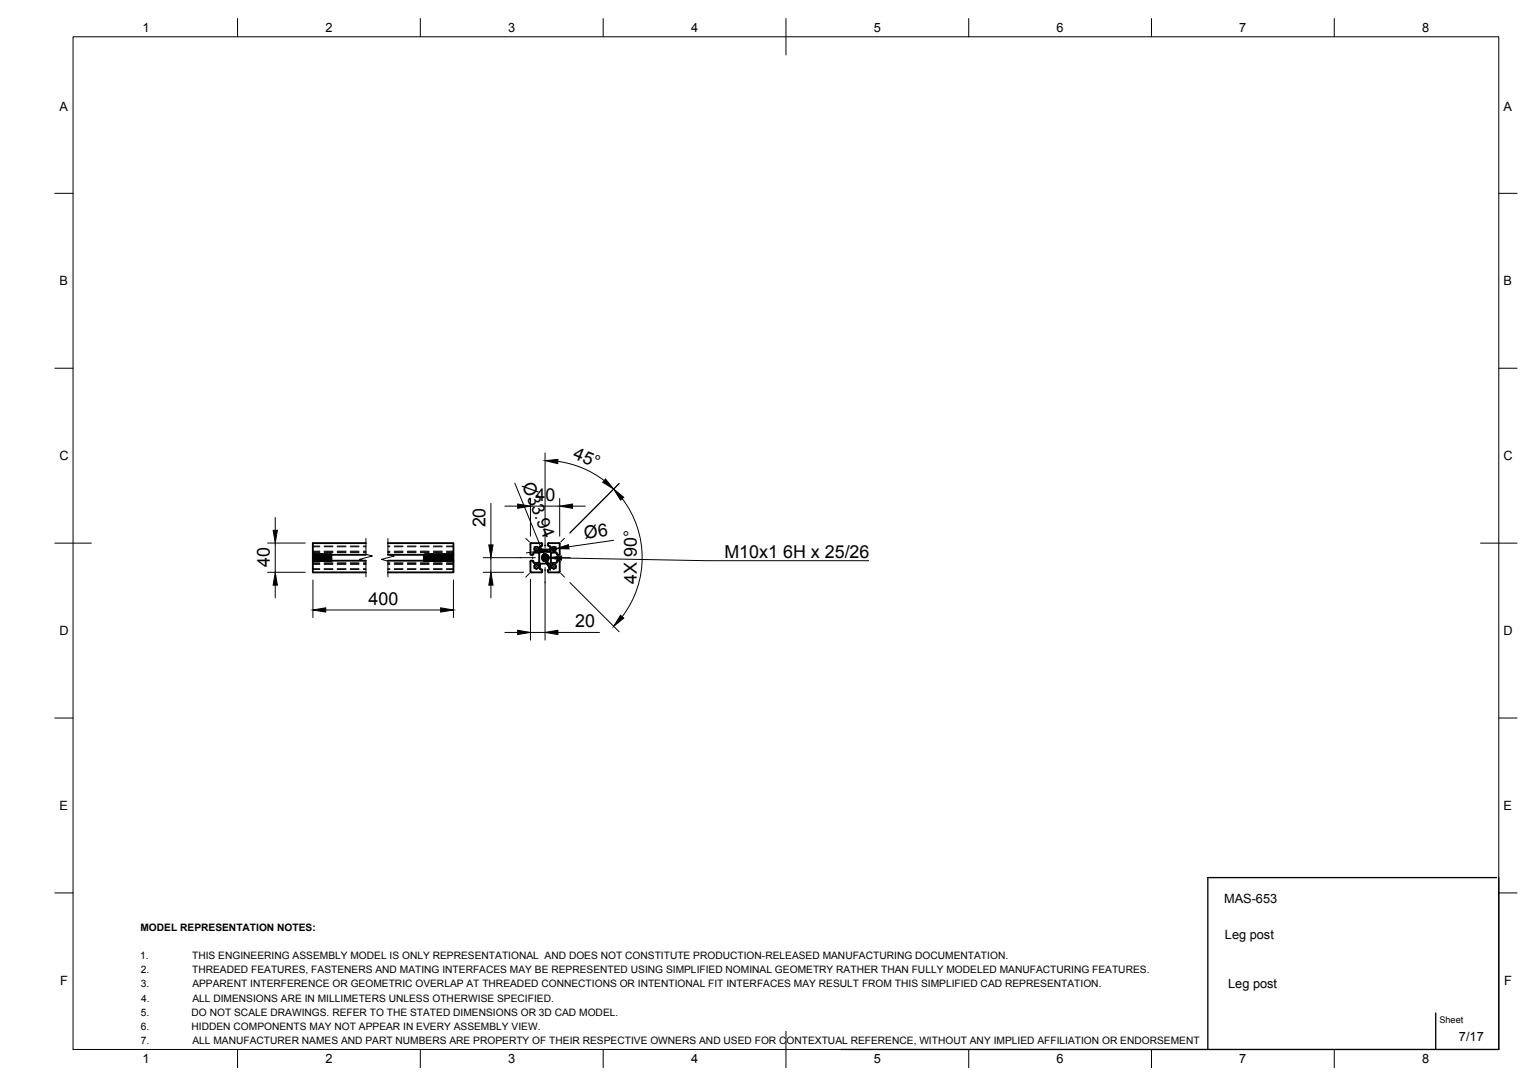
ISO-10303-21;
HEADER;
/* Generated by software containing ST-Developer
 * from STEP Tools, Inc. (www.steptools.com) 
 */

FILE_DESCRIPTION(
/* description */ ('Independent compact industrial fixture table, bolted aluminum worktop
 on connected adjustable support base. Whole-mm nominal dimensions. No
 load rating assigned.'),
/* implementation_level */ '2;1');

FILE_NAME(
/* name */ 'Leg post.step',
/* time_stamp */ '2026-11-07T17:47:58-08:00',
/* author */ (''),
/* organization */ (''),
/* preprocessor_version */ 'ST-DEVELOPER v20.2',
/* originating_system */ 'Autodesk Translation Framework v15.17.0.0',
/* authorisation */ '');

FILE_SCHEMA (('AUTOMOTIVE_DESIGN { 1 0 10303 214 3 1 1 }'));
ENDSEC;

DATA;
#10=MECHANICAL_DESIGN_GEOMETRIC_PRESENTATION_REPRESENTATION('',(#2255),#97475);
#344=B_SPLINE_SURFACE_WITH_KNOTS('',3,3,((#45406,#45407,#45408,#45409,#45410,
#45411,#45412,#45413,#45414,#45415,#45416,#45417,#45418,#45419,#45420,#45421,
#45422,#45423,#45424,#45425,#45426,#45427,#45428,#45429,#45430,#45431,#45432,
#45433,#45434,#45435,#45436,#45437,#45438,#45439,#45440,#45441,#45442,#45443,
#45444,#45445,#45446,#45447,#45448,#45449,#45450,#45451,#45452,#45453,#45454,
#45455,#45456,#45457,#45458,#45459,#45460,#45461,#45462,#45463,#45464,#45465,
#45466,#45467,#45468,#45469,#45470,#45471,#45472,#45473,#45474,#45475,#45476,
#45477,#45478,#45479,#45480,#45481,#45482,#45483,#45484,#45485,#45486,#45487,
#45488,#45489,#45490,#45491,#45492,#45493,#45494,#45495,#45496,#45497,#45498,
#45499,#45500,#45501,#45502,#45503,#45504,#45505,#45506,#45507,#45508,#45509,
#45510,#45511,#45512,#45513,#45514,#45515,#45516,#45517,#45518,#45519,#45520,
#45521,#45522,#45523,#45524,#45525,#45526,#45527,#45528,#45529,#45530,#45531,
#45532,#45533,#45534,#45535,#45536,#45537,#45538,#45539,#45540,#45541,#45542,
#45543,#45544,#45545,#45546,#45547,#45548,#45549,#45550,#45551,#45552,#45553,
#45554,#45555,#45556,#45557,#45558,#45559,#45560,#45561,#45562,#45563,#45564,
#45565,#45566,#45567,#45568,#45569,#45570,#45571,#45572,#45573,#45574,#45575,
#45576,#45577,#45578,#45579,#45580,#45581,#45582,#45583,#45584,#45585,#45586,
#45587,#45588,#45589,#45590,#45591,#45592,#45593,#45594,#45595,#45596,#45597,
#45598,#45599,#45600,#45601,#45602,#45603,#45604,#45605,#45606,#45607,#45608,
#45609,#45610,#45611,#45612,#45613,#45614,#45615,#45616,#45617,#45618,#45619,
#45620,#45621,#45622,#45623,#45624,#45625,#45626,#45627,#45628,#45629,#45630,
#45631,#45632,#45633,#45634,#45635,#45636,#45637,#45638,#45639,#45640,#45641,
#45642,#45643,#45644,#45645,#45646,#45647,#45648,#45649,#45650,#45651,#45652,
#45653,#45654,#45655,#45656,#45657,#45658,#45659,#45660,#45661,#45662,#45663,
#45664,#45665,#45666,#45667,#45668,#45669,#45670,#45671,#45672,#45673,#45674,
#45675,#45676,#45677,#45678,#45679,#45680,#45681,#45682,#45683,#45684,#45685,
#45686,#45687,#45688,#45689,#45690,#45691,#45692,#45693,#45694,#45695,#45696,
#45697,#45698,#45699,#45700,#45701,#45702,#45703,#45704,#45705,#45706,#45707,
#45708,#45709,#45710,#45711,#45712,#45713,#45714,#45715,#45716,#45717,#45718,
#45719,#45720,#45721,#45722,#45723,#45724,#45725,#45726,#45727,#45728,#45729,
#45730,#45731,#45732,#45733,#45734,#45735,#45736,#45737,#45738,#45739,#45740,
#45741,#45742,#45743,#45744,#45745,#45746,#45747,#45748,#45749,#45750,#45751,
#45752,#45753,#45754,#45755,#45756,#45757,#45758,#45759,#45760,#45761,#45762,
#45763,#45764,#45765,#45766,#45767,#45768,#45769,#45770,#45771,#45772,#45773,
#45774,#45775,#45776,#45777,#45778,#45779,#45780,#45781,#45782,#45783,#45784,
#45785,#45786,#45787,#45788,#45789,#45790,#45791,#45792,#45793,#45794,#45795,
#45796,#45797,#45798,#45799,#45800,#45801,#45802,#45803,#45804,#45805,#45806,
#45807,#45808,#45809,#45810,#45811,#45812,#45813,#45814,#45815,#45816,#45817,
#45818,#45819,#45820,#45821,#45822,#45823,#45824,#45825,#45826,#45827,#45828,
#45829,#45830,#45831,#45832,#45833,#45834,#45835,#45836,#45837,#45838,#45839,
#45840,#45841,#45842,#45843,#45844,#45845,#45846,#45847,#45848,#45849,#45850,
#45851,#45852,#45853,#45854,#45855,#45856,#45857,#45858,#45859,#45860,#45861,
#45862,#45863,#45864,#45865,#45866,#45867,#45868,#45869,#45870,#45871,#45872,
#45873,#45874,#45875,#45876,#45877,#45878,#45879,#45880,#45881,#45882,#45883,
#45884,#45885,#45886,#45887,#45888,#45889,#45890,#45891,#45892,#45893,#45894,
#45895,#45896,#45897,#45898,#45899,#45900,#45901,#45902),(#45903,#45904,
#45905,#45906,#45907,#45908,#45909,#45910,#45911,#45912,#45913,#45914,#45915,
#45916,#45917,#45918,#45919,#45920,#45921,#45922,#45923,#45924,#45925,#45926,
#45927,#45928,#45929,#45930,#45931,#45932,#45933,#45934,#45935,#45936,#45937,
#45938,#45939,#45940,#45941,#45942,#45943,#45944,#45945,#45946,#45947,#45948,
#45949,#45950,#45951,#45952,#45953,#45954,#45955,#45956,#45957,#45958,#45959,
#45960,#45961,#45962,#45963,#45964,#45965,#45966,#45967,#45968,#45969,#45970,
#45971,#45972,#45973,#45974,#45975,#45976,#45977,#45978,#45979,#45980,#45981,
#45982,#45983,#45984,#45985,#45986,#45987,#45988,#45989,#45990,#45991,#45992,
#45993,#45994,#45995,#45996,#45997,#45998,#45999,#46000,#46001,#46002,#46003,
#46004,#46005,#46006,#46007,#46008,#46009,#46010,#46011,#46012,#46013,#46014,
#46015,#46016,#46017,#46018,#46019,#46020,#46021,#46022,#46023,#46024,#46025,
#46026,#46027,#46028,#46029,#46030,#46031,#46032,#46033,#46034,#46035,#46036,
#46037,#46038,#46039,#46040,#46041,#46042,#46043,#46044,#46045,#46046,#46047,
#46048,#46049,#46050,#46051,#46052,#46053,#46054,#46055,#46056,#46057,#46058,
#46059,#46060,#46061,#46062,#46063,#46064,#46065,#46066,#46067,#46068,#46069,
#46070,#46071,#46072,#46073,#46074,#46075,#46076,#46077,#46078,#46079,#46080,
#46081,#46082,#46083,#46084,#46085,#46086,#46087,#46088,#46089,#46090,#46091,
#46092,#46093,#46094,#46095,#46096,#46097,#46098,#46099,#46100,#46101,#46102,
#46103,#46104,#46105,#46106,#46107,#46108,#46109,#46110,#46111,#46112,#46113,
#46114,#46115,#46116,#46117,#46118,#46119,#46120,#46121,#46122,#46123,#46124,
#46125,#46126,#46127,#46128,#46129,#46130,#46131,#46132,#46133,#46134,#46135,
#46136,#46137,#46138,#46139,#46140,#46141,#46142,#46143,#46144,#46145,#46146,
#46147,#46148,#46149,#46150,#46151,#46152,#46153,#46154,#46155,#46156,#46157,
#46158,#46159,#46160,#46161,#46162,#46163,#46164,#46165,#46166,#46167,#46168,
#46169,#46170,#46171,#46172,#46173,#46174,#46175,#46176,#46177,#46178,#46179,
#46180,#46181,#46182,#46183,#46184,#46185,#46186,#46187,#46188,#46189,#46190,
#46191,#46192,#46193,#46194,#46195,#46196,#46197,#46198,#46199,#46200,#46201,
#46202,#46203,#46204,#46205,#46206,#46207,#46208,#46209,#46210,#46211,#46212,
#46213,#46214,#46215,#46216,#46217,#46218,#46219,#46220,#46221,#46222,#46223,
#46224,#46225,#46226,#46227,#46228,#46229,#46230,#46231,#46232,#46233,#46234,
#46235,#46236,#46237,#46238,#46239,#46240,#46241,#46242,#46243,#46244,#46245,
#46246,#46247,#46248,#46249,#46250,#46251,#46252,#46253,#46254,#46255,#46256,
#46257,#46258,#46259,#46260,#46261,#46262,#46263,#46264,#46265,#46266,#46267,
#46268,#46269,#46270,#46271,#46272,#46273,#46274,#46275,#46276,#46277,#46278,
#46279,#46280,#46281,#46282,#46283,#46284,#46285,#46286,#46287,#46288,#46289,
#46290,#46291,#46292,#46293,#46294,#46295,#46296,#46297,#46298,#46299,#46300,
#46301,#46302,#46303,#46304,#46305,#46306,#46307,#46308,#46309,#46310,#46311,
#46312,#46313,#46314,#46315,#46316,#46317,#46318,#46319,#46320,#46321,#46322,
#46323,#46324,#46325,#46326,#46327,#46328,#46329,#46330,#46331,#46332,#46333,
#46334,#46335,#46336,#46337,#46338,#46339,#46340,#46341,#46342,#46343,#46344,
#46345,#46346,#46347,#46348,#46349,#46350,#46351,#46352,#46353,#46354,#46355,
#46356,#46357,#46358,#46359,#46360,#46361,#46362,#46363,#46364,#46365,#46366,
#46367,#46368,#46369,#46370,#46371,#46372,#46373,#46374,#46375,#46376,#46377,
#46378,#46379,#46380,#46381,#46382,#46383,#46384,#46385,#46386,#46387,#46388,
#46389,#46390,#46391,#46392,#46393,#46394,#46395,#46396,#46397,#46398,#46399),
(#46400,#46401,#46402,#46403,#46404,#46405,#46406,#46407,#46408,#46409,
#46410,#46411,#46412,#46413,#46414,#46415,#46416,#46417,#46418,#46419,#46420,
#46421,#46422,#46423,#46424,#46425,#46426,#46427,#46428,#46429,#46430,#46431,
#46432,#46433,#46434,#46435,#46436,#46437,#46438,#46439,#46440,#46441,#46442,
#46443,#46444,#46445,#46446,#46447,#46448,#46449,#46450,#46451,#46452,#46453,
#46454,#46455,#46456,#46457,#46458,#46459,#46460,#46461,#46462,#46463,#46464,
#46465,#46466,#46467,#46468,#46469,#46470,#46471,#46472,#46473,#46474,#46475,
#46476,#46477,#46478,#46479,#46480,#46481,#46482,#46483,#46484,#46485,#46486,
#46487,#46488,#46489,#46490,#46491,#46492,#46493,#46494,#46495,#46496,#46497,
#46498,#46499,#46500,#46501,#46502,#46503,#46504,#46505,#46506,#46507,#46508,
#46509,#46510,#46511,#46512,#46513,#46514,#46515,#46516,#46517,#46518,#46519,
#46520,#46521,#46522,#46523,#46524,#46525,#46526,#46527,#46528,#46529,#46530,
#46531,#46532,#46533,#46534,#46535,#46536,#46537,#46538,#46539,#46540,#46541,
#46542,#46543,#46544,#46545,#46546,#46547,#46548,#46549,#46550,#46551,#46552,
#46553,#46554,#46555,#46556,#46557,#46558,#46559,#46560,#46561,#46562,#46563,
#46564,#46565,#46566,#46567,#46568,#46569,#46570,#46571,#46572,#46573,#46574,
#46575,#46576,#46577,#46578,#46579,#46580,#46581,#46582,#46583,#46584,#46585,
#46586,#46587,#46588,#46589,#46590,#46591,#46592,#46593,#46594,#46595,#46596,
#46597,#46598,#46599,#46600,#46601,#46602,#46603,#46604,#46605,#46606,#46607,
#46608,#46609,#46610,#46611,#46612,#46613,#46614,#46615,#46616,#46617,#46618,
#46619,#46620,#46621,#46622,#46623,#46624,#46625,#46626,#46627,#46628,#46629,
#46630,#46631,#46632,#46633,#46634,#46635,#46636,#46637,#46638,#46639,#46640,
#46641,#46642,#46643,#46644,#46645,#46646,#46647,#46648,#46649,#46650,#46651,
#46652,#46653,#46654,#46655,#46656,#46657,#46658,#46659,#46660,#46661,#46662,
#46663,#46664,#46665,#46666,#46667,#46668,#46669,#46670,#46671,#46672,#46673,
#46674,#46675,#46676,#46677,#46678,#46679,#46680,#46681,#46682,#46683,#46684,
#46685,#46686,#46687,#46688,#46689,#46690,#46691,#46692,#46693,#46694,#46695,
#46696,#46697,#46698,#46699,#46700,#46701,#46702,#46703,#46704,#46705,#46706,
#46707,#46708,#46709,#46710,#46711,#46712,#46713,#46714,#46715,#46716,#46717,
#46718,#46719,#46720,#46721,#46722,#46723,#46724,#46725,#46726,#46727,#46728,
#46729,#46730,#46731,#46732,#46733,#46734,#46735,#46736,#46737,#46738,#46739,
#46740,#46741,#46742,#46743,#46744,#46745,#46746,#46747,#46748,#46749,#46750,
#46751,#46752,#46753,#46754,#46755,#46756,#46757,#46758,#46759,#46760,#46761,
#46762,#46763,#46764,#46765,#46766,#46767,#46768,#46769,#46770,#46771,#46772,
#46773,#46774,#46775,#46776,#46777,#46778,#46779,#46780,#46781,#46782,#46783,
#46784,#46785,#46786,#46787,#46788,#46789,#46790,#46791,#46792,#46793,#46794,
#46795,#46796,#46797,#46798,#46799,#46800,#46801,#46802,#46803,#46804,#46805,
#46806,#46807,#46808,#46809,#46810,#46811,#46812,#46813,#46814,#46815,#46816,
#46817,#46818,#46819,#46820,#46821,#46822,#46823,#46824,#46825,#46826,#46827,
#46828,#46829,#46830,#46831,#46832,#46833,#46834,#46835,#46836,#46837,#46838,
#46839,#46840,#46841,#46842,#46843,#46844,#46845,#46846,#46847,#46848,#46849,
#46850,#46851,#46852,#46853,#46854,#46855,#46856,#46857,#46858,#46859,#46860,
#46861,#46862,#46863,#46864,#46865,#46866,#46867,#46868,#46869,#46870,#46871,
#46872,#46873,#46874,#46875,#46876,#46877,#46878,#46879,#46880,#46881,#46882,
#46883,#46884,#46885,#46886,#46887,#46888,#46889,#46890,#46891,#46892,#46893,
#46894,#46895,#46896),(#46897,#46898,#46899,#46900,#46901,#46902,#46903,
#46904,#46905,#46906,#46907,#46908,#46909,#46910,#46911,#46912,#46913,#46914,
#46915,#46916,#46917,#46918,#46919,#46920,#46921,#46922,#46923,#46924,#46925,
#46926,#46927,#46928,#46929,#46930,#46931,#46932,#46933,#46934,#46935,#46936,
#46937,#46938,#46939,#46940,#46941,#46942,#46943,#46944,#46945,#46946,#46947,
#46948,#46949,#46950,#46951,#46952,#46953,#46954,#46955,#46956,#46957,#46958,
#46959,#46960,#46961,#46962,#46963,#46964,#46965,#46966,#46967,#46968,#46969,
#46970,#46971,#46972,#46973,#46974,#46975,#46976,#46977,#46978,#46979,#46980,
#46981,#46982,#46983,#46984,#46985,#46986,#46987,#46988,#46989,#46990,#46991,
#46992,#46993,#46994,#46995,#46996,#46997,#46998,#46999,#47000,#47001,#47002,
#47003,#47004,#47005,#47006,#47007,#47008,#47009,#47010,#47011,#47012,#47013,
#47014,#47015,#47016,#47017,#47018,#47019,#47020,#47021,#47022,#47023,#47024,
#47025,#47026,#47027,#47028,#47029,#47030,#47031,#47032,#47033,#47034,#47035,
#47036,#47037,#47038,#47039,#47040,#47041,#47042,#47043,#47044,#47045,#47046,
#47047,#47048,#47049,#47050,#47051,#47052,#47053,#47054,#47055,#47056,#47057,
#47058,#47059,#47060,#47061,#47062,#47063,#47064,#47065,#47066,#47067,#47068,
#47069,#47070,#47071,#47072,#47073,#47074,#47075,#47076,#47077,#47078,#47079,
#47080,#47081,#47082,#47083,#47084,#47085,#47086,#47087,#47088,#47089,#47090,
#47091,#47092,#47093,#47094,#47095,#47096,#47097,#47098,#47099,#47100,#47101,
#47102,#47103,#47104,#47105,#47106,#47107,#47108,#47109,#47110,#47111,#47112,
#47113,#47114,#47115,#47116,#47117,#47118,#47119,#47120,#47121,#47122,#47123,
#47124,#47125,#47126,#47127,#47128,#47129,#47130,#47131,#47132,#47133,#47134,
#47135,#47136,#47137,#47138,#47139,#47140,#47141,#47142,#47143,#47144,#47145,
#47146,#47147,#47148,#47149,#47150,#47151,#47152,#47153,#47154,#47155,#47156,
#47157,#47158,#47159,#47160,#47161,#47162,#47163,#47164,#47165,#47166,#47167,
#47168,#47169,#47170,#47171,#47172,#47173,#47174,#47175,#47176,#47177,#47178,
#47179,#47180,#47181,#47182,#47183,#47184,#47185,#47186,#47187,#47188,#47189,
#47190,#47191,#47192,#47193,#47194,#47195,#47196,#47197,#47198,#47199,#47200,
#47201,#47202,#47203,#47204,#47205,#47206,#47207,#47208,#47209,#47210,#47211,
#47212,#47213,#47214,#47215,#47216,#47217,#47218,#47219,#47220,#47221,#47222,
#47223,#47224,#47225,#47226,#47227,#47228,#47229,#47230,#47231,#47232,#47233,
#47234,#47235,#47236,#47237,#47238,#47239,#47240,#47241,#47242,#47243,#47244,
#47245,#47246,#47247,#47248,#47249,#47250,#47251,#47252,#47253,#47254,#47255,
#47256,#47257,#47258,#47259,#47260,#47261,#47262,#47263,#47264,#47265,#47266,
#47267,#47268,#47269,#47270,#47271,#47272,#47273,#47274,#47275,#47276,#47277,
#47278,#47279,#47280,#47281,#47282,#47283,#47284,#47285,#47286,#47287,#47288,
#47289,#47290,#47291,#47292,#47293,#47294,#47295,#47296,#47297,#47298,#47299,
#47300,#47301,#47302,#47303,#47304,#47305,#47306,#47307,#47308,#47309,#47310,
#47311,#47312,#47313,#47314,#47315,#47316,#47317,#47318,#47319,#47320,#47321,
#47322,#47323,#47324,#47325,#47326,#47327,#47328,#47329,#47330,#47331,#47332,
#47333,#47334,#47335,#47336,#47337,#47338,#47339,#47340,#47341,#47342,#47343,
#47344,#47345,#47346,#47347,#47348,#47349,#47350,#47351,#47352,#47353,#47354,
#47355,#47356,#47357,#47358,#47359,#47360,#47361,#47362,#47363,#47364,#47365,
#47366,#47367,#47368,#47369,#47370,#47371,#47372,#47373,#47374,#47375,#47376,
#47377,#47378,#47379,#47380,#47381,#47382,#47383,#47384,#47385,#47386,#47387,
#47388,#47389,#47390,#47391,#47392,#47393)),.UNSPECIFIED.,.F.,.F.,.F.,(4,
4),(4,1,1,1,1,1,1,1,1,1,1,1,1,1,1,1,1,1,1,1,1,1,1,1,1,1,1,1,1,1,1,1,1,1,
1,1,1,1,1,1,1,1,1,1,1,1,1,1,1,1,1,1,1,1,1,1,1,1,1,1,1,1,1,1,1,1,1,1,1,1,
1,1,1,1,1,1,1,1,1,1,1,1,1,1,1,1,1,1,1,1,1,1,1,1,1,1,1,1,1,1,1,1,1,1,1,1,
1,1,1,1,1,1,1,1,1,1,1,1,1,1,1,1,1,1,1,1,1,1,1,1,1,1,1,1,1,1,1,1,1,1,1,1,
1,1,1,1,1,1,1,1,1,1,1,1,1,1,1,1,1,1,1,1,1,1,1,1,1,1,1,1,1,1,1,1,1,1,1,1,
1,1,1,1,1,1,1,1,1,1,1,1,1,1,1,1,1,1,1,1,1,1,1,1,1,1,1,1,1,1,1,1,1,1,1,1,
1,1,1,1,1,1,1,1,1,1,1,1,1,1,1,1,1,1,1,1,1,1,1,1,1,1,1,1,1,1,1,1,1,1,1,1,
1,1,1,1,1,1,1,1,1,1,1,1,1,1,1,1,1,1,1,1,1,1,1,1,1,1,1,1,1,1,1,1,1,1,1,1,
1,1,1,1,1,1,1,1,1,1,1,1,1,1,1,1,1,1,1,1,1,1,1,1,1,1,1,1,1,1,1,1,1,1,1,1,
1,1,1,1,1,1,1,1,1,1,1,1,1,1,1,1,1,1,1,1,1,1,1,1,1,1,1,1,1,1,1,1,1,1,1,1,
1,1,1,1,1,1,1,1,1,1,1,1,1,1,1,1,1,1,1,1,1,1,1,1,1,1,1,1,1,1,1,1,1,1,1,1,
1,1,1,1,1,1,1,1,1,1,1,1,1,1,1,1,1,1,1,1,1,1,1,1,1,1,1,1,1,1,1,1,1,1,1,1,
1,1,1,1,1,1,1,1,1,1,1,1,1,1,1,1,1,1,1,1,1,1,1,1,1,1,1,1,1,1,1,1,1,1,1,1,
1,1,1,1,1,1,1,1,1,1,1,1,1,1,1,1,1,1,1,1,1,1,1,1,1,1,1,1,4),(0.,0.0641840294258107),
(11.8589888623082,12.3576971556948,12.8564054490814,13.355113742468,13.8538220358547,
14.3525303292413,14.8512386226279,15.3499469160145,15.8486552094011,16.3473635027878,
16.8460717961744,17.344780089561,17.8434883829476,18.3421966763342,18.8409049697209,
19.3396132631075,19.8383215564941,20.3370298498807,20.8357381432673,21.334446436654,
21.8331547300406,22.3318630234272,22.8305713168138,23.3292796102004,23.8279879035871,
24.3266961969737,24.8254044903603,25.3241127837469,25.8228210771335,26.3215293705201,
26.8202376639068,27.3189459572934,27.81765425068,28.3163625440666,28.8150708374532,
29.3137791308399,29.8124874242265,30.3111957176131,30.8099040109997,31.3086123043863,
31.807320597773,32.3060288911596,32.8047371845462,33.3034454779328,33.8021537713194,
34.3008620647061,34.7995703580927,35.2982786514793,35.7969869448659,36.2956952382525,
36.7944035316392,37.2931118250258,37.7918201184124,38.290528411799,38.7892367051856,
39.2879449985723,39.7866532919589,40.2853615853455,40.7840698787321,41.2827781721187,
41.7814864655054,42.280194758892,42.7789030522786,43.2776113456652,43.7763196390518,
44.2750279324384,44.7737362258251,45.2724445192117,45.7711528125983,46.2698611059849,
46.7685693993716,47.2672776927582,47.7659859861448,48.2646942795314,48.763402572918,
49.2621108663046,49.7608191596913,50.2595274530779,50.7582357464645,51.2569440398511,
51.7556523332377,52.2543606266244,52.753068920011,53.2517772133976,53.7504855067842,
54.2491938001708,54.7479020935575,55.2466103869441,55.7453186803307,56.2440269737173,
56.7427352671039,57.2414435604906,57.7401518538772,58.2388601472638,58.7375684406504,
59.236276734037,59.7349850274237,60.2336933208103,60.7324016141969,61.2311099075835,
61.7298182009701,62.2285264943567,62.7272347877434,63.22594308113,63.7246513745166,
64.2233596679032,64.7220679612898,65.2207762546765,65.7194845480631,66.2181928414497,
66.7169011348363,67.2156094282229,67.7143177216096,68.2130260149962,68.7117343083828,
69.2104426017694,69.709150895156,70.2078591885427,70.7065674819293,71.2052757753159,
71.7039840687025,72.2026923620891,72.7014006554758,73.2001089488624,73.698817242249,
74.1975255356356,74.6962338290222,75.1949421224089,75.6936504157955,76.1923587091821,
76.6910670025687,77.1897752959553,77.6884835893419,78.1871918827286,78.6859001761152,
79.1846084695018,79.6833167628884,80.1820250562751,80.6807333496617,81.1794416430483,
81.6781499364349,82.1768582298215,82.6755665232081,83.1742748165948,83.6729831099814,
84.171691403368,84.6703996967546,85.1691079901412,85.6678162835279,86.1665245769145,
86.6652328703011,87.1639411636877,87.6626494570743,88.161357750461,88.6600660438476,
89.1587743372342,89.6574826306208,90.1561909240074,90.654899217394,91.1536075107807,
91.6523158041673,92.1510240975539,92.6497323909405,93.1484406843271,93.6471489777138,
94.1458572711004,94.644565564487,95.1432738578736,95.6419821512603,96.1406904446469,
96.6393987380335,97.1381070314201,97.6368153248067,98.1355236181933,98.63423191158,
99.1329402049666,99.6316484983532,100.13035679174,100.629065085126,101.127773378513,
101.6264816719,102.125189965286,102.623898258673,103.12260655206,103.621314845446,
104.120023138833,104.618731432219,105.117439725606,105.616148018993,106.114856312379,
106.613564605766,107.112272899152,107.610981192539,108.109689485926,108.608397779312,
109.107106072699,109.605814366086,110.104522659472,110.603230952859,111.101939246245,
111.600647539632,112.099355833019,112.598064126405,113.096772419792,113.595480713179,
114.094189006565,114.592897299952,115.091605593338,115.590313886725,116.089022180112,
116.587730473498,117.086438766885,117.585147060271,118.083855353658,118.582563647045,
119.081271940431,119.579980233818,120.078688527205,120.577396820591,121.076105113978,
121.574813407364,122.073521700751,122.572229994138,123.070938287524,123.569646580911,
124.068354874298,124.567063167684,125.065771461071,125.564479754457,126.063188047844,
126.561896341231,127.060604634617,127.559312928004,128.058021221391,128.556729514777,
129.055437808164,129.55414610155,130.052854394937,130.551562688324,131.05027098171,
131.548979275097,132.54639586187,133.543812448643,134.541229035417,135.53864562219,
136.536062208963,137.533478795736,138.53089538251,139.528311969283,140.525728556056,
141.523145142829,142.520561729602,143.517978316376,144.515394903149,145.512811489922,
146.011519783309,146.510228076695,147.008936370082,147.507644663469,148.006352956855,
148.505061250242,149.003769543629,149.502477837015,150.001186130402,150.499894423788,
150.998602717175,151.497311010562,151.996019303948,152.494727597335,152.993435890721,
153.492144184108,153.990852477495,154.489560770881,154.988269064268,155.486977357655,
155.985685651041,156.484393944428,156.983102237814,157.481810531201,157.980518824588,
158.479227117974,158.977935411361,159.476643704748,159.975351998134,160.474060291521,
160.972768584907,161.471476878294,161.970185171681,162.468893465067,162.967601758454,
163.466310051841,163.965018345227,164.463726638614,164.962434932,165.461143225387,
165.959851518774,166.45855981216,166.957268105547,167.455976398933,167.95468469232,
168.453392985707,168.952101279093,169.45080957248,169.949517865867,170.448226159253,
170.94693445264,171.445642746026,171.944351039413,172.4430593328,172.941767626186,
173.440475919573,173.93918421296,174.437892506346,174.936600799733,175.435309093119,
175.934017386506,176.432725679893,176.931433973279,177.430142266666,177.928850560052,
178.427558853439,178.926267146826,179.424975440212,179.923683733599,180.422392026986,
180.921100320372,181.419808613759,181.918516907145,182.417225200532,182.915933493919,
183.414641787305,183.913350080692,184.412058374079,184.910766667465,185.409474960852,
185.908183254238,186.406891547625,186.905599841012,187.404308134398,187.903016427785,
188.401724721171,188.900433014558,189.399141307945,189.897849601331,190.396557894718,
190.895266188105,191.393974481491,191.892682774878,192.391391068264,192.890099361651,
193.388807655038,193.887515948424,194.386224241811,194.884932535198,195.383640828584,
195.882349121971,196.381057415357,196.879765708744,197.378474002131,197.877182295517,
198.375890588904,198.87459888229,199.373307175677,199.872015469064,200.37072376245,
200.869432055837,201.368140349224,201.86684864261,202.365556935997,202.864265229383,
203.36297352277,203.861681816157,204.360390109543,204.85909840293,205.357806696317,
205.856514989703,206.35522328309,206.853931576476,207.352639869863,207.85134816325,
208.350056456636,208.848764750023,209.347473043409,209.846181336796,210.344889630183,
210.843597923569,211.342306216956,211.841014510343,212.339722803729,212.838431097116,
213.337139390502,213.835847683889,214.334555977276,214.833264270662,215.331972564049,
215.830680857436,216.329389150822,216.828097444209,217.326805737595,217.825514030982,
218.324222324369,218.822930617755,219.321638911142,219.820347204529,220.319055497915,
220.817763791302,221.316472084688,221.815180378075,222.313888671462,222.812596964848,
223.311305258235,223.810013551621,224.308721845008,224.807430138395,225.306138431781,
225.804846725168,226.303555018555,226.802263311941,227.300971605328,227.799679898714,
228.298388192101,228.797096485488,229.295804778874,229.794513072261,230.293221365647,
230.791929659034,231.290637952421,231.789346245807,232.288054539194,232.786762832581,
233.285471125967,233.784179419354,234.28288771274,234.781596006127,235.280304299514,
235.7790125929,236.277720886287,236.776429179674,237.27513747306,237.773845766447,
238.272554059833,238.77126235322,239.269970646607,239.768678939993,240.26738723338,
240.766095526767,241.264803820153,241.76351211354,242.262220406926,242.760928700313,
243.2596369937,243.758345287086,244.257053580473,244.755761873859,245.254470167246,
245.753178460633,246.251886754019,246.750595047406,247.249303340793,247.748011634179,
248.246719927566,248.745428220952,249.244136514339,249.742844807726,250.241553101112,
250.740261394499,251.238969687886,251.737677981272,252.236386274659,252.735094568045,
253.233802861432,253.732511154819,254.231219448205,254.729927741592,255.228636034978,
255.727344328365,256.226052621752,256.724760915138,257.223469208525,257.722177501912,
258.220885795298,258.719594088685,259.218302382071,259.717010675458,260.215718968845,
260.714427262231,261.213135555618,261.711843849004,262.210552142391,262.709260435778,
263.207968729164,263.706677022551,264.205385315938,264.704093609324,265.202801902711),
 .UNSPECIFIED.);
#345=B_SPLINE_SURFACE_WITH_KNOTS('',3,3,((#47543,#47544,#47545,#47546,#47547,
#47548,#47549,#47550,#47551,#47552,#47553,#47554,#47555,#47556,#47557,#47558,
#47559,#47560,#47561,#47562,#47563,#47564,#47565,#47566,#47567,#47568,#47569,
#47570,#47571,#47572,#47573,#47574,#47575,#47576,#47577,#47578,#47579,#47580,
#47581,#47582,#47583,#47584,#47585,#47586,#47587,#47588,#47589,#47590,#47591,
#47592,#47593,#47594,#47595,#47596,#47597,#47598,#47599,#47600,#47601,#47602,
#47603,#47604,#47605,#47606,#47607,#47608,#47609,#47610,#47611,#47612,#47613,
#47614,#47615,#47616,#47617,#47618,#47619,#47620,#47621,#47622,#47623,#47624,
#47625,#47626,#47627,#47628,#47629,#47630,#47631,#47632,#47633,#47634,#47635,
#47636,#47637,#47638,#47639,#47640,#47641,#47642,#47643,#47644,#47645,#47646,
#47647,#47648,#47649,#47650,#47651,#47652,#47653,#47654,#47655,#47656,#47657,
#47658,#47659,#47660,#47661,#47662,#47663,#47664,#47665,#47666,#47667,#47668,
#47669,#47670,#47671,#47672,#47673,#47674,#47675,#47676,#47677,#47678,#47679,
#47680,#47681,#47682,#47683,#47684,#47685,#47686,#47687,#47688,#47689,#47690,
#47691,#47692,#47693,#47694,#47695,#47696,#47697,#47698,#47699,#47700,#47701,
#47702,#47703,#47704,#47705,#47706,#47707,#47708,#47709,#47710,#47711,#47712,
#47713,#47714,#47715,#47716,#47717,#47718,#47719,#47720,#47721,#47722,#47723,
#47724,#47725,#47726,#47727,#47728,#47729,#47730,#47731,#47732,#47733,#47734,
#47735,#47736,#47737,#47738,#47739,#47740,#47741,#47742,#47743,#47744,#47745,
#47746,#47747,#47748,#47749,#47750,#47751,#47752,#47753,#47754,#47755,#47756,
#47757,#47758,#47759,#47760,#47761,#47762,#47763,#47764,#47765,#47766,#47767,
#47768,#47769,#47770,#47771,#47772,#47773,#47774,#47775,#47776,#47777,#47778,
#47779,#47780,#47781,#47782,#47783,#47784,#47785,#47786,#47787,#47788,#47789,
#47790,#47791,#47792,#47793,#47794,#47795,#47796,#47797,#47798,#47799,#47800,
#47801,#47802,#47803,#47804,#47805,#47806,#47807,#47808,#47809,#47810,#47811,
#47812,#47813,#47814,#47815,#47816,#47817,#47818,#47819,#47820,#47821,#47822,
#47823,#47824,#47825,#47826,#47827,#47828,#47829,#47830,#47831,#47832,#47833,
#47834,#47835,#47836,#47837,#47838,#47839,#47840,#47841,#47842,#47843,#47844,
#47845,#47846,#47847,#47848,#47849,#47850,#47851,#47852,#47853,#47854,#47855,
#47856,#47857,#47858,#47859,#47860,#47861,#47862,#47863,#47864,#47865,#47866,
#47867,#47868,#47869,#47870,#47871,#47872,#47873,#47874,#47875,#47876,#47877,
#47878,#47879,#47880,#47881,#47882,#47883,#47884,#47885,#47886,#47887,#47888,
#47889,#47890,#47891,#47892,#47893,#47894,#47895,#47896,#47897,#47898,#47899,
#47900,#47901,#47902,#47903,#47904,#47905,#47906,#47907,#47908,#47909,#47910,
#47911,#47912,#47913,#47914,#47915,#47916,#47917,#47918,#47919,#47920,#47921,
#47922,#47923,#47924,#47925,#47926,#47927,#47928,#47929,#47930,#47931,#47932,
#47933,#47934,#47935,#47936,#47937,#47938,#47939,#47940,#47941,#47942,#47943,
#47944,#47945,#47946,#47947,#47948,#47949,#47950,#47951,#47952,#47953,#47954,
#47955,#47956,#47957,#47958,#47959,#47960,#47961,#47962,#47963,#47964,#47965,
#47966,#47967,#47968,#47969,#47970,#47971,#47972,#47973,#47974,#47975,#47976,
#47977,#47978,#47979,#47980,#47981,#47982,#47983,#47984,#47985,#47986,#47987,
#47988,#47989,#47990,#47991,#47992,#47993,#47994,#47995,#47996,#47997,#47998,
#47999,#48000,#48001,#48002,#48003,#48004,#48005,#48006,#48007,#48008,#48009,
#48010,#48011,#48012,#48013,#48014,#48015,#48016,#48017,#48018,#48019,#48020,
#48021,#48022,#48023,#48024,#48025,#48026,#48027,#48028,#48029,#48030,#48031,
#48032,#48033,#48034,#48035,#48036,#48037,#48038,#48039),(#48040,#48041,
#48042,#48043,#48044,#48045,#48046,#48047,#48048,#48049,#48050,#48051,#48052,
#48053,#48054,#48055,#48056,#48057,#48058,#48059,#48060,#48061,#48062,#48063,
#48064,#48065,#48066,#48067,#48068,#48069,#48070,#48071,#48072,#48073,#48074,
#48075,#48076,#48077,#48078,#48079,#48080,#48081,#48082,#48083,#48084,#48085,
#48086,#48087,#48088,#48089,#48090,#48091,#48092,#48093,#48094,#48095,#48096,
#48097,#48098,#48099,#48100,#48101,#48102,#48103,#48104,#48105,#48106,#48107,
#48108,#48109,#48110,#48111,#48112,#48113,#48114,#48115,#48116,#48117,#48118,
#48119,#48120,#48121,#48122,#48123,#48124,#48125,#48126,#48127,#48128,#48129,
#48130,#48131,#48132,#48133,#48134,#48135,#48136,#48137,#48138,#48139,#48140,
#48141,#48142,#48143,#48144,#48145,#48146,#48147,#48148,#48149,#48150,#48151,
#48152,#48153,#48154,#48155,#48156,#48157,#48158,#48159,#48160,#48161,#48162,
#48163,#48164,#48165,#48166,#48167,#48168,#48169,#48170,#48171,#48172,#48173,
#48174,#48175,#48176,#48177,#48178,#48179,#48180,#48181,#48182,#48183,#48184,
#48185,#48186,#48187,#48188,#48189,#48190,#48191,#48192,#48193,#48194,#48195,
#48196,#48197,#48198,#48199,#48200,#48201,#48202,#48203,#48204,#48205,#48206,
#48207,#48208,#48209,#48210,#48211,#48212,#48213,#48214,#48215,#48216,#48217,
#48218,#48219,#48220,#48221,#48222,#48223,#48224,#48225,#48226,#48227,#48228,
#48229,#48230,#48231,#48232,#48233,#48234,#48235,#48236,#48237,#48238,#48239,
#48240,#48241,#48242,#48243,#48244,#48245,#48246,#48247,#48248,#48249,#48250,
#48251,#48252,#48253,#48254,#48255,#48256,#48257,#48258,#48259,#48260,#48261,
#48262,#48263,#48264,#48265,#48266,#48267,#48268,#48269,#48270,#48271,#48272,
#48273,#48274,#48275,#48276,#48277,#48278,#48279,#48280,#48281,#48282,#48283,
#48284,#48285,#48286,#48287,#48288,#48289,#48290,#48291,#48292,#48293,#48294,
#48295,#48296,#48297,#48298,#48299,#48300,#48301,#48302,#48303,#48304,#48305,
#48306,#48307,#48308,#48309,#48310,#48311,#48312,#48313,#48314,#48315,#48316,
#48317,#48318,#48319,#48320,#48321,#48322,#48323,#48324,#48325,#48326,#48327,
#48328,#48329,#48330,#48331,#48332,#48333,#48334,#48335,#48336,#48337,#48338,
#48339,#48340,#48341,#48342,#48343,#48344,#48345,#48346,#48347,#48348,#48349,
#48350,#48351,#48352,#48353,#48354,#48355,#48356,#48357,#48358,#48359,#48360,
#48361,#48362,#48363,#48364,#48365,#48366,#48367,#48368,#48369,#48370,#48371,
#48372,#48373,#48374,#48375,#48376,#48377,#48378,#48379,#48380,#48381,#48382,
#48383,#48384,#48385,#48386,#48387,#48388,#48389,#48390,#48391,#48392,#48393,
#48394,#48395,#48396,#48397,#48398,#48399,#48400,#48401,#48402,#48403,#48404,
#48405,#48406,#48407,#48408,#48409,#48410,#48411,#48412,#48413,#48414,#48415,
#48416,#48417,#48418,#48419,#48420,#48421,#48422,#48423,#48424,#48425,#48426,
#48427,#48428,#48429,#48430,#48431,#48432,#48433,#48434,#48435,#48436,#48437,
#48438,#48439,#48440,#48441,#48442,#48443,#48444,#48445,#48446,#48447,#48448,
#48449,#48450,#48451,#48452,#48453,#48454,#48455,#48456,#48457,#48458,#48459,
#48460,#48461,#48462,#48463,#48464,#48465,#48466,#48467,#48468,#48469,#48470,
#48471,#48472,#48473,#48474,#48475,#48476,#48477,#48478,#48479,#48480,#48481,
#48482,#48483,#48484,#48485,#48486,#48487,#48488,#48489,#48490,#48491,#48492,
#48493,#48494,#48495,#48496,#48497,#48498,#48499,#48500,#48501,#48502,#48503,
#48504,#48505,#48506,#48507,#48508,#48509,#48510,#48511,#48512,#48513,#48514,
#48515,#48516,#48517,#48518,#48519,#48520,#48521,#48522,#48523,#48524,#48525,
#48526,#48527,#48528,#48529,#48530,#48531,#48532,#48533,#48534,#48535,#48536),
(#48537,#48538,#48539,#48540,#48541,#48542,#48543,#48544,#48545,#48546,
#48547,#48548,#48549,#48550,#48551,#48552,#48553,#48554,#48555,#48556,#48557,
#48558,#48559,#48560,#48561,#48562,#48563,#48564,#48565,#48566,#48567,#48568,
#48569,#48570,#48571,#48572,#48573,#48574,#48575,#48576,#48577,#48578,#48579,
#48580,#48581,#48582,#48583,#48584,#48585,#48586,#48587,#48588,#48589,#48590,
#48591,#48592,#48593,#48594,#48595,#48596,#48597,#48598,#48599,#48600,#48601,
#48602,#48603,#48604,#48605,#48606,#48607,#48608,#48609,#48610,#48611,#48612,
#48613,#48614,#48615,#48616,#48617,#48618,#48619,#48620,#48621,#48622,#48623,
#48624,#48625,#48626,#48627,#48628,#48629,#48630,#48631,#48632,#48633,#48634,
#48635,#48636,#48637,#48638,#48639,#48640,#48641,#48642,#48643,#48644,#48645,
#48646,#48647,#48648,#48649,#48650,#48651,#48652,#48653,#48654,#48655,#48656,
#48657,#48658,#48659,#48660,#48661,#48662,#48663,#48664,#48665,#48666,#48667,
#48668,#48669,#48670,#48671,#48672,#48673,#48674,#48675,#48676,#48677,#48678,
#48679,#48680,#48681,#48682,#48683,#48684,#48685,#48686,#48687,#48688,#48689,
#48690,#48691,#48692,#48693,#48694,#48695,#48696,#48697,#48698,#48699,#48700,
#48701,#48702,#48703,#48704,#48705,#48706,#48707,#48708,#48709,#48710,#48711,
#48712,#48713,#48714,#48715,#48716,#48717,#48718,#48719,#48720,#48721,#48722,
#48723,#48724,#48725,#48726,#48727,#48728,#48729,#48730,#48731,#48732,#48733,
#48734,#48735,#48736,#48737,#48738,#48739,#48740,#48741,#48742,#48743,#48744,
#48745,#48746,#48747,#48748,#48749,#48750,#48751,#48752,#48753,#48754,#48755,
#48756,#48757,#48758,#48759,#48760,#48761,#48762,#48763,#48764,#48765,#48766,
#48767,#48768,#48769,#48770,#48771,#48772,#48773,#48774,#48775,#48776,#48777,
#48778,#48779,#48780,#48781,#48782,#48783,#48784,#48785,#48786,#48787,#48788,
#48789,#48790,#48791,#48792,#48793,#48794,#48795,#48796,#48797,#48798,#48799,
#48800,#48801,#48802,#48803,#48804,#48805,#48806,#48807,#48808,#48809,#48810,
#48811,#48812,#48813,#48814,#48815,#48816,#48817,#48818,#48819,#48820,#48821,
#48822,#48823,#48824,#48825,#48826,#48827,#48828,#48829,#48830,#48831,#48832,
#48833,#48834,#48835,#48836,#48837,#48838,#48839,#48840,#48841,#48842,#48843,
#48844,#48845,#48846,#48847,#48848,#48849,#48850,#48851,#48852,#48853,#48854,
#48855,#48856,#48857,#48858,#48859,#48860,#48861,#48862,#48863,#48864,#48865,
#48866,#48867,#48868,#48869,#48870,#48871,#48872,#48873,#48874,#48875,#48876,
#48877,#48878,#48879,#48880,#48881,#48882,#48883,#48884,#48885,#48886,#48887,
#48888,#48889,#48890,#48891,#48892,#48893,#48894,#48895,#48896,#48897,#48898,
#48899,#48900,#48901,#48902,#48903,#48904,#48905,#48906,#48907,#48908,#48909,
#48910,#48911,#48912,#48913,#48914,#48915,#48916,#48917,#48918,#48919,#48920,
#48921,#48922,#48923,#48924,#48925,#48926,#48927,#48928,#48929,#48930,#48931,
#48932,#48933,#48934,#48935,#48936,#48937,#48938,#48939,#48940,#48941,#48942,
#48943,#48944,#48945,#48946,#48947,#48948,#48949,#48950,#48951,#48952,#48953,
#48954,#48955,#48956,#48957,#48958,#48959,#48960,#48961,#48962,#48963,#48964,
#48965,#48966,#48967,#48968,#48969,#48970,#48971,#48972,#48973,#48974,#48975,
#48976,#48977,#48978,#48979,#48980,#48981,#48982,#48983,#48984,#48985,#48986,
#48987,#48988,#48989,#48990,#48991,#48992,#48993,#48994,#48995,#48996,#48997,
#48998,#48999,#49000,#49001,#49002,#49003,#49004,#49005,#49006,#49007,#49008,
#49009,#49010,#49011,#49012,#49013,#49014,#49015,#49016,#49017,#49018,#49019,
#49020,#49021,#49022,#49023,#49024,#49025,#49026,#49027,#49028,#49029,#49030,
#49031,#49032,#49033),(#49034,#49035,#49036,#49037,#49038,#49039,#49040,
#49041,#49042,#49043,#49044,#49045,#49046,#49047,#49048,#49049,#49050,#49051,
#49052,#49053,#49054,#49055,#49056,#49057,#49058,#49059,#49060,#49061,#49062,
#49063,#49064,#49065,#49066,#49067,#49068,#49069,#49070,#49071,#49072,#49073,
#49074,#49075,#49076,#49077,#49078,#49079,#49080,#49081,#49082,#49083,#49084,
#49085,#49086,#49087,#49088,#49089,#49090,#49091,#49092,#49093,#49094,#49095,
#49096,#49097,#49098,#49099,#49100,#49101,#49102,#49103,#49104,#49105,#49106,
#49107,#49108,#49109,#49110,#49111,#49112,#49113,#49114,#49115,#49116,#49117,
#49118,#49119,#49120,#49121,#49122,#49123,#49124,#49125,#49126,#49127,#49128,
#49129,#49130,#49131,#49132,#49133,#49134,#49135,#49136,#49137,#49138,#49139,
#49140,#49141,#49142,#49143,#49144,#49145,#49146,#49147,#49148,#49149,#49150,
#49151,#49152,#49153,#49154,#49155,#49156,#49157,#49158,#49159,#49160,#49161,
#49162,#49163,#49164,#49165,#49166,#49167,#49168,#49169,#49170,#49171,#49172,
#49173,#49174,#49175,#49176,#49177,#49178,#49179,#49180,#49181,#49182,#49183,
#49184,#49185,#49186,#49187,#49188,#49189,#49190,#49191,#49192,#49193,#49194,
#49195,#49196,#49197,#49198,#49199,#49200,#49201,#49202,#49203,#49204,#49205,
#49206,#49207,#49208,#49209,#49210,#49211,#49212,#49213,#49214,#49215,#49216,
#49217,#49218,#49219,#49220,#49221,#49222,#49223,#49224,#49225,#49226,#49227,
#49228,#49229,#49230,#49231,#49232,#49233,#49234,#49235,#49236,#49237,#49238,
#49239,#49240,#49241,#49242,#49243,#49244,#49245,#49246,#49247,#49248,#49249,
#49250,#49251,#49252,#49253,#49254,#49255,#49256,#49257,#49258,#49259,#49260,
#49261,#49262,#49263,#49264,#49265,#49266,#49267,#49268,#49269,#49270,#49271,
#49272,#49273,#49274,#49275,#49276,#49277,#49278,#49279,#49280,#49281,#49282,
#49283,#49284,#49285,#49286,#49287,#49288,#49289,#49290,#49291,#49292,#49293,
#49294,#49295,#49296,#49297,#49298,#49299,#49300,#49301,#49302,#49303,#49304,
#49305,#49306,#49307,#49308,#49309,#49310,#49311,#49312,#49313,#49314,#49315,
#49316,#49317,#49318,#49319,#49320,#49321,#49322,#49323,#49324,#49325,#49326,
#49327,#49328,#49329,#49330,#49331,#49332,#49333,#49334,#49335,#49336,#49337,
#49338,#49339,#49340,#49341,#49342,#49343,#49344,#49345,#49346,#49347,#49348,
#49349,#49350,#49351,#49352,#49353,#49354,#49355,#49356,#49357,#49358,#49359,
#49360,#49361,#49362,#49363,#49364,#49365,#49366,#49367,#49368,#49369,#49370,
#49371,#49372,#49373,#49374,#49375,#49376,#49377,#49378,#49379,#49380,#49381,
#49382,#49383,#49384,#49385,#49386,#49387,#49388,#49389,#49390,#49391,#49392,
#49393,#49394,#49395,#49396,#49397,#49398,#49399,#49400,#49401,#49402,#49403,
#49404,#49405,#49406,#49407,#49408,#49409,#49410,#49411,#49412,#49413,#49414,
#49415,#49416,#49417,#49418,#49419,#49420,#49421,#49422,#49423,#49424,#49425,
#49426,#49427,#49428,#49429,#49430,#49431,#49432,#49433,#49434,#49435,#49436,
#49437,#49438,#49439,#49440,#49441,#49442,#49443,#49444,#49445,#49446,#49447,
#49448,#49449,#49450,#49451,#49452,#49453,#49454,#49455,#49456,#49457,#49458,
#49459,#49460,#49461,#49462,#49463,#49464,#49465,#49466,#49467,#49468,#49469,
#49470,#49471,#49472,#49473,#49474,#49475,#49476,#49477,#49478,#49479,#49480,
#49481,#49482,#49483,#49484,#49485,#49486,#49487,#49488,#49489,#49490,#49491,
#49492,#49493,#49494,#49495,#49496,#49497,#49498,#49499,#49500,#49501,#49502,
#49503,#49504,#49505,#49506,#49507,#49508,#49509,#49510,#49511,#49512,#49513,
#49514,#49515,#49516,#49517,#49518,#49519,#49520,#49521,#49522,#49523,#49524,
#49525,#49526,#49527,#49528,#49529,#49530)),.UNSPECIFIED.,.F.,.F.,.F.,(4,
4),(4,1,1,1,1,1,1,1,1,1,1,1,1,1,1,1,1,1,1,1,1,1,1,1,1,1,1,1,1,1,1,1,1,1,
1,1,1,1,1,1,1,1,1,1,1,1,1,1,1,1,1,1,1,1,1,1,1,1,1,1,1,1,1,1,1,1,1,1,1,1,
1,1,1,1,1,1,1,1,1,1,1,1,1,1,1,1,1,1,1,1,1,1,1,1,1,1,1,1,1,1,1,1,1,1,1,1,
1,1,1,1,1,1,1,1,1,1,1,1,1,1,1,1,1,1,1,1,1,1,1,1,1,1,1,1,1,1,1,1,1,1,1,1,
1,1,1,1,1,1,1,1,1,1,1,1,1,1,1,1,1,1,1,1,1,1,1,1,1,1,1,1,1,1,1,1,1,1,1,1,
1,1,1,1,1,1,1,1,1,1,1,1,1,1,1,1,1,1,1,1,1,1,1,1,1,1,1,1,1,1,1,1,1,1,1,1,
1,1,1,1,1,1,1,1,1,1,1,1,1,1,1,1,1,1,1,1,1,1,1,1,1,1,1,1,1,1,1,1,1,1,1,1,
1,1,1,1,1,1,1,1,1,1,1,1,1,1,1,1,1,1,1,1,1,1,1,1,1,1,1,1,1,1,1,1,1,1,1,1,
1,1,1,1,1,1,1,1,1,1,1,1,1,1,1,1,1,1,1,1,1,1,1,1,1,1,1,1,1,1,1,1,1,1,1,1,
1,1,1,1,1,1,1,1,1,1,1,1,1,1,1,1,1,1,1,1,1,1,1,1,1,1,1,1,1,1,1,1,1,1,1,1,
1,1,1,1,1,1,1,1,1,1,1,1,1,1,1,1,1,1,1,1,1,1,1,1,1,1,1,1,1,1,1,1,1,1,1,1,
1,1,1,1,1,1,1,1,1,1,1,1,1,1,1,1,1,1,1,1,1,1,1,1,1,1,1,1,1,1,1,1,1,1,1,1,
1,1,1,1,1,1,1,1,1,1,1,1,1,1,1,1,1,1,1,1,1,1,1,1,1,1,1,1,1,1,1,1,1,1,1,1,
1,1,1,1,1,1,1,1,1,1,1,1,1,1,1,1,1,1,1,1,1,1,1,1,1,1,1,1,4),(0.,0.0641840294258107),
(14.3989442667815,14.8976525601681,15.3963608535547,15.8950691469414,16.393777440328,
16.8924857337146,17.3911940271012,17.8899023204878,18.3886106138744,18.8873189072611,
19.3860272006477,19.8847354940343,20.3834437874209,20.8821520808075,21.3808603741942,
21.8795686675808,22.3782769609674,22.876985254354,23.3756935477406,23.8744018411273,
24.3731101345139,24.8718184279005,25.3705267212871,25.8692350146737,26.3679433080604,
26.866651601447,27.3653598948336,27.8640681882202,28.3627764816068,28.8614847749935,
29.3601930683801,29.8589013617667,30.3576096551533,30.8563179485399,31.3550262419266,
31.8537345353132,32.3524428286998,32.8511511220864,33.349859415473,33.8485677088597,
34.3472760022463,34.8459842956329,35.3446925890195,35.8434008824061,36.3421091757927,
36.8408174691794,37.339525762566,37.8382340559526,38.3369423493392,38.8356506427259,
39.3343589361125,39.8330672294991,40.3317755228857,40.8304838162723,41.3291921096589,
41.8279004030456,42.3266086964322,42.8253169898188,43.3240252832054,43.822733576592,
44.3214418699787,44.8201501633653,45.3188584567519,45.8175667501385,46.3162750435251,
46.8149833369118,47.3136916302984,47.812399923685,48.3111082170716,48.8098165104582,
49.3085248038449,49.8072330972315,50.3059413906181,50.8046496840047,51.3033579773913,
51.802066270778,52.3007745641646,52.7994828575512,53.2981911509378,53.7968994443244,
54.2956077377111,54.7943160310977,55.2930243244843,55.7917326178709,56.2904409112575,
56.7891492046442,57.2878574980308,57.7865657914174,58.285274084804,58.7839823781906,
59.2826906715772,59.7813989649639,60.2801072583505,60.7788155517371,61.2775238451237,
61.7762321385104,62.274940431897,62.7736487252836,63.2723570186702,63.7710653120568,
64.2697736054434,64.7684818988301,65.2671901922167,65.7658984856033,66.2646067789899,
66.7633150723765,67.2620233657632,67.7607316591498,68.2594399525364,68.758148245923,
69.2568565393096,69.7555648326963,70.2542731260829,70.7529814194695,71.2516897128561,
71.7503980062427,72.2491062996294,72.747814593016,73.2465228864026,73.7452311797892,
74.2439394731758,74.7426477665625,75.2413560599491,75.7400643533357,76.2387726467223,
76.7374809401089,77.2361892334956,77.7348975268822,78.2336058202688,78.7323141136554,
79.231022407042,79.7297307004287,80.2284389938153,80.7271472872019,81.2258555805885,
81.7245638739751,82.2232721673618,82.7219804607484,83.220688754135,83.7193970475216,
84.2181053409082,84.7168136342949,85.2155219276815,85.7142302210681,86.2129385144547,
86.7116468078413,87.2103551012279,87.7090633946146,88.2077716880012,88.7064799813878,
89.2051882747744,89.703896568161,90.2026048615477,90.7013131549343,91.2000214483209,
91.6987297417075,92.1974380350942,92.6961463284808,93.1948546218674,93.693562915254,
94.1922712086406,94.6909795020272,95.1896877954139,95.6883960888005,96.1871043821871,
96.6858126755737,97.1845209689603,97.683229262347,98.1819375557336,98.6806458491202,
99.1793541425068,99.6780624358935,100.17677072928,100.675479022667,101.174187316053,
101.67289560944,102.171603902827,102.670312196213,103.1690204896,103.667728782986,
104.166437076373,104.66514536976,105.163853663146,105.662561956533,106.161270249919,
106.659978543306,107.158686836693,107.657395130079,108.156103423466,108.654811716853,
109.153520010239,109.652228303626,110.150936597012,110.649644890399,111.148353183786,
111.647061477172,112.145769770559,112.644478063946,113.143186357332,113.641894650719,
114.140602944105,114.639311237492,115.138019530879,115.636727824265,116.135436117652,
116.634144411039,117.132852704425,117.631560997812,118.130269291198,118.628977584585,
119.127685877972,119.626394171358,120.125102464745,120.623810758131,121.122519051518,
121.621227344905,122.119935638291,122.618643931678,123.117352225065,123.616060518451,
124.114768811838,124.613477105224,125.112185398611,125.610893691998,126.109601985384,
126.608310278771,127.107018572158,127.605726865544,128.104435158931,128.603143452317,
129.101851745704,129.600560039091,130.099268332477,130.597976625864,131.09668491925,
131.595393212637,132.094101506024,132.59280979941,133.091518092797,133.590226386184,
134.08893467957,135.086351266343,136.083767853117,137.08118443989,138.078601026663,
139.076017613436,140.07343420021,141.070850786983,142.068267373756,143.065683960529,
144.063100547303,145.060517134076,146.057933720849,147.055350307622,148.052766894396,
148.551475187782,149.050183481169,149.548891774555,150.047600067942,150.546308361329,
151.045016654715,151.543724948102,152.042433241488,152.541141534875,153.039849828262,
153.538558121648,154.037266415035,154.535974708422,155.034683001808,155.533391295195,
156.032099588581,156.530807881968,157.029516175355,157.528224468741,158.026932762128,
158.525641055515,159.024349348901,159.523057642288,160.021765935674,160.520474229061,
161.019182522448,161.517890815834,162.016599109221,162.515307402608,163.014015695994,
163.512723989381,164.011432282767,164.510140576154,165.008848869541,165.507557162927,
166.006265456314,166.5049737497,167.003682043087,167.502390336474,168.00109862986,
168.499806923247,168.998515216634,169.49722351002,169.995931803407,170.494640096793,
170.99334839018,171.492056683567,171.990764976953,172.48947327034,172.988181563726,
173.486889857113,173.9855981505,174.484306443886,174.983014737273,175.48172303066,
175.980431324046,176.479139617433,176.977847910819,177.476556204206,177.975264497593,
178.473972790979,178.972681084366,179.471389377753,179.970097671139,180.468805964526,
180.967514257912,181.466222551299,181.964930844686,182.463639138072,182.962347431459,
183.461055724845,183.959764018232,184.458472311619,184.957180605005,185.455888898392,
185.954597191779,186.453305485165,186.952013778552,187.450722071938,187.949430365325,
188.448138658712,188.946846952098,189.445555245485,189.944263538872,190.442971832258,
190.941680125645,191.440388419031,191.939096712418,192.437805005805,192.936513299191,
193.435221592578,193.933929885965,194.432638179351,194.931346472738,195.430054766124,
195.928763059511,196.427471352898,196.926179646284,197.424887939671,197.923596233057,
198.422304526444,198.921012819831,199.419721113217,199.918429406604,200.417137699991,
200.915845993377,201.414554286764,201.91326258015,202.411970873537,202.910679166924,
203.40938746031,203.908095753697,204.406804047084,204.90551234047,205.404220633857,
205.902928927243,206.40163722063,206.900345514017,207.399053807403,207.89776210079,
208.396470394177,208.895178687563,209.39388698095,209.892595274336,210.391303567723,
210.89001186111,211.388720154496,211.887428447883,212.386136741269,212.884845034656,
213.383553328043,213.882261621429,214.380969914816,214.879678208203,215.378386501589,
215.877094794976,216.375803088362,216.874511381749,217.373219675136,217.871927968522,
218.370636261909,218.869344555295,219.368052848682,219.866761142069,220.365469435455,
220.864177728842,221.362886022229,221.861594315615,222.360302609002,222.859010902388,
223.357719195775,223.856427489162,224.355135782548,224.853844075935,225.352552369322,
225.851260662708,226.349968956095,226.848677249481,227.347385542868,227.846093836255,
228.344802129641,228.843510423028,229.342218716414,229.840927009801,230.339635303188,
230.838343596574,231.337051889961,231.835760183348,232.334468476734,232.833176770121,
233.331885063507,233.830593356894,234.329301650281,234.828009943667,235.326718237054,
235.825426530441,236.324134823827,236.822843117214,237.3215514106,237.820259703987,
238.318967997374,238.81767629076,239.316384584147,239.815092877534,240.31380117092,
240.812509464307,241.311217757693,241.80992605108,242.308634344467,242.807342637853,
243.30605093124,243.804759224626,244.303467518013,244.8021758114,245.300884104786,
245.799592398173,246.29830069156,246.797008984946,247.295717278333,247.794425571719,
248.293133865106,248.791842158493,249.290550451879,249.789258745266,250.287967038653,
250.786675332039,251.285383625426,251.784091918812,252.282800212199,252.781508505586,
253.280216798972,253.778925092359,254.277633385745,254.776341679132,255.275049972519,
255.773758265905,256.272466559292,256.771174852679,257.269883146065,257.768591439452,
258.267299732838,258.766008026225,259.264716319612,259.763424612998,260.262132906385,
260.760841199772,261.259549493158,261.758257786545,262.256966079931,262.755674373318,
263.254382666705,263.753090960091,264.251799253478,264.750507546865,265.249215840251,
265.747924133638,266.246632427024,266.745340720411,267.244049013798,267.742757307184),
 .UNSPECIFIED.);
#346=B_SPLINE_SURFACE_WITH_KNOTS('',3,3,((#49923,#49924,#49925,#49926,#49927,
#49928,#49929,#49930,#49931,#49932,#49933,#49934,#49935,#49936,#49937,#49938,
#49939,#49940,#49941,#49942,#49943,#49944,#49945,#49946,#49947,#49948,#49949,
#49950,#49951,#49952,#49953,#49954,#49955,#49956,#49957,#49958,#49959,#49960,
#49961,#49962,#49963,#49964,#49965,#49966,#49967,#49968,#49969,#49970,#49971,
#49972,#49973,#49974,#49975,#49976,#49977,#49978,#49979,#49980,#49981,#49982,
#49983,#49984,#49985,#49986,#49987,#49988,#49989,#49990,#49991,#49992,#49993,
#49994,#49995,#49996,#49997,#49998,#49999,#50000,#50001,#50002,#50003,#50004,
#50005,#50006,#50007,#50008,#50009,#50010,#50011,#50012,#50013,#50014,#50015,
#50016,#50017,#50018,#50019,#50020,#50021,#50022,#50023,#50024,#50025,#50026,
#50027,#50028,#50029,#50030,#50031,#50032,#50033,#50034,#50035,#50036,#50037,
#50038,#50039,#50040,#50041,#50042,#50043,#50044,#50045,#50046,#50047,#50048,
#50049,#50050,#50051,#50052,#50053,#50054,#50055,#50056,#50057,#50058,#50059,
#50060,#50061,#50062,#50063,#50064,#50065,#50066,#50067,#50068,#50069,#50070,
#50071,#50072,#50073,#50074,#50075,#50076,#50077,#50078,#50079,#50080,#50081,
#50082,#50083,#50084,#50085,#50086,#50087,#50088,#50089,#50090,#50091,#50092,
#50093,#50094,#50095,#50096,#50097,#50098,#50099,#50100,#50101,#50102,#50103,
#50104,#50105,#50106,#50107,#50108,#50109,#50110,#50111,#50112,#50113,#50114,
#50115,#50116,#50117,#50118,#50119,#50120,#50121,#50122,#50123,#50124,#50125,
#50126,#50127,#50128,#50129,#50130,#50131,#50132,#50133,#50134,#50135,#50136,
#50137,#50138,#50139,#50140,#50141,#50142,#50143,#50144,#50145,#50146,#50147,
#50148,#50149,#50150,#50151,#50152,#50153,#50154,#50155,#50156,#50157,#50158,
#50159,#50160,#50161,#50162,#50163,#50164,#50165,#50166,#50167,#50168,#50169,
#50170,#50171,#50172,#50173,#50174,#50175,#50176,#50177,#50178,#50179,#50180,
#50181,#50182,#50183,#50184,#50185,#50186,#50187,#50188,#50189,#50190,#50191,
#50192,#50193,#50194,#50195,#50196,#50197,#50198,#50199,#50200,#50201,#50202,
#50203,#50204,#50205,#50206,#50207,#50208,#50209,#50210,#50211,#50212,#50213,
#50214,#50215,#50216,#50217,#50218,#50219,#50220,#50221,#50222,#50223,#50224,
#50225,#50226,#50227,#50228,#50229,#50230,#50231,#50232,#50233,#50234,#50235,
#50236,#50237,#50238,#50239,#50240,#50241,#50242,#50243,#50244,#50245),
(#50246,#50247,#50248,#50249,#50250,#50251,#50252,#50253,#50254,#50255,
#50256,#50257,#50258,#50259,#50260,#50261,#50262,#50263,#50264,#50265,#50266,
#50267,#50268,#50269,#50270,#50271,#50272,#50273,#50274,#50275,#50276,#50277,
#50278,#50279,#50280,#50281,#50282,#50283,#50284,#50285,#50286,#50287,#50288,
#50289,#50290,#50291,#50292,#50293,#50294,#50295,#50296,#50297,#50298,#50299,
#50300,#50301,#50302,#50303,#50304,#50305,#50306,#50307,#50308,#50309,#50310,
#50311,#50312,#50313,#50314,#50315,#50316,#50317,#50318,#50319,#50320,#50321,
#50322,#50323,#50324,#50325,#50326,#50327,#50328,#50329,#50330,#50331,#50332,
#50333,#50334,#50335,#50336,#50337,#50338,#50339,#50340,#50341,#50342,#50343,
#50344,#50345,#50346,#50347,#50348,#50349,#50350,#50351,#50352,#50353,#50354,
#50355,#50356,#50357,#50358,#50359,#50360,#50361,#50362,#50363,#50364,#50365,
#50366,#50367,#50368,#50369,#50370,#50371,#50372,#50373,#50374,#50375,#50376,
#50377,#50378,#50379,#50380,#50381,#50382,#50383,#50384,#50385,#50386,#50387,
#50388,#50389,#50390,#50391,#50392,#50393,#50394,#50395,#50396,#50397,#50398,
#50399,#50400,#50401,#50402,#50403,#50404,#50405,#50406,#50407,#50408,#50409,
#50410,#50411,#50412,#50413,#50414,#50415,#50416,#50417,#50418,#50419,#50420,
#50421,#50422,#50423,#50424,#50425,#50426,#50427,#50428,#50429,#50430,#50431,
#50432,#50433,#50434,#50435,#50436,#50437,#50438,#50439,#50440,#50441,#50442,
#50443,#50444,#50445,#50446,#50447,#50448,#50449,#50450,#50451,#50452,#50453,
#50454,#50455,#50456,#50457,#50458,#50459,#50460,#50461,#50462,#50463,#50464,
#50465,#50466,#50467,#50468,#50469,#50470,#50471,#50472,#50473,#50474,#50475,
#50476,#50477,#50478,#50479,#50480,#50481,#50482,#50483,#50484,#50485,#50486,
#50487,#50488,#50489,#50490,#50491,#50492,#50493,#50494,#50495,#50496,#50497,
#50498,#50499,#50500,#50501,#50502,#50503,#50504,#50505,#50506,#50507,#50508,
#50509,#50510,#50511,#50512,#50513,#50514,#50515,#50516,#50517,#50518,#50519,
#50520,#50521,#50522,#50523,#50524,#50525,#50526,#50527,#50528,#50529,#50530,
#50531,#50532,#50533,#50534,#50535,#50536,#50537,#50538,#50539,#50540,#50541,
#50542,#50543,#50544,#50545,#50546,#50547,#50548,#50549,#50550,#50551,#50552,
#50553,#50554,#50555,#50556,#50557,#50558,#50559,#50560,#50561,#50562,#50563,
#50564,#50565,#50566,#50567,#50568),(#50569,#50570,#50571,#50572,#50573,
#50574,#50575,#50576,#50577,#50578,#50579,#50580,#50581,#50582,#50583,#50584,
#50585,#50586,#50587,#50588,#50589,#50590,#50591,#50592,#50593,#50594,#50595,
#50596,#50597,#50598,#50599,#50600,#50601,#50602,#50603,#50604,#50605,#50606,
#50607,#50608,#50609,#50610,#50611,#50612,#50613,#50614,#50615,#50616,#50617,
#50618,#50619,#50620,#50621,#50622,#50623,#50624,#50625,#50626,#50627,#50628,
#50629,#50630,#50631,#50632,#50633,#50634,#50635,#50636,#50637,#50638,#50639,
#50640,#50641,#50642,#50643,#50644,#50645,#50646,#50647,#50648,#50649,#50650,
#50651,#50652,#50653,#50654,#50655,#50656,#50657,#50658,#50659,#50660,#50661,
#50662,#50663,#50664,#50665,#50666,#50667,#50668,#50669,#50670,#50671,#50672,
#50673,#50674,#50675,#50676,#50677,#50678,#50679,#50680,#50681,#50682,#50683,
#50684,#50685,#50686,#50687,#50688,#50689,#50690,#50691,#50692,#50693,#50694,
#50695,#50696,#50697,#50698,#50699,#50700,#50701,#50702,#50703,#50704,#50705,
#50706,#50707,#50708,#50709,#50710,#50711,#50712,#50713,#50714,#50715,#50716,
#50717,#50718,#50719,#50720,#50721,#50722,#50723,#50724,#50725,#50726,#50727,
#50728,#50729,#50730,#50731,#50732,#50733,#50734,#50735,#50736,#50737,#50738,
#50739,#50740,#50741,#50742,#50743,#50744,#50745,#50746,#50747,#50748,#50749,
#50750,#50751,#50752,#50753,#50754,#50755,#50756,#50757,#50758,#50759,#50760,
#50761,#50762,#50763,#50764,#50765,#50766,#50767,#50768,#50769,#50770,#50771,
#50772,#50773,#50774,#50775,#50776,#50777,#50778,#50779,#50780,#50781,#50782,
#50783,#50784,#50785,#50786,#50787,#50788,#50789,#50790,#50791,#50792,#50793,
#50794,#50795,#50796,#50797,#50798,#50799,#50800,#50801,#50802,#50803,#50804,
#50805,#50806,#50807,#50808,#50809,#50810,#50811,#50812,#50813,#50814,#50815,
#50816,#50817,#50818,#50819,#50820,#50821,#50822,#50823,#50824,#50825,#50826,
#50827,#50828,#50829,#50830,#50831,#50832,#50833,#50834,#50835,#50836,#50837,
#50838,#50839,#50840,#50841,#50842,#50843,#50844,#50845,#50846,#50847,#50848,
#50849,#50850,#50851,#50852,#50853,#50854,#50855,#50856,#50857,#50858,#50859,
#50860,#50861,#50862,#50863,#50864,#50865,#50866,#50867,#50868,#50869,#50870,
#50871,#50872,#50873,#50874,#50875,#50876,#50877,#50878,#50879,#50880,#50881,
#50882,#50883,#50884,#50885,#50886,#50887,#50888,#50889,#50890,#50891),
(#50892,#50893,#50894,#50895,#50896,#50897,#50898,#50899,#50900,#50901,
#50902,#50903,#50904,#50905,#50906,#50907,#50908,#50909,#50910,#50911,#50912,
#50913,#50914,#50915,#50916,#50917,#50918,#50919,#50920,#50921,#50922,#50923,
#50924,#50925,#50926,#50927,#50928,#50929,#50930,#50931,#50932,#50933,#50934,
#50935,#50936,#50937,#50938,#50939,#50940,#50941,#50942,#50943,#50944,#50945,
#50946,#50947,#50948,#50949,#50950,#50951,#50952,#50953,#50954,#50955,#50956,
#50957,#50958,#50959,#50960,#50961,#50962,#50963,#50964,#50965,#50966,#50967,
#50968,#50969,#50970,#50971,#50972,#50973,#50974,#50975,#50976,#50977,#50978,
#50979,#50980,#50981,#50982,#50983,#50984,#50985,#50986,#50987,#50988,#50989,
#50990,#50991,#50992,#50993,#50994,#50995,#50996,#50997,#50998,#50999,#51000,
#51001,#51002,#51003,#51004,#51005,#51006,#51007,#51008,#51009,#51010,#51011,
#51012,#51013,#51014,#51015,#51016,#51017,#51018,#51019,#51020,#51021,#51022,
#51023,#51024,#51025,#51026,#51027,#51028,#51029,#51030,#51031,#51032,#51033,
#51034,#51035,#51036,#51037,#51038,#51039,#51040,#51041,#51042,#51043,#51044,
#51045,#51046,#51047,#51048,#51049,#51050,#51051,#51052,#51053,#51054,#51055,
#51056,#51057,#51058,#51059,#51060,#51061,#51062,#51063,#51064,#51065,#51066,
#51067,#51068,#51069,#51070,#51071,#51072,#51073,#51074,#51075,#51076,#51077,
#51078,#51079,#51080,#51081,#51082,#51083,#51084,#51085,#51086,#51087,#51088,
#51089,#51090,#51091,#51092,#51093,#51094,#51095,#51096,#51097,#51098,#51099,
#51100,#51101,#51102,#51103,#51104,#51105,#51106,#51107,#51108,#51109,#51110,
#51111,#51112,#51113,#51114,#51115,#51116,#51117,#51118,#51119,#51120,#51121,
#51122,#51123,#51124,#51125,#51126,#51127,#51128,#51129,#51130,#51131,#51132,
#51133,#51134,#51135,#51136,#51137,#51138,#51139,#51140,#51141,#51142,#51143,
#51144,#51145,#51146,#51147,#51148,#51149,#51150,#51151,#51152,#51153,#51154,
#51155,#51156,#51157,#51158,#51159,#51160,#51161,#51162,#51163,#51164,#51165,
#51166,#51167,#51168,#51169,#51170,#51171,#51172,#51173,#51174,#51175,#51176,
#51177,#51178,#51179,#51180,#51181,#51182,#51183,#51184,#51185,#51186,#51187,
#51188,#51189,#51190,#51191,#51192,#51193,#51194,#51195,#51196,#51197,#51198,
#51199,#51200,#51201,#51202,#51203,#51204,#51205,#51206,#51207,#51208,#51209,
#51210,#51211,#51212,#51213,#51214)),.UNSPECIFIED.,.F.,.F.,.F.,(4,4),(4,
1,1,1,1,1,1,1,1,1,1,1,1,1,1,1,1,1,1,1,1,1,1,1,1,1,1,1,1,1,1,1,1,1,1,1,1,
1,1,1,1,1,1,1,1,1,1,1,1,1,1,1,1,1,1,1,1,1,1,1,1,1,1,1,1,1,1,1,1,1,1,1,1,
1,1,1,1,1,1,1,1,1,1,1,1,1,1,1,1,1,1,1,1,1,1,1,1,1,1,1,1,1,1,1,1,1,1,1,1,
1,1,1,1,1,1,1,1,1,1,1,1,1,1,1,1,1,1,1,1,1,1,1,1,1,1,1,1,1,1,1,1,1,1,1,1,
1,1,1,1,1,1,1,1,1,1,1,1,1,1,1,1,1,1,1,1,1,1,1,1,1,1,1,1,1,1,1,1,1,1,1,1,
1,1,1,1,1,1,1,1,1,1,1,1,1,1,1,1,1,1,1,1,1,1,1,1,1,1,1,1,1,1,1,1,1,1,1,1,
1,1,1,1,1,1,1,1,1,1,1,1,1,1,1,1,1,1,1,1,1,1,1,1,1,1,1,1,1,1,1,1,1,1,1,1,
1,1,1,1,1,1,1,1,1,1,1,1,1,1,1,1,1,1,1,1,1,1,1,1,1,1,1,1,1,1,1,1,1,1,1,1,
1,1,1,1,1,1,1,1,1,1,1,1,1,1,1,1,1,1,1,1,1,1,1,1,1,1,1,1,1,1,1,4),(0.,0.0641840294258124),
(11.8589888623079,12.3561639667852,12.8533390712624,13.3505141757396,13.8476892802168,
14.344864384694,14.8420394891712,15.3392145936484,15.8363896981257,16.3335648026029,
16.8307399070801,17.3279150115573,17.8250901160345,18.3222652205117,18.8194403249889,
19.3166154294662,19.8137905339434,20.3109656384206,20.8081407428978,21.305315847375,
21.8024909518522,22.2996660563294,22.7968411608067,23.2940162652839,23.7911913697611,
24.2883664742383,24.7855415787155,25.2827166831927,25.7798917876699,26.2770668921472,
26.7742419966244,27.2714171011016,27.7685922055788,28.265767310056,28.7629424145332,
29.2601175190104,29.7572926234877,30.2544677279649,30.7516428324421,31.2488179369193,
31.7459930413965,32.2431681458737,32.7403432503509,33.2375183548282,33.7346934593054,
34.2318685637826,34.7290436682598,35.226218772737,35.7233938772142,36.2205689816915,
36.7177440861687,37.2149191906459,37.7120942951231,38.2092693996003,38.7064445040775,
39.2036196085547,39.700794713032,40.1979698175092,40.6951449219864,41.1923200264636,
41.6894951309408,42.186670235418,42.6838453398952,43.1810204443725,43.6781955488497,
44.1753706533269,44.6725457578041,45.1697208622813,45.6668959667585,46.1640710712357,
46.661246175713,47.1584212801902,47.6555963846674,48.1527714891446,48.6499465936218,
49.147121698099,49.6442968025762,50.1414719070535,50.6386470115307,51.1358221160079,
51.6329972204851,52.1301723249623,52.6273474294395,53.1245225339167,53.621697638394,
54.1188727428712,54.6160478473484,55.1132229518256,55.6103980563028,56.10757316078,
56.6047482652572,57.1019233697345,57.5990984742117,58.0962735786889,58.5934486831661,
59.0906237876433,59.5877988921205,60.0849739965977,60.582149101075,61.0793242055522,
61.5764993100294,62.0736744145066,62.5708495189838,63.068024623461,63.5651997279382,
64.0623748324155,64.5595499368927,65.0567250413699,65.5539001458471,66.0510752503243,
66.5482503548015,67.0454254592788,67.542600563756,68.0397756682332,68.5369507727104,
69.0341258771876,69.5313009816648,70.028476086142,70.5256511906192,71.0228262950965,
71.5200013995737,72.0171765040509,72.5143516085281,73.0115267130053,73.5087018174825,
74.0058769219598,74.503052026437,75.0002271309142,75.4974022353914,75.9945773398686,
76.4917524443458,76.988927548823,77.4861026533003,77.9832777577775,78.4804528622547,
78.9776279667319,79.4748030712091,79.9719781756863,80.4691532801635,80.9663283846407,
81.463503489118,81.9606785935952,82.4578536980724,82.9550288025496,83.4522039070268,
83.949379011504,84.4465541159813,84.9437292204585,85.4409043249357,85.9380794294129,
86.4352545338901,86.9324296383673,87.4296047428445,87.9267798473217,88.423954951799,
88.9211300562762,89.4183051607534,89.9154802652306,90.4126553697078,90.909830474185,
91.4070055786623,91.9041806831395,92.4013557876167,92.8985308920939,93.3957059965711,
93.8928811010483,94.3900562055255,94.8872313100028,95.38440641448,95.8815815189572,
96.3787566234344,96.8759317279116,97.3731068323888,97.870281936866,98.3674570413433,
98.8646321458205,99.3618072502977,99.8589823547749,100.356157459252,100.853332563729,
101.350507668207,101.847682772684,102.344857877161,102.842032981638,103.339208086115,
103.836383190593,104.33355829507,104.830733399547,105.327908504024,105.825083608501,
106.322258712979,106.819433817456,107.316608921933,107.81378402641,108.310959130888,
108.808134235365,109.305309339842,109.802484444319,110.299659548796,110.796834653274,
111.294009757751,111.791184862228,112.288359966705,112.785535071182,113.28271017566,
113.779885280137,114.277060384614,114.774235489091,115.271410593569,115.768585698046,
116.265760802523,116.762935907,117.260111011477,117.757286115955,118.254461220432,
118.751636324909,119.248811429386,119.745986533863,120.243161638341,120.740336742818,
121.237511847295,121.734686951772,122.23186205625,122.729037160727,123.226212265204,
123.723387369681,124.220562474158,124.717737578636,125.214912683113,125.71208778759,
126.209262892067,126.706437996544,127.203613101022,127.700788205499,128.197963309976,
128.695138414453,129.192313518931,129.689488623408,130.186663727885,130.683838832362,
131.181013936839,131.678189041317,132.175364145794,132.672539250271,133.169714354748,
133.666889459226,134.164064563703,134.66123966818,135.158414772657,135.655589877134,
136.152764981612,136.649940086089,137.147115190566,137.644290295043,138.14146539952,
138.638640503998,139.135815608475,139.632990712952,140.130165817429,140.627340921906,
141.124516026384,141.621691130861,142.118866235338,142.616041339815,143.113216444293,
143.61039154877,144.107566653247,144.604741757724,145.101916862201,145.599091966679,
146.096267071156,146.593442175633,147.09061728011,147.587792384587,148.084967489065,
148.582142593542,149.079317698019,149.576492802496,150.073667906974,150.570843011451,
151.068018115928,151.565193220405,152.062368324882,152.55954342936,153.056718533837,
153.553893638314,154.051068742791,154.548243847269,155.045418951746,155.542594056223,
156.0397691607,156.536944265177,157.034119369655,157.531294474132,158.028469578609,
158.525644683086,159.022819787563,159.519994892041,160.017169996518,160.514345100995,
161.011520205472,161.508695309949,162.005870414427,162.503045518904,163.000220623381,
163.497395727858,163.994570832336,164.491745936813,164.98892104129,165.486096145767,
165.983271250244,166.480446354722,166.977621459199,167.474796563676,167.971971668153,
168.46914677263,168.966321877108,169.463496981585,169.960672086062,170.457847190539,
170.955022295017),.UNSPECIFIED.);
#347=B_SPLINE_SURFACE_WITH_KNOTS('',3,3,((#51364,#51365,#51366,#51367,#51368,
#51369,#51370,#51371,#51372,#51373,#51374,#51375,#51376,#51377,#51378,#51379,
#51380,#51381,#51382,#51383,#51384,#51385,#51386,#51387,#51388,#51389,#51390,
#51391,#51392,#51393,#51394,#51395,#51396,#51397,#51398,#51399,#51400,#51401,
#51402,#51403,#51404,#51405,#51406,#51407,#51408,#51409,#51410,#51411,#51412,
#51413,#51414,#51415,#51416,#51417,#51418,#51419,#51420,#51421,#51422,#51423,
#51424,#51425,#51426,#51427,#51428,#51429,#51430,#51431,#51432,#51433,#51434,
#51435,#51436,#51437,#51438,#51439,#51440,#51441,#51442,#51443,#51444,#51445,
#51446,#51447,#51448,#51449,#51450,#51451,#51452,#51453,#51454,#51455,#51456,
#51457,#51458,#51459,#51460,#51461,#51462,#51463,#51464,#51465,#51466,#51467,
#51468,#51469,#51470,#51471,#51472,#51473,#51474,#51475,#51476,#51477,#51478,
#51479,#51480,#51481,#51482,#51483,#51484,#51485,#51486,#51487,#51488,#51489,
#51490,#51491,#51492,#51493,#51494,#51495,#51496,#51497,#51498,#51499,#51500,
#51501,#51502,#51503,#51504,#51505,#51506,#51507,#51508,#51509,#51510,#51511,
#51512,#51513,#51514,#51515,#51516,#51517,#51518,#51519,#51520,#51521,#51522,
#51523,#51524,#51525,#51526,#51527,#51528,#51529,#51530,#51531,#51532,#51533,
#51534,#51535,#51536,#51537,#51538,#51539,#51540,#51541,#51542,#51543,#51544,
#51545,#51546,#51547,#51548,#51549,#51550,#51551,#51552,#51553,#51554,#51555,
#51556,#51557,#51558,#51559,#51560,#51561,#51562,#51563,#51564,#51565,#51566,
#51567,#51568,#51569,#51570,#51571,#51572,#51573,#51574,#51575,#51576,#51577,
#51578,#51579,#51580,#51581,#51582,#51583,#51584,#51585,#51586,#51587,#51588,
#51589,#51590,#51591,#51592,#51593,#51594,#51595,#51596,#51597,#51598,#51599,
#51600,#51601,#51602,#51603,#51604,#51605,#51606,#51607,#51608,#51609,#51610,
#51611,#51612,#51613,#51614,#51615,#51616,#51617,#51618,#51619,#51620,#51621,
#51622,#51623,#51624,#51625,#51626,#51627,#51628,#51629,#51630,#51631,#51632,
#51633,#51634,#51635,#51636,#51637,#51638,#51639,#51640,#51641,#51642,#51643,
#51644,#51645,#51646,#51647,#51648,#51649,#51650,#51651,#51652,#51653,#51654,
#51655,#51656,#51657,#51658,#51659,#51660,#51661,#51662,#51663,#51664,#51665,
#51666,#51667,#51668,#51669,#51670,#51671,#51672,#51673,#51674,#51675,#51676,
#51677,#51678,#51679,#51680,#51681,#51682,#51683,#51684,#51685,#51686),
(#51687,#51688,#51689,#51690,#51691,#51692,#51693,#51694,#51695,#51696,
#51697,#51698,#51699,#51700,#51701,#51702,#51703,#51704,#51705,#51706,#51707,
#51708,#51709,#51710,#51711,#51712,#51713,#51714,#51715,#51716,#51717,#51718,
#51719,#51720,#51721,#51722,#51723,#51724,#51725,#51726,#51727,#51728,#51729,
#51730,#51731,#51732,#51733,#51734,#51735,#51736,#51737,#51738,#51739,#51740,
#51741,#51742,#51743,#51744,#51745,#51746,#51747,#51748,#51749,#51750,#51751,
#51752,#51753,#51754,#51755,#51756,#51757,#51758,#51759,#51760,#51761,#51762,
#51763,#51764,#51765,#51766,#51767,#51768,#51769,#51770,#51771,#51772,#51773,
#51774,#51775,#51776,#51777,#51778,#51779,#51780,#51781,#51782,#51783,#51784,
#51785,#51786,#51787,#51788,#51789,#51790,#51791,#51792,#51793,#51794,#51795,
#51796,#51797,#51798,#51799,#51800,#51801,#51802,#51803,#51804,#51805,#51806,
#51807,#51808,#51809,#51810,#51811,#51812,#51813,#51814,#51815,#51816,#51817,
#51818,#51819,#51820,#51821,#51822,#51823,#51824,#51825,#51826,#51827,#51828,
#51829,#51830,#51831,#51832,#51833,#51834,#51835,#51836,#51837,#51838,#51839,
#51840,#51841,#51842,#51843,#51844,#51845,#51846,#51847,#51848,#51849,#51850,
#51851,#51852,#51853,#51854,#51855,#51856,#51857,#51858,#51859,#51860,#51861,
#51862,#51863,#51864,#51865,#51866,#51867,#51868,#51869,#51870,#51871,#51872,
#51873,#51874,#51875,#51876,#51877,#51878,#51879,#51880,#51881,#51882,#51883,
#51884,#51885,#51886,#51887,#51888,#51889,#51890,#51891,#51892,#51893,#51894,
#51895,#51896,#51897,#51898,#51899,#51900,#51901,#51902,#51903,#51904,#51905,
#51906,#51907,#51908,#51909,#51910,#51911,#51912,#51913,#51914,#51915,#51916,
#51917,#51918,#51919,#51920,#51921,#51922,#51923,#51924,#51925,#51926,#51927,
#51928,#51929,#51930,#51931,#51932,#51933,#51934,#51935,#51936,#51937,#51938,
#51939,#51940,#51941,#51942,#51943,#51944,#51945,#51946,#51947,#51948,#51949,
#51950,#51951,#51952,#51953,#51954,#51955,#51956,#51957,#51958,#51959,#51960,
#51961,#51962,#51963,#51964,#51965,#51966,#51967,#51968,#51969,#51970,#51971,
#51972,#51973,#51974,#51975,#51976,#51977,#51978,#51979,#51980,#51981,#51982,
#51983,#51984,#51985,#51986,#51987,#51988,#51989,#51990,#51991,#51992,#51993,
#51994,#51995,#51996,#51997,#51998,#51999,#52000,#52001,#52002,#52003,#52004,
#52005,#52006,#52007,#52008,#52009),(#52010,#52011,#52012,#52013,#52014,
#52015,#52016,#52017,#52018,#52019,#52020,#52021,#52022,#52023,#52024,#52025,
#52026,#52027,#52028,#52029,#52030,#52031,#52032,#52033,#52034,#52035,#52036,
#52037,#52038,#52039,#52040,#52041,#52042,#52043,#52044,#52045,#52046,#52047,
#52048,#52049,#52050,#52051,#52052,#52053,#52054,#52055,#52056,#52057,#52058,
#52059,#52060,#52061,#52062,#52063,#52064,#52065,#52066,#52067,#52068,#52069,
#52070,#52071,#52072,#52073,#52074,#52075,#52076,#52077,#52078,#52079,#52080,
#52081,#52082,#52083,#52084,#52085,#52086,#52087,#52088,#52089,#52090,#52091,
#52092,#52093,#52094,#52095,#52096,#52097,#52098,#52099,#52100,#52101,#52102,
#52103,#52104,#52105,#52106,#52107,#52108,#52109,#52110,#52111,#52112,#52113,
#52114,#52115,#52116,#52117,#52118,#52119,#52120,#52121,#52122,#52123,#52124,
#52125,#52126,#52127,#52128,#52129,#52130,#52131,#52132,#52133,#52134,#52135,
#52136,#52137,#52138,#52139,#52140,#52141,#52142,#52143,#52144,#52145,#52146,
#52147,#52148,#52149,#52150,#52151,#52152,#52153,#52154,#52155,#52156,#52157,
#52158,#52159,#52160,#52161,#52162,#52163,#52164,#52165,#52166,#52167,#52168,
#52169,#52170,#52171,#52172,#52173,#52174,#52175,#52176,#52177,#52178,#52179,
#52180,#52181,#52182,#52183,#52184,#52185,#52186,#52187,#52188,#52189,#52190,
#52191,#52192,#52193,#52194,#52195,#52196,#52197,#52198,#52199,#52200,#52201,
#52202,#52203,#52204,#52205,#52206,#52207,#52208,#52209,#52210,#52211,#52212,
#52213,#52214,#52215,#52216,#52217,#52218,#52219,#52220,#52221,#52222,#52223,
#52224,#52225,#52226,#52227,#52228,#52229,#52230,#52231,#52232,#52233,#52234,
#52235,#52236,#52237,#52238,#52239,#52240,#52241,#52242,#52243,#52244,#52245,
#52246,#52247,#52248,#52249,#52250,#52251,#52252,#52253,#52254,#52255,#52256,
#52257,#52258,#52259,#52260,#52261,#52262,#52263,#52264,#52265,#52266,#52267,
#52268,#52269,#52270,#52271,#52272,#52273,#52274,#52275,#52276,#52277,#52278,
#52279,#52280,#52281,#52282,#52283,#52284,#52285,#52286,#52287,#52288,#52289,
#52290,#52291,#52292,#52293,#52294,#52295,#52296,#52297,#52298,#52299,#52300,
#52301,#52302,#52303,#52304,#52305,#52306,#52307,#52308,#52309,#52310,#52311,
#52312,#52313,#52314,#52315,#52316,#52317,#52318,#52319,#52320,#52321,#52322,
#52323,#52324,#52325,#52326,#52327,#52328,#52329,#52330,#52331,#52332),
(#52333,#52334,#52335,#52336,#52337,#52338,#52339,#52340,#52341,#52342,
#52343,#52344,#52345,#52346,#52347,#52348,#52349,#52350,#52351,#52352,#52353,
#52354,#52355,#52356,#52357,#52358,#52359,#52360,#52361,#52362,#52363,#52364,
#52365,#52366,#52367,#52368,#52369,#52370,#52371,#52372,#52373,#52374,#52375,
#52376,#52377,#52378,#52379,#52380,#52381,#52382,#52383,#52384,#52385,#52386,
#52387,#52388,#52389,#52390,#52391,#52392,#52393,#52394,#52395,#52396,#52397,
#52398,#52399,#52400,#52401,#52402,#52403,#52404,#52405,#52406,#52407,#52408,
#52409,#52410,#52411,#52412,#52413,#52414,#52415,#52416,#52417,#52418,#52419,
#52420,#52421,#52422,#52423,#52424,#52425,#52426,#52427,#52428,#52429,#52430,
#52431,#52432,#52433,#52434,#52435,#52436,#52437,#52438,#52439,#52440,#52441,
#52442,#52443,#52444,#52445,#52446,#52447,#52448,#52449,#52450,#52451,#52452,
#52453,#52454,#52455,#52456,#52457,#52458,#52459,#52460,#52461,#52462,#52463,
#52464,#52465,#52466,#52467,#52468,#52469,#52470,#52471,#52472,#52473,#52474,
#52475,#52476,#52477,#52478,#52479,#52480,#52481,#52482,#52483,#52484,#52485,
#52486,#52487,#52488,#52489,#52490,#52491,#52492,#52493,#52494,#52495,#52496,
#52497,#52498,#52499,#52500,#52501,#52502,#52503,#52504,#52505,#52506,#52507,
#52508,#52509,#52510,#52511,#52512,#52513,#52514,#52515,#52516,#52517,#52518,
#52519,#52520,#52521,#52522,#52523,#52524,#52525,#52526,#52527,#52528,#52529,
#52530,#52531,#52532,#52533,#52534,#52535,#52536,#52537,#52538,#52539,#52540,
#52541,#52542,#52543,#52544,#52545,#52546,#52547,#52548,#52549,#52550,#52551,
#52552,#52553,#52554,#52555,#52556,#52557,#52558,#52559,#52560,#52561,#52562,
#52563,#52564,#52565,#52566,#52567,#52568,#52569,#52570,#52571,#52572,#52573,
#52574,#52575,#52576,#52577,#52578,#52579,#52580,#52581,#52582,#52583,#52584,
#52585,#52586,#52587,#52588,#52589,#52590,#52591,#52592,#52593,#52594,#52595,
#52596,#52597,#52598,#52599,#52600,#52601,#52602,#52603,#52604,#52605,#52606,
#52607,#52608,#52609,#52610,#52611,#52612,#52613,#52614,#52615,#52616,#52617,
#52618,#52619,#52620,#52621,#52622,#52623,#52624,#52625,#52626,#52627,#52628,
#52629,#52630,#52631,#52632,#52633,#52634,#52635,#52636,#52637,#52638,#52639,
#52640,#52641,#52642,#52643,#52644,#52645,#52646,#52647,#52648,#52649,#52650,
#52651,#52652,#52653,#52654,#52655)),.UNSPECIFIED.,.F.,.F.,.F.,(4,4),(4,
1,1,1,1,1,1,1,1,1,1,1,1,1,1,1,1,1,1,1,1,1,1,1,1,1,1,1,1,1,1,1,1,1,1,1,1,
1,1,1,1,1,1,1,1,1,1,1,1,1,1,1,1,1,1,1,1,1,1,1,1,1,1,1,1,1,1,1,1,1,1,1,1,
1,1,1,1,1,1,1,1,1,1,1,1,1,1,1,1,1,1,1,1,1,1,1,1,1,1,1,1,1,1,1,1,1,1,1,1,
1,1,1,1,1,1,1,1,1,1,1,1,1,1,1,1,1,1,1,1,1,1,1,1,1,1,1,1,1,1,1,1,1,1,1,1,
1,1,1,1,1,1,1,1,1,1,1,1,1,1,1,1,1,1,1,1,1,1,1,1,1,1,1,1,1,1,1,1,1,1,1,1,
1,1,1,1,1,1,1,1,1,1,1,1,1,1,1,1,1,1,1,1,1,1,1,1,1,1,1,1,1,1,1,1,1,1,1,1,
1,1,1,1,1,1,1,1,1,1,1,1,1,1,1,1,1,1,1,1,1,1,1,1,1,1,1,1,1,1,1,1,1,1,1,1,
1,1,1,1,1,1,1,1,1,1,1,1,1,1,1,1,1,1,1,1,1,1,1,1,1,1,1,1,1,1,1,1,1,1,1,1,
1,1,1,1,1,1,1,1,1,1,1,1,1,1,1,1,1,1,1,1,1,1,1,1,1,1,1,1,1,1,1,4),(0.,0.0641840294258124),
(14.398944266781,14.8961193712582,15.3932944757354,15.8904695802126,16.3876446846898,
16.884819789167,17.3819948936443,17.8791699981215,18.3763451025987,18.8735202070759,
19.3706953115531,19.8678704160303,20.3650455205075,20.8622206249848,21.359395729462,
21.8565708339392,22.3537459384164,22.8509210428936,23.3480961473708,23.845271251848,
24.3424463563253,24.8396214608025,25.3367965652797,25.8339716697569,26.3311467742341,
26.8283218787113,27.3254969831885,27.8226720876658,28.319847192143,28.8170222966202,
29.3141974010974,29.8113725055746,30.3085476100518,30.805722714529,31.3028978190063,
31.8000729234835,32.2972480279607,32.7944231324379,33.2915982369151,33.7887733413923,
34.2859484458695,34.7831235503468,35.280298654824,35.7774737593012,36.2746488637784,
36.7718239682556,37.2689990727328,37.76617417721,38.2633492816873,38.7605243861645,
39.2576994906417,39.7548745951189,40.2520496995961,40.7492248040733,41.2463999085505,
41.7435750130278,42.240750117505,42.7379252219822,43.2351003264594,43.7322754309366,
44.2294505354138,44.726625639891,45.2238007443683,45.7209758488455,46.2181509533227,
46.7153260577999,47.2125011622771,47.7096762667543,48.2068513712315,48.7040264757088,
49.201201580186,49.6983766846632,50.1955517891404,50.6927268936176,51.1899019980948,
51.687077102572,52.1842522070493,52.6814273115265,53.1786024160037,53.6757775204809,
54.1729526249581,54.6701277294353,55.1673028339125,55.6644779383898,56.161653042867,
56.6588281473442,57.1560032518214,57.6531783562986,58.1503534607758,58.647528565253,
59.1447036697303,59.6418787742075,60.1390538786847,60.6362289831619,61.1334040876391,
61.6305791921163,62.1277542965935,62.6249294010708,63.122104505548,63.6192796100252,
64.1164547145024,64.6136298189796,65.1108049234568,65.607980027934,66.1051551324113,
66.6023302368885,67.0995053413657,67.5966804458429,68.0938555503201,68.5910306547973,
69.0882057592745,69.5853808637518,70.082555968229,70.5797310727062,71.0769061771834,
71.5740812816606,72.0712563861378,72.568431490615,73.0656065950923,73.5627816995695,
74.0599568040467,74.5571319085239,75.0543070130011,75.5514821174783,76.0486572219556,
76.5458323264328,77.04300743091,77.5401825353872,78.0373576398644,78.5345327443416,
79.0317078488188,79.528882953296,80.0260580577733,80.5232331622505,81.0204082667277,
81.5175833712049,82.0147584756821,82.5119335801593,83.0091086846365,83.5062837891138,
84.003458893591,84.5006339980682,84.9978091025454,85.4949842070226,85.9921593114998,
86.4893344159771,86.9865095204543,87.4836846249315,87.9808597294087,88.4780348338859,
88.9752099383631,89.4723850428403,89.9695601473175,90.4667352517948,90.963910356272,
91.4610854607492,91.9582605652264,92.4554356697036,92.9526107741808,93.449785878658,
93.9469609831353,94.4441360876125,94.9413111920897,95.4384862965669,95.9356614010441,
96.4328365055213,96.9300116099986,97.4271867144758,97.924361818953,98.4215369234302,
98.9187120279074,99.4158871323846,99.9130622368618,100.410237341339,100.907412445816,
101.404587550293,101.901762654771,102.398937759248,102.896112863725,103.393287968202,
103.89046307268,104.387638177157,104.884813281634,105.381988386111,105.879163490588,
106.376338595066,106.873513699543,107.37068880402,107.867863908497,108.365039012974,
108.862214117452,109.359389221929,109.856564326406,110.353739430883,110.850914535361,
111.348089639838,111.845264744315,112.342439848792,112.839614953269,113.336790057747,
113.833965162224,114.331140266701,114.828315371178,115.325490475655,115.822665580133,
116.31984068461,116.817015789087,117.314190893564,117.811365998042,118.308541102519,
118.805716206996,119.302891311473,119.80006641595,120.297241520428,120.794416624905,
121.291591729382,121.788766833859,122.285941938336,122.783117042814,123.280292147291,
123.777467251768,124.274642356245,124.771817460723,125.2689925652,125.766167669677,
126.263342774154,126.760517878631,127.257692983109,127.754868087586,128.252043192063,
128.74921829654,129.246393401017,129.743568505495,130.240743609972,130.737918714449,
131.235093818926,131.732268923404,132.229444027881,132.726619132358,133.223794236835,
133.720969341312,134.21814444579,134.715319550267,135.212494654744,135.709669759221,
136.206844863698,136.704019968176,137.201195072653,137.69837017713,138.195545281607,
138.692720386085,139.189895490562,139.687070595039,140.184245699516,140.681420803993,
141.178595908471,141.675771012948,142.172946117425,142.670121221902,143.167296326379,
143.664471430857,144.161646535334,144.658821639811,145.155996744288,145.653171848766,
146.150346953243,146.64752205772,147.144697162197,147.641872266674,148.139047371152,
148.636222475629,149.133397580106,149.630572684583,150.12774778906,150.624922893538,
151.122097998015,151.619273102492,152.116448206969,152.613623311447,153.110798415924,
153.607973520401,154.105148624878,154.602323729355,155.099498833833,155.59667393831,
156.093849042787,156.591024147264,157.088199251742,157.585374356219,158.082549460696,
158.579724565173,159.07689966965,159.574074774128,160.071249878605,160.568424983082,
161.065600087559,161.562775192036,162.059950296514,162.557125400991,163.054300505468,
163.551475609945,164.048650714422,164.5458258189,165.043000923377,165.540176027854,
166.037351132331,166.534526236809,167.031701341286,167.528876445763,168.02605155024,
168.523226654717,169.020401759195,169.517576863672,170.014751968149,170.511927072626,
171.009102177104,171.506277281581,172.003452386058,172.500627490535,172.997802595012,
173.49497769949),.UNSPECIFIED.);
#641=B_SPLINE_CURVE_WITH_KNOTS('',3,(#37345,#37346,#37347,#37348,#37349,
#37350,#37351),.UNSPECIFIED.,.F.,.F.,(4,3,4),(158.388651680658,158.598858328231,
159.096033432709),.UNSPECIFIED.);
#642=B_SPLINE_CURVE_WITH_KNOTS('',3,(#37359,#37360,#37361,#37362,#37363,
#37364,#37365,#37366,#37367,#37368,#37369,#37370,#37371,#37372,#37373,#37374),
 .UNSPECIFIED.,.F.,.F.,(4,3,3,3,3,4),(-157.079632679489,-156.610157910323,
-156.112982805845,-155.615807701368,-155.118632596891,-154.645421777951),
 .UNSPECIFIED.);
#643=B_SPLINE_CURVE_WITH_KNOTS('',3,(#37379,#37380,#37381,#37382,#37383,
#37384,#37385,#37386,#37387,#37388,#37389,#37390,#37391,#37392,#37393,#37394,
#37395,#37396,#37397,#37398,#37399,#37400,#37401,#37402,#37403,#37404,#37405,
#37406,#37407,#37408,#37409,#37410,#37411,#37412,#37413,#37414,#37415,#37416,
#37417,#37418,#37419,#37420,#37421),.UNSPECIFIED.,.F.,.F.,(4,3,3,3,3,3,
3,3,3,3,3,3,3,3,4),(152.105466373478,152.135581970028,152.632757074505,
153.129932178982,153.627107283459,154.124282387936,154.621457492414,155.118632596891,
155.615807701368,156.112982805845,156.610157910323,157.1073330148,157.604508119277,
158.101683223754,158.388651680658),.UNSPECIFIED.);
#644=B_SPLINE_CURVE_WITH_KNOTS('',3,(#37422,#37423,#37424,#37425,#37426,
#37427,#37428,#37429,#37430,#37431,#37432,#37433,#37434,#37435,#37436,#37437,
#37438,#37439,#37440,#37441,#37442,#37443,#37444,#37445,#37446,#37447,#37448,
#37449,#37450,#37451,#37452,#37453,#37454,#37455,#37456,#37457,#37458,#37459,
#37460,#37461,#37462,#37463,#37464),.UNSPECIFIED.,.F.,.F.,(4,3,3,3,3,3,
3,3,3,3,3,3,3,3,4),(-154.645421777951,-154.621457492414,-154.124282387936,
-153.627107283459,-153.129932178982,-152.632757074505,-152.135581970028,
-151.63840686555,-151.141231761073,-150.644056656596,-150.146881552119,
-149.649706447642,-149.152531343164,-148.655356238687,-148.362236470772),
 .UNSPECIFIED.);
#645=B_SPLINE_CURVE_WITH_KNOTS('',3,(#37469,#37470,#37471,#37472,#37473,
#37474,#37475,#37476,#37477,#37478,#37479,#37480,#37481,#37482,#37483,#37484,
#37485,#37486,#37487,#37488,#37489,#37490,#37491,#37492,#37493,#37494,#37495,
#37496,#37497,#37498,#37499,#37500,#37501,#37502,#37503,#37504,#37505,#37506,
#37507,#37508),.UNSPECIFIED.,.F.,.F.,(4,3,3,3,3,3,3,3,3,3,3,3,3,4),(145.822281066299,
146.169480716301,146.666655820778,147.163830925255,147.661006029733,148.15818113421,
148.655356238687,149.152531343164,149.649706447642,150.146881552119,150.644056656596,
151.141231761073,151.63840686555,152.105466373478),.UNSPECIFIED.);
#646=B_SPLINE_CURVE_WITH_KNOTS('',3,(#37509,#37510,#37511,#37512,#37513,
#37514,#37515,#37516,#37517,#37518,#37519,#37520,#37521,#37522,#37523,#37524,
#37525,#37526,#37527,#37528,#37529,#37530,#37531,#37532,#37533,#37534,#37535,
#37536,#37537,#37538,#37539,#37540,#37541,#37542,#37543,#37544,#37545,#37546,
#37547,#37548,#37549,#37550,#37551),.UNSPECIFIED.,.F.,.F.,(4,3,3,3,3,3,
3,3,3,3,3,3,3,3,4),(-148.362236470772,-148.15818113421,-147.661006029733,
-147.163830925255,-146.666655820778,-146.169480716301,-145.672305611824,
-145.175130507347,-144.677955402869,-144.180780298392,-143.683605193915,
-143.186430089438,-142.689254984961,-142.192079880483,-142.079051163592),
 .UNSPECIFIED.);
#647=B_SPLINE_CURVE_WITH_KNOTS('',3,(#37556,#37557,#37558,#37559,#37560,
#37561,#37562,#37563,#37564,#37565,#37566,#37567,#37568,#37569,#37570,#37571,
#37572,#37573,#37574,#37575,#37576,#37577,#37578,#37579,#37580,#37581,#37582,
#37583,#37584,#37585,#37586,#37587,#37588,#37589,#37590,#37591,#37592,#37593,
#37594,#37595,#37596,#37597,#37598),.UNSPECIFIED.,.F.,.F.,(4,3,3,3,3,3,
3,3,3,3,3,3,3,3,4),(139.539095759119,139.706204358097,140.203379462574,
140.700554567052,141.197729671529,141.694904776006,142.192079880483,142.689254984961,
143.186430089438,143.683605193915,144.180780298392,144.677955402869,145.175130507347,
145.672305611824,145.822281066299),.UNSPECIFIED.);
#648=B_SPLINE_CURVE_WITH_KNOTS('',3,(#37599,#37600,#37601,#37602,#37603,
#37604,#37605,#37606,#37607,#37608,#37609,#37610,#37611,#37612,#37613,#37614,
#37615,#37616,#37617,#37618,#37619,#37620,#37621,#37622,#37623,#37624,#37625,
#37626,#37627,#37628,#37629,#37630,#37631,#37632,#37633,#37634,#37635,#37636,
#37637,#37638),.UNSPECIFIED.,.F.,.F.,(4,3,3,3,3,3,3,3,3,3,3,3,3,4),(-142.079051163592,
-141.694904776006,-141.197729671529,-140.700554567052,-140.203379462574,
-139.706204358097,-139.20902925362,-138.711854149143,-138.214679044666,
-137.717503940188,-137.220328835711,-136.723153731234,-136.225978626757,
-135.795865856412),.UNSPECIFIED.);
#649=B_SPLINE_CURVE_WITH_KNOTS('',3,(#37643,#37644,#37645,#37646,#37647,
#37648,#37649,#37650,#37651,#37652,#37653,#37654,#37655,#37656,#37657,#37658,
#37659,#37660,#37661,#37662,#37663,#37664,#37665,#37666,#37667,#37668,#37669,
#37670,#37671,#37672,#37673,#37674,#37675,#37676,#37677,#37678,#37679,#37680,
#37681,#37682),.UNSPECIFIED.,.F.,.F.,(4,3,3,3,3,3,3,3,3,3,3,3,3,4),(133.255910451939,
133.740103104371,134.237278208848,134.734453313325,135.231628417802,135.72880352228,
136.225978626757,136.723153731234,137.220328835711,137.717503940188,138.214679044666,
138.711854149143,139.20902925362,139.539095759119),.UNSPECIFIED.);
#650=B_SPLINE_CURVE_WITH_KNOTS('',3,(#37683,#37684,#37685,#37686,#37687,
#37688,#37689,#37690,#37691,#37692,#37693,#37694,#37695,#37696,#37697,#37698,
#37699,#37700,#37701,#37702,#37703,#37704,#37705,#37706,#37707,#37708,#37709,
#37710,#37711,#37712,#37713,#37714,#37715,#37716,#37717,#37718,#37719,#37720,
#37721,#37722,#37723,#37724,#37725),.UNSPECIFIED.,.F.,.F.,(4,3,3,3,3,3,
3,3,3,3,3,3,3,3,4),(-135.795865856412,-135.72880352228,-135.231628417802,
-134.734453313325,-134.237278208848,-133.740103104371,-133.242927999893,
-132.745752895416,-132.248577790939,-131.751402686462,-131.254227581985,
-130.757052477507,-130.25987737303,-129.762702268553,-129.512680549233),
 .UNSPECIFIED.);
#651=B_SPLINE_CURVE_WITH_KNOTS('',3,(#37730,#37731,#37732,#37733,#37734,
#37735,#37736,#37737,#37738,#37739,#37740,#37741,#37742,#37743,#37744,#37745,
#37746,#37747,#37748,#37749,#37750,#37751,#37752,#37753,#37754,#37755,#37756,
#37757,#37758,#37759,#37760,#37761,#37762,#37763,#37764,#37765,#37766,#37767,
#37768,#37769,#37770,#37771,#37772),.UNSPECIFIED.,.F.,.F.,(4,3,3,3,3,3,
3,3,3,3,3,3,3,3,4),(126.97272514476,127.276826746167,127.774001850644,128.271176955121,
128.768352059598,129.265527164076,129.762702268553,130.25987737303,130.757052477507,
131.254227581985,131.751402686462,132.248577790939,132.745752895416,133.242927999893,
133.255910451939),.UNSPECIFIED.);
#652=B_SPLINE_CURVE_WITH_KNOTS('',3,(#37773,#37774,#37775,#37776,#37777,
#37778,#37779,#37780,#37781,#37782,#37783,#37784,#37785,#37786,#37787,#37788,
#37789,#37790,#37791,#37792,#37793,#37794,#37795,#37796,#37797,#37798,#37799,
#37800,#37801,#37802,#37803,#37804,#37805,#37806,#37807,#37808,#37809,#37810,
#37811,#37812,#37813,#37814,#37815),.UNSPECIFIED.,.F.,.F.,(4,3,3,3,3,3,
3,3,3,3,3,3,3,3,4),(-129.512680549233,-129.265527164076,-128.768352059599,
-128.271176955121,-127.774001850644,-127.276826746167,-126.77965164169,
-126.282476537213,-125.785301432735,-125.288126328258,-124.790951223781,
-124.293776119304,-123.796601014826,-123.299425910349,-123.229495242054),
 .UNSPECIFIED.);
#653=B_SPLINE_CURVE_WITH_KNOTS('',3,(#37820,#37821,#37822,#37823,#37824,
#37825,#37826,#37827,#37828,#37829,#37830,#37831,#37832,#37833,#37834,#37835,
#37836,#37837,#37838,#37839,#37840,#37841,#37842,#37843,#37844,#37845,#37846,
#37847,#37848,#37849,#37850,#37851,#37852,#37853,#37854,#37855,#37856,#37857,
#37858,#37859,#37860,#37861,#37862),.UNSPECIFIED.,.F.,.F.,(4,3,3,3,3,3,
3,3,3,3,3,3,3,3,4),(120.68953983758,120.813550387963,121.31072549244,121.807900596918,
122.305075701395,122.802250805872,123.299425910349,123.796601014826,124.293776119304,
124.790951223781,125.288126328258,125.785301432735,126.282476537212,126.77965164169,
126.97272514476),.UNSPECIFIED.);
#654=B_SPLINE_CURVE_WITH_KNOTS('',3,(#37863,#37864,#37865,#37866,#37867,
#37868,#37869,#37870,#37871,#37872,#37873,#37874,#37875,#37876,#37877,#37878,
#37879,#37880,#37881,#37882,#37883,#37884,#37885,#37886,#37887,#37888,#37889,
#37890,#37891,#37892,#37893,#37894,#37895,#37896,#37897,#37898,#37899,#37900,
#37901,#37902),.UNSPECIFIED.,.F.,.F.,(4,3,3,3,3,3,3,3,3,3,3,3,3,4),(-123.229495242054,
-122.802250805872,-122.305075701395,-121.807900596918,-121.31072549244,
-120.813550387963,-120.316375283486,-119.819200179009,-119.322025074531,
-118.824849970054,-118.327674865577,-117.8304997611,-117.333324656623,-116.946309934874),
 .UNSPECIFIED.);
#655=B_SPLINE_CURVE_WITH_KNOTS('',3,(#37907,#37908,#37909,#37910,#37911,
#37912,#37913,#37914,#37915,#37916,#37917,#37918,#37919,#37920,#37921,#37922,
#37923,#37924,#37925,#37926,#37927,#37928,#37929,#37930,#37931,#37932,#37933,
#37934,#37935,#37936,#37937,#37938,#37939,#37940,#37941,#37942,#37943,#37944,
#37945,#37946),.UNSPECIFIED.,.F.,.F.,(4,3,3,3,3,3,3,3,3,3,3,3,3,4),(114.406354530401,
114.847449134237,115.344624238714,115.841799343191,116.338974447668,116.836149552145,
117.333324656623,117.8304997611,118.327674865577,118.824849970054,119.322025074531,
119.819200179009,120.316375283486,120.68953983758),.UNSPECIFIED.);
#656=B_SPLINE_CURVE_WITH_KNOTS('',3,(#37947,#37948,#37949,#37950,#37951,
#37952,#37953,#37954,#37955,#37956,#37957,#37958,#37959,#37960,#37961,#37962,
#37963,#37964,#37965,#37966,#37967,#37968,#37969,#37970,#37971,#37972,#37973,
#37974,#37975,#37976,#37977,#37978,#37979,#37980,#37981,#37982,#37983,#37984,
#37985,#37986,#37987,#37988,#37989),.UNSPECIFIED.,.F.,.F.,(4,3,3,3,3,3,
3,3,3,3,3,3,3,3,4),(-116.946309934874,-116.836149552145,-116.338974447668,
-115.841799343191,-115.344624238714,-114.847449134237,-114.350274029759,
-113.853098925282,-113.355923820805,-112.858748716328,-112.36157361185,
-111.864398507373,-111.367223402896,-110.870048298419,-110.663124627694),
 .UNSPECIFIED.);
#657=B_SPLINE_CURVE_WITH_KNOTS('',3,(#37994,#37995,#37996,#37997,#37998,
#37999,#38000,#38001,#38002,#38003,#38004,#38005,#38006,#38007,#38008,#38009,
#38010,#38011,#38012,#38013,#38014,#38015,#38016,#38017,#38018,#38019,#38020,
#38021,#38022,#38023,#38024,#38025,#38026,#38027,#38028,#38029,#38030,#38031,
#38032,#38033,#38034,#38035,#38036),.UNSPECIFIED.,.F.,.F.,(4,3,3,3,3,3,
3,3,3,3,3,3,3,3,4),(108.123169223221,108.384172776033,108.88134788051,109.378522984987,
109.875698089464,110.372873193942,110.870048298419,111.367223402896,111.864398507373,
112.36157361185,112.858748716328,113.355923820805,113.853098925282,114.350274029759,
114.406354530401),.UNSPECIFIED.);
#658=B_SPLINE_CURVE_WITH_KNOTS('',3,(#38037,#38038,#38039,#38040,#38041,
#38042,#38043,#38044,#38045,#38046,#38047,#38048,#38049,#38050,#38051,#38052,
#38053,#38054,#38055,#38056,#38057,#38058,#38059,#38060,#38061,#38062,#38063,
#38064,#38065,#38066,#38067,#38068,#38069,#38070,#38071,#38072,#38073,#38074,
#38075,#38076,#38077,#38078,#38079),.UNSPECIFIED.,.F.,.F.,(4,3,3,3,3,3,
3,3,3,3,3,3,3,3,4),(-110.663124627694,-110.372873193942,-109.875698089464,
-109.378522984987,-108.88134788051,-108.384172776033,-107.886997671556,
-107.389822567078,-106.892647462601,-106.395472358124,-105.898297253647,
-105.401122149169,-104.903947044692,-104.406771940215,-104.379939320514),
 .UNSPECIFIED.);
#659=B_SPLINE_CURVE_WITH_KNOTS('',3,(#38084,#38085,#38086,#38087,#38088,
#38089,#38090,#38091,#38092,#38093,#38094,#38095,#38096,#38097,#38098,#38099,
#38100,#38101,#38102,#38103,#38104,#38105,#38106,#38107,#38108,#38109,#38110,
#38111,#38112,#38113,#38114,#38115,#38116,#38117,#38118,#38119,#38120,#38121,
#38122,#38123,#38124,#38125,#38126),.UNSPECIFIED.,.F.,.F.,(4,3,3,3,3,3,
3,3,3,3,3,3,3,3,4),(101.839983916041,101.920896417829,102.418071522306,
102.915246626783,103.412421731261,103.909596835738,104.406771940215,104.903947044692,
105.401122149169,105.898297253647,106.395472358124,106.892647462601,107.389822567078,
107.886997671556,108.123169223221),.UNSPECIFIED.);
#660=B_SPLINE_CURVE_WITH_KNOTS('',3,(#38127,#38128,#38129,#38130,#38131,
#38132,#38133,#38134,#38135,#38136,#38137,#38138,#38139,#38140,#38141,#38142,
#38143,#38144,#38145,#38146,#38147,#38148,#38149,#38150,#38151,#38152,#38153,
#38154,#38155,#38156,#38157,#38158,#38159,#38160,#38161,#38162,#38163,#38164,
#38165,#38166),.UNSPECIFIED.,.F.,.F.,(4,3,3,3,3,3,3,3,3,3,3,3,3,4),(-104.379939320514,
-103.909596835738,-103.412421731261,-102.915246626783,-102.418071522306,
-101.920896417829,-101.423721313352,-100.926546208875,-100.429371104397,
-99.9321959999201,-99.4350208954429,-98.9378457909657,-98.4406706864885,
-98.0967540133348),.UNSPECIFIED.);
#661=B_SPLINE_CURVE_WITH_KNOTS('',3,(#38171,#38172,#38173,#38174,#38175,
#38176,#38177,#38178,#38179,#38180,#38181,#38182,#38183,#38184,#38185,#38186,
#38187,#38188,#38189,#38190,#38191,#38192,#38193,#38194,#38195,#38196,#38197,
#38198,#38199,#38200,#38201,#38202,#38203,#38204,#38205,#38206,#38207,#38208,
#38209,#38210),.UNSPECIFIED.,.F.,.F.,(4,3,3,3,3,3,3,3,3,3,3,3,3,4),(95.5567986088618,
95.9547951641024,96.4519702685796,96.9491453730568,97.446320477534,97.9434955820112,
98.4406706864884,98.9378457909657,99.4350208954429,99.9321959999201,100.429371104397,
100.926546208875,101.423721313352,101.839983916041),.UNSPECIFIED.);
#662=B_SPLINE_CURVE_WITH_KNOTS('',3,(#38211,#38212,#38213,#38214,#38215,
#38216,#38217,#38218,#38219,#38220,#38221,#38222,#38223,#38224,#38225,#38226,
#38227,#38228,#38229,#38230,#38231,#38232,#38233,#38234,#38235,#38236,#38237,
#38238,#38239,#38240,#38241,#38242,#38243,#38244,#38245,#38246,#38247,#38248,
#38249,#38250,#38251,#38252,#38253),.UNSPECIFIED.,.F.,.F.,(4,3,3,3,3,3,
3,3,3,3,3,3,3,3,4),(-98.0967540133348,-97.9434955820113,-97.446320477534,
-96.9491453730568,-96.4519702685796,-95.9547951641024,-95.4576200596252,
-94.960444955148,-94.4632698506707,-93.9660947461935,-93.4689196417163,
-92.9717445372391,-92.4745694327619,-91.9773943282847,-91.8135687061551),
 .UNSPECIFIED.);
#663=B_SPLINE_CURVE_WITH_KNOTS('',3,(#38258,#38259,#38260,#38261,#38262,
#38263,#38264,#38265,#38266,#38267,#38268,#38269,#38270,#38271,#38272,#38273,
#38274,#38275,#38276,#38277,#38278,#38279,#38280,#38281,#38282,#38283,#38284,
#38285,#38286,#38287,#38288,#38289,#38290,#38291,#38292,#38293,#38294,#38295,
#38296,#38297,#38298,#38299,#38300),.UNSPECIFIED.,.F.,.F.,(4,3,3,3,3,3,
3,3,3,3,3,3,3,3,4),(89.2736133016821,89.4915188058986,89.9886939103758,
90.485869014853,90.9830441193302,91.4802192238075,91.9773943282847,92.4745694327619,
92.9717445372391,93.4689196417163,93.9660947461935,94.4632698506707,94.9604449551479,
95.4576200596252,95.5567986088618),.UNSPECIFIED.);
#664=B_SPLINE_CURVE_WITH_KNOTS('',3,(#38301,#38302,#38303,#38304,#38305,
#38306,#38307,#38308,#38309,#38310,#38311,#38312,#38313,#38314,#38315,#38316,
#38317,#38318,#38319,#38320,#38321,#38322,#38323,#38324,#38325,#38326,#38327,
#38328,#38329,#38330,#38331,#38332,#38333,#38334,#38335,#38336,#38337,#38338,
#38339,#38340),.UNSPECIFIED.,.F.,.F.,(4,3,3,3,3,3,3,3,3,3,3,3,3,4),(-91.8135687061551,
-91.4802192238075,-90.9830441193302,-90.485869014853,-89.9886939103758,
-89.4915188058986,-88.9943437014214,-88.4971685969442,-87.9999934924669,
-87.5028183879897,-87.0056432835125,-86.5084681790353,-86.0112930745581,
-85.5303833989759),.UNSPECIFIED.);
#665=B_SPLINE_CURVE_WITH_KNOTS('',3,(#38345,#38346,#38347,#38348,#38349,
#38350,#38351,#38352,#38353,#38354,#38355,#38356,#38357,#38358,#38359,#38360,
#38361,#38362,#38363,#38364,#38365,#38366,#38367,#38368,#38369,#38370,#38371,
#38372,#38373,#38374,#38375,#38376,#38377,#38378,#38379,#38380,#38381,#38382,
#38383,#38384,#38385,#38386,#38387),.UNSPECIFIED.,.F.,.F.,(4,3,3,3,3,3,
3,3,3,3,3,3,3,3,4),(82.9904279945029,83.0282424476948,83.525417552172,84.0225926566493,
84.5197677611265,85.0169428656037,85.5141179700809,86.0112930745581,86.5084681790353,
87.0056432835125,87.5028183879897,87.9999934924669,88.4971685969441,88.9943437014214,
89.2736133016821),.UNSPECIFIED.);
#666=B_SPLINE_CURVE_WITH_KNOTS('',3,(#38388,#38389,#38390,#38391,#38392,
#38393,#38394,#38395,#38396,#38397,#38398,#38399,#38400,#38401,#38402,#38403,
#38404,#38405,#38406,#38407,#38408,#38409,#38410,#38411,#38412,#38413,#38414,
#38415,#38416,#38417,#38418,#38419,#38420,#38421,#38422,#38423,#38424,#38425,
#38426,#38427,#38428,#38429,#38430),.UNSPECIFIED.,.F.,.F.,(4,3,3,3,3,3,
3,3,3,3,3,3,3,3,4),(-85.5303833989759,-85.5141179700809,-85.0169428656037,
-84.5197677611264,-84.0225926566492,-83.525417552172,-83.0282424476948,
-82.5310673432176,-82.0338922387404,-81.5367171342632,-81.039542029786,
-80.5423669253087,-80.0451918208315,-79.5480167163543,-79.2471980917962),
 .UNSPECIFIED.);
#667=B_SPLINE_CURVE_WITH_KNOTS('',3,(#38435,#38436,#38437,#38438,#38439,
#38440,#38441,#38442,#38443,#38444,#38445,#38446,#38447,#38448,#38449,#38450,
#38451,#38452,#38453,#38454,#38455,#38456,#38457,#38458,#38459,#38460,#38461,
#38462,#38463,#38464,#38465,#38466,#38467,#38468,#38469,#38470,#38471,#38472,
#38473,#38474),.UNSPECIFIED.,.F.,.F.,(4,3,3,3,3,3,3,3,3,3,3,3,3,4),(76.7072426873232,
77.0621411939682,77.5593162984454,78.0564914029227,78.5536665073999,79.0508416118771,
79.5480167163543,80.0451918208315,80.5423669253087,81.0395420297859,81.5367171342632,
82.0338922387404,82.5310673432176,82.9904279945029),.UNSPECIFIED.);
#668=B_SPLINE_CURVE_WITH_KNOTS('',3,(#38475,#38476,#38477,#38478,#38479,
#38480,#38481,#38482,#38483,#38484,#38485,#38486,#38487,#38488,#38489,#38490,
#38491,#38492,#38493,#38494,#38495,#38496,#38497,#38498,#38499,#38500,#38501,
#38502,#38503,#38504,#38505,#38506,#38507,#38508,#38509,#38510,#38511,#38512,
#38513,#38514,#38515,#38516,#38517),.UNSPECIFIED.,.F.,.F.,(4,3,3,3,3,3,
3,3,3,3,3,3,3,3,4),(-79.2471980917962,-79.0508416118771,-78.5536665073999,
-78.0564914029227,-77.5593162984455,-77.0621411939683,-76.564966089491,
-76.0677909850138,-75.5706158805366,-75.0734407760594,-74.5762656715822,
-74.079090567105,-73.5819154626277,-73.0847403581505,-72.9640127846165),
 .UNSPECIFIED.);
#669=B_SPLINE_CURVE_WITH_KNOTS('',3,(#38522,#38523,#38524,#38525,#38526,
#38527,#38528,#38529,#38530,#38531,#38532,#38533,#38534,#38535,#38536,#38537,
#38538,#38539,#38540,#38541,#38542,#38543,#38544,#38545,#38546,#38547,#38548,
#38549,#38550,#38551,#38552,#38553,#38554,#38555,#38556,#38557,#38558,#38559,
#38560,#38561,#38562,#38563,#38564),.UNSPECIFIED.,.F.,.F.,(4,3,3,3,3,3,
3,3,3,3,3,3,3,3,4),(70.4240573801435,70.5988648357644,71.0960399402417,
71.5932150447189,72.0903901491961,72.5875652536733,73.0847403581505,73.5819154626277,
74.0790905671049,74.5762656715822,75.0734407760594,75.5706158805366,76.0677909850138,
76.564966089491,76.7072426873232),.UNSPECIFIED.);
#670=B_SPLINE_CURVE_WITH_KNOTS('',3,(#38565,#38566,#38567,#38568,#38569,
#38570,#38571,#38572,#38573,#38574,#38575,#38576,#38577,#38578,#38579,#38580,
#38581,#38582,#38583,#38584,#38585,#38586,#38587,#38588,#38589,#38590,#38591,
#38592,#38593,#38594,#38595,#38596,#38597,#38598,#38599,#38600,#38601,#38602,
#38603,#38604),.UNSPECIFIED.,.F.,.F.,(4,3,3,3,3,3,3,3,3,3,3,3,3,4),(-72.9640127846165,
-72.5875652536733,-72.0903901491961,-71.5932150447189,-71.0960399402417,
-70.5988648357645,-70.1016897312873,-69.60451462681,-69.1073395223328,-68.6101644178556,
-68.1129893133784,-67.6158142089012,-67.1186391044239,-66.6808274774369),
 .UNSPECIFIED.);
#671=B_SPLINE_CURVE_WITH_KNOTS('',3,(#38609,#38610,#38611,#38612,#38613,
#38614,#38615,#38616,#38617,#38618,#38619,#38620,#38621,#38622,#38623,#38624,
#38625,#38626,#38627,#38628,#38629,#38630,#38631,#38632,#38633,#38634,#38635,
#38636,#38637,#38638,#38639,#38640,#38641,#38642,#38643,#38644,#38645,#38646,
#38647,#38648),.UNSPECIFIED.,.F.,.F.,(4,3,3,3,3,3,3,3,3,3,3,3,3,4),(64.1408720729639,
64.6327635820379,65.1299386865151,65.6271137909923,66.1242888954695,66.6214639999467,
67.1186391044239,67.6158142089012,68.1129893133784,68.6101644178556,69.1073395223328,
69.60451462681,70.1016897312872,70.4240573801435),.UNSPECIFIED.);
#672=B_SPLINE_CURVE_WITH_KNOTS('',3,(#38649,#38650,#38651,#38652,#38653,
#38654,#38655,#38656,#38657,#38658,#38659,#38660,#38661,#38662,#38663,#38664,
#38665,#38666,#38667,#38668,#38669,#38670,#38671,#38672,#38673,#38674,#38675,
#38676,#38677,#38678,#38679,#38680,#38681,#38682,#38683,#38684,#38685,#38686,
#38687,#38688,#38689,#38690,#38691),.UNSPECIFIED.,.F.,.F.,(4,3,3,3,3,3,
3,3,3,3,3,3,3,3,4),(-66.6808274774369,-66.6214639999467,-66.1242888954695,
-65.6271137909923,-65.1299386865151,-64.6327635820379,-64.1355884775607,
-63.6384133730835,-63.1412382686062,-62.644063164129,-62.1468880596518,
-61.6497129551746,-61.1525378506974,-60.6553627462202,-60.3976421702572),
 .UNSPECIFIED.);
#673=B_SPLINE_CURVE_WITH_KNOTS('',3,(#38696,#38697,#38698,#38699,#38700,
#38701,#38702,#38703,#38704,#38705,#38706,#38707,#38708,#38709,#38710,#38711,
#38712,#38713,#38714,#38715,#38716,#38717,#38718,#38719,#38720,#38721,#38722,
#38723,#38724,#38725,#38726,#38727,#38728,#38729,#38730,#38731,#38732,#38733,
#38734,#38735,#38736,#38737,#38738),.UNSPECIFIED.,.F.,.F.,(4,3,3,3,3,3,
3,3,3,3,3,3,3,3,4),(57.8576867657842,58.1694872238341,58.6666623283113,
59.1638374327885,59.6610125372657,60.1581876417429,60.6553627462201,61.1525378506974,
61.6497129551746,62.1468880596518,62.644063164129,63.1412382686062,63.6384133730835,
64.1355884775607,64.1408720729639),.UNSPECIFIED.);
#674=B_SPLINE_CURVE_WITH_KNOTS('',3,(#38739,#38740,#38741,#38742,#38743,
#38744,#38745,#38746,#38747,#38748,#38749,#38750,#38751,#38752,#38753,#38754,
#38755,#38756,#38757,#38758,#38759,#38760,#38761,#38762,#38763,#38764,#38765,
#38766,#38767,#38768,#38769,#38770,#38771,#38772,#38773,#38774,#38775,#38776,
#38777,#38778,#38779,#38780,#38781),.UNSPECIFIED.,.F.,.F.,(4,3,3,3,3,3,
3,3,3,3,3,3,3,3,4),(-60.3976421702572,-60.158187641743,-59.6610125372657,
-59.1638374327885,-58.6666623283113,-58.1694872238341,-57.6723121193569,
-57.1751370148797,-56.6779619104025,-56.1807868059252,-55.683611701448,
-55.1864365969708,-54.6892614924936,-54.1920863880164,-54.114456863078),
 .UNSPECIFIED.);
#675=B_SPLINE_CURVE_WITH_KNOTS('',3,(#38786,#38787,#38788,#38789,#38790,
#38791,#38792,#38793,#38794,#38795,#38796,#38797,#38798,#38799,#38800,#38801,
#38802,#38803,#38804,#38805,#38806,#38807,#38808,#38809,#38810,#38811,#38812,
#38813,#38814,#38815,#38816,#38817,#38818,#38819,#38820,#38821,#38822,#38823,
#38824,#38825,#38826,#38827,#38828),.UNSPECIFIED.,.F.,.F.,(4,3,3,3,3,3,
3,3,3,3,3,3,3,3,4),(51.5745014586045,51.7062108656303,52.2033859701075,
52.7005610745847,53.1977361790619,53.6949112835391,54.1920863880164,54.6892614924936,
55.1864365969708,55.683611701448,56.1807868059252,56.6779619104024,57.1751370148797,
57.6723121193569,57.8576867657842),.UNSPECIFIED.);
#676=B_SPLINE_CURVE_WITH_KNOTS('',3,(#38829,#38830,#38831,#38832,#38833,
#38834,#38835,#38836,#38837,#38838,#38839,#38840,#38841,#38842,#38843,#38844,
#38845,#38846,#38847,#38848,#38849,#38850,#38851,#38852,#38853,#38854,#38855,
#38856,#38857,#38858,#38859,#38860,#38861,#38862,#38863,#38864,#38865,#38866,
#38867,#38868),.UNSPECIFIED.,.F.,.F.,(4,3,3,3,3,3,3,3,3,3,3,3,3,4),(-54.114456863078,
-53.6949112835392,-53.197736179062,-52.7005610745847,-52.2033859701075,
-51.7062108656303,-51.2090357611531,-50.7118606566759,-50.2146855521987,
-49.7175104477215,-49.2203353432442,-48.723160238767,-48.2259851342898,
-47.8312715558983),.UNSPECIFIED.);
#677=B_SPLINE_CURVE_WITH_KNOTS('',3,(#38873,#38874,#38875,#38876,#38877,
#38878,#38879,#38880,#38881,#38882,#38883,#38884,#38885,#38886,#38887,#38888,
#38889,#38890,#38891,#38892,#38893,#38894,#38895,#38896,#38897,#38898,#38899,
#38900,#38901,#38902,#38903,#38904,#38905,#38906,#38907,#38908,#38909,#38910,
#38911,#38912),.UNSPECIFIED.,.F.,.F.,(4,3,3,3,3,3,3,3,3,3,3,3,3,4),(45.2913161514253,
45.7401096119037,46.2372847163809,46.7344598208582,47.2316349253354,47.7288100298126,
48.2259851342898,48.723160238767,49.2203353432442,49.7175104477214,50.2146855521987,
50.7118606566759,51.2090357611531,51.5745014586045),.UNSPECIFIED.);
#678=B_SPLINE_CURVE_WITH_KNOTS('',3,(#38913,#38914,#38915,#38916,#38917,
#38918,#38919,#38920,#38921,#38922,#38923,#38924,#38925,#38926,#38927,#38928,
#38929,#38930,#38931,#38932,#38933,#38934,#38935,#38936,#38937,#38938,#38939,
#38940,#38941,#38942,#38943,#38944,#38945,#38946,#38947,#38948,#38949,#38950,
#38951,#38952,#38953,#38954,#38955),.UNSPECIFIED.,.F.,.F.,(4,3,3,3,3,3,
3,3,3,3,3,3,3,3,4),(-47.8312715558983,-47.7288100298126,-47.2316349253354,
-46.7344598208582,-46.2372847163809,-45.7401096119037,-45.2429345074265,
-44.7457594029493,-44.2485842984721,-43.7514091939949,-43.2542340895177,
-42.7570589850404,-42.2598838805632,-41.762708776086,-41.5480862487186),
 .UNSPECIFIED.);
#679=B_SPLINE_CURVE_WITH_KNOTS('',3,(#38960,#38961,#38962,#38963,#38964,
#38965,#38966,#38967,#38968,#38969,#38970,#38971,#38972,#38973,#38974,#38975,
#38976,#38977,#38978,#38979,#38980,#38981,#38982,#38983,#38984,#38985,#38986,
#38987,#38988,#38989,#38990,#38991,#38992,#38993,#38994,#38995,#38996,#38997,
#38998,#38999,#39000,#39001,#39002),.UNSPECIFIED.,.F.,.F.,(4,3,3,3,3,3,
3,3,3,3,3,3,3,3,4),(39.0081308442456,39.2768332536999,39.7740083581771,
40.2711834626544,40.7683585671316,41.2655336716088,41.762708776086,42.2598838805632,
42.7570589850404,43.2542340895177,43.7514091939949,44.2485842984721,44.7457594029493,
45.2429345074265,45.2913161514253),.UNSPECIFIED.);
#680=B_SPLINE_CURVE_WITH_KNOTS('',3,(#39003,#39004,#39005,#39006,#39007,
#39008,#39009,#39010,#39011,#39012,#39013,#39014,#39015,#39016,#39017,#39018,
#39019,#39020,#39021,#39022,#39023,#39024,#39025,#39026,#39027,#39028,#39029,
#39030,#39031,#39032,#39033,#39034,#39035,#39036,#39037,#39038,#39039,#39040,
#39041,#39042,#39043,#39044,#39045),.UNSPECIFIED.,.F.,.F.,(4,3,3,3,3,3,
3,3,3,3,3,3,3,3,4),(-41.5480862487186,-41.2655336716088,-40.7683585671316,
-40.2711834626544,-39.7740083581772,-39.2768332536999,-38.7796581492227,
-38.2824830447455,-37.7853079402683,-37.2881328357911,-36.7909577313139,
-36.2937826268367,-35.7966075223594,-35.2994324178822,-35.2649009415389),
 .UNSPECIFIED.);
#681=B_SPLINE_CURVE_WITH_KNOTS('',3,(#39050,#39051,#39052,#39053,#39054,
#39055,#39056,#39057,#39058,#39059,#39060,#39061,#39062,#39063,#39064,#39065,
#39066,#39067,#39068,#39069,#39070,#39071,#39072,#39073,#39074,#39075,#39076,
#39077,#39078,#39079,#39080,#39081,#39082,#39083,#39084,#39085,#39086,#39087,
#39088,#39089,#39090,#39091,#39092),.UNSPECIFIED.,.F.,.F.,(4,3,3,3,3,3,
3,3,3,3,3,3,3,3,4),(32.7249455370659,32.8135568954961,33.3107319999734,
33.8079071044506,34.3050822089278,34.802257313405,35.2994324178822,35.7966075223594,
36.2937826268367,36.7909577313139,37.2881328357911,37.7853079402683,38.2824830447455,
38.7796581492227,39.0081308442456),.UNSPECIFIED.);
#682=B_SPLINE_CURVE_WITH_KNOTS('',3,(#39093,#39094,#39095,#39096,#39097,
#39098,#39099,#39100,#39101,#39102,#39103,#39104,#39105,#39106,#39107,#39108,
#39109,#39110,#39111,#39112,#39113,#39114,#39115,#39116,#39117,#39118,#39119,
#39120,#39121,#39122,#39123,#39124,#39125,#39126,#39127,#39128,#39129,#39130,
#39131,#39132),.UNSPECIFIED.,.F.,.F.,(4,3,3,3,3,3,3,3,3,3,3,3,3,4),(-35.2649009415389,
-34.802257313405,-34.3050822089278,-33.8079071044506,-33.3107319999734,
-32.8135568954962,-32.3163817910189,-31.8192066865417,-31.3220315820645,
-30.8248564775873,-30.3276813731101,-29.8305062686329,-29.3333311641557,
-28.9817156343593),.UNSPECIFIED.);
#683=B_SPLINE_CURVE_WITH_KNOTS('',3,(#39137,#39138,#39139,#39140,#39141,
#39142,#39143,#39144,#39145,#39146,#39147,#39148,#39149,#39150,#39151,#39152,
#39153,#39154,#39155,#39156,#39157,#39158,#39159,#39160,#39161,#39162,#39163,
#39164,#39165,#39166,#39167,#39168,#39169,#39170,#39171,#39172,#39173,#39174,
#39175,#39176),.UNSPECIFIED.,.F.,.F.,(4,3,3,3,3,3,3,3,3,3,3,3,3,4),(26.4417602298863,
26.8474556417696,27.3446307462468,27.841805850724,28.3389809552012,28.8361560596784,
29.3333311641556,29.8305062686329,30.3276813731101,30.8248564775873,31.3220315820645,
31.8192066865417,32.3163817910189,32.7249455370659),.UNSPECIFIED.);
#684=B_SPLINE_CURVE_WITH_KNOTS('',3,(#39177,#39178,#39179,#39180,#39181,
#39182,#39183,#39184,#39185,#39186,#39187,#39188,#39189,#39190,#39191,#39192,
#39193,#39194,#39195,#39196,#39197,#39198,#39199,#39200,#39201,#39202,#39203,
#39204,#39205,#39206,#39207,#39208,#39209,#39210,#39211,#39212,#39213,#39214,
#39215,#39216,#39217,#39218,#39219),.UNSPECIFIED.,.F.,.F.,(4,3,3,3,3,3,
3,3,3,3,3,3,3,3,4),(-28.9817156343593,-28.8361560596784,-28.3389809552012,
-27.841805850724,-27.3446307462468,-26.8474556417696,-26.3502805372924,
-25.8531054328152,-25.3559303283379,-24.8587552238607,-24.3615801193835,
-23.8644050149063,-23.3672299104291,-22.8700548059519,-22.69853032718),
 .UNSPECIFIED.);
#685=B_SPLINE_CURVE_WITH_KNOTS('',3,(#39224,#39225,#39226,#39227,#39228,
#39229,#39230,#39231,#39232,#39233,#39234,#39235,#39236,#39237,#39238,#39239,
#39240,#39241,#39242,#39243,#39244,#39245,#39246,#39247,#39248,#39249,#39250,
#39251,#39252,#39253,#39254,#39255,#39256,#39257,#39258,#39259,#39260,#39261,
#39262,#39263,#39264,#39265,#39266),.UNSPECIFIED.,.F.,.F.,(4,3,3,3,3,3,
3,3,3,3,3,3,3,3,4),(20.1585749227066,20.3841792835658,20.881354388043,21.3785294925202,
21.8757045969974,22.3728797014746,22.8700548059519,23.3672299104291,23.8644050149063,
24.3615801193835,24.8587552238607,25.3559303283379,25.8531054328151,26.3502805372924,
26.4417602298863),.UNSPECIFIED.);
#686=B_SPLINE_CURVE_WITH_KNOTS('',3,(#39267,#39268,#39269,#39270,#39271,
#39272,#39273,#39274,#39275,#39276,#39277,#39278,#39279,#39280,#39281,#39282,
#39283,#39284,#39285,#39286,#39287,#39288,#39289,#39290,#39291,#39292,#39293,
#39294,#39295,#39296,#39297,#39298,#39299,#39300,#39301,#39302,#39303,#39304,
#39305,#39306),.UNSPECIFIED.,.F.,.F.,(4,3,3,3,3,3,3,3,3,3,3,3,3,4),(-22.69853032718,
-22.3728797014747,-21.8757045969974,-21.3785294925202,-20.881354388043,
-20.3841792835658,-19.8870041790886,-19.3898290746114,-18.8926539701342,
-18.3954788656569,-17.8983037611797,-17.4011286567025,-16.9039535522253,
-16.4153450200004),.UNSPECIFIED.);
#687=B_SPLINE_CURVE_WITH_KNOTS('',3,(#39311,#39312,#39313,#39314,#39315,
#39316,#39317,#39318,#39319,#39320,#39321,#39322,#39323,#39324,#39325,#39326,
#39327,#39328,#39329,#39330,#39331,#39332,#39333,#39334,#39335,#39336,#39337,
#39338,#39339,#39340,#39341,#39342,#39343,#39344,#39345,#39346,#39347,#39348,
#39349,#39350,#39351,#39352,#39353),.UNSPECIFIED.,.F.,.F.,(4,3,3,3,3,3,
3,3,3,3,3,3,3,3,4),(13.8753896155273,13.920902925362,14.4180780298392,14.9152531343164,
15.4124282387936,15.9096033432709,16.4067784477481,16.9039535522253,17.4011286567025,
17.8983037611797,18.3954788656569,18.8926539701341,19.3898290746114,19.8870041790886,
20.1585749227066),.UNSPECIFIED.);
#688=B_SPLINE_CURVE_WITH_KNOTS('',3,(#39354,#39355,#39356,#39357,#39358,
#39359,#39360,#39361,#39362,#39363,#39364,#39365,#39366,#39367,#39368,#39369,
#39370,#39371,#39372,#39373,#39374,#39375,#39376,#39377,#39378,#39379,#39380,
#39381,#39382,#39383,#39384,#39385,#39386,#39387,#39388,#39389,#39390,#39391,
#39392,#39393,#39394,#39395,#39396),.UNSPECIFIED.,.F.,.F.,(4,3,3,3,3,3,
3,3,3,3,3,3,3,3,4),(-16.4153450200004,-16.4067784477481,-15.9096033432709,
-15.4124282387936,-14.9152531343164,-14.4180780298392,-13.920902925362,
-13.4237278208848,-12.9265527164076,-12.4293776119304,-11.9322025074531,
-11.4350274029759,-10.9378522984987,-10.4406771940215,-10.1321597128207),
 .UNSPECIFIED.);
#689=B_SPLINE_CURVE_WITH_KNOTS('',3,(#39402,#39403,#39404,#39405,#39406,
#39407,#39408,#39409,#39410,#39411,#39412,#39413,#39414,#39415,#39416,#39417,
#39418,#39419,#39420,#39421,#39422,#39423,#39424,#39425,#39426),
 .UNSPECIFIED.,.F.,.F.,(4,3,3,3,3,3,3,3,4),(-3.848974405641,-3.4802257313405,
-2.98305062686329,-2.48587552238607,-1.98870041790886,-1.49152531343164,
-0.99435020895443,-0.497175104477215,0.),.UNSPECIFIED.);
#690=B_SPLINE_CURVE_WITH_KNOTS('',3,(#39429,#39430,#39431,#39432,#39433,
#39434,#39435,#39436,#39437,#39438,#39439,#39440,#39441,#39442,#39443,#39444,
#39445,#39446,#39447,#39448,#39449,#39450,#39451,#39452,#39453,#39454,#39455,
#39456,#39457,#39458,#39459,#39460,#39461,#39462,#39463,#39464,#39465),
 .UNSPECIFIED.,.F.,.F.,(4,3,3,3,3,3,3,3,3,3,3,3,4),(2.01640075321939,2.48587552238607,
2.98305062686328,3.4802257313405,3.97740083581771,4.47457594029493,4.97175104477214,
5.46892614924935,5.96610125372657,6.46327635820378,6.960451462681,7.45762656715821,
7.59220430834767),.UNSPECIFIED.);
#691=B_SPLINE_CURVE_WITH_KNOTS('',3,(#39471,#39472,#39473,#39474,#39475,
#39476,#39477,#39478,#39479,#39480,#39481,#39482),.UNSPECIFIED.,.F.,.F.,
(4,1,1,1,1,1,1,1,1,4),(166.504410640259,166.977621459199,167.474796563676,
167.971971668153,168.46914677263,168.966321877108,169.463496981585,169.960672086062,
170.457847190539,170.955022295017),.UNSPECIFIED.);
#692=B_SPLINE_CURVE_WITH_KNOTS('',3,(#39485,#39486,#39487,#39488,#39489,
#39490,#39491,#39492,#39493,#39494,#39495,#39496,#39497,#39498),
 .UNSPECIFIED.,.F.,.F.,(4,1,1,1,1,1,1,1,1,1,1,4),(166.504410640259,166.534526236809,
167.031701341286,167.528876445763,168.02605155024,168.523226654717,169.020401759195,
169.517576863672,170.014751968149,170.511927072626,171.009102177104,171.47857694627),
 .UNSPECIFIED.);
#693=B_SPLINE_CURVE_WITH_KNOTS('',3,(#39503,#39504,#39505,#39506,#39507,
#39508,#39509,#39510,#39511,#39512,#39513,#39514,#39515,#39516,#39517,#39518,
#39519),.UNSPECIFIED.,.F.,.F.,(4,1,1,1,1,1,1,1,1,1,1,1,1,1,4),(160.22122533308,
160.514345100995,161.011520205472,161.508695309949,162.005870414427,162.503045518904,
163.000220623381,163.497395727858,163.994570832336,164.491745936813,164.98892104129,
165.486096145767,165.983271250244,166.480446354722,166.504410640259),
 .UNSPECIFIED.);
#694=B_SPLINE_CURVE_WITH_KNOTS('',3,(#39520,#39521,#39522,#39523,#39524,
#39525,#39526,#39527,#39528,#39529,#39530,#39531,#39532,#39533,#39534,#39535),
 .UNSPECIFIED.,.F.,.F.,(4,1,1,1,1,1,1,1,1,1,1,1,1,4),(160.22122533308,160.568424983082,
161.065600087559,161.562775192036,162.059950296514,162.557125400991,163.054300505468,
163.551475609945,164.048650714422,164.5458258189,165.043000923377,165.540176027854,
166.037351132331,166.504410640259),.UNSPECIFIED.);
#695=B_SPLINE_CURVE_WITH_KNOTS('',3,(#39540,#39541,#39542,#39543,#39544,
#39545,#39546,#39547,#39548,#39549,#39550,#39551,#39552,#39553,#39554,#39555,
#39556),.UNSPECIFIED.,.F.,.F.,(4,1,1,1,1,1,1,1,1,1,1,1,1,1,4),(153.9380400259,
154.051068742791,154.548243847269,155.045418951746,155.542594056223,156.0397691607,
156.536944265177,157.034119369655,157.531294474132,158.028469578609,158.525644683086,
159.022819787563,159.519994892041,160.017169996518,160.22122533308),
 .UNSPECIFIED.);
#696=B_SPLINE_CURVE_WITH_KNOTS('',3,(#39557,#39558,#39559,#39560,#39561,
#39562,#39563,#39564,#39565,#39566,#39567,#39568,#39569,#39570,#39571,#39572,
#39573),.UNSPECIFIED.,.F.,.F.,(4,1,1,1,1,1,1,1,1,1,1,1,1,1,4),(153.9380400259,
154.105148624878,154.602323729355,155.099498833833,155.59667393831,156.093849042787,
156.591024147264,157.088199251742,157.585374356219,158.082549460696,158.579724565173,
159.07689966965,159.574074774128,160.071249878605,160.22122533308),
 .UNSPECIFIED.);
#697=B_SPLINE_CURVE_WITH_KNOTS('',3,(#39578,#39579,#39580,#39581,#39582,
#39583,#39584,#39585,#39586,#39587,#39588,#39589,#39590,#39591,#39592,#39593),
 .UNSPECIFIED.,.F.,.F.,(4,1,1,1,1,1,1,1,1,1,1,1,1,4),(147.65485471872,148.084967489065,
148.582142593542,149.079317698019,149.576492802496,150.073667906974,150.570843011451,
151.068018115928,151.565193220405,152.062368324882,152.55954342936,153.056718533837,
153.553893638314,153.9380400259),.UNSPECIFIED.);
#698=B_SPLINE_CURVE_WITH_KNOTS('',3,(#39594,#39595,#39596,#39597,#39598,
#39599,#39600,#39601,#39602,#39603,#39604,#39605,#39606,#39607,#39608,#39609),
 .UNSPECIFIED.,.F.,.F.,(4,1,1,1,1,1,1,1,1,1,1,1,1,4),(147.65485471872,148.139047371152,
148.636222475629,149.133397580106,149.630572684583,150.12774778906,150.624922893538,
151.122097998015,151.619273102492,152.116448206969,152.613623311447,153.110798415924,
153.607973520401,153.9380400259),.UNSPECIFIED.);
#699=B_SPLINE_CURVE_WITH_KNOTS('',3,(#39614,#39615,#39616,#39617,#39618,
#39619,#39620,#39621,#39622,#39623,#39624,#39625,#39626,#39627,#39628,#39629,
#39630),.UNSPECIFIED.,.F.,.F.,(4,1,1,1,1,1,1,1,1,1,1,1,1,1,4),(141.371669411541,
141.621691130861,142.118866235338,142.616041339815,143.113216444293,143.61039154877,
144.107566653247,144.604741757724,145.101916862201,145.599091966679,146.096267071156,
146.593442175633,147.09061728011,147.587792384587,147.65485471872),
 .UNSPECIFIED.);
#700=B_SPLINE_CURVE_WITH_KNOTS('',3,(#39631,#39632,#39633,#39634,#39635,
#39636,#39637,#39638,#39639,#39640,#39641,#39642,#39643,#39644,#39645,#39646,
#39647),.UNSPECIFIED.,.F.,.F.,(4,1,1,1,1,1,1,1,1,1,1,1,1,1,4),(141.371669411541,
141.675771012948,142.172946117425,142.670121221902,143.167296326379,143.664471430857,
144.161646535334,144.658821639811,145.155996744288,145.653171848766,146.150346953243,
146.64752205772,147.144697162197,147.641872266674,147.65485471872),
 .UNSPECIFIED.);
#701=B_SPLINE_CURVE_WITH_KNOTS('',3,(#39652,#39653,#39654,#39655,#39656,
#39657,#39658,#39659,#39660,#39661,#39662,#39663,#39664,#39665,#39666,#39667,
#39668),.UNSPECIFIED.,.F.,.F.,(4,1,1,1,1,1,1,1,1,1,1,1,1,1,4),(135.088484104361,
135.158414772657,135.655589877134,136.152764981612,136.649940086089,137.147115190566,
137.644290295043,138.14146539952,138.638640503998,139.135815608475,139.632990712952,
140.130165817429,140.627340921906,141.124516026384,141.371669411541),
 .UNSPECIFIED.);
#702=B_SPLINE_CURVE_WITH_KNOTS('',3,(#39669,#39670,#39671,#39672,#39673,
#39674,#39675,#39676,#39677,#39678,#39679,#39680,#39681,#39682,#39683,#39684,
#39685),.UNSPECIFIED.,.F.,.F.,(4,1,1,1,1,1,1,1,1,1,1,1,1,1,4),(135.088484104361,
135.212494654744,135.709669759221,136.206844863698,136.704019968176,137.201195072653,
137.69837017713,138.195545281607,138.692720386085,139.189895490562,139.687070595039,
140.184245699516,140.681420803993,141.178595908471,141.371669411541),
 .UNSPECIFIED.);
#703=B_SPLINE_CURVE_WITH_KNOTS('',3,(#39690,#39691,#39692,#39693,#39694,
#39695,#39696,#39697,#39698,#39699,#39700,#39701,#39702,#39703,#39704,#39705),
 .UNSPECIFIED.,.F.,.F.,(4,1,1,1,1,1,1,1,1,1,1,1,1,4),(128.805298797182,
129.192313518931,129.689488623408,130.186663727885,130.683838832362,131.181013936839,
131.678189041317,132.175364145794,132.672539250271,133.169714354748,133.666889459226,
134.164064563703,134.66123966818,135.088484104361),.UNSPECIFIED.);
#704=B_SPLINE_CURVE_WITH_KNOTS('',3,(#39706,#39707,#39708,#39709,#39710,
#39711,#39712,#39713,#39714,#39715,#39716,#39717,#39718,#39719,#39720,#39721),
 .UNSPECIFIED.,.F.,.F.,(4,1,1,1,1,1,1,1,1,1,1,1,1,4),(128.805298797182,
129.246393401017,129.743568505495,130.240743609972,130.737918714449,131.235093818926,
131.732268923404,132.229444027881,132.726619132358,133.223794236835,133.720969341312,
134.21814444579,134.715319550267,135.088484104361),.UNSPECIFIED.);
#705=B_SPLINE_CURVE_WITH_KNOTS('',3,(#39726,#39727,#39728,#39729,#39730,
#39731,#39732,#39733,#39734,#39735,#39736,#39737,#39738,#39739,#39740,#39741,
#39742),.UNSPECIFIED.,.F.,.F.,(4,1,1,1,1,1,1,1,1,1,1,1,1,1,4),(122.522113490002,
122.729037160727,123.226212265204,123.723387369681,124.220562474158,124.717737578636,
125.214912683113,125.71208778759,126.209262892067,126.706437996544,127.203613101022,
127.700788205499,128.197963309976,128.695138414453,128.805298797182),
 .UNSPECIFIED.);
#706=B_SPLINE_CURVE_WITH_KNOTS('',3,(#39743,#39744,#39745,#39746,#39747,
#39748,#39749,#39750,#39751,#39752,#39753,#39754,#39755,#39756,#39757,#39758,
#39759),.UNSPECIFIED.,.F.,.F.,(4,1,1,1,1,1,1,1,1,1,1,1,1,1,4),(122.522113490002,
122.783117042814,123.280292147291,123.777467251768,124.274642356245,124.771817460723,
125.2689925652,125.766167669677,126.263342774154,126.760517878631,127.257692983109,
127.754868087586,128.252043192063,128.74921829654,128.805298797182),
 .UNSPECIFIED.);
#707=B_SPLINE_CURVE_WITH_KNOTS('',3,(#39764,#39765,#39766,#39767,#39768,
#39769,#39770,#39771,#39772,#39773,#39774,#39775,#39776,#39777,#39778,#39779,
#39780),.UNSPECIFIED.,.F.,.F.,(4,1,1,1,1,1,1,1,1,1,1,1,1,1,4),(116.238928182822,
116.265760802523,116.762935907,117.260111011477,117.757286115955,118.254461220432,
118.751636324909,119.248811429386,119.745986533863,120.243161638341,120.740336742818,
121.237511847295,121.734686951772,122.23186205625,122.522113490002),
 .UNSPECIFIED.);
#708=B_SPLINE_CURVE_WITH_KNOTS('',3,(#39781,#39782,#39783,#39784,#39785,
#39786,#39787,#39788,#39789,#39790,#39791,#39792,#39793,#39794,#39795,#39796,
#39797),.UNSPECIFIED.,.F.,.F.,(4,1,1,1,1,1,1,1,1,1,1,1,1,1,4),(116.238928182822,
116.31984068461,116.817015789087,117.314190893564,117.811365998042,118.308541102519,
118.805716206996,119.302891311473,119.80006641595,120.297241520428,120.794416624905,
121.291591729382,121.788766833859,122.285941938336,122.522113490002),
 .UNSPECIFIED.);
#709=B_SPLINE_CURVE_WITH_KNOTS('',3,(#39802,#39803,#39804,#39805,#39806,
#39807,#39808,#39809,#39810,#39811,#39812,#39813,#39814,#39815,#39816,#39817),
 .UNSPECIFIED.,.F.,.F.,(4,1,1,1,1,1,1,1,1,1,1,1,1,4),(109.955742875643,
110.299659548796,110.796834653274,111.294009757751,111.791184862228,112.288359966705,
112.785535071182,113.28271017566,113.779885280137,114.277060384614,114.774235489091,
115.271410593569,115.768585698046,116.238928182822),.UNSPECIFIED.);
#710=B_SPLINE_CURVE_WITH_KNOTS('',3,(#39818,#39819,#39820,#39821,#39822,
#39823,#39824,#39825,#39826,#39827,#39828,#39829,#39830,#39831,#39832,#39833),
 .UNSPECIFIED.,.F.,.F.,(4,1,1,1,1,1,1,1,1,1,1,1,1,4),(109.955742875643,
110.353739430883,110.850914535361,111.348089639838,111.845264744315,112.342439848792,
112.839614953269,113.336790057747,113.833965162224,114.331140266701,114.828315371178,
115.325490475655,115.822665580133,116.238928182822),.UNSPECIFIED.);
#711=B_SPLINE_CURVE_WITH_KNOTS('',3,(#39838,#39839,#39840,#39841,#39842,
#39843,#39844,#39845,#39846,#39847,#39848,#39849,#39850,#39851,#39852,#39853,
#39854),.UNSPECIFIED.,.F.,.F.,(4,1,1,1,1,1,1,1,1,1,1,1,1,1,4),(103.672557568463,
103.836383190593,104.33355829507,104.830733399547,105.327908504024,105.825083608501,
106.322258712979,106.819433817456,107.316608921933,107.81378402641,108.310959130888,
108.808134235365,109.305309339842,109.802484444319,109.955742875643),
 .UNSPECIFIED.);
#712=B_SPLINE_CURVE_WITH_KNOTS('',3,(#39855,#39856,#39857,#39858,#39859,
#39860,#39861,#39862,#39863,#39864,#39865,#39866,#39867,#39868,#39869,#39870,
#39871),.UNSPECIFIED.,.F.,.F.,(4,1,1,1,1,1,1,1,1,1,1,1,1,1,4),(103.672557568463,
103.89046307268,104.387638177157,104.884813281634,105.381988386111,105.879163490588,
106.376338595066,106.873513699543,107.37068880402,107.867863908497,108.365039012974,
108.862214117452,109.359389221929,109.856564326406,109.955742875643),
 .UNSPECIFIED.);
#713=B_SPLINE_CURVE_WITH_KNOTS('',3,(#39876,#39877,#39878,#39879,#39880,
#39881,#39882,#39883,#39884,#39885,#39886,#39887,#39888,#39889,#39890,#39891),
 .UNSPECIFIED.,.F.,.F.,(4,1,1,1,1,1,1,1,1,1,1,1,1,4),(97.3893722612839,
97.870281936866,98.3674570413433,98.8646321458205,99.3618072502977,99.8589823547749,
100.356157459252,100.853332563729,101.350507668207,101.847682772684,102.344857877161,
102.842032981638,103.339208086115,103.672557568463),.UNSPECIFIED.);
#714=B_SPLINE_CURVE_WITH_KNOTS('',3,(#39892,#39893,#39894,#39895,#39896,
#39897,#39898,#39899,#39900,#39901,#39902,#39903,#39904,#39905,#39906,#39907,
#39908),.UNSPECIFIED.,.F.,.F.,(4,1,1,1,1,1,1,1,1,1,1,1,1,1,4),(97.3893722612839,
97.4271867144758,97.924361818953,98.4215369234302,98.9187120279074,99.4158871323846,
99.9130622368618,100.410237341339,100.907412445816,101.404587550293,101.901762654771,
102.398937759248,102.896112863725,103.393287968202,103.672557568463),
 .UNSPECIFIED.);
#715=B_SPLINE_CURVE_WITH_KNOTS('',3,(#39913,#39914,#39915,#39916,#39917,
#39918,#39919,#39920,#39921,#39922,#39923,#39924,#39925,#39926,#39927,#39928,
#39929),.UNSPECIFIED.,.F.,.F.,(4,1,1,1,1,1,1,1,1,1,1,1,1,1,4),(91.1061869541042,
91.4070055786623,91.9041806831395,92.4013557876167,92.8985308920939,93.3957059965711,
93.8928811010483,94.3900562055255,94.8872313100028,95.38440641448,95.8815815189572,
96.3787566234344,96.8759317279116,97.3731068323888,97.3893722612839),
 .UNSPECIFIED.);
#716=B_SPLINE_CURVE_WITH_KNOTS('',3,(#39930,#39931,#39932,#39933,#39934,
#39935,#39936,#39937,#39938,#39939,#39940,#39941,#39942,#39943,#39944,#39945),
 .UNSPECIFIED.,.F.,.F.,(4,1,1,1,1,1,1,1,1,1,1,1,1,4),(91.1061869541042,
91.4610854607492,91.9582605652264,92.4554356697036,92.9526107741808,93.449785878658,
93.9469609831353,94.4441360876125,94.9413111920897,95.4384862965669,95.9356614010441,
96.4328365055213,96.9300116099986,97.3893722612839),.UNSPECIFIED.);
#717=B_SPLINE_CURVE_WITH_KNOTS('',3,(#39950,#39951,#39952,#39953,#39954,
#39955,#39956,#39957,#39958,#39959,#39960,#39961,#39962,#39963,#39964,#39965,
#39966),.UNSPECIFIED.,.F.,.F.,(4,1,1,1,1,1,1,1,1,1,1,1,1,1,4),(84.8230016469245,
84.9437292204585,85.4409043249357,85.9380794294129,86.4352545338901,86.9324296383673,
87.4296047428445,87.9267798473217,88.423954951799,88.9211300562762,89.4183051607534,
89.9154802652306,90.4126553697078,90.909830474185,91.1061869541042),
 .UNSPECIFIED.);
#718=B_SPLINE_CURVE_WITH_KNOTS('',3,(#39967,#39968,#39969,#39970,#39971,
#39972,#39973,#39974,#39975,#39976,#39977,#39978,#39979,#39980,#39981,#39982,
#39983),.UNSPECIFIED.,.F.,.F.,(4,1,1,1,1,1,1,1,1,1,1,1,1,1,4),(84.8230016469245,
84.9978091025454,85.4949842070226,85.9921593114998,86.4893344159771,86.9865095204543,
87.4836846249315,87.9808597294087,88.4780348338859,88.9752099383631,89.4723850428403,
89.9695601473175,90.4667352517948,90.963910356272,91.1061869541042),
 .UNSPECIFIED.);
#719=B_SPLINE_CURVE_WITH_KNOTS('',3,(#39988,#39989,#39990,#39991,#39992,
#39993,#39994,#39995,#39996,#39997,#39998,#39999,#40000,#40001,#40002,#40003),
 .UNSPECIFIED.,.F.,.F.,(4,1,1,1,1,1,1,1,1,1,1,1,1,4),(78.5398163397448,
78.9776279667319,79.4748030712091,79.9719781756863,80.4691532801635,80.9663283846407,
81.463503489118,81.9606785935952,82.4578536980724,82.9550288025496,83.4522039070268,
83.949379011504,84.4465541159813,84.8230016469245),.UNSPECIFIED.);
#720=B_SPLINE_CURVE_WITH_KNOTS('',3,(#40004,#40005,#40006,#40007,#40008,
#40009,#40010,#40011,#40012,#40013,#40014,#40015,#40016,#40017,#40018,#40019),
 .UNSPECIFIED.,.F.,.F.,(4,1,1,1,1,1,1,1,1,1,1,1,1,4),(78.5398163397448,
79.0317078488188,79.528882953296,80.0260580577733,80.5232331622505,81.0204082667277,
81.5175833712049,82.0147584756821,82.5119335801593,83.0091086846365,83.5062837891138,
84.003458893591,84.5006339980682,84.8230016469245),.UNSPECIFIED.);
#721=B_SPLINE_CURVE_WITH_KNOTS('',3,(#40024,#40025,#40026,#40027,#40028,
#40029,#40030,#40031,#40032,#40033,#40034,#40035,#40036,#40037,#40038,#40039,
#40040),.UNSPECIFIED.,.F.,.F.,(4,1,1,1,1,1,1,1,1,1,1,1,1,1,4),(72.2566310325651,
72.5143516085281,73.0115267130053,73.5087018174825,74.0058769219598,74.503052026437,
75.0002271309142,75.4974022353914,75.9945773398686,76.4917524443458,76.988927548823,
77.4861026533003,77.9832777577775,78.4804528622547,78.5398163397448),
 .UNSPECIFIED.);
#722=B_SPLINE_CURVE_WITH_KNOTS('',3,(#40041,#40042,#40043,#40044,#40045,
#40046,#40047,#40048,#40049,#40050,#40051,#40052,#40053,#40054,#40055,#40056,
#40057),.UNSPECIFIED.,.F.,.F.,(4,1,1,1,1,1,1,1,1,1,1,1,1,1,4),(72.2566310325651,
72.568431490615,73.0656065950923,73.5627816995695,74.0599568040467,74.5571319085239,
75.0543070130011,75.5514821174783,76.0486572219556,76.5458323264328,77.04300743091,
77.5401825353872,78.0373576398644,78.5345327443416,78.5398163397448),
 .UNSPECIFIED.);
#723=B_SPLINE_CURVE_WITH_KNOTS('',3,(#40062,#40063,#40064,#40065,#40066,
#40067,#40068,#40069,#40070,#40071,#40072,#40073,#40074,#40075,#40076,#40077,
#40078),.UNSPECIFIED.,.F.,.F.,(4,1,1,1,1,1,1,1,1,1,1,1,1,1,4),(65.9734457253859,
66.0510752503243,66.5482503548015,67.0454254592788,67.542600563756,68.0397756682332,
68.5369507727104,69.0341258771876,69.5313009816648,70.028476086142,70.5256511906192,
71.0228262950965,71.5200013995737,72.0171765040509,72.2566310325651),
 .UNSPECIFIED.);
#724=B_SPLINE_CURVE_WITH_KNOTS('',3,(#40079,#40080,#40081,#40082,#40083,
#40084,#40085,#40086,#40087,#40088,#40089,#40090,#40091,#40092,#40093,#40094,
#40095),.UNSPECIFIED.,.F.,.F.,(4,1,1,1,1,1,1,1,1,1,1,1,1,1,4),(65.9734457253859,
66.1051551324113,66.6023302368885,67.0995053413657,67.5966804458429,68.0938555503201,
68.5910306547973,69.0882057592745,69.5853808637518,70.082555968229,70.5797310727062,
71.0769061771834,71.5740812816606,72.0712563861378,72.2566310325651),
 .UNSPECIFIED.);
#725=B_SPLINE_CURVE_WITH_KNOTS('',3,(#40100,#40101,#40102,#40103,#40104,
#40105,#40106,#40107,#40108,#40109,#40110,#40111,#40112,#40113,#40114,#40115),
 .UNSPECIFIED.,.F.,.F.,(4,1,1,1,1,1,1,1,1,1,1,1,1,4),(59.6902604182062,
60.0849739965977,60.582149101075,61.0793242055522,61.5764993100294,62.0736744145066,
62.5708495189838,63.068024623461,63.5651997279382,64.0623748324155,64.5595499368927,
65.0567250413699,65.5539001458471,65.9734457253859),.UNSPECIFIED.);
#726=B_SPLINE_CURVE_WITH_KNOTS('',3,(#40116,#40117,#40118,#40119,#40120,
#40121,#40122,#40123,#40124,#40125,#40126,#40127,#40128,#40129,#40130,#40131),
 .UNSPECIFIED.,.F.,.F.,(4,1,1,1,1,1,1,1,1,1,1,1,1,4),(59.6902604182062,
60.1390538786847,60.6362289831619,61.1334040876391,61.6305791921163,62.1277542965935,
62.6249294010708,63.122104505548,63.6192796100252,64.1164547145024,64.6136298189796,
65.1108049234568,65.607980027934,65.9734457253859),.UNSPECIFIED.);
#727=B_SPLINE_CURVE_WITH_KNOTS('',3,(#40136,#40137,#40138,#40139,#40140,
#40141,#40142,#40143,#40144,#40145,#40146,#40147,#40148,#40149,#40150,#40151,
#40152),.UNSPECIFIED.,.F.,.F.,(4,1,1,1,1,1,1,1,1,1,1,1,1,1,4),(53.4070751110266,
53.621697638394,54.1188727428712,54.6160478473484,55.1132229518256,55.6103980563028,
56.10757316078,56.6047482652572,57.1019233697345,57.5990984742117,58.0962735786889,
58.5934486831661,59.0906237876433,59.5877988921205,59.6902604182062),
 .UNSPECIFIED.);
#728=B_SPLINE_CURVE_WITH_KNOTS('',3,(#40153,#40154,#40155,#40156,#40157,
#40158,#40159,#40160,#40161,#40162,#40163,#40164,#40165,#40166,#40167,#40168,
#40169),.UNSPECIFIED.,.F.,.F.,(4,1,1,1,1,1,1,1,1,1,1,1,1,1,4),(53.4070751110266,
53.6757775204809,54.1729526249581,54.6701277294353,55.1673028339125,55.6644779383898,
56.161653042867,56.6588281473442,57.1560032518214,57.6531783562986,58.1503534607758,
58.647528565253,59.1447036697303,59.6418787742075,59.6902604182062),
 .UNSPECIFIED.);
#729=B_SPLINE_CURVE_WITH_KNOTS('',3,(#40174,#40175,#40176,#40177,#40178,
#40179,#40180,#40181,#40182,#40183,#40184,#40185,#40186,#40187,#40188,#40189,
#40190),.UNSPECIFIED.,.F.,.F.,(4,1,1,1,1,1,1,1,1,1,1,1,1,1,4),(47.1238898038469,
47.1584212801902,47.6555963846674,48.1527714891446,48.6499465936218,49.147121698099,
49.6442968025762,50.1414719070535,50.6386470115307,51.1358221160079,51.6329972204851,
52.1301723249623,52.6273474294395,53.1245225339167,53.4070751110266),
 .UNSPECIFIED.);
#730=B_SPLINE_CURVE_WITH_KNOTS('',3,(#40191,#40192,#40193,#40194,#40195,
#40196,#40197,#40198,#40199,#40200,#40201,#40202,#40203,#40204,#40205,#40206,
#40207),.UNSPECIFIED.,.F.,.F.,(4,1,1,1,1,1,1,1,1,1,1,1,1,1,4),(47.1238898038469,
47.2125011622771,47.7096762667543,48.2068513712315,48.7040264757088,49.201201580186,
49.6983766846632,50.1955517891404,50.6927268936176,51.1899019980948,51.687077102572,
52.1842522070493,52.6814273115265,53.1786024160037,53.4070751110266),
 .UNSPECIFIED.);
#731=B_SPLINE_CURVE_WITH_KNOTS('',3,(#40212,#40213,#40214,#40215,#40216,
#40217,#40218,#40219,#40220,#40221,#40222,#40223,#40224,#40225,#40226,#40227),
 .UNSPECIFIED.,.F.,.F.,(4,1,1,1,1,1,1,1,1,1,1,1,1,4),(40.8407044966672,
41.1923200264636,41.6894951309408,42.186670235418,42.6838453398952,43.1810204443725,
43.6781955488497,44.1753706533269,44.6725457578041,45.1697208622813,45.6668959667585,
46.1640710712357,46.661246175713,47.1238898038469),.UNSPECIFIED.);
#732=B_SPLINE_CURVE_WITH_KNOTS('',3,(#40228,#40229,#40230,#40231,#40232,
#40233,#40234,#40235,#40236,#40237,#40238,#40239,#40240,#40241,#40242,#40243),
 .UNSPECIFIED.,.F.,.F.,(4,1,1,1,1,1,1,1,1,1,1,1,1,4),(40.8407044966672,
41.2463999085505,41.7435750130278,42.240750117505,42.7379252219822,43.2351003264594,
43.7322754309366,44.2294505354138,44.726625639891,45.2238007443683,45.7209758488455,
46.2181509533227,46.7153260577999,47.1238898038469),.UNSPECIFIED.);
#733=B_SPLINE_CURVE_WITH_KNOTS('',3,(#40248,#40249,#40250,#40251,#40252,
#40253,#40254,#40255,#40256,#40257,#40258,#40259,#40260,#40261,#40262,#40263,
#40264),.UNSPECIFIED.,.F.,.F.,(4,1,1,1,1,1,1,1,1,1,1,1,1,1,4),(34.557519189488,
34.7290436682598,35.226218772737,35.7233938772142,36.2205689816915,36.7177440861687,
37.2149191906459,37.7120942951231,38.2092693996003,38.7064445040775,39.2036196085547,
39.700794713032,40.1979698175092,40.6951449219864,40.8407044966672),
 .UNSPECIFIED.);
#734=B_SPLINE_CURVE_WITH_KNOTS('',3,(#40265,#40266,#40267,#40268,#40269,
#40270,#40271,#40272,#40273,#40274,#40275,#40276,#40277,#40278,#40279,#40280,
#40281),.UNSPECIFIED.,.F.,.F.,(4,1,1,1,1,1,1,1,1,1,1,1,1,1,4),(34.557519189488,
34.7831235503468,35.280298654824,35.7774737593012,36.2746488637784,36.7718239682556,
37.2689990727328,37.76617417721,38.2633492816873,38.7605243861645,39.2576994906417,
39.7548745951189,40.2520496995961,40.7492248040733,40.8407044966672),
 .UNSPECIFIED.);
#735=B_SPLINE_CURVE_WITH_KNOTS('',3,(#40286,#40287,#40288,#40289,#40290,
#40291,#40292,#40293,#40294,#40295,#40296,#40297,#40298,#40299,#40300,#40301),
 .UNSPECIFIED.,.F.,.F.,(4,1,1,1,1,1,1,1,1,1,1,1,1,4),(28.2743338823083,
28.7629424145332,29.2601175190104,29.7572926234877,30.2544677279649,30.7516428324421,
31.2488179369193,31.7459930413965,32.2431681458737,32.7403432503509,33.2375183548282,
33.7346934593054,34.2318685637826,34.557519189488),.UNSPECIFIED.);
#736=B_SPLINE_CURVE_WITH_KNOTS('',3,(#40302,#40303,#40304,#40305,#40306,
#40307,#40308,#40309,#40310,#40311,#40312,#40313,#40314,#40315,#40316,#40317,
#40318),.UNSPECIFIED.,.F.,.F.,(4,1,1,1,1,1,1,1,1,1,1,1,1,1,4),(28.2743338823083,
28.319847192143,28.8170222966202,29.3141974010974,29.8113725055746,30.3085476100518,
30.805722714529,31.3028978190063,31.8000729234835,32.2972480279607,32.7944231324379,
33.2915982369151,33.7887733413923,34.2859484458695,34.557519189488),
 .UNSPECIFIED.);
#737=B_SPLINE_CURVE_WITH_KNOTS('',3,(#40323,#40324,#40325,#40326,#40327,
#40328,#40329,#40330,#40331,#40332,#40333,#40334,#40335,#40336,#40337,#40338,
#40339),.UNSPECIFIED.,.F.,.F.,(4,1,1,1,1,1,1,1,1,1,1,1,1,1,4),(21.9911485751286,
22.2996660563294,22.7968411608067,23.2940162652839,23.7911913697611,24.2883664742383,
24.7855415787155,25.2827166831927,25.7798917876699,26.2770668921472,26.7742419966244,
27.2714171011016,27.7685922055788,28.265767310056,28.2743338823083),
 .UNSPECIFIED.);
#738=B_SPLINE_CURVE_WITH_KNOTS('',3,(#40340,#40341,#40342,#40343,#40344,
#40345,#40346,#40347,#40348,#40349,#40350,#40351,#40352,#40353,#40354,#40355),
 .UNSPECIFIED.,.F.,.F.,(4,1,1,1,1,1,1,1,1,1,1,1,1,4),(21.9911485751286,
22.3537459384164,22.8509210428936,23.3480961473708,23.845271251848,24.3424463563253,
24.8396214608025,25.3367965652797,25.8339716697569,26.3311467742341,26.8283218787113,
27.3254969831885,27.8226720876658,28.2743338823083),.UNSPECIFIED.);
#739=B_SPLINE_CURVE_WITH_KNOTS('',3,(#40361,#40362,#40363,#40364,#40365,
#40366),.UNSPECIFIED.,.F.,.F.,(4,1,1,4),(14.398944266781,14.8961193712582,
15.3932944757354,15.707963267949),.UNSPECIFIED.);
#740=B_SPLINE_CURVE_WITH_KNOTS('',3,(#40369,#40370,#40371,#40372,#40373,
#40374,#40375),.UNSPECIFIED.,.F.,.F.,(4,1,1,1,4),(13.8753896155273,14.344864384694,
14.8420394891712,15.3392145936484,15.707963267949),.UNSPECIFIED.);
#741=B_SPLINE_CURVE_WITH_KNOTS('',3,(#40381,#40382,#40383,#40384,#40385,
#40386,#40387),.UNSPECIFIED.,.F.,.F.,(4,3,4),(252.636431288351,252.845104747016,
253.343813040403),.UNSPECIFIED.);
#742=B_SPLINE_CURVE_WITH_KNOTS('',3,(#40395,#40396,#40397,#40398,#40399,
#40400,#40401,#40402,#40403,#40404,#40405,#40406,#40407,#40408,#40409,#40410),
 .UNSPECIFIED.,.F.,.F.,(4,3,3,3,3,4),(-251.327412287183,-250.85027157347,
-250.351563280083,-249.852854986696,-249.35414669331,-248.893201385645),
 .UNSPECIFIED.);
#743=B_SPLINE_CURVE_WITH_KNOTS('',3,(#40415,#40416,#40417,#40418,#40419,
#40420,#40421,#40422,#40423,#40424,#40425,#40426,#40427,#40428,#40429,#40430,
#40431,#40432,#40433,#40434,#40435,#40436,#40437,#40438,#40439,#40440,#40441,
#40442,#40443,#40444,#40445,#40446,#40447,#40448,#40449,#40450,#40451,#40452,
#40453,#40454,#40455,#40456,#40457),.UNSPECIFIED.,.F.,.F.,(4,3,3,3,3,3,
3,3,3,3,3,3,3,3,4),(246.353245981172,246.36189693299,246.860605226377,247.359313519763,
247.85802181315,248.356730106537,248.855438399923,249.35414669331,249.852854986696,
250.351563280083,250.85027157347,251.348979866856,251.847688160243,252.346396453629,
252.636431288351),.UNSPECIFIED.);
#744=B_SPLINE_CURVE_WITH_KNOTS('',3,(#40458,#40459,#40460,#40461,#40462,
#40463,#40464,#40465,#40466,#40467,#40468,#40469,#40470,#40471,#40472,#40473,
#40474,#40475,#40476,#40477,#40478,#40479,#40480,#40481,#40482,#40483,#40484,
#40485,#40486,#40487,#40488,#40489,#40490,#40491,#40492,#40493,#40494,#40495,
#40496,#40497,#40498,#40499,#40500),.UNSPECIFIED.,.F.,.F.,(4,3,3,3,3,3,
3,3,3,3,3,3,3,3,4),(-248.893201385645,-248.855438399923,-248.356730106536,
-247.85802181315,-247.359313519763,-246.860605226377,-246.36189693299,-245.863188639603,
-245.364480346217,-244.86577205283,-244.367063759444,-243.868355466057,
-243.36964717267,-242.870938879284,-242.610016078465),.UNSPECIFIED.);
#745=B_SPLINE_CURVE_WITH_KNOTS('',3,(#40505,#40506,#40507,#40508,#40509,
#40510,#40511,#40512,#40513,#40514,#40515,#40516,#40517,#40518,#40519,#40520,
#40521,#40522,#40523,#40524,#40525,#40526,#40527,#40528,#40529,#40530,#40531,
#40532,#40533,#40534,#40535,#40536,#40537,#40538,#40539,#40540,#40541,#40542,
#40543,#40544),.UNSPECIFIED.,.F.,.F.,(4,3,3,3,3,3,3,3,3,3,3,3,3,4),(240.070060673992,
240.377397412351,240.876105705737,241.374813999124,241.873522292511,242.372230585897,
242.870938879284,243.36964717267,243.868355466057,244.367063759444,244.86577205283,
245.364480346217,245.863188639603,246.353245981172),.UNSPECIFIED.);
#746=B_SPLINE_CURVE_WITH_KNOTS('',3,(#40545,#40546,#40547,#40548,#40549,
#40550,#40551,#40552,#40553,#40554,#40555,#40556,#40557,#40558,#40559,#40560,
#40561,#40562,#40563,#40564,#40565,#40566,#40567,#40568,#40569,#40570,#40571,
#40572,#40573,#40574,#40575,#40576,#40577,#40578,#40579,#40580,#40581,#40582,
#40583,#40584,#40585,#40586,#40587),.UNSPECIFIED.,.F.,.F.,(4,3,3,3,3,3,
3,3,3,3,3,3,3,3,4),(-242.610016078465,-242.372230585897,-241.87352229251,
-241.374813999124,-240.876105705737,-240.377397412351,-239.878689118964,
-239.379980825577,-238.881272532191,-238.382564238804,-237.883855945417,
-237.385147652031,-236.886439358644,-236.387731065258,-236.326830771286),
 .UNSPECIFIED.);
#747=B_SPLINE_CURVE_WITH_KNOTS('',3,(#40592,#40593,#40594,#40595,#40596,
#40597,#40598,#40599,#40600,#40601,#40602,#40603,#40604,#40605,#40606,#40607,
#40608,#40609,#40610,#40611,#40612,#40613,#40614,#40615,#40616,#40617,#40618,
#40619,#40620,#40621,#40622,#40623,#40624,#40625,#40626,#40627,#40628,#40629,
#40630,#40631,#40632,#40633,#40634),.UNSPECIFIED.,.F.,.F.,(4,3,3,3,3,3,
3,3,3,3,3,3,3,3,4),(233.786875366813,233.894189598325,234.392897891711,
234.891606185098,235.390314478484,235.889022771871,236.387731065258,236.886439358644,
237.385147652031,237.883855945418,238.382564238804,238.881272532191,239.379980825577,
239.878689118964,240.070060673992),.UNSPECIFIED.);
#748=B_SPLINE_CURVE_WITH_KNOTS('',3,(#40635,#40636,#40637,#40638,#40639,
#40640,#40641,#40642,#40643,#40644,#40645,#40646,#40647,#40648,#40649,#40650,
#40651,#40652,#40653,#40654,#40655,#40656,#40657,#40658,#40659,#40660,#40661,
#40662,#40663,#40664,#40665,#40666,#40667,#40668,#40669,#40670,#40671,#40672,
#40673,#40674),.UNSPECIFIED.,.F.,.F.,(4,3,3,3,3,3,3,3,3,3,3,3,3,4),(-236.326830771286,
-235.889022771871,-235.390314478484,-234.891606185098,-234.392897891711,
-233.894189598325,-233.395481304938,-232.896773011551,-232.398064718165,
-231.899356424778,-231.400648131391,-230.901939838005,-230.403231544618,
-230.043645464106),.UNSPECIFIED.);
#749=B_SPLINE_CURVE_WITH_KNOTS('',3,(#40679,#40680,#40681,#40682,#40683,
#40684,#40685,#40686,#40687,#40688,#40689,#40690,#40691,#40692,#40693,#40694,
#40695,#40696,#40697,#40698,#40699,#40700,#40701,#40702,#40703,#40704,#40705,
#40706,#40707,#40708,#40709,#40710,#40711,#40712,#40713,#40714,#40715,#40716,
#40717,#40718),.UNSPECIFIED.,.F.,.F.,(4,3,3,3,3,3,3,3,3,3,3,3,3,4),(227.503690059633,
227.909690077685,228.408398371072,228.907106664458,229.405814957845,229.904523251232,
230.403231544618,230.901939838005,231.400648131391,231.899356424778,232.398064718165,
232.896773011551,233.395481304938,233.786875366813),.UNSPECIFIED.);
#750=B_SPLINE_CURVE_WITH_KNOTS('',3,(#40719,#40720,#40721,#40722,#40723,
#40724,#40725,#40726,#40727,#40728,#40729,#40730,#40731,#40732,#40733,#40734,
#40735,#40736,#40737,#40738,#40739,#40740,#40741,#40742,#40743,#40744,#40745,
#40746,#40747,#40748,#40749,#40750,#40751,#40752,#40753,#40754,#40755,#40756,
#40757,#40758,#40759,#40760,#40761),.UNSPECIFIED.,.F.,.F.,(4,3,3,3,3,3,
3,3,3,3,3,3,3,3,4),(-230.043645464106,-229.904523251232,-229.405814957845,
-228.907106664458,-228.408398371072,-227.909690077685,-227.410981784298,
-226.912273490912,-226.413565197525,-225.914856904139,-225.416148610752,
-224.917440317365,-224.418732023979,-223.920023730592,-223.760460156926),
 .UNSPECIFIED.);
#751=B_SPLINE_CURVE_WITH_KNOTS('',3,(#40766,#40767,#40768,#40769,#40770,
#40771,#40772,#40773,#40774,#40775,#40776,#40777,#40778,#40779,#40780,#40781,
#40782,#40783,#40784,#40785,#40786,#40787,#40788,#40789,#40790,#40791,#40792,
#40793,#40794,#40795,#40796,#40797,#40798,#40799,#40800,#40801,#40802,#40803,
#40804,#40805,#40806,#40807,#40808),.UNSPECIFIED.,.F.,.F.,(4,3,3,3,3,3,
3,3,3,3,3,3,3,3,4),(221.220504752453,221.426482263659,221.925190557046,
222.423898850432,222.922607143819,223.421315437206,223.920023730592,224.418732023979,
224.917440317365,225.416148610752,225.914856904139,226.413565197525,226.912273490912,
227.410981784299,227.503690059633),.UNSPECIFIED.);
#752=B_SPLINE_CURVE_WITH_KNOTS('',3,(#40809,#40810,#40811,#40812,#40813,
#40814,#40815,#40816,#40817,#40818,#40819,#40820,#40821,#40822,#40823,#40824,
#40825,#40826,#40827,#40828,#40829,#40830,#40831,#40832,#40833,#40834,#40835,
#40836,#40837,#40838,#40839,#40840,#40841,#40842,#40843,#40844,#40845,#40846,
#40847,#40848),.UNSPECIFIED.,.F.,.F.,(4,3,3,3,3,3,3,3,3,3,3,3,3,4),(-223.760460156926,
-223.421315437206,-222.922607143819,-222.423898850432,-221.925190557046,
-221.426482263659,-220.927773970272,-220.429065676886,-219.930357383499,
-219.431649090113,-218.932940796726,-218.434232503339,-217.935524209953,
-217.477274849747),.UNSPECIFIED.);
#753=B_SPLINE_CURVE_WITH_KNOTS('',3,(#40853,#40854,#40855,#40856,#40857,
#40858,#40859,#40860,#40861,#40862,#40863,#40864,#40865,#40866,#40867,#40868,
#40869,#40870,#40871,#40872,#40873,#40874,#40875,#40876,#40877,#40878,#40879,
#40880,#40881,#40882,#40883,#40884,#40885,#40886,#40887,#40888,#40889,#40890,
#40891,#40892,#40893,#40894,#40895),.UNSPECIFIED.,.F.,.F.,(4,3,3,3,3,3,
3,3,3,3,3,3,3,3,4),(214.937319445274,214.943274449633,215.44198274302,215.940691036406,
216.439399329793,216.93810762318,217.436815916566,217.935524209953,218.434232503339,
218.932940796726,219.431649090113,219.930357383499,220.429065676886,220.927773970272,
221.220504752453),.UNSPECIFIED.);
#754=B_SPLINE_CURVE_WITH_KNOTS('',3,(#40896,#40897,#40898,#40899,#40900,
#40901,#40902,#40903,#40904,#40905,#40906,#40907,#40908,#40909,#40910,#40911,
#40912,#40913,#40914,#40915,#40916,#40917,#40918,#40919,#40920,#40921,#40922,
#40923,#40924,#40925,#40926,#40927,#40928,#40929,#40930,#40931,#40932,#40933,
#40934,#40935,#40936,#40937,#40938),.UNSPECIFIED.,.F.,.F.,(4,3,3,3,3,3,
3,3,3,3,3,3,3,3,4),(-217.477274849747,-217.436815916566,-216.938107623179,
-216.439399329793,-215.940691036406,-215.44198274302,-214.943274449633,
-214.444566156246,-213.94585786286,-213.447149569473,-212.948441276087,
-212.4497329827,-211.951024689313,-211.452316395927,-211.194089542567),
 .UNSPECIFIED.);
#755=B_SPLINE_CURVE_WITH_KNOTS('',3,(#40943,#40944,#40945,#40946,#40947,
#40948,#40949,#40950,#40951,#40952,#40953,#40954,#40955,#40956,#40957,#40958,
#40959,#40960,#40961,#40962,#40963,#40964,#40965,#40966,#40967,#40968,#40969,
#40970,#40971,#40972,#40973,#40974,#40975,#40976,#40977,#40978,#40979,#40980,
#40981,#40982),.UNSPECIFIED.,.F.,.F.,(4,3,3,3,3,3,3,3,3,3,3,3,3,4),(208.654134138094,
208.958774928994,209.45748322238,209.956191515767,210.454899809153,210.95360810254,
211.452316395927,211.951024689313,212.4497329827,212.948441276087,213.447149569473,
213.94585786286,214.444566156246,214.937319445274),.UNSPECIFIED.);
#756=B_SPLINE_CURVE_WITH_KNOTS('',3,(#40983,#40984,#40985,#40986,#40987,
#40988,#40989,#40990,#40991,#40992,#40993,#40994,#40995,#40996,#40997,#40998,
#40999,#41000,#41001,#41002,#41003,#41004,#41005,#41006,#41007,#41008,#41009,
#41010,#41011,#41012,#41013,#41014,#41015,#41016,#41017,#41018,#41019,#41020,
#41021,#41022,#41023,#41024,#41025),.UNSPECIFIED.,.F.,.F.,(4,3,3,3,3,3,
3,3,3,3,3,3,3,3,4),(-211.194089542567,-210.95360810254,-210.454899809153,
-209.956191515767,-209.45748322238,-208.958774928994,-208.460066635607,
-207.96135834222,-207.462650048834,-206.963941755447,-206.46523346206,-205.966525168674,
-205.467816875287,-204.969108581901,-204.910904235388),.UNSPECIFIED.);
#757=B_SPLINE_CURVE_WITH_KNOTS('',3,(#41030,#41031,#41032,#41033,#41034,
#41035,#41036,#41037,#41038,#41039,#41040,#41041,#41042,#41043,#41044,#41045,
#41046,#41047,#41048,#41049,#41050,#41051,#41052,#41053,#41054,#41055,#41056,
#41057,#41058,#41059,#41060,#41061,#41062,#41063,#41064,#41065,#41066,#41067,
#41068,#41069,#41070,#41071,#41072),.UNSPECIFIED.,.F.,.F.,(4,3,3,3,3,3,
3,3,3,3,3,3,3,3,4),(202.370948830915,202.475567114968,202.974275408354,
203.472983701741,203.971691995127,204.470400288514,204.969108581901,205.467816875287,
205.966525168674,206.46523346206,206.963941755447,207.462650048834,207.96135834222,
208.460066635607,208.654134138094),.UNSPECIFIED.);
#758=B_SPLINE_CURVE_WITH_KNOTS('',3,(#41073,#41074,#41075,#41076,#41077,
#41078,#41079,#41080,#41081,#41082,#41083,#41084,#41085,#41086,#41087,#41088,
#41089,#41090,#41091,#41092,#41093,#41094,#41095,#41096,#41097,#41098,#41099,
#41100,#41101,#41102,#41103,#41104,#41105,#41106,#41107,#41108,#41109,#41110,
#41111,#41112),.UNSPECIFIED.,.F.,.F.,(4,3,3,3,3,3,3,3,3,3,3,3,3,4),(-204.910904235388,
-204.470400288514,-203.971691995127,-203.472983701741,-202.974275408354,
-202.475567114968,-201.976858821581,-201.478150528194,-200.979442234808,
-200.480733941421,-199.982025648034,-199.483317354648,-198.984609061261,
-198.627718928208),.UNSPECIFIED.);
#759=B_SPLINE_CURVE_WITH_KNOTS('',3,(#41117,#41118,#41119,#41120,#41121,
#41122,#41123,#41124,#41125,#41126,#41127,#41128,#41129,#41130,#41131,#41132,
#41133,#41134,#41135,#41136,#41137,#41138,#41139,#41140,#41141,#41142,#41143,
#41144,#41145,#41146,#41147,#41148,#41149,#41150,#41151,#41152,#41153,#41154,
#41155,#41156),.UNSPECIFIED.,.F.,.F.,(4,3,3,3,3,3,3,3,3,3,3,3,3,4),(196.087763523735,
196.491067594328,196.989775887715,197.488484181101,197.987192474488,198.485900767875,
198.984609061261,199.483317354648,199.982025648034,200.480733941421,200.979442234808,
201.478150528194,201.976858821581,202.370948830915),.UNSPECIFIED.);
#760=B_SPLINE_CURVE_WITH_KNOTS('',3,(#41157,#41158,#41159,#41160,#41161,
#41162,#41163,#41164,#41165,#41166,#41167,#41168,#41169,#41170,#41171,#41172,
#41173,#41174,#41175,#41176,#41177,#41178,#41179,#41180,#41181,#41182,#41183,
#41184,#41185,#41186,#41187,#41188,#41189,#41190,#41191,#41192,#41193,#41194,
#41195,#41196,#41197,#41198,#41199),.UNSPECIFIED.,.F.,.F.,(4,3,3,3,3,3,
3,3,3,3,3,3,3,3,4),(-198.627718928208,-198.485900767875,-197.987192474488,
-197.488484181101,-196.989775887715,-196.491067594328,-195.992359300941,
-195.493651007555,-194.994942714168,-194.496234420782,-193.997526127395,
-193.498817834008,-193.000109540622,-192.501401247235,-192.344533621029),
 .UNSPECIFIED.);
#761=B_SPLINE_CURVE_WITH_KNOTS('',3,(#41204,#41205,#41206,#41207,#41208,
#41209,#41210,#41211,#41212,#41213,#41214,#41215,#41216,#41217,#41218,#41219,
#41220,#41221,#41222,#41223,#41224,#41225,#41226,#41227,#41228,#41229,#41230,
#41231,#41232,#41233,#41234,#41235,#41236,#41237,#41238,#41239,#41240,#41241,
#41242,#41243,#41244,#41245,#41246),.UNSPECIFIED.,.F.,.F.,(4,3,3,3,3,3,
3,3,3,3,3,3,3,3,4),(189.804578216556,190.007859780302,190.506568073689,
191.005276367075,191.503984660462,192.002692953849,192.501401247235,193.000109540622,
193.498817834008,193.997526127395,194.496234420782,194.994942714168,195.493651007555,
195.992359300941,196.087763523735),.UNSPECIFIED.);
#762=B_SPLINE_CURVE_WITH_KNOTS('',3,(#41247,#41248,#41249,#41250,#41251,
#41252,#41253,#41254,#41255,#41256,#41257,#41258,#41259,#41260,#41261,#41262,
#41263,#41264,#41265,#41266,#41267,#41268,#41269,#41270,#41271,#41272,#41273,
#41274,#41275,#41276,#41277,#41278,#41279,#41280,#41281,#41282,#41283,#41284,
#41285,#41286),.UNSPECIFIED.,.F.,.F.,(4,3,3,3,3,3,3,3,3,3,3,3,3,4),(-192.344533621029,
-192.002692953848,-191.503984660462,-191.005276367075,-190.506568073689,
-190.007859780302,-189.509151486915,-189.010443193529,-188.511734900142,
-188.013026606756,-187.514318313369,-187.015610019982,-186.516901726596,
-186.061348313849),.UNSPECIFIED.);
#763=B_SPLINE_CURVE_WITH_KNOTS('',3,(#41291,#41292,#41293,#41294,#41295,
#41296,#41297,#41298,#41299,#41300,#41301,#41302,#41303,#41304,#41305,#41306,
#41307,#41308,#41309,#41310,#41311,#41312,#41313,#41314,#41315,#41316,#41317,
#41318,#41319,#41320,#41321,#41322,#41323,#41324,#41325,#41326,#41327,#41328,
#41329,#41330,#41331,#41332,#41333),.UNSPECIFIED.,.F.,.F.,(4,3,3,3,3,3,
3,3,3,3,3,3,3,3,4),(183.521392909376,183.524651966276,184.023360259663,
184.522068553049,185.020776846436,185.519485139823,186.018193433209,186.516901726596,
187.015610019982,187.514318313369,188.013026606756,188.511734900142,189.010443193529,
189.509151486915,189.804578216556),.UNSPECIFIED.);
#764=B_SPLINE_CURVE_WITH_KNOTS('',3,(#41334,#41335,#41336,#41337,#41338,
#41339,#41340,#41341,#41342,#41343,#41344,#41345,#41346,#41347,#41348,#41349,
#41350,#41351,#41352,#41353,#41354,#41355,#41356,#41357,#41358,#41359,#41360,
#41361,#41362,#41363,#41364,#41365,#41366,#41367,#41368,#41369,#41370,#41371,
#41372,#41373,#41374,#41375,#41376),.UNSPECIFIED.,.F.,.F.,(4,3,3,3,3,3,
3,3,3,3,3,3,3,3,4),(-186.061348313849,-186.018193433209,-185.519485139822,
-185.020776846436,-184.522068553049,-184.023360259663,-183.524651966276,
-183.025943672889,-182.527235379503,-182.028527086116,-181.529818792729,
-181.031110499343,-180.532402205956,-180.03369391257,-179.77816300667),
 .UNSPECIFIED.);
#765=B_SPLINE_CURVE_WITH_KNOTS('',3,(#41381,#41382,#41383,#41384,#41385,
#41386,#41387,#41388,#41389,#41390,#41391,#41392,#41393,#41394,#41395,#41396,
#41397,#41398,#41399,#41400,#41401,#41402,#41403,#41404,#41405,#41406,#41407,
#41408,#41409,#41410,#41411,#41412,#41413,#41414,#41415,#41416,#41417,#41418,
#41419,#41420),.UNSPECIFIED.,.F.,.F.,(4,3,3,3,3,3,3,3,3,3,3,3,3,4),(177.238207602196,
177.540152445637,178.038860739023,178.53756903241,179.036277325796,179.534985619183,
180.03369391257,180.532402205956,181.031110499343,181.52981879273,182.028527086116,
182.527235379503,183.025943672889,183.521392909376),.UNSPECIFIED.);
#766=B_SPLINE_CURVE_WITH_KNOTS('',3,(#41421,#41422,#41423,#41424,#41425,
#41426,#41427,#41428,#41429,#41430,#41431,#41432,#41433,#41434,#41435,#41436,
#41437,#41438,#41439,#41440,#41441,#41442,#41443,#41444,#41445,#41446,#41447,
#41448,#41449,#41450,#41451,#41452,#41453,#41454,#41455,#41456,#41457,#41458,
#41459,#41460,#41461,#41462,#41463),.UNSPECIFIED.,.F.,.F.,(4,3,3,3,3,3,
3,3,3,3,3,3,3,3,4),(-179.77816300667,-179.534985619183,-179.036277325796,
-178.53756903241,-178.038860739023,-177.540152445637,-177.04144415225,-176.542735858863,
-176.044027565477,-175.54531927209,-175.046610978703,-174.547902685317,
-174.04919439193,-173.550486098544,-173.49497769949),.UNSPECIFIED.);
#767=B_SPLINE_CURVE_WITH_KNOTS('',3,(#41468,#41469,#41470,#41471,#41472,
#41473,#41474,#41475,#41476,#41477,#41478,#41479,#41480,#41481,#41482,#41483,
#41484,#41485,#41486,#41487,#41488,#41489,#41490,#41491,#41492,#41493,#41494,
#41495,#41496,#41497,#41498,#41499,#41500,#41501,#41502,#41503,#41504,#41505,
#41506,#41507,#41508,#41509,#41510),.UNSPECIFIED.,.F.,.F.,(4,3,3,3,3,3,
3,3,3,3,3,3,3,3,4),(170.955022295017,171.056944631611,171.555652924997,
172.054361218384,172.55306951177,173.051777805157,173.550486098544,174.04919439193,
174.547902685317,175.046610978703,175.54531927209,176.044027565477,176.542735858863,
177.04144415225,177.238207602196),.UNSPECIFIED.);
#768=B_SPLINE_CURVE_WITH_KNOTS('',3,(#41511,#41512,#41513,#41514,#41515,
#41516,#41517,#41518,#41519,#41520,#41521,#41522,#41523,#41524,#41525,#41526,
#41527,#41528,#41529,#41530,#41531,#41532,#41533,#41534,#41535,#41536,#41537,
#41538,#41539,#41540,#41541,#41542,#41543,#41544,#41545,#41546,#41547,#41548,
#41549,#41550),.UNSPECIFIED.,.F.,.F.,(4,3,3,3,3,3,3,3,3,3,3,3,3,4),(-173.49497769949,
-173.051777805157,-172.55306951177,-172.054361218384,-171.555652924997,
-171.05694463161,-170.558236338224,-170.059528044837,-169.560819751451,
-169.062111458064,-168.563403164677,-168.064694871291,-167.565986577904,
-167.21179239231),.UNSPECIFIED.);
#769=B_SPLINE_CURVE_WITH_KNOTS('',3,(#41555,#41556,#41557,#41558,#41559,
#41560,#41561,#41562,#41563,#41564,#41565,#41566,#41567,#41568,#41569,#41570,
#41571,#41572,#41573,#41574,#41575,#41576,#41577,#41578,#41579,#41580,#41581,
#41582,#41583,#41584,#41585,#41586,#41587,#41588,#41589,#41590,#41591,#41592,
#41593,#41594),.UNSPECIFIED.,.F.,.F.,(4,3,3,3,3,3,3,3,3,3,3,3,3,4),(164.671836987837,
165.072445110971,165.571153404358,166.069861697744,166.568569991131,167.067278284518,
167.565986577904,168.064694871291,168.563403164677,169.062111458064,169.560819751451,
170.059528044837,170.558236338224,170.955022295017),.UNSPECIFIED.);
#770=B_SPLINE_CURVE_WITH_KNOTS('',3,(#41595,#41596,#41597,#41598,#41599,
#41600,#41601,#41602,#41603,#41604,#41605,#41606,#41607,#41608,#41609,#41610,
#41611,#41612,#41613,#41614,#41615,#41616,#41617,#41618,#41619,#41620,#41621,
#41622,#41623,#41624,#41625,#41626,#41627,#41628,#41629,#41630,#41631,#41632,
#41633,#41634,#41635,#41636,#41637),.UNSPECIFIED.,.F.,.F.,(4,3,3,3,3,3,
3,3,3,3,3,3,3,3,4),(-167.21179239231,-167.067278284517,-166.568569991131,
-166.069861697744,-165.571153404358,-165.072445110971,-164.573736817584,
-164.075028524198,-163.576320230811,-163.077611937425,-162.578903644038,
-162.080195350651,-161.581487057265,-161.082778763878,-160.928607085131),
 .UNSPECIFIED.);
#771=B_SPLINE_CURVE_WITH_KNOTS('',3,(#41642,#41643,#41644,#41645,#41646,
#41647,#41648,#41649,#41650,#41651,#41652,#41653,#41654,#41655,#41656,#41657,
#41658,#41659,#41660,#41661,#41662,#41663,#41664,#41665,#41666,#41667,#41668,
#41669,#41670,#41671,#41672,#41673,#41674,#41675,#41676,#41677,#41678,#41679,
#41680,#41681,#41682,#41683,#41684),.UNSPECIFIED.,.F.,.F.,(4,3,3,3,3,3,
3,3,3,3,3,3,3,3,4),(158.388651680658,158.589237296945,159.087945590332,
159.586653883718,160.085362177105,160.584070470491,161.082778763878,161.581487057265,
162.080195350651,162.578903644038,163.077611937425,163.576320230811,164.075028524198,
164.573736817584,164.671836987837),.UNSPECIFIED.);
#772=B_SPLINE_CURVE_WITH_KNOTS('',3,(#41685,#41686,#41687,#41688,#41689,
#41690,#41691,#41692,#41693,#41694,#41695,#41696,#41697,#41698,#41699,#41700,
#41701,#41702,#41703,#41704,#41705,#41706,#41707,#41708,#41709,#41710,#41711,
#41712,#41713,#41714,#41715,#41716,#41717,#41718,#41719,#41720,#41721,#41722,
#41723,#41724),.UNSPECIFIED.,.F.,.F.,(4,3,3,3,3,3,3,3,3,3,3,3,3,4),(-160.928607085131,
-160.584070470491,-160.085362177105,-159.586653883718,-159.087945590332,
-158.589237296945,-158.090529003558,-157.591820710172,-157.093112416785,
-156.594404123399,-156.095695830012,-155.596987536625,-155.098279243239,
-154.645421777951),.UNSPECIFIED.);
#773=B_SPLINE_CURVE_WITH_KNOTS('',3,(#41729,#41730,#41731,#41732,#41733,
#41734,#41735,#41736,#41737,#41738,#41739,#41740,#41741,#41742,#41743,#41744,
#41745,#41746,#41747,#41748,#41749,#41750,#41751,#41752,#41753,#41754,#41755,
#41756,#41757,#41758,#41759,#41760,#41761,#41762,#41763,#41764,#41765,#41766,
#41767,#41768),.UNSPECIFIED.,.F.,.F.,(4,3,3,3,3,3,3,3,3,3,3,3,3,4),(152.105466373478,
152.604737776306,153.103446069692,153.602154363079,154.100862656465,154.599570949852,
155.098279243239,155.596987536625,156.095695830012,156.594404123399,157.093112416785,
157.591820710172,158.090529003558,158.388651680658),.UNSPECIFIED.);
#774=B_SPLINE_CURVE_WITH_KNOTS('',3,(#41769,#41770,#41771,#41772,#41773,
#41774,#41775,#41776,#41777,#41778,#41779,#41780,#41781,#41782,#41783,#41784,
#41785,#41786,#41787,#41788,#41789,#41790,#41791,#41792,#41793,#41794,#41795,
#41796,#41797,#41798,#41799,#41800,#41801,#41802,#41803,#41804,#41805,#41806,
#41807,#41808,#41809,#41810,#41811),.UNSPECIFIED.,.F.,.F.,(4,3,3,3,3,3,
3,3,3,3,3,3,3,3,4),(-154.645421777951,-154.599570949852,-154.100862656465,
-153.602154363079,-153.103446069692,-152.604737776306,-152.106029482919,
-151.607321189532,-151.108612896146,-150.609904602759,-150.111196309372,
-149.612488015986,-149.113779722599,-148.615071429213,-148.362236470772),
 .UNSPECIFIED.);
#775=B_SPLINE_CURVE_WITH_KNOTS('',3,(#41816,#41817,#41818,#41819,#41820,
#41821,#41822,#41823,#41824,#41825,#41826,#41827,#41828,#41829,#41830,#41831,
#41832,#41833,#41834,#41835,#41836,#41837,#41838,#41839,#41840,#41841,#41842,
#41843,#41844,#41845,#41846,#41847,#41848,#41849,#41850,#41851,#41852,#41853,
#41854,#41855),.UNSPECIFIED.,.F.,.F.,(4,3,3,3,3,3,3,3,3,3,3,3,3,4),(145.822281066299,
146.121529962279,146.620238255666,147.118946549053,147.617654842439,148.116363135826,
148.615071429213,149.113779722599,149.612488015986,150.111196309372,150.609904602759,
151.108612896146,151.607321189532,152.105466373478),.UNSPECIFIED.);
#776=B_SPLINE_CURVE_WITH_KNOTS('',3,(#41856,#41857,#41858,#41859,#41860,
#41861,#41862,#41863,#41864,#41865,#41866,#41867,#41868,#41869,#41870,#41871,
#41872,#41873,#41874,#41875,#41876,#41877,#41878,#41879,#41880,#41881,#41882,
#41883,#41884,#41885,#41886,#41887,#41888,#41889,#41890,#41891,#41892,#41893,
#41894,#41895,#41896,#41897,#41898),.UNSPECIFIED.,.F.,.F.,(4,3,3,3,3,3,
3,3,3,3,3,3,3,3,4),(-148.362236470772,-148.116363135826,-147.617654842439,
-147.118946549053,-146.620238255666,-146.12152996228,-145.622821668893,
-145.124113375506,-144.62540508212,-144.126696788733,-143.627988495346,
-143.12928020196,-142.630571908573,-142.131863615187,-142.079051163592),
 .UNSPECIFIED.);
#777=B_SPLINE_CURVE_WITH_KNOTS('',3,(#41903,#41904,#41905,#41906,#41907,
#41908,#41909,#41910,#41911,#41912,#41913,#41914,#41915,#41916,#41917,#41918,
#41919,#41920,#41921,#41922,#41923,#41924,#41925,#41926,#41927,#41928,#41929,
#41930,#41931,#41932,#41933,#41934,#41935,#41936,#41937,#41938,#41939,#41940,
#41941,#41942,#41943,#41944,#41945),.UNSPECIFIED.,.F.,.F.,(4,3,3,3,3,3,
3,3,3,3,3,3,3,3,4),(139.539095759119,139.638322148253,140.13703044164,140.635738735027,
141.134447028413,141.6331553218,142.131863615187,142.630571908573,143.12928020196,
143.627988495346,144.126696788733,144.62540508212,145.124113375506,145.622821668893,
145.822281066299),.UNSPECIFIED.);
#778=B_SPLINE_CURVE_WITH_KNOTS('',3,(#41946,#41947,#41948,#41949,#41950,
#41951,#41952,#41953,#41954,#41955,#41956,#41957,#41958,#41959,#41960,#41961,
#41962,#41963,#41964,#41965,#41966,#41967,#41968,#41969,#41970,#41971,#41972,
#41973,#41974,#41975,#41976,#41977,#41978,#41979,#41980,#41981,#41982,#41983,
#41984,#41985),.UNSPECIFIED.,.F.,.F.,(4,3,3,3,3,3,3,3,3,3,3,3,3,4),(-142.079051163592,
-141.6331553218,-141.134447028413,-140.635738735027,-140.13703044164,-139.638322148253,
-139.139613854867,-138.64090556148,-138.142197268094,-137.643488974707,
-137.14478068132,-136.646072387934,-136.147364094547,-135.795865856413),
 .UNSPECIFIED.);
#779=B_SPLINE_CURVE_WITH_KNOTS('',3,(#41990,#41991,#41992,#41993,#41994,
#41995,#41996,#41997,#41998,#41999,#42000,#42001,#42002,#42003,#42004,#42005,
#42006,#42007,#42008,#42009,#42010,#42011,#42012,#42013,#42014,#42015,#42016,
#42017,#42018,#42019,#42020,#42021,#42022,#42023,#42024,#42025,#42026,#42027,
#42028,#42029),.UNSPECIFIED.,.F.,.F.,(4,3,3,3,3,3,3,3,3,3,3,3,3,4),(133.25591045194,
133.653822627614,134.152530921001,134.651239214387,135.149947507774,135.648655801161,
136.147364094547,136.646072387934,137.14478068132,137.643488974707,138.142197268094,
138.64090556148,139.139613854867,139.539095759119),.UNSPECIFIED.);
#780=B_SPLINE_CURVE_WITH_KNOTS('',3,(#42030,#42031,#42032,#42033,#42034,
#42035,#42036,#42037,#42038,#42039,#42040,#42041,#42042,#42043,#42044,#42045,
#42046,#42047,#42048,#42049,#42050,#42051,#42052,#42053,#42054,#42055,#42056,
#42057,#42058,#42059,#42060),.UNSPECIFIED.,.F.,.F.,(4,3,3,3,3,3,3,3,3,3,
4),(-135.795865856413,-135.648655801161,-135.149947507774,-134.651239214387,
-134.152530921001,-133.653822627614,-132.656406040841,-131.658989454068,
-130.661572867294,-129.664156280521,-129.512680549233),.UNSPECIFIED.);
#781=B_SPLINE_CURVE_WITH_KNOTS('',3,(#42065,#42066,#42067,#42068,#42069,
#42070,#42071,#42072,#42073,#42074,#42075,#42076,#42077,#42078,#42079,#42080,
#42081,#42082,#42083,#42084,#42085,#42086),.UNSPECIFIED.,.F.,.F.,(4,3,3,
3,3,3,3,4),(126.97272514476,127.669323106975,128.666739693748,129.664156280521,
130.661572867294,131.658989454068,132.656406040841,133.25591045194),
 .UNSPECIFIED.);
#782=B_SPLINE_CURVE_WITH_KNOTS('',3,(#42087,#42088,#42089,#42090,#42091,
#42092,#42093,#42094,#42095,#42096,#42097,#42098,#42099,#42100,#42101,#42102,
#42103,#42104,#42105,#42106,#42107,#42108),.UNSPECIFIED.,.F.,.F.,(4,3,3,
3,3,3,3,4),(-129.512680549233,-128.666739693748,-127.669323106975,-126.671906520201,
-125.674489933428,-124.677073346655,-123.679656759882,-123.229495242053),
 .UNSPECIFIED.);
#783=B_SPLINE_CURVE_WITH_KNOTS('',3,(#42113,#42114,#42115,#42116,#42117,
#42118,#42119,#42120,#42121,#42122,#42123,#42124,#42125,#42126,#42127,#42128,
#42129,#42130,#42131,#42132,#42133,#42134),.UNSPECIFIED.,.F.,.F.,(4,3,3,
3,3,3,3,4),(120.68953983758,121.684823586335,122.682240173108,123.679656759882,
124.677073346655,125.674489933428,126.671906520201,126.97272514476),
 .UNSPECIFIED.);
#784=B_SPLINE_CURVE_WITH_KNOTS('',3,(#42135,#42136,#42137,#42138,#42139,
#42140,#42141,#42142,#42143,#42144,#42145,#42146,#42147,#42148,#42149,#42150,
#42151,#42152,#42153,#42154,#42155,#42156,#42157,#42158,#42159,#42160,#42161,
#42162,#42163,#42164,#42165),.UNSPECIFIED.,.F.,.F.,(4,3,3,3,3,3,3,3,3,3,
4),(-123.229495242053,-122.682240173108,-121.684823586335,-120.687406999562,
-119.689990412789,-119.191282119402,-118.692573826015,-118.193865532629,
-117.695157239242,-117.196448945856,-116.946309934874),.UNSPECIFIED.);
#785=B_SPLINE_CURVE_WITH_KNOTS('',3,(#42170,#42171,#42172,#42173,#42174,
#42175,#42176,#42177,#42178,#42179,#42180,#42181,#42182,#42183,#42184,#42185,
#42186,#42187,#42188,#42189,#42190,#42191,#42192,#42193,#42194,#42195,#42196,
#42197,#42198,#42199,#42200,#42201,#42202,#42203,#42204,#42205,#42206,#42207,
#42208,#42209),.UNSPECIFIED.,.F.,.F.,(4,3,3,3,3,3,3,3,3,3,3,3,3,4),(114.406354530401,
114.702907478922,115.201615772309,115.700324065696,116.199032359082,116.697740652469,
117.196448945856,117.695157239242,118.193865532629,118.692573826015,119.191282119402,
119.689990412789,120.687406999562,120.68953983758),.UNSPECIFIED.);
#786=B_SPLINE_CURVE_WITH_KNOTS('',3,(#42210,#42211,#42212,#42213,#42214,
#42215,#42216,#42217,#42218,#42219,#42220,#42221,#42222,#42223,#42224,#42225,
#42226,#42227,#42228,#42229,#42230,#42231,#42232,#42233,#42234,#42235,#42236,
#42237,#42238,#42239,#42240,#42241,#42242,#42243,#42244,#42245,#42246,#42247,
#42248,#42249,#42250,#42251,#42252),.UNSPECIFIED.,.F.,.F.,(4,3,3,3,3,3,
3,3,3,3,3,3,3,3,4),(-116.946309934874,-116.697740652469,-116.199032359082,
-115.700324065696,-115.201615772309,-114.702907478922,-114.204199185536,
-113.705490892149,-113.206782598763,-112.708074305376,-112.209366011989,
-111.710657718603,-111.211949425216,-110.71324113183,-110.663124627694),
 .UNSPECIFIED.);
#787=B_SPLINE_CURVE_WITH_KNOTS('',3,(#42257,#42258,#42259,#42260,#42261,
#42262,#42263,#42264,#42265,#42266,#42267,#42268,#42269,#42270,#42271,#42272,
#42273,#42274,#42275,#42276,#42277,#42278,#42279,#42280,#42281,#42282,#42283,
#42284,#42285,#42286,#42287,#42288,#42289,#42290,#42291,#42292,#42293,#42294,
#42295,#42296,#42297,#42298,#42299),.UNSPECIFIED.,.F.,.F.,(4,3,3,3,3,3,
3,3,3,3,3,3,3,3,4),(108.123169223221,108.219699664896,108.718407958283,
109.21711625167,109.715824545056,110.214532838443,110.71324113183,111.211949425216,
111.710657718603,112.209366011989,112.708074305376,113.206782598763,113.705490892149,
114.204199185536,114.406354530401),.UNSPECIFIED.);
#788=B_SPLINE_CURVE_WITH_KNOTS('',3,(#42300,#42301,#42302,#42303,#42304,
#42305,#42306,#42307,#42308,#42309,#42310,#42311,#42312,#42313,#42314,#42315,
#42316,#42317,#42318,#42319,#42320,#42321,#42322,#42323,#42324,#42325,#42326,
#42327,#42328,#42329,#42330,#42331,#42332,#42333,#42334,#42335,#42336,#42337,
#42338,#42339),.UNSPECIFIED.,.F.,.F.,(4,3,3,3,3,3,3,3,3,3,3,3,3,4),(-110.663124627694,
-110.214532838443,-109.715824545056,-109.21711625167,-108.718407958283,
-108.219699664896,-107.72099137151,-107.222283078123,-106.723574784737,
-106.22486649135,-105.726158197963,-105.227449904577,-104.72874161119,-104.379939320515),
 .UNSPECIFIED.);
#789=B_SPLINE_CURVE_WITH_KNOTS('',3,(#42344,#42345,#42346,#42347,#42348,
#42349,#42350,#42351,#42352,#42353,#42354,#42355,#42356,#42357,#42358,#42359,
#42360,#42361,#42362,#42363,#42364,#42365,#42366,#42367,#42368,#42369,#42370,
#42371,#42372,#42373,#42374,#42375,#42376,#42377,#42378,#42379,#42380,#42381,
#42382,#42383),.UNSPECIFIED.,.F.,.F.,(4,3,3,3,3,3,3,3,3,3,3,3,3,4),(101.839983916042,
102.235200144257,102.733908437644,103.23261673103,103.731325024417,104.230033317804,
104.72874161119,105.227449904577,105.726158197963,106.22486649135,106.723574784737,
107.222283078123,107.72099137151,108.123169223221),.UNSPECIFIED.);
#790=B_SPLINE_CURVE_WITH_KNOTS('',3,(#42384,#42385,#42386,#42387,#42388,
#42389,#42390,#42391,#42392,#42393,#42394,#42395,#42396,#42397,#42398,#42399,
#42400,#42401,#42402,#42403,#42404,#42405,#42406,#42407,#42408,#42409,#42410,
#42411,#42412,#42413,#42414,#42415,#42416,#42417,#42418,#42419,#42420,#42421,
#42422,#42423,#42424,#42425,#42426),.UNSPECIFIED.,.F.,.F.,(4,3,3,3,3,3,
3,3,3,3,3,3,3,3,4),(-104.379939320515,-104.230033317803,-103.731325024417,
-103.23261673103,-102.733908437644,-102.235200144257,-101.73649185087,-101.237783557484,
-100.739075264097,-100.24036697071,-99.7416586773239,-99.2429503839373,
-98.7442420905506,-98.245533797164,-98.096754013335),.UNSPECIFIED.);
#791=B_SPLINE_CURVE_WITH_KNOTS('',3,(#42431,#42432,#42433,#42434,#42435,
#42436,#42437,#42438,#42439,#42440,#42441,#42442,#42443,#42444,#42445,#42446,
#42447,#42448,#42449,#42450,#42451,#42452,#42453,#42454,#42455,#42456,#42457,
#42458,#42459,#42460,#42461,#42462,#42463,#42464,#42465,#42466,#42467,#42468,
#42469,#42470,#42471,#42472,#42473),.UNSPECIFIED.,.F.,.F.,(4,3,3,3,3,3,
3,3,3,3,3,3,3,3,4),(95.556798608862,95.751992330231,96.2507006236176,96.7494089170042,
97.2481172103908,97.7468255037774,98.2455337971641,98.7442420905507,99.2429503839373,
99.7416586773239,100.240366970711,100.739075264097,101.237783557484,101.73649185087,
101.839983916042),.UNSPECIFIED.);
#792=B_SPLINE_CURVE_WITH_KNOTS('',3,(#42474,#42475,#42476,#42477,#42478,
#42479,#42480,#42481,#42482,#42483,#42484,#42485,#42486,#42487,#42488,#42489,
#42490,#42491,#42492,#42493,#42494,#42495,#42496,#42497,#42498,#42499,#42500,
#42501,#42502,#42503,#42504,#42505,#42506,#42507,#42508,#42509,#42510,#42511,
#42512,#42513),.UNSPECIFIED.,.F.,.F.,(4,3,3,3,3,3,3,3,3,3,3,3,3,4),(-98.096754013335,
-97.7468255037774,-97.2481172103908,-96.7494089170042,-96.2507006236176,
-95.7519923302309,-95.2532840368443,-94.7545757434577,-94.2558674500711,
-93.7571591566845,-93.2584508632978,-92.7597425699112,-92.2610342765246,
-91.8135687061554),.UNSPECIFIED.);
#793=B_SPLINE_CURVE_WITH_KNOTS('',3,(#42518,#42519,#42520,#42521,#42522,
#42523,#42524,#42525,#42526,#42527,#42528,#42529,#42530,#42531,#42532,#42533,
#42534,#42535,#42536,#42537,#42538,#42539,#42540,#42541,#42542,#42543,#42544,
#42545,#42546,#42547,#42548,#42549,#42550,#42551,#42552,#42553,#42554,#42555,
#42556,#42557),.UNSPECIFIED.,.F.,.F.,(4,3,3,3,3,3,3,3,3,3,3,3,3,4),(89.2736133016824,
89.7674928095915,90.2662011029781,90.7649093963648,91.2636176897514,91.762325983138,
92.2610342765246,92.7597425699113,93.2584508632979,93.7571591566845,94.2558674500711,
94.7545757434577,95.2532840368443,95.556798608862),.UNSPECIFIED.);
#794=B_SPLINE_CURVE_WITH_KNOTS('',3,(#42558,#42559,#42560,#42561,#42562,
#42563,#42564,#42565,#42566,#42567,#42568,#42569,#42570,#42571,#42572,#42573,
#42574,#42575,#42576,#42577,#42578,#42579,#42580,#42581,#42582,#42583,#42584,
#42585,#42586,#42587,#42588,#42589,#42590,#42591,#42592,#42593,#42594,#42595,
#42596,#42597,#42598,#42599,#42600),.UNSPECIFIED.,.F.,.F.,(4,3,3,3,3,3,
3,3,3,3,3,3,3,3,4),(-91.8135687061554,-91.762325983138,-91.2636176897513,
-90.7649093963647,-90.2662011029781,-89.7674928095915,-89.2687845162049,
-88.7700762228182,-88.2713679294316,-87.772659636045,-87.2739513426584,
-86.7752430492718,-86.2765347558852,-85.7778264624986,-85.5303833989758),
 .UNSPECIFIED.);
#795=B_SPLINE_CURVE_WITH_KNOTS('',3,(#42605,#42606,#42607,#42608,#42609,
#42610,#42611,#42612,#42613,#42614,#42615,#42616,#42617,#42618,#42619,#42620,
#42621,#42622,#42623,#42624,#42625,#42626,#42627,#42628,#42629,#42630,#42631,
#42632,#42633,#42634,#42635,#42636,#42637,#42638,#42639,#42640,#42641,#42642,
#42643,#42644,#42645,#42646,#42647),.UNSPECIFIED.,.F.,.F.,(4,3,3,3,3,3,
3,3,3,3,3,3,3,3,4),(82.9904279945028,83.2842849955655,83.7829932889521,
84.2817015823387,84.7804098757253,85.279118169112,85.7778264624986,86.2765347558852,
86.7752430492718,87.2739513426584,87.772659636045,88.2713679294317,88.7700762228183,
89.2687845162049,89.2736133016824),.UNSPECIFIED.);
#796=B_SPLINE_CURVE_WITH_KNOTS('',3,(#42648,#42649,#42650,#42651,#42652,
#42653,#42654,#42655,#42656,#42657,#42658,#42659,#42660,#42661,#42662,#42663,
#42664,#42665,#42666,#42667,#42668,#42669,#42670,#42671,#42672,#42673,#42674,
#42675,#42676,#42677,#42678,#42679,#42680,#42681,#42682,#42683,#42684,#42685,
#42686,#42687,#42688,#42689,#42690),.UNSPECIFIED.,.F.,.F.,(4,3,3,3,3,3,
3,3,3,3,3,3,3,3,4),(-85.5303833989758,-85.2791181691119,-84.7804098757253,
-84.2817015823387,-83.7829932889521,-83.2842849955654,-82.7855767021788,
-82.2868684087922,-81.7881601154056,-81.289451822019,-80.7907435286323,
-80.2920352352457,-79.7933269418591,-79.2946186484725,-79.2471980917962),
 .UNSPECIFIED.);
#797=B_SPLINE_CURVE_WITH_KNOTS('',3,(#42695,#42696,#42697,#42698,#42699,
#42700,#42701,#42702,#42703,#42704,#42705,#42706,#42707,#42708,#42709,#42710,
#42711,#42712,#42713,#42714,#42715,#42716,#42717,#42718,#42719,#42720,#42721,
#42722,#42723,#42724,#42725,#42726,#42727,#42728,#42729,#42730,#42731,#42732,
#42733,#42734,#42735,#42736,#42737),.UNSPECIFIED.,.F.,.F.,(4,3,3,3,3,3,
3,3,3,3,3,3,3,3,4),(76.7072426873232,76.8010771815394,77.299785474926,77.7984937683127,
78.2972020616993,78.7959103550859,79.2946186484725,79.7933269418591,80.2920352352457,
80.7907435286324,81.289451822019,81.7881601154056,82.2868684087922,82.7855767021789,
82.9904279945028),.UNSPECIFIED.);
#798=B_SPLINE_CURVE_WITH_KNOTS('',3,(#42738,#42739,#42740,#42741,#42742,
#42743,#42744,#42745,#42746,#42747,#42748,#42749,#42750,#42751,#42752,#42753,
#42754,#42755,#42756,#42757,#42758,#42759,#42760,#42761,#42762,#42763,#42764,
#42765,#42766,#42767,#42768,#42769,#42770,#42771,#42772,#42773,#42774,#42775,
#42776,#42777),.UNSPECIFIED.,.F.,.F.,(4,3,3,3,3,3,3,3,3,3,3,3,3,4),(-79.2471980917962,
-78.7959103550859,-78.2972020616993,-77.7984937683126,-77.299785474926,
-76.8010771815394,-76.3023688881528,-75.8036605947662,-75.3049523013795,
-74.8062440079929,-74.3075357146063,-73.8088274212197,-73.3101191278331,
-72.9640127846166),.UNSPECIFIED.);
#799=B_SPLINE_CURVE_WITH_KNOTS('',3,(#42782,#42783,#42784,#42785,#42786,
#42787,#42788,#42789,#42790,#42791,#42792,#42793,#42794,#42795,#42796,#42797,
#42798,#42799,#42800,#42801,#42802,#42803,#42804,#42805,#42806,#42807,#42808,
#42809,#42810,#42811,#42812,#42813,#42814,#42815,#42816,#42817,#42818,#42819,
#42820,#42821),.UNSPECIFIED.,.F.,.F.,(4,3,3,3,3,3,3,3,3,3,3,3,3,4),(70.4240573801436,
70.8165776609,71.3152859542866,71.8139942476732,72.3127025410598,72.8114108344465,
73.3101191278331,73.8088274212197,74.3075357146063,74.8062440079929,75.3049523013796,
75.8036605947662,76.3023688881528,76.7072426873232),.UNSPECIFIED.);
#800=B_SPLINE_CURVE_WITH_KNOTS('',3,(#42822,#42823,#42824,#42825,#42826,
#42827,#42828,#42829,#42830,#42831,#42832,#42833,#42834,#42835,#42836,#42837,
#42838,#42839,#42840,#42841,#42842,#42843,#42844,#42845,#42846,#42847,#42848,
#42849,#42850,#42851,#42852,#42853,#42854,#42855,#42856,#42857,#42858,#42859,
#42860,#42861,#42862,#42863,#42864),.UNSPECIFIED.,.F.,.F.,(4,3,3,3,3,3,
3,3,3,3,3,3,3,3,4),(-72.9640127846166,-72.8114108344464,-72.3127025410598,
-71.8139942476732,-71.3152859542866,-70.8165776609,-70.3178693675133,-69.8191610741267,
-69.3204527807401,-68.8217444873535,-68.3230361939669,-67.8243279005802,
-67.3256196071936,-66.826911313807,-66.680827477437),.UNSPECIFIED.);
#801=B_SPLINE_CURVE_WITH_KNOTS('',3,(#42869,#42870,#42871,#42872,#42873,
#42874,#42875,#42876,#42877,#42878,#42879,#42880,#42881,#42882,#42883,#42884,
#42885,#42886,#42887,#42888,#42889,#42890,#42891,#42892,#42893,#42894,#42895,
#42896,#42897,#42898,#42899,#42900,#42901,#42902,#42903,#42904,#42905,#42906,
#42907,#42908,#42909,#42910,#42911),.UNSPECIFIED.,.F.,.F.,(4,3,3,3,3,3,
3,3,3,3,3,3,3,3,4),(64.140872072964,64.3333698468739,64.8320781402605,65.3307864336472,
65.8294947270338,66.3282030204204,66.826911313807,67.3256196071937,67.8243279005803,
68.3230361939669,68.8217444873535,69.3204527807401,69.8191610741268,70.3178693675134,
70.4240573801436),.UNSPECIFIED.);
#802=B_SPLINE_CURVE_WITH_KNOTS('',3,(#42912,#42913,#42914,#42915,#42916,
#42917,#42918,#42919,#42920,#42921,#42922,#42923,#42924,#42925,#42926,#42927,
#42928,#42929,#42930,#42931,#42932,#42933,#42934,#42935,#42936,#42937,#42938,
#42939,#42940,#42941,#42942,#42943,#42944,#42945,#42946,#42947,#42948,#42949,
#42950,#42951),.UNSPECIFIED.,.F.,.F.,(4,3,3,3,3,3,3,3,3,3,3,3,3,4),(-66.680827477437,
-66.3282030204204,-65.8294947270337,-65.3307864336471,-64.8320781402605,
-64.3333698468739,-63.8346615534873,-63.3359532601007,-62.837244966714,
-62.3385366733274,-61.8398283799408,-61.3411200865542,-60.8424117931676,
-60.3976421702575),.UNSPECIFIED.);
#803=B_SPLINE_CURVE_WITH_KNOTS('',3,(#42956,#42957,#42958,#42959,#42960,
#42961,#42962,#42963,#42964,#42965,#42966,#42967,#42968,#42969,#42970,#42971,
#42972,#42973,#42974,#42975,#42976,#42977,#42978,#42979,#42980,#42981,#42982,
#42983,#42984,#42985,#42986,#42987,#42988,#42989,#42990,#42991,#42992,#42993,
#42994,#42995),.UNSPECIFIED.,.F.,.F.,(4,3,3,3,3,3,3,3,3,3,3,3,3,4),(57.8576867657844,
58.3488703262345,58.8475786196211,59.3462869130077,59.8449952063944,60.343703499781,
60.8424117931676,61.3411200865542,61.8398283799408,62.3385366733274,62.8372449667141,
63.3359532601007,63.8346615534873,64.140872072964),.UNSPECIFIED.);
#804=B_SPLINE_CURVE_WITH_KNOTS('',3,(#42996,#42997,#42998,#42999,#43000,
#43001,#43002,#43003,#43004,#43005,#43006,#43007,#43008,#43009,#43010,#43011,
#43012,#43013,#43014,#43015,#43016,#43017,#43018,#43019,#43020,#43021,#43022,
#43023,#43024,#43025,#43026,#43027,#43028,#43029,#43030,#43031,#43032,#43033,
#43034,#43035,#43036,#43037,#43038),.UNSPECIFIED.,.F.,.F.,(4,3,3,3,3,3,
3,3,3,3,3,3,3,3,4),(-60.3976421702575,-60.3437034997809,-59.8449952063943,
-59.3462869130077,-58.8475786196211,-58.3488703262345,-57.8501620328479,
-57.3514537394612,-56.8527454460746,-56.354037152688,-55.8553288593014,
-55.3566205659148,-54.8579122725281,-54.3592039791415,-54.1144568630779),
 .UNSPECIFIED.);
#805=B_SPLINE_CURVE_WITH_KNOTS('',3,(#43043,#43044,#43045,#43046,#43047,
#43048,#43049,#43050,#43051,#43052,#43053,#43054,#43055,#43056,#43057,#43058,
#43059,#43060,#43061,#43062,#43063,#43064,#43065,#43066,#43067,#43068,#43069,
#43070,#43071,#43072,#43073,#43074,#43075,#43076,#43077,#43078,#43079,#43080,
#43081,#43082,#43083,#43084,#43085),.UNSPECIFIED.,.F.,.F.,(4,3,3,3,3,3,
3,3,3,3,3,3,3,3,4),(51.5745014586048,51.8656625122084,52.3643708055951,
52.8630790989817,53.3617873923683,53.8604956857549,54.3592039791415,54.8579122725282,
55.3566205659148,55.8553288593014,56.354037152688,56.8527454460746,57.3514537394612,
57.8501620328479,57.8576867657844),.UNSPECIFIED.);
#806=B_SPLINE_CURVE_WITH_KNOTS('',3,(#43086,#43087,#43088,#43089,#43090,
#43091,#43092,#43093,#43094,#43095,#43096,#43097,#43098,#43099,#43100,#43101,
#43102,#43103,#43104,#43105,#43106,#43107,#43108,#43109,#43110,#43111,#43112,
#43113,#43114,#43115,#43116,#43117,#43118,#43119,#43120,#43121,#43122,#43123,
#43124,#43125,#43126,#43127,#43128),.UNSPECIFIED.,.F.,.F.,(4,3,3,3,3,3,
3,3,3,3,3,3,3,3,4),(-54.1144568630779,-53.8604956857549,-53.3617873923683,
-52.8630790989817,-52.3643708055951,-51.8656625122084,-51.3669542188218,
-50.8682459254352,-50.3695376320486,-49.8708293386619,-49.3721210452753,
-48.8734127518887,-48.3747044585021,-47.8759961651155,-47.8312715558983),
 .UNSPECIFIED.);
#807=B_SPLINE_CURVE_WITH_KNOTS('',3,(#43133,#43134,#43135,#43136,#43137,
#43138,#43139,#43140,#43141,#43142,#43143,#43144,#43145,#43146,#43147,#43148,
#43149,#43150,#43151,#43152,#43153,#43154,#43155,#43156,#43157,#43158,#43159,
#43160,#43161,#43162,#43163,#43164,#43165,#43166,#43167,#43168,#43169,#43170,
#43171,#43172,#43173,#43174,#43175),.UNSPECIFIED.,.F.,.F.,(4,3,3,3,3,3,
3,3,3,3,3,3,3,3,4),(45.2913161514252,45.3824546981824,45.881162991569,46.3798712849556,
46.8785795783422,47.3772878717289,47.8759961651155,48.3747044585021,48.8734127518887,
49.3721210452753,49.870829338662,50.3695376320486,50.8682459254352,51.3669542188218,
51.5745014586048),.UNSPECIFIED.);
#808=B_SPLINE_CURVE_WITH_KNOTS('',3,(#43176,#43177,#43178,#43179,#43180,
#43181,#43182,#43183,#43184,#43185,#43186,#43187,#43188,#43189,#43190,#43191,
#43192,#43193,#43194,#43195,#43196,#43197,#43198,#43199,#43200,#43201,#43202,
#43203,#43204,#43205,#43206,#43207,#43208,#43209,#43210,#43211,#43212,#43213,
#43214,#43215),.UNSPECIFIED.,.F.,.F.,(4,3,3,3,3,3,3,3,3,3,3,3,3,4),(-47.8312715558983,
-47.3772878717289,-46.8785795783422,-46.3798712849556,-45.881162991569,
-45.3824546981824,-44.8837464047958,-44.3850381114091,-43.8863298180225,
-43.3876215246359,-42.8889132312493,-42.3902049378627,-41.891496644476,
-41.5480862487187),.UNSPECIFIED.);
#809=B_SPLINE_CURVE_WITH_KNOTS('',3,(#43220,#43221,#43222,#43223,#43224,
#43225,#43226,#43227,#43228,#43229,#43230,#43231,#43232,#43233,#43234,#43235,
#43236,#43237,#43238,#43239,#43240,#43241,#43242,#43243,#43244,#43245,#43246,
#43247,#43248,#43249,#43250,#43251,#43252,#43253,#43254,#43255,#43256,#43257,
#43258,#43259),.UNSPECIFIED.,.F.,.F.,(4,3,3,3,3,3,3,3,3,3,3,3,3,4),(39.0081308442456,
39.3979551775429,39.8966634709296,40.3953717643162,40.8940800577028,41.3927883510894,
41.891496644476,42.3902049378627,42.8889132312493,43.3876215246359,43.8863298180225,
44.3850381114091,44.8837464047958,45.2913161514252),.UNSPECIFIED.);
#810=B_SPLINE_CURVE_WITH_KNOTS('',3,(#43260,#43261,#43262,#43263,#43264,
#43265,#43266,#43267,#43268,#43269,#43270,#43271,#43272,#43273,#43274,#43275,
#43276,#43277,#43278,#43279,#43280,#43281,#43282,#43283,#43284,#43285,#43286,
#43287,#43288,#43289,#43290,#43291,#43292,#43293,#43294,#43295,#43296,#43297,
#43298,#43299,#43300,#43301,#43302),.UNSPECIFIED.,.F.,.F.,(4,3,3,3,3,3,
3,3,3,3,3,3,3,3,4),(-41.5480862487187,-41.3927883510894,-40.8940800577028,
-40.3953717643162,-39.8966634709296,-39.3979551775429,-38.8992468841563,
-38.4005385907697,-37.9018302973831,-37.4031220039965,-36.9044137106098,
-36.4057054172232,-35.9069971238366,-35.40828883045,-35.2649009415391),
 .UNSPECIFIED.);
#811=B_SPLINE_CURVE_WITH_KNOTS('',3,(#43307,#43308,#43309,#43310,#43311,
#43312,#43313,#43314,#43315,#43316,#43317,#43318,#43319,#43320,#43321,#43322,
#43323,#43324,#43325,#43326,#43327,#43328,#43329,#43330,#43331,#43332,#43333,
#43334,#43335,#43336,#43337,#43338,#43339,#43340,#43341,#43342,#43343,#43344,
#43345,#43346,#43347,#43348,#43349),.UNSPECIFIED.,.F.,.F.,(4,3,3,3,3,3,
3,3,3,3,3,3,3,3,4),(32.7249455370661,32.9147473635169,33.4134556569035,
33.9121639502901,34.4108722436767,34.9095805370634,35.40828883045,35.9069971238366,
36.4057054172232,36.9044137106099,37.4031220039965,37.9018302973831,38.4005385907697,
38.8992468841563,39.0081308442456),.UNSPECIFIED.);
#812=B_SPLINE_CURVE_WITH_KNOTS('',3,(#43350,#43351,#43352,#43353,#43354,
#43355,#43356,#43357,#43358,#43359,#43360,#43361,#43362,#43363,#43364,#43365,
#43366,#43367,#43368,#43369,#43370,#43371,#43372,#43373,#43374,#43375,#43376,
#43377,#43378,#43379,#43380,#43381,#43382,#43383,#43384,#43385,#43386,#43387,
#43388,#43389),.UNSPECIFIED.,.F.,.F.,(4,3,3,3,3,3,3,3,3,3,3,3,3,4),(-35.2649009415391,
-34.9095805370634,-34.4108722436767,-33.9121639502901,-33.4134556569035,
-32.9147473635169,-32.4160390701303,-31.9173307767436,-31.418622483357,
-30.9199141899704,-30.4212058965838,-29.9224976031972,-29.4237893098105,
-28.9817156343595),.UNSPECIFIED.);
#813=B_SPLINE_CURVE_WITH_KNOTS('',3,(#43394,#43395,#43396,#43397,#43398,
#43399,#43400,#43401,#43402,#43403,#43404,#43405,#43406,#43407,#43408,#43409,
#43410,#43411,#43412,#43413,#43414,#43415,#43416,#43417,#43418,#43419,#43420,
#43421,#43422,#43423,#43424,#43425,#43426,#43427,#43428,#43429,#43430,#43431,
#43432,#43433),.UNSPECIFIED.,.F.,.F.,(4,3,3,3,3,3,3,3,3,3,3,3,3,4),(26.4417602298865,
26.9302478428775,27.4289561362641,27.9276644296507,28.4263727230373,28.9250810164239,
29.4237893098106,29.9224976031972,30.4212058965838,30.9199141899704,31.418622483357,
31.9173307767437,32.4160390701303,32.7249455370661),.UNSPECIFIED.);
#814=B_SPLINE_CURVE_WITH_KNOTS('',3,(#43434,#43435,#43436,#43437,#43438,
#43439,#43440,#43441,#43442,#43443,#43444,#43445,#43446,#43447,#43448,#43449,
#43450,#43451,#43452,#43453,#43454,#43455,#43456,#43457,#43458,#43459,#43460,
#43461,#43462,#43463,#43464,#43465,#43466,#43467,#43468,#43469,#43470,#43471,
#43472,#43473,#43474,#43475,#43476),.UNSPECIFIED.,.F.,.F.,(4,3,3,3,3,3,
3,3,3,3,3,3,3,3,4),(-28.9817156343595,-28.9250810164239,-28.4263727230373,
-27.9276644296507,-27.4289561362641,-26.9302478428774,-26.4315395494908,
-25.9328312561042,-25.4341229627176,-24.935414669331,-24.4367063759443,
-23.9379980825577,-23.4392897891711,-22.9405814957845,-22.6985303271799),
 .UNSPECIFIED.);
#815=B_SPLINE_CURVE_WITH_KNOTS('',3,(#43481,#43482,#43483,#43484,#43485,
#43486,#43487,#43488,#43489,#43490,#43491,#43492,#43493,#43494,#43495,#43496,
#43497,#43498,#43499,#43500,#43501,#43502,#43503,#43504,#43505,#43506,#43507,
#43508,#43509,#43510,#43511,#43512,#43513,#43514,#43515,#43516,#43517,#43518,
#43519,#43520,#43521,#43522,#43523),.UNSPECIFIED.,.F.,.F.,(4,3,3,3,3,3,
3,3,3,3,3,3,3,3,4),(20.1585749227069,20.4470400288514,20.945748322238,21.4444566156246,
21.9431649090113,22.4418732023979,22.9405814957845,23.4392897891711,23.9379980825577,
24.4367063759444,24.935414669331,25.4341229627176,25.9328312561042,26.4315395494908,
26.4417602298865),.UNSPECIFIED.);
#816=B_SPLINE_CURVE_WITH_KNOTS('',3,(#43524,#43525,#43526,#43527,#43528,
#43529,#43530,#43531,#43532,#43533,#43534,#43535,#43536,#43537,#43538,#43539,
#43540,#43541,#43542,#43543,#43544,#43545,#43546,#43547,#43548,#43549,#43550,
#43551,#43552,#43553,#43554,#43555,#43556,#43557,#43558,#43559,#43560,#43561,
#43562,#43563,#43564,#43565,#43566),.UNSPECIFIED.,.F.,.F.,(4,3,3,3,3,3,
3,3,3,3,3,3,3,3,4),(-22.6985303271799,-22.4418732023979,-21.9431649090112,
-21.4444566156246,-20.945748322238,-20.4470400288514,-19.9483317354648,
-19.4496234420782,-18.9509151486915,-18.4522068553049,-17.9534985619183,
-17.4547902685317,-16.9560819751451,-16.4573736817584,-16.4153450200003),
 .UNSPECIFIED.);
#817=B_SPLINE_CURVE_WITH_KNOTS('',3,(#43571,#43572,#43573,#43574,#43575,
#43576,#43577,#43578,#43579,#43580,#43581,#43582,#43583,#43584,#43585,#43586,
#43587,#43588,#43589,#43590,#43591,#43592,#43593,#43594,#43595,#43596,#43597,
#43598,#43599,#43600,#43601,#43602,#43603,#43604,#43605,#43606,#43607,#43608,
#43609,#43610,#43611,#43612,#43613),.UNSPECIFIED.,.F.,.F.,(4,3,3,3,3,3,
3,3,3,3,3,3,3,3,4),(13.8753896155273,13.9638322148253,14.462540508212,14.9612488015986,
15.4599570949852,15.9586653883718,16.4573736817584,16.9560819751451,17.4547902685317,
17.9534985619183,18.4522068553049,18.9509151486915,19.4496234420782,19.9483317354648,
20.1585749227069),.UNSPECIFIED.);
#818=B_SPLINE_CURVE_WITH_KNOTS('',3,(#43614,#43615,#43616,#43617,#43618,
#43619,#43620,#43621,#43622,#43623,#43624,#43625,#43626,#43627,#43628,#43629,
#43630,#43631,#43632,#43633,#43634,#43635,#43636,#43637,#43638,#43639,#43640,
#43641,#43642,#43643,#43644,#43645,#43646,#43647,#43648,#43649,#43650,#43651,
#43652,#43653),.UNSPECIFIED.,.F.,.F.,(4,3,3,3,3,3,3,3,3,3,3,3,3,4),(-16.4153450200003,
-15.9586653883718,-15.4599570949852,-14.9612488015986,-14.462540508212,
-13.9638322148253,-13.4651239214387,-12.9664156280521,-12.4677073346655,
-11.9689990412789,-11.4702907478922,-10.9715824545056,-10.472874161119,
-10.1321597128207),.UNSPECIFIED.);
#819=B_SPLINE_CURVE_WITH_KNOTS('',3,(#43659,#43660,#43661,#43662,#43663,
#43664,#43665,#43666,#43667,#43668,#43669,#43670,#43671,#43672,#43673,#43674,
#43675,#43676,#43677,#43678,#43679,#43680,#43681,#43682,#43683),
 .UNSPECIFIED.,.F.,.F.,(4,3,3,3,3,3,3,3,4),(-3.84897440564115,-3.49095805370634,
-2.99224976031972,-2.4935414669331,-1.99483317354648,-1.49612488015986,
-0.997416586773239,-0.49870829338662,0.),.UNSPECIFIED.);
#820=B_SPLINE_CURVE_WITH_KNOTS('',3,(#43686,#43687,#43688,#43689,#43690,
#43691,#43692,#43693,#43694,#43695,#43696,#43697,#43698,#43699,#43700,#43701,
#43702,#43703,#43704,#43705,#43706,#43707,#43708,#43709,#43710,#43711,#43712,
#43713,#43714,#43715,#43716,#43717,#43718,#43719,#43720,#43721,#43722),
 .UNSPECIFIED.,.F.,.F.,(4,3,3,3,3,3,3,3,3,3,3,3,4),(2.01640075321917,2.4935414669331,
2.99224976031972,3.49095805370634,3.98966634709296,4.48837464047958,4.9870829338662,
5.48579122725282,5.98449952063944,6.48320781402605,6.98191610741268,7.48062440079929,
7.59220430834772),.UNSPECIFIED.);
#821=B_SPLINE_CURVE_WITH_KNOTS('',3,(#43728,#43729,#43730,#43731,#43732,
#43733,#43734,#43735,#43736,#43737,#43738,#43739),.UNSPECIFIED.,.F.,.F.,
(4,1,1,1,1,1,1,1,1,4),(260.752190247953,261.213135555618,261.711843849004,
262.210552142391,262.709260435778,263.207968729164,263.706677022551,264.205385315938,
264.704093609324,265.202801902711),.UNSPECIFIED.);
#822=B_SPLINE_CURVE_WITH_KNOTS('',3,(#43742,#43743,#43744,#43745,#43746,
#43747,#43748,#43749,#43750,#43751,#43752,#43753,#43754,#43755),
 .UNSPECIFIED.,.F.,.F.,(4,1,1,1,1,1,1,1,1,1,1,4),(260.752190247953,260.760841199772,
261.259549493158,261.758257786545,262.256966079931,262.755674373318,263.254382666705,
263.753090960091,264.251799253478,264.750507546865,265.249215840251,265.726356553965),
 .UNSPECIFIED.);
#823=B_SPLINE_CURVE_WITH_KNOTS('',3,(#43760,#43761,#43762,#43763,#43764,
#43765,#43766,#43767,#43768,#43769,#43770,#43771,#43772,#43773,#43774,#43775,
#43776),.UNSPECIFIED.,.F.,.F.,(4,1,1,1,1,1,1,1,1,1,1,1,1,1,4),(254.469004940773,
254.729927741592,255.228636034978,255.727344328365,256.226052621752,256.724760915138,
257.223469208525,257.722177501912,258.220885795298,258.719594088685,259.218302382071,
259.717010675458,260.215718968845,260.714427262231,260.752190247953),
 .UNSPECIFIED.);
#824=B_SPLINE_CURVE_WITH_KNOTS('',3,(#43777,#43778,#43779,#43780,#43781,
#43782,#43783,#43784,#43785,#43786,#43787,#43788,#43789,#43790,#43791,#43792),
 .UNSPECIFIED.,.F.,.F.,(4,1,1,1,1,1,1,1,1,1,1,1,1,4),(254.469004940773,
254.776341679132,255.275049972519,255.773758265905,256.272466559292,256.771174852679,
257.269883146065,257.768591439452,258.267299732838,258.766008026225,259.264716319612,
259.763424612998,260.262132906385,260.752190247953),.UNSPECIFIED.);
#825=B_SPLINE_CURVE_WITH_KNOTS('',3,(#43797,#43798,#43799,#43800,#43801,
#43802,#43803,#43804,#43805,#43806,#43807,#43808,#43809,#43810,#43811,#43812,
#43813),.UNSPECIFIED.,.F.,.F.,(4,1,1,1,1,1,1,1,1,1,1,1,1,1,4),(248.185819633594,
248.246719927566,248.745428220952,249.244136514339,249.742844807726,250.241553101112,
250.740261394499,251.238969687886,251.737677981272,252.236386274659,252.735094568045,
253.233802861432,253.732511154819,254.231219448205,254.469004940773),
 .UNSPECIFIED.);
#826=B_SPLINE_CURVE_WITH_KNOTS('',3,(#43814,#43815,#43816,#43817,#43818,
#43819,#43820,#43821,#43822,#43823,#43824,#43825,#43826,#43827,#43828,#43829,
#43830),.UNSPECIFIED.,.F.,.F.,(4,1,1,1,1,1,1,1,1,1,1,1,1,1,4),(248.185819633594,
248.293133865106,248.791842158493,249.290550451879,249.789258745266,250.287967038653,
250.786675332039,251.285383625426,251.784091918812,252.282800212199,252.781508505586,
253.280216798972,253.778925092359,254.277633385745,254.469004940773),
 .UNSPECIFIED.);
#827=B_SPLINE_CURVE_WITH_KNOTS('',3,(#43835,#43836,#43837,#43838,#43839,
#43840,#43841,#43842,#43843,#43844,#43845,#43846,#43847,#43848,#43849,#43850),
 .UNSPECIFIED.,.F.,.F.,(4,1,1,1,1,1,1,1,1,1,1,1,1,4),(241.902634326414,
242.262220406926,242.760928700313,243.2596369937,243.758345287086,244.257053580473,
244.755761873859,245.254470167246,245.753178460633,246.251886754019,246.750595047406,
247.249303340793,247.748011634179,248.185819633594),.UNSPECIFIED.);
#828=B_SPLINE_CURVE_WITH_KNOTS('',3,(#43851,#43852,#43853,#43854,#43855,
#43856,#43857,#43858,#43859,#43860,#43861,#43862,#43863,#43864,#43865,#43866),
 .UNSPECIFIED.,.F.,.F.,(4,1,1,1,1,1,1,1,1,1,1,1,1,4),(241.902634326414,
242.308634344467,242.807342637853,243.30605093124,243.804759224626,244.303467518013,
244.8021758114,245.300884104786,245.799592398173,246.29830069156,246.797008984946,
247.295717278333,247.794425571719,248.185819633594),.UNSPECIFIED.);
#829=B_SPLINE_CURVE_WITH_KNOTS('',3,(#43871,#43872,#43873,#43874,#43875,
#43876,#43877,#43878,#43879,#43880,#43881,#43882,#43883,#43884,#43885,#43886,
#43887),.UNSPECIFIED.,.F.,.F.,(4,1,1,1,1,1,1,1,1,1,1,1,1,1,4),(235.619449019235,
235.7790125929,236.277720886287,236.776429179674,237.27513747306,237.773845766447,
238.272554059833,238.77126235322,239.269970646607,239.768678939993,240.26738723338,
240.766095526767,241.264803820153,241.76351211354,241.902634326414),
 .UNSPECIFIED.);
#830=B_SPLINE_CURVE_WITH_KNOTS('',3,(#43888,#43889,#43890,#43891,#43892,
#43893,#43894,#43895,#43896,#43897,#43898,#43899,#43900,#43901,#43902,#43903,
#43904),.UNSPECIFIED.,.F.,.F.,(4,1,1,1,1,1,1,1,1,1,1,1,1,1,4),(235.619449019235,
235.825426530441,236.324134823827,236.822843117214,237.3215514106,237.820259703987,
238.318967997374,238.81767629076,239.316384584147,239.815092877534,240.31380117092,
240.812509464307,241.311217757693,241.80992605108,241.902634326414),
 .UNSPECIFIED.);
#831=B_SPLINE_CURVE_WITH_KNOTS('',3,(#43909,#43910,#43911,#43912,#43913,
#43914,#43915,#43916,#43917,#43918,#43919,#43920,#43921,#43922,#43923,#43924),
 .UNSPECIFIED.,.F.,.F.,(4,1,1,1,1,1,1,1,1,1,1,1,1,4),(229.336263712055,
229.794513072261,230.293221365647,230.791929659034,231.290637952421,231.789346245807,
232.288054539194,232.786762832581,233.285471125967,233.784179419354,234.28288771274,
234.781596006127,235.280304299514,235.619449019235),.UNSPECIFIED.);
#832=B_SPLINE_CURVE_WITH_KNOTS('',3,(#43925,#43926,#43927,#43928,#43929,
#43930,#43931,#43932,#43933,#43934,#43935,#43936,#43937,#43938,#43939,#43940,
#43941),.UNSPECIFIED.,.F.,.F.,(4,1,1,1,1,1,1,1,1,1,1,1,1,1,4),(229.336263712055,
229.342218716414,229.840927009801,230.339635303188,230.838343596574,231.337051889961,
231.835760183348,232.334468476734,232.833176770121,233.331885063507,233.830593356894,
234.329301650281,234.828009943667,235.326718237054,235.619449019235),
 .UNSPECIFIED.);
#833=B_SPLINE_CURVE_WITH_KNOTS('',3,(#43946,#43947,#43948,#43949,#43950,
#43951,#43952,#43953,#43954,#43955,#43956,#43957,#43958,#43959,#43960,#43961,
#43962),.UNSPECIFIED.,.F.,.F.,(4,1,1,1,1,1,1,1,1,1,1,1,1,1,4),(223.053078404875,
223.311305258235,223.810013551621,224.308721845008,224.807430138395,225.306138431781,
225.804846725168,226.303555018555,226.802263311941,227.300971605328,227.799679898714,
228.298388192101,228.797096485488,229.295804778874,229.336263712055),
 .UNSPECIFIED.);
#834=B_SPLINE_CURVE_WITH_KNOTS('',3,(#43963,#43964,#43965,#43966,#43967,
#43968,#43969,#43970,#43971,#43972,#43973,#43974,#43975,#43976,#43977,#43978),
 .UNSPECIFIED.,.F.,.F.,(4,1,1,1,1,1,1,1,1,1,1,1,1,4),(223.053078404875,
223.357719195775,223.856427489162,224.355135782548,224.853844075935,225.352552369322,
225.851260662708,226.349968956095,226.848677249481,227.347385542868,227.846093836255,
228.344802129641,228.843510423028,229.336263712055),.UNSPECIFIED.);
#835=B_SPLINE_CURVE_WITH_KNOTS('',3,(#43983,#43984,#43985,#43986,#43987,
#43988,#43989,#43990,#43991,#43992,#43993,#43994,#43995,#43996,#43997,#43998,
#43999),.UNSPECIFIED.,.F.,.F.,(4,1,1,1,1,1,1,1,1,1,1,1,1,1,4),(216.769893097696,
216.828097444209,217.326805737595,217.825514030982,218.324222324369,218.822930617755,
219.321638911142,219.820347204529,220.319055497915,220.817763791302,221.316472084688,
221.815180378075,222.313888671462,222.812596964848,223.053078404875),
 .UNSPECIFIED.);
#836=B_SPLINE_CURVE_WITH_KNOTS('',3,(#44000,#44001,#44002,#44003,#44004,
#44005,#44006,#44007,#44008,#44009,#44010,#44011,#44012,#44013,#44014,#44015,
#44016),.UNSPECIFIED.,.F.,.F.,(4,1,1,1,1,1,1,1,1,1,1,1,1,1,4),(216.769893097696,
216.874511381749,217.373219675136,217.871927968522,218.370636261909,218.869344555295,
219.368052848682,219.866761142069,220.365469435455,220.864177728842,221.362886022229,
221.861594315615,222.360302609002,222.859010902388,223.053078404875),
 .UNSPECIFIED.);
#837=B_SPLINE_CURVE_WITH_KNOTS('',3,(#44021,#44022,#44023,#44024,#44025,
#44026,#44027,#44028,#44029,#44030,#44031,#44032,#44033,#44034,#44035,#44036),
 .UNSPECIFIED.,.F.,.F.,(4,1,1,1,1,1,1,1,1,1,1,1,1,4),(210.486707790516,
210.843597923569,211.342306216956,211.841014510343,212.339722803729,212.838431097116,
213.337139390502,213.835847683889,214.334555977276,214.833264270662,215.331972564049,
215.830680857436,216.329389150822,216.769893097696),.UNSPECIFIED.);
#838=B_SPLINE_CURVE_WITH_KNOTS('',3,(#44037,#44038,#44039,#44040,#44041,
#44042,#44043,#44044,#44045,#44046,#44047,#44048,#44049,#44050,#44051,#44052),
 .UNSPECIFIED.,.F.,.F.,(4,1,1,1,1,1,1,1,1,1,1,1,1,4),(210.486707790516,
210.89001186111,211.388720154496,211.887428447883,212.386136741269,212.884845034656,
213.383553328043,213.882261621429,214.380969914816,214.879678208203,215.378386501589,
215.877094794976,216.375803088362,216.769893097696),.UNSPECIFIED.);
#839=B_SPLINE_CURVE_WITH_KNOTS('',3,(#44057,#44058,#44059,#44060,#44061,
#44062,#44063,#44064,#44065,#44066,#44067,#44068,#44069,#44070,#44071,#44072,
#44073),.UNSPECIFIED.,.F.,.F.,(4,1,1,1,1,1,1,1,1,1,1,1,1,1,4),(204.203522483337,
204.360390109543,204.85909840293,205.357806696317,205.856514989703,206.35522328309,
206.853931576476,207.352639869863,207.85134816325,208.350056456636,208.848764750023,
209.347473043409,209.846181336796,210.344889630183,210.486707790516),
 .UNSPECIFIED.);
#840=B_SPLINE_CURVE_WITH_KNOTS('',3,(#44074,#44075,#44076,#44077,#44078,
#44079,#44080,#44081,#44082,#44083,#44084,#44085,#44086,#44087,#44088,#44089,
#44090),.UNSPECIFIED.,.F.,.F.,(4,1,1,1,1,1,1,1,1,1,1,1,1,1,4),(204.203522483337,
204.406804047084,204.90551234047,205.404220633857,205.902928927243,206.40163722063,
206.900345514017,207.399053807403,207.89776210079,208.396470394177,208.895178687563,
209.39388698095,209.892595274336,210.391303567723,210.486707790516),
 .UNSPECIFIED.);
#841=B_SPLINE_CURVE_WITH_KNOTS('',3,(#44095,#44096,#44097,#44098,#44099,
#44100,#44101,#44102,#44103,#44104,#44105,#44106,#44107,#44108,#44109,#44110),
 .UNSPECIFIED.,.F.,.F.,(4,1,1,1,1,1,1,1,1,1,1,1,1,4),(197.920337176157,
198.375890588904,198.87459888229,199.373307175677,199.872015469064,200.37072376245,
200.869432055837,201.368140349224,201.86684864261,202.365556935997,202.864265229383,
203.36297352277,203.861681816157,204.203522483337),.UNSPECIFIED.);
#842=B_SPLINE_CURVE_WITH_KNOTS('',3,(#44111,#44112,#44113,#44114,#44115,
#44116,#44117,#44118,#44119,#44120,#44121,#44122,#44123,#44124,#44125,#44126,
#44127),.UNSPECIFIED.,.F.,.F.,(4,1,1,1,1,1,1,1,1,1,1,1,1,1,4),(197.920337176157,
197.923596233057,198.422304526444,198.921012819831,199.419721113217,199.918429406604,
200.417137699991,200.915845993377,201.414554286764,201.91326258015,202.411970873537,
202.910679166924,203.40938746031,203.908095753697,204.203522483337),
 .UNSPECIFIED.);
#843=B_SPLINE_CURVE_WITH_KNOTS('',3,(#44132,#44133,#44134,#44135,#44136,
#44137,#44138,#44139,#44140,#44141,#44142,#44143,#44144,#44145,#44146,#44147,
#44148),.UNSPECIFIED.,.F.,.F.,(4,1,1,1,1,1,1,1,1,1,1,1,1,1,4),(191.637151868978,
191.892682774878,192.391391068264,192.890099361651,193.388807655038,193.887515948424,
194.386224241811,194.884932535198,195.383640828584,195.882349121971,196.381057415357,
196.879765708744,197.378474002131,197.877182295517,197.920337176157),
 .UNSPECIFIED.);
#844=B_SPLINE_CURVE_WITH_KNOTS('',3,(#44149,#44150,#44151,#44152,#44153,
#44154,#44155,#44156,#44157,#44158,#44159,#44160,#44161,#44162,#44163,#44164),
 .UNSPECIFIED.,.F.,.F.,(4,1,1,1,1,1,1,1,1,1,1,1,1,4),(191.637151868978,
191.939096712418,192.437805005805,192.936513299191,193.435221592578,193.933929885965,
194.432638179351,194.931346472738,195.430054766124,195.928763059511,196.427471352898,
196.926179646284,197.424887939671,197.920337176157),.UNSPECIFIED.);
#845=B_SPLINE_CURVE_WITH_KNOTS('',3,(#44169,#44170,#44171,#44172,#44173,
#44174,#44175,#44176,#44177,#44178,#44179,#44180,#44181,#44182,#44183,#44184,
#44185),.UNSPECIFIED.,.F.,.F.,(4,1,1,1,1,1,1,1,1,1,1,1,1,1,4),(185.353966561798,
185.409474960852,185.908183254238,186.406891547625,186.905599841012,187.404308134398,
187.903016427785,188.401724721171,188.900433014558,189.399141307945,189.897849601331,
190.396557894718,190.895266188105,191.393974481491,191.637151868978),
 .UNSPECIFIED.);
#846=B_SPLINE_CURVE_WITH_KNOTS('',3,(#44186,#44187,#44188,#44189,#44190,
#44191,#44192,#44193,#44194,#44195,#44196,#44197,#44198,#44199,#44200,#44201,
#44202),.UNSPECIFIED.,.F.,.F.,(4,1,1,1,1,1,1,1,1,1,1,1,1,1,4),(185.353966561798,
185.455888898392,185.954597191779,186.453305485165,186.952013778552,187.450722071938,
187.949430365325,188.448138658712,188.946846952098,189.445555245485,189.944263538872,
190.442971832258,190.941680125645,191.440388419031,191.637151868978),
 .UNSPECIFIED.);
#847=B_SPLINE_CURVE_WITH_KNOTS('',3,(#44207,#44208,#44209,#44210,#44211,
#44212,#44213,#44214,#44215,#44216,#44217,#44218,#44219,#44220,#44221,#44222),
 .UNSPECIFIED.,.F.,.F.,(4,1,1,1,1,1,1,1,1,1,1,1,1,4),(179.070781254618,
179.424975440212,179.923683733599,180.422392026986,180.921100320372,181.419808613759,
181.918516907145,182.417225200532,182.915933493919,183.414641787305,183.913350080692,
184.412058374079,184.910766667465,185.353966561798),.UNSPECIFIED.);
#848=B_SPLINE_CURVE_WITH_KNOTS('',3,(#44223,#44224,#44225,#44226,#44227,
#44228,#44229,#44230,#44231,#44232,#44233,#44234,#44235,#44236,#44237,#44238),
 .UNSPECIFIED.,.F.,.F.,(4,1,1,1,1,1,1,1,1,1,1,1,1,4),(179.070781254618,
179.471389377753,179.970097671139,180.468805964526,180.967514257912,181.466222551299,
181.964930844686,182.463639138072,182.962347431459,183.461055724845,183.959764018232,
184.458472311619,184.957180605005,185.353966561798),.UNSPECIFIED.);
#849=B_SPLINE_CURVE_WITH_KNOTS('',3,(#44243,#44244,#44245,#44246,#44247,
#44248,#44249,#44250,#44251,#44252,#44253,#44254,#44255,#44256,#44257,#44258,
#44259),.UNSPECIFIED.,.F.,.F.,(4,1,1,1,1,1,1,1,1,1,1,1,1,1,4),(172.787595947439,
172.941767626186,173.440475919573,173.93918421296,174.437892506346,174.936600799733,
175.435309093119,175.934017386506,176.432725679893,176.931433973279,177.430142266666,
177.928850560052,178.427558853439,178.926267146826,179.070781254618),
 .UNSPECIFIED.);
#850=B_SPLINE_CURVE_WITH_KNOTS('',3,(#44260,#44261,#44262,#44263,#44264,
#44265,#44266,#44267,#44268,#44269,#44270,#44271,#44272,#44273,#44274,#44275,
#44276),.UNSPECIFIED.,.F.,.F.,(4,1,1,1,1,1,1,1,1,1,1,1,1,1,4),(172.787595947439,
172.988181563726,173.486889857113,173.9855981505,174.484306443886,174.983014737273,
175.48172303066,175.980431324046,176.479139617433,176.977847910819,177.476556204206,
177.975264497593,178.473972790979,178.972681084366,179.070781254618),
 .UNSPECIFIED.);
#851=B_SPLINE_CURVE_WITH_KNOTS('',3,(#44281,#44282,#44283,#44284,#44285,
#44286,#44287,#44288,#44289,#44290,#44291,#44292,#44293,#44294,#44295,#44296),
 .UNSPECIFIED.,.F.,.F.,(4,1,1,1,1,1,1,1,1,1,1,1,1,4),(166.504410640259,
166.957268105547,167.455976398933,167.95468469232,168.453392985707,168.952101279093,
169.45080957248,169.949517865867,170.448226159253,170.94693445264,171.445642746026,
171.944351039413,172.4430593328,172.787595947439),.UNSPECIFIED.);
#852=B_SPLINE_CURVE_WITH_KNOTS('',3,(#44297,#44298,#44299,#44300,#44301,
#44302,#44303,#44304,#44305,#44306,#44307,#44308,#44309,#44310,#44311,#44312,
#44313),.UNSPECIFIED.,.F.,.F.,(4,1,1,1,1,1,1,1,1,1,1,1,1,1,4),(166.504410640259,
166.5049737497,167.003682043087,167.502390336474,168.00109862986,168.499806923247,
168.998515216634,169.49722351002,169.995931803407,170.494640096793,170.99334839018,
171.492056683567,171.990764976953,172.48947327034,172.787595947439),
 .UNSPECIFIED.);
#853=B_SPLINE_CURVE_WITH_KNOTS('',3,(#44318,#44319,#44320,#44321,#44322,
#44323,#44324,#44325,#44326,#44327,#44328,#44329,#44330,#44331,#44332,#44333,
#44334),.UNSPECIFIED.,.F.,.F.,(4,1,1,1,1,1,1,1,1,1,1,1,1,1,4),(160.22122533308,
160.474060291521,160.972768584907,161.471476878294,161.970185171681,162.468893465067,
162.967601758454,163.466310051841,163.965018345227,164.463726638614,164.962434932,
165.461143225387,165.959851518774,166.45855981216,166.504410640259),
 .UNSPECIFIED.);
#854=B_SPLINE_CURVE_WITH_KNOTS('',3,(#44335,#44336,#44337,#44338,#44339,
#44340,#44341,#44342,#44343,#44344,#44345,#44346,#44347,#44348,#44349,#44350),
 .UNSPECIFIED.,.F.,.F.,(4,1,1,1,1,1,1,1,1,1,1,1,1,4),(160.22122533308,160.520474229061,
161.019182522448,161.517890815834,162.016599109221,162.515307402608,163.014015695994,
163.512723989381,164.011432282767,164.510140576154,165.008848869541,165.507557162927,
166.006265456314,166.504410640259),.UNSPECIFIED.);
#855=B_SPLINE_CURVE_WITH_KNOTS('',3,(#44355,#44356,#44357,#44358,#44359,
#44360,#44361,#44362,#44363,#44364,#44365,#44366,#44367,#44368,#44369,#44370,
#44371),.UNSPECIFIED.,.F.,.F.,(4,1,1,1,1,1,1,1,1,1,1,1,1,1,4),(153.9380400259,
153.990852477495,154.489560770881,154.988269064268,155.486977357655,155.985685651041,
156.484393944428,156.983102237814,157.481810531201,157.980518824588,158.479227117974,
158.977935411361,159.476643704748,159.975351998134,160.22122533308),
 .UNSPECIFIED.);
#856=B_SPLINE_CURVE_WITH_KNOTS('',3,(#44372,#44373,#44374,#44375,#44376,
#44377,#44378,#44379,#44380,#44381,#44382,#44383,#44384,#44385,#44386,#44387,
#44388),.UNSPECIFIED.,.F.,.F.,(4,1,1,1,1,1,1,1,1,1,1,1,1,1,4),(153.9380400259,
154.037266415035,154.535974708422,155.034683001808,155.533391295195,156.032099588581,
156.530807881968,157.029516175355,157.528224468741,158.026932762128,158.525641055515,
159.024349348901,159.523057642288,160.021765935674,160.22122533308),
 .UNSPECIFIED.);
#857=B_SPLINE_CURVE_WITH_KNOTS('',3,(#44393,#44394,#44395,#44396,#44397,
#44398,#44399,#44400,#44401,#44402,#44403,#44404,#44405,#44406,#44407,#44408),
 .UNSPECIFIED.,.F.,.F.,(4,1,1,1,1,1,1,1,1,1,1,1,1,4),(147.654854718721,
148.006352956855,148.505061250242,149.003769543629,149.502477837015,150.001186130402,
150.499894423788,150.998602717175,151.497311010562,151.996019303948,152.494727597335,
152.993435890721,153.492144184108,153.9380400259),.UNSPECIFIED.);
#858=B_SPLINE_CURVE_WITH_KNOTS('',3,(#44409,#44410,#44411,#44412,#44413,
#44414,#44415,#44416,#44417,#44418,#44419,#44420,#44421,#44422,#44423,#44424),
 .UNSPECIFIED.,.F.,.F.,(4,1,1,1,1,1,1,1,1,1,1,1,1,4),(147.654854718721,
148.052766894396,148.551475187782,149.050183481169,149.548891774555,150.047600067942,
150.546308361329,151.045016654715,151.543724948102,152.042433241488,152.541141534875,
153.039849828262,153.538558121648,153.9380400259),.UNSPECIFIED.);
#859=B_SPLINE_CURVE_WITH_KNOTS('',3,(#44429,#44430,#44431,#44432,#44433,
#44434,#44435,#44436,#44437,#44438,#44439,#44440,#44441),.UNSPECIFIED.,
 .F.,.F.,(4,1,1,1,1,1,1,1,1,1,4),(141.371669411541,141.523145142829,142.520561729602,
143.517978316376,144.515394903149,145.512811489922,146.011519783309,146.510228076695,
147.008936370082,147.507644663469,147.654854718721),.UNSPECIFIED.);
#860=B_SPLINE_CURVE_WITH_KNOTS('',3,(#44442,#44443,#44444,#44445,#44446,
#44447,#44448,#44449,#44450,#44451),.UNSPECIFIED.,.F.,.F.,(4,1,1,1,1,1,
1,4),(141.371669411541,142.068267373756,143.065683960529,144.063100547303,
145.060517134076,146.057933720849,147.055350307622,147.654854718721),
 .UNSPECIFIED.);
#861=B_SPLINE_CURVE_WITH_KNOTS('',3,(#44456,#44457,#44458,#44459,#44460,
#44461,#44462,#44463,#44464,#44465),.UNSPECIFIED.,.F.,.F.,(4,1,1,1,1,1,
1,4),(135.088484104362,135.53864562219,136.536062208963,137.533478795736,
138.53089538251,139.528311969283,140.525728556056,141.371669411541),
 .UNSPECIFIED.);
#862=B_SPLINE_CURVE_WITH_KNOTS('',3,(#44466,#44467,#44468,#44469,#44470,
#44471,#44472,#44473,#44474,#44475),.UNSPECIFIED.,.F.,.F.,(4,1,1,1,1,1,
1,4),(135.088484104362,136.083767853117,137.08118443989,138.078601026663,
139.076017613436,140.07343420021,141.070850786983,141.371669411541),
 .UNSPECIFIED.);
#863=B_SPLINE_CURVE_WITH_KNOTS('',3,(#44480,#44481,#44482,#44483,#44484,
#44485,#44486,#44487,#44488,#44489,#44490,#44491,#44492),.UNSPECIFIED.,
 .F.,.F.,(4,1,1,1,1,1,1,1,1,1,4),(128.805298797182,129.055437808164,129.55414610155,
130.052854394937,130.551562688324,131.05027098171,131.548979275097,132.54639586187,
133.543812448643,134.541229035417,135.088484104362),.UNSPECIFIED.);
#864=B_SPLINE_CURVE_WITH_KNOTS('',3,(#44493,#44494,#44495,#44496,#44497,
#44498,#44499,#44500,#44501,#44502,#44503,#44504,#44505,#44506,#44507,#44508),
 .UNSPECIFIED.,.F.,.F.,(4,1,1,1,1,1,1,1,1,1,1,1,1,4),(128.805298797182,
129.101851745704,129.600560039091,130.099268332477,130.597976625864,131.09668491925,
131.595393212637,132.094101506024,132.59280979941,133.091518092797,133.590226386184,
134.08893467957,135.086351266343,135.088484104362),.UNSPECIFIED.);
#865=B_SPLINE_CURVE_WITH_KNOTS('',3,(#44513,#44514,#44515,#44516,#44517,
#44518,#44519,#44520,#44521,#44522,#44523,#44524,#44525,#44526,#44527,#44528,
#44529),.UNSPECIFIED.,.F.,.F.,(4,1,1,1,1,1,1,1,1,1,1,1,1,1,4),(122.522113490002,
122.572229994138,123.070938287524,123.569646580911,124.068354874298,124.567063167684,
125.065771461071,125.564479754457,126.063188047844,126.561896341231,127.060604634617,
127.559312928004,128.058021221391,128.556729514777,128.805298797182),
 .UNSPECIFIED.);
#866=B_SPLINE_CURVE_WITH_KNOTS('',3,(#44530,#44531,#44532,#44533,#44534,
#44535,#44536,#44537,#44538,#44539,#44540,#44541,#44542,#44543,#44544,#44545,
#44546),.UNSPECIFIED.,.F.,.F.,(4,1,1,1,1,1,1,1,1,1,1,1,1,1,4),(122.522113490002,
122.618643931678,123.117352225065,123.616060518451,124.114768811838,124.613477105224,
125.112185398611,125.610893691998,126.109601985384,126.608310278771,127.107018572158,
127.605726865544,128.104435158931,128.603143452317,128.805298797182),
 .UNSPECIFIED.);
#867=B_SPLINE_CURVE_WITH_KNOTS('',3,(#44551,#44552,#44553,#44554,#44555,
#44556,#44557,#44558,#44559,#44560,#44561,#44562,#44563,#44564,#44565,#44566),
 .UNSPECIFIED.,.F.,.F.,(4,1,1,1,1,1,1,1,1,1,1,1,1,4),(116.238928182823,
116.587730473498,117.086438766885,117.585147060271,118.083855353658,118.582563647045,
119.081271940431,119.579980233818,120.078688527205,120.577396820591,121.076105113978,
121.574813407364,122.073521700751,122.522113490002),.UNSPECIFIED.);
#868=B_SPLINE_CURVE_WITH_KNOTS('',3,(#44567,#44568,#44569,#44570,#44571,
#44572,#44573,#44574,#44575,#44576,#44577,#44578,#44579,#44580,#44581,#44582),
 .UNSPECIFIED.,.F.,.F.,(4,1,1,1,1,1,1,1,1,1,1,1,1,4),(116.238928182823,
116.634144411039,117.132852704425,117.631560997812,118.130269291198,118.628977584585,
119.127685877972,119.626394171358,120.125102464745,120.623810758131,121.122519051518,
121.621227344905,122.119935638291,122.522113490002),.UNSPECIFIED.);
#869=B_SPLINE_CURVE_WITH_KNOTS('',3,(#44587,#44588,#44589,#44590,#44591,
#44592,#44593,#44594,#44595,#44596,#44597,#44598,#44599,#44600,#44601,#44602,
#44603),.UNSPECIFIED.,.F.,.F.,(4,1,1,1,1,1,1,1,1,1,1,1,1,1,4),(109.955742875643,
110.104522659472,110.603230952859,111.101939246245,111.600647539632,112.099355833019,
112.598064126405,113.096772419792,113.595480713179,114.094189006565,114.592897299952,
115.091605593338,115.590313886725,116.089022180112,116.238928182823),
 .UNSPECIFIED.);
#870=B_SPLINE_CURVE_WITH_KNOTS('',3,(#44604,#44605,#44606,#44607,#44608,
#44609,#44610,#44611,#44612,#44613,#44614,#44615,#44616,#44617,#44618,#44619,
#44620),.UNSPECIFIED.,.F.,.F.,(4,1,1,1,1,1,1,1,1,1,1,1,1,1,4),(109.955742875643,
110.150936597012,110.649644890399,111.148353183786,111.647061477172,112.145769770559,
112.644478063946,113.143186357332,113.641894650719,114.140602944105,114.639311237492,
115.138019530879,115.636727824265,116.135436117652,116.238928182823),
 .UNSPECIFIED.);
#871=B_SPLINE_CURVE_WITH_KNOTS('',3,(#44625,#44626,#44627,#44628,#44629,
#44630,#44631,#44632,#44633,#44634,#44635,#44636,#44637,#44638,#44639,#44640),
 .UNSPECIFIED.,.F.,.F.,(4,1,1,1,1,1,1,1,1,1,1,1,1,4),(103.672557568464,
104.120023138833,104.618731432219,105.117439725606,105.616148018993,106.114856312379,
106.613564605766,107.112272899152,107.610981192539,108.109689485926,108.608397779312,
109.107106072699,109.605814366086,109.955742875643),.UNSPECIFIED.);
#872=B_SPLINE_CURVE_WITH_KNOTS('',3,(#44641,#44642,#44643,#44644,#44645,
#44646,#44647,#44648,#44649,#44650,#44651,#44652,#44653,#44654,#44655,#44656),
 .UNSPECIFIED.,.F.,.F.,(4,1,1,1,1,1,1,1,1,1,1,1,1,4),(103.672557568464,
104.166437076373,104.66514536976,105.163853663146,105.662561956533,106.161270249919,
106.659978543306,107.158686836693,107.657395130079,108.156103423466,108.654811716853,
109.153520010239,109.652228303626,109.955742875643),.UNSPECIFIED.);
#873=B_SPLINE_CURVE_WITH_KNOTS('',3,(#44661,#44662,#44663,#44664,#44665,
#44666,#44667,#44668,#44669,#44670,#44671,#44672,#44673,#44674,#44675,#44676,
#44677),.UNSPECIFIED.,.F.,.F.,(4,1,1,1,1,1,1,1,1,1,1,1,1,1,4),(97.389372261284,
97.6368153248067,98.1355236181933,98.63423191158,99.1329402049666,99.6316484983532,
100.13035679174,100.629065085126,101.127773378513,101.6264816719,102.125189965286,
102.623898258673,103.12260655206,103.621314845446,103.672557568464),
 .UNSPECIFIED.);
#874=B_SPLINE_CURVE_WITH_KNOTS('',3,(#44678,#44679,#44680,#44681,#44682,
#44683,#44684,#44685,#44686,#44687,#44688,#44689,#44690,#44691,#44692,#44693,
#44694),.UNSPECIFIED.,.F.,.F.,(4,1,1,1,1,1,1,1,1,1,1,1,1,1,4),(97.389372261284,
97.683229262347,98.1819375557336,98.6806458491202,99.1793541425068,99.6780624358935,
100.17677072928,100.675479022667,101.174187316053,101.67289560944,102.171603902827,
102.670312196213,103.1690204896,103.667728782986,103.672557568464),
 .UNSPECIFIED.);
#875=B_SPLINE_CURVE_WITH_KNOTS('',3,(#44699,#44700,#44701,#44702,#44703,
#44704,#44705,#44706,#44707,#44708,#44709,#44710,#44711,#44712,#44713,#44714,
#44715),.UNSPECIFIED.,.F.,.F.,(4,1,1,1,1,1,1,1,1,1,1,1,1,1,4),(91.1061869541044,
91.1536075107807,91.6523158041673,92.1510240975539,92.6497323909405,93.1484406843271,
93.6471489777138,94.1458572711004,94.644565564487,95.1432738578736,95.6419821512603,
96.1406904446469,96.6393987380335,97.1381070314201,97.389372261284),
 .UNSPECIFIED.);
#876=B_SPLINE_CURVE_WITH_KNOTS('',3,(#44716,#44717,#44718,#44719,#44720,
#44721,#44722,#44723,#44724,#44725,#44726,#44727,#44728,#44729,#44730,#44731,
#44732),.UNSPECIFIED.,.F.,.F.,(4,1,1,1,1,1,1,1,1,1,1,1,1,1,4),(91.1061869541044,
91.2000214483209,91.6987297417075,92.1974380350942,92.6961463284808,93.1948546218674,
93.693562915254,94.1922712086406,94.6909795020272,95.1896877954139,95.6883960888005,
96.1871043821871,96.6858126755737,97.1845209689603,97.389372261284),
 .UNSPECIFIED.);
#877=B_SPLINE_CURVE_WITH_KNOTS('',3,(#44737,#44738,#44739,#44740,#44741,
#44742,#44743,#44744,#44745,#44746,#44747,#44748,#44749,#44750,#44751,#44752),
 .UNSPECIFIED.,.F.,.F.,(4,1,1,1,1,1,1,1,1,1,1,1,1,4),(84.8230016469248,
85.1691079901412,85.6678162835279,86.1665245769145,86.6652328703011,87.1639411636877,
87.6626494570743,88.161357750461,88.6600660438476,89.1587743372342,89.6574826306208,
90.1561909240074,90.654899217394,91.1061869541044),.UNSPECIFIED.);
#878=B_SPLINE_CURVE_WITH_KNOTS('',3,(#44753,#44754,#44755,#44756,#44757,
#44758,#44759,#44760,#44761,#44762,#44763,#44764,#44765,#44766,#44767,#44768),
 .UNSPECIFIED.,.F.,.F.,(4,1,1,1,1,1,1,1,1,1,1,1,1,4),(84.8230016469248,
85.2155219276815,85.7142302210681,86.2129385144547,86.7116468078413,87.2103551012279,
87.7090633946146,88.2077716880012,88.7064799813878,89.2051882747744,89.703896568161,
90.2026048615477,90.7013131549343,91.1061869541044),.UNSPECIFIED.);
#879=B_SPLINE_CURVE_WITH_KNOTS('',3,(#44773,#44774,#44775,#44776,#44777,
#44778,#44779,#44780,#44781,#44782,#44783,#44784,#44785,#44786,#44787,#44788,
#44789),.UNSPECIFIED.,.F.,.F.,(4,1,1,1,1,1,1,1,1,1,1,1,1,1,4),(78.5398163397452,
78.6859001761152,79.1846084695018,79.6833167628884,80.1820250562751,80.6807333496617,
81.1794416430483,81.6781499364349,82.1768582298215,82.6755665232081,83.1742748165948,
83.6729831099814,84.171691403368,84.6703996967546,84.8230016469248),
 .UNSPECIFIED.);
#880=B_SPLINE_CURVE_WITH_KNOTS('',3,(#44790,#44791,#44792,#44793,#44794,
#44795,#44796,#44797,#44798,#44799,#44800,#44801,#44802,#44803,#44804,#44805,
#44806),.UNSPECIFIED.,.F.,.F.,(4,1,1,1,1,1,1,1,1,1,1,1,1,1,4),(78.5398163397452,
78.7323141136554,79.231022407042,79.7297307004287,80.2284389938153,80.7271472872019,
81.2258555805885,81.7245638739751,82.2232721673618,82.7219804607484,83.220688754135,
83.7193970475216,84.2181053409082,84.7168136342949,84.8230016469248),
 .UNSPECIFIED.);
#881=B_SPLINE_CURVE_WITH_KNOTS('',3,(#44811,#44812,#44813,#44814,#44815,
#44816,#44817,#44818,#44819,#44820,#44821,#44822,#44823,#44824,#44825,#44826),
 .UNSPECIFIED.,.F.,.F.,(4,1,1,1,1,1,1,1,1,1,1,1,1,4),(72.2566310325657,
72.7014006554758,73.2001089488624,73.698817242249,74.1975255356356,74.6962338290222,
75.1949421224089,75.6936504157955,76.1923587091821,76.6910670025687,77.1897752959553,
77.6884835893419,78.1871918827286,78.5398163397452),.UNSPECIFIED.);
#882=B_SPLINE_CURVE_WITH_KNOTS('',3,(#44827,#44828,#44829,#44830,#44831,
#44832,#44833,#44834,#44835,#44836,#44837,#44838,#44839,#44840,#44841,#44842),
 .UNSPECIFIED.,.F.,.F.,(4,1,1,1,1,1,1,1,1,1,1,1,1,4),(72.2566310325657,
72.747814593016,73.2465228864026,73.7452311797892,74.2439394731758,74.7426477665625,
75.2413560599491,75.7400643533357,76.2387726467223,76.7374809401089,77.2361892334956,
77.7348975268822,78.2336058202688,78.5398163397452),.UNSPECIFIED.);
#883=B_SPLINE_CURVE_WITH_KNOTS('',3,(#44847,#44848,#44849,#44850,#44851,
#44852,#44853,#44854,#44855,#44856,#44857,#44858,#44859,#44860,#44861,#44862,
#44863),.UNSPECIFIED.,.F.,.F.,(4,1,1,1,1,1,1,1,1,1,1,1,1,1,4),(65.973445725386,
66.2181928414497,66.7169011348363,67.2156094282229,67.7143177216096,68.2130260149962,
68.7117343083828,69.2104426017694,69.709150895156,70.2078591885427,70.7065674819293,
71.2052757753159,71.7039840687025,72.2026923620891,72.2566310325657),
 .UNSPECIFIED.);
#884=B_SPLINE_CURVE_WITH_KNOTS('',3,(#44864,#44865,#44866,#44867,#44868,
#44869,#44870,#44871,#44872,#44873,#44874,#44875,#44876,#44877,#44878,#44879,
#44880),.UNSPECIFIED.,.F.,.F.,(4,1,1,1,1,1,1,1,1,1,1,1,1,1,4),(65.973445725386,
66.2646067789899,66.7633150723765,67.2620233657632,67.7607316591498,68.2594399525364,
68.758148245923,69.2568565393096,69.7555648326963,70.2542731260829,70.7529814194695,
71.2516897128561,71.7503980062427,72.2491062996294,72.2566310325657),
 .UNSPECIFIED.);
#885=B_SPLINE_CURVE_WITH_KNOTS('',3,(#44885,#44886,#44887,#44888,#44889,
#44890,#44891,#44892,#44893,#44894,#44895,#44896,#44897,#44898,#44899,#44900,
#44901),.UNSPECIFIED.,.F.,.F.,(4,1,1,1,1,1,1,1,1,1,1,1,1,1,4),(59.6902604182065,
59.7349850274237,60.2336933208103,60.7324016141969,61.2311099075835,61.7298182009701,
62.2285264943567,62.7272347877434,63.22594308113,63.7246513745166,64.2233596679032,
64.7220679612898,65.2207762546765,65.7194845480631,65.973445725386),
 .UNSPECIFIED.);
#886=B_SPLINE_CURVE_WITH_KNOTS('',3,(#44902,#44903,#44904,#44905,#44906,
#44907,#44908,#44909,#44910,#44911,#44912,#44913,#44914,#44915,#44916,#44917,
#44918),.UNSPECIFIED.,.F.,.F.,(4,1,1,1,1,1,1,1,1,1,1,1,1,1,4),(59.6902604182065,
59.7813989649639,60.2801072583505,60.7788155517371,61.2775238451237,61.7762321385104,
62.274940431897,62.7736487252836,63.2723570186702,63.7710653120568,64.2697736054434,
64.7684818988301,65.2671901922167,65.7658984856033,65.973445725386),
 .UNSPECIFIED.);
#887=B_SPLINE_CURVE_WITH_KNOTS('',3,(#44923,#44924,#44925,#44926,#44927,
#44928,#44929,#44930,#44931,#44932,#44933,#44934,#44935,#44936,#44937,#44938),
 .UNSPECIFIED.,.F.,.F.,(4,1,1,1,1,1,1,1,1,1,1,1,1,4),(53.4070751110269,
53.7504855067842,54.2491938001708,54.7479020935575,55.2466103869441,55.7453186803307,
56.2440269737173,56.7427352671039,57.2414435604906,57.7401518538772,58.2388601472638,
58.7375684406504,59.236276734037,59.6902604182065),.UNSPECIFIED.);
#888=B_SPLINE_CURVE_WITH_KNOTS('',3,(#44939,#44940,#44941,#44942,#44943,
#44944,#44945,#44946,#44947,#44948,#44949,#44950,#44951,#44952,#44953,#44954),
 .UNSPECIFIED.,.F.,.F.,(4,1,1,1,1,1,1,1,1,1,1,1,1,4),(53.4070751110269,
53.7968994443244,54.2956077377111,54.7943160310977,55.2930243244843,55.7917326178709,
56.2904409112575,56.7891492046442,57.2878574980308,57.7865657914174,58.285274084804,
58.7839823781906,59.2826906715772,59.6902604182065),.UNSPECIFIED.);
#889=B_SPLINE_CURVE_WITH_KNOTS('',3,(#44959,#44960,#44961,#44962,#44963,
#44964,#44965,#44966,#44967,#44968,#44969,#44970,#44971,#44972,#44973,#44974,
#44975),.UNSPECIFIED.,.F.,.F.,(4,1,1,1,1,1,1,1,1,1,1,1,1,1,4),(47.1238898038473,
47.2672776927582,47.7659859861448,48.2646942795314,48.763402572918,49.2621108663046,
49.7608191596913,50.2595274530779,50.7582357464645,51.2569440398511,51.7556523332377,
52.2543606266244,52.753068920011,53.2517772133976,53.4070751110269),
 .UNSPECIFIED.);
#890=B_SPLINE_CURVE_WITH_KNOTS('',3,(#44976,#44977,#44978,#44979,#44980,
#44981,#44982,#44983,#44984,#44985,#44986,#44987,#44988,#44989,#44990,#44991,
#44992),.UNSPECIFIED.,.F.,.F.,(4,1,1,1,1,1,1,1,1,1,1,1,1,1,4),(47.1238898038473,
47.3136916302984,47.812399923685,48.3111082170716,48.8098165104582,49.3085248038449,
49.8072330972315,50.3059413906181,50.8046496840047,51.3033579773913,51.802066270778,
52.3007745641646,52.7994828575512,53.2981911509378,53.4070751110269),
 .UNSPECIFIED.);
#891=B_SPLINE_CURVE_WITH_KNOTS('',3,(#44997,#44998,#44999,#45000,#45001,
#45002,#45003,#45004,#45005,#45006,#45007,#45008,#45009,#45010,#45011,#45012),
 .UNSPECIFIED.,.F.,.F.,(4,1,1,1,1,1,1,1,1,1,1,1,1,4),(40.8407044966677,
41.2827781721187,41.7814864655054,42.280194758892,42.7789030522786,43.2776113456652,
43.7763196390518,44.2750279324384,44.7737362258251,45.2724445192117,45.7711528125983,
46.2698611059849,46.7685693993716,47.1238898038473),.UNSPECIFIED.);
#892=B_SPLINE_CURVE_WITH_KNOTS('',3,(#45013,#45014,#45015,#45016,#45017,
#45018,#45019,#45020,#45021,#45022,#45023,#45024,#45025,#45026,#45027,#45028),
 .UNSPECIFIED.,.F.,.F.,(4,1,1,1,1,1,1,1,1,1,1,1,1,4),(40.8407044966677,
41.3291921096589,41.8279004030456,42.3266086964322,42.8253169898188,43.3240252832054,
43.822733576592,44.3214418699787,44.8201501633653,45.3188584567519,45.8175667501385,
46.3162750435251,46.8149833369118,47.1238898038473),.UNSPECIFIED.);
#893=B_SPLINE_CURVE_WITH_KNOTS('',3,(#45033,#45034,#45035,#45036,#45037,
#45038,#45039,#45040,#45041,#45042,#45043,#45044,#45045,#45046,#45047,#45048,
#45049),.UNSPECIFIED.,.F.,.F.,(4,1,1,1,1,1,1,1,1,1,1,1,1,1,4),(34.5575191894881,
34.7995703580927,35.2982786514793,35.7969869448659,36.2956952382525,36.7944035316392,
37.2931118250258,37.7918201184124,38.290528411799,38.7892367051856,39.2879449985723,
39.7866532919589,40.2853615853455,40.7840698787321,40.8407044966677),
 .UNSPECIFIED.);
#894=B_SPLINE_CURVE_WITH_KNOTS('',3,(#45050,#45051,#45052,#45053,#45054,
#45055,#45056,#45057,#45058,#45059,#45060,#45061,#45062,#45063,#45064,#45065,
#45066),.UNSPECIFIED.,.F.,.F.,(4,1,1,1,1,1,1,1,1,1,1,1,1,1,4),(34.5575191894881,
34.8459842956329,35.3446925890195,35.8434008824061,36.3421091757927,36.8408174691794,
37.339525762566,37.8382340559526,38.3369423493392,38.8356506427259,39.3343589361125,
39.8330672294991,40.3317755228857,40.8304838162723,40.8407044966677),
 .UNSPECIFIED.);
#895=B_SPLINE_CURVE_WITH_KNOTS('',3,(#45071,#45072,#45073,#45074,#45075,
#45076,#45077,#45078,#45079,#45080,#45081,#45082,#45083,#45084,#45085,#45086,
#45087),.UNSPECIFIED.,.F.,.F.,(4,1,1,1,1,1,1,1,1,1,1,1,1,1,4),(28.2743338823085,
28.3163625440666,28.8150708374532,29.3137791308399,29.8124874242265,30.3111957176131,
30.8099040109997,31.3086123043863,31.807320597773,32.3060288911596,32.8047371845462,
33.3034454779328,33.8021537713194,34.3008620647061,34.5575191894881),
 .UNSPECIFIED.);
#896=B_SPLINE_CURVE_WITH_KNOTS('',3,(#45088,#45089,#45090,#45091,#45092,
#45093,#45094,#45095,#45096,#45097,#45098,#45099,#45100,#45101,#45102,#45103,
#45104),.UNSPECIFIED.,.F.,.F.,(4,1,1,1,1,1,1,1,1,1,1,1,1,1,4),(28.2743338823085,
28.3627764816068,28.8614847749935,29.3601930683801,29.8589013617667,30.3576096551533,
30.8563179485399,31.3550262419266,31.8537345353132,32.3524428286998,32.8511511220864,
33.349859415473,33.8485677088597,34.3472760022463,34.5575191894881),
 .UNSPECIFIED.);
#897=B_SPLINE_CURVE_WITH_KNOTS('',3,(#45109,#45110,#45111,#45112,#45113,
#45114,#45115,#45116,#45117,#45118,#45119,#45120,#45121,#45122,#45123,#45124),
 .UNSPECIFIED.,.F.,.F.,(4,1,1,1,1,1,1,1,1,1,1,1,1,4),(21.9911485751289,
22.3318630234272,22.8305713168138,23.3292796102004,23.8279879035871,24.3266961969737,
24.8254044903603,25.3241127837469,25.8228210771335,26.3215293705201,26.8202376639068,
27.3189459572934,27.81765425068,28.2743338823085),.UNSPECIFIED.);
#898=B_SPLINE_CURVE_WITH_KNOTS('',3,(#45125,#45126,#45127,#45128,#45129,
#45130,#45131,#45132,#45133,#45134,#45135,#45136,#45137,#45138,#45139,#45140),
 .UNSPECIFIED.,.F.,.F.,(4,1,1,1,1,1,1,1,1,1,1,1,1,4),(21.9911485751289,
22.3782769609674,22.876985254354,23.3756935477406,23.8744018411273,24.3731101345139,
24.8718184279005,25.3705267212871,25.8692350146737,26.3679433080604,26.866651601447,
27.3653598948336,27.8640681882202,28.2743338823085),.UNSPECIFIED.);
#899=B_SPLINE_CURVE_WITH_KNOTS('',3,(#45146,#45147,#45148,#45149,#45150,
#45151),.UNSPECIFIED.,.F.,.F.,(4,1,1,4),(14.3989442667815,14.8976525601681,
15.3963608535547,15.7079632679493),.UNSPECIFIED.);
#900=B_SPLINE_CURVE_WITH_KNOTS('',3,(#45154,#45155,#45156,#45157,#45158,
#45159,#45160),.UNSPECIFIED.,.F.,.F.,(4,1,1,1,4),(13.8753896155274,14.3525303292413,
14.8512386226279,15.3499469160145,15.7079632679493),.UNSPECIFIED.);
#901=B_SPLINE_CURVE_WITH_KNOTS('',3,(#45162,#45163,#45164,#45165,#45166,
#45167,#45168,#45169,#45170,#45171,#45172,#45173,#45174,#45175,#45176,#45177,
#45178,#45179,#45180,#45181,#45182,#45183,#45184,#45185,#45186,#45187,#45188,
#45189,#45190,#45191,#45192,#45193,#45194,#45195,#45196,#45197,#45198,#45199,
#45200,#45201,#45202,#45203,#45204,#45205,#45206,#45207,#45208,#45209,#45210,
#45211,#45212,#45213,#45214,#45215,#45216,#45217,#45218,#45219,#45220,#45221,
#45222,#45223,#45224,#45225,#45226,#45227,#45228,#45229,#45230,#45231,#45232,
#45233,#45234,#45235,#45236,#45237,#45238,#45239,#45240,#45241,#45242,#45243,
#45244,#45245,#45246,#45247,#45248,#45249,#45250,#45251,#45252,#45253,#45254,
#45255,#45256,#45257,#45258,#45259,#45260,#45261,#45262,#45263,#45264,#45265,
#45266,#45267),.UNSPECIFIED.,.F.,.F.,(4,3,3,3,3,3,3,3,3,3,3,3,3,3,3,3,3,
3,3,3,3,3,3,3,3,3,3,3,3,3,3,3,3,3,3,4),(-0.972375876542216,-0.931557379101648,
-0.890218542042487,-0.869392708916521,-0.861677237530619,-0.819813801882793,
-0.781167845425456,-0.769475619651221,-0.760546025724648,-0.754411794373795,
-0.74252188896812,-0.700976733031894,-0.65877791376378,-0.616292150528589,
-0.588572673703484,-0.579879678859757,-0.574332463387633,-0.531223905437004,
-0.505414243228169,-0.462559206201071,-0.419378313085458,-0.399643768345371,
-0.391565714980685,-0.383732909736738,-0.340135839018284,-0.296193649678293,
-0.261501955164762,-0.217668074296404,-0.204748702273309,-0.197210738162037,
-0.192140598791969,-0.1468449795757,-0.102253744983165,-0.0566059334550285,
-0.0109581219268922,0.),.UNSPECIFIED.);
#902=B_SPLINE_CURVE_WITH_KNOTS('',3,(#45268,#45269,#45270,#45271,#45272,
#45273,#45274,#45275,#45276,#45277,#45278,#45279,#45280,#45281,#45282,#45283,
#45284,#45285,#45286,#45287,#45288,#45289,#45290,#45291,#45292,#45293,#45294,
#45295,#45296,#45297,#45298,#45299,#45300,#45301,#45302,#45303,#45304,#45305,
#45306,#45307,#45308,#45309,#45310,#45311,#45312,#45313,#45314,#45315,#45316,
#45317,#45318,#45319,#45320,#45321,#45322,#45323,#45324,#45325,#45326,#45327,
#45328,#45329,#45330,#45331,#45332,#45333,#45334,#45335,#45336,#45337,#45338,
#45339,#45340,#45341,#45342,#45343,#45344,#45345,#45346,#45347,#45348,#45349,
#45350,#45351,#45352,#45353,#45354,#45355,#45356,#45357,#45358,#45359,#45360,
#45361,#45362,#45363,#45364,#45365,#45366,#45367,#45368,#45369,#45370),
 .UNSPECIFIED.,.F.,.F.,(4,3,3,3,3,3,3,3,3,3,3,3,3,3,3,3,3,3,3,3,3,3,3,3,
3,3,3,3,3,3,3,3,3,3,4),(-0.970006587573357,-0.925489021709122,-0.880831606117785,
-0.860106336836479,-0.852213503588024,-0.808023919462815,-0.764142093829507,
-0.741127929891385,-0.732995659095006,-0.720260268196198,-0.676886083169421,
-0.633189091074775,-0.58989356338977,-0.561603730397805,-0.548456029491321,
-0.542926374323804,-0.500045602531121,-0.476734231421911,-0.433752968122039,
-0.390893110149348,-0.372012672166435,-0.363955407652349,-0.356648068723258,
-0.314412819484753,-0.272458136815843,-0.239849606286048,-0.197688110523089,
-0.185715478561588,-0.179206252930902,-0.173732780061183,-0.132200928727762,
-0.0907046629355285,-0.0499294541163457,-0.00977294415302305,0.),
 .UNSPECIFIED.);
#903=B_SPLINE_CURVE_WITH_KNOTS('',3,(#45372,#45373,#45374,#45375,#45376,
#45377,#45378,#45379,#45380,#45381,#45382,#45383,#45384,#45385,#45386,#45387,
#45388),.UNSPECIFIED.,.F.,.F.,(4,1,1,1,1,1,1,1,1,1,1,1,1,1,4),(15.7079632679493,
15.8486552094011,16.3473635027878,16.8460717961744,17.344780089561,17.8434883829476,
18.3421966763342,18.8409049697209,19.3396132631075,19.8383215564941,20.3370298498807,
20.8357381432673,21.334446436654,21.8331547300406,21.9911485751289),
 .UNSPECIFIED.);
#904=B_SPLINE_CURVE_WITH_KNOTS('',3,(#45389,#45390,#45391,#45392,#45393,
#45394,#45395,#45396,#45397,#45398,#45399,#45400,#45401,#45402,#45403,#45404,
#45405),.UNSPECIFIED.,.F.,.F.,(4,1,1,1,1,1,1,1,1,1,1,1,1,1,4),(15.7079632679493,
15.8950691469414,16.393777440328,16.8924857337146,17.3911940271012,17.8899023204878,
18.3886106138744,18.8873189072611,19.3860272006477,19.8847354940343,20.3834437874209,
20.8821520808075,21.3808603741942,21.8795686675808,21.9911485751289),
 .UNSPECIFIED.);
#905=B_SPLINE_CURVE_WITH_KNOTS('',3,(#47394,#47395,#47396,#47397,#47398,
#47399,#47400,#47401,#47402,#47403,#47404,#47405,#47406,#47407,#47408,#47409,
#47410,#47411,#47412,#47413,#47414,#47415,#47416,#47417,#47418,#47419,#47420,
#47421,#47422,#47423,#47424,#47425,#47426,#47427,#47428,#47429,#47430,#47431,
#47432,#47433,#47434,#47435,#47436,#47437,#47438,#47439,#47440,#47441,#47442,
#47443,#47444,#47445,#47446,#47447,#47448,#47449,#47450,#47451,#47452,#47453,
#47454,#47455,#47456,#47457,#47458,#47459,#47460,#47461,#47462,#47463,#47464,
#47465,#47466,#47467,#47468,#47469,#47470,#47471,#47472,#47473,#47474,#47475,
#47476,#47477,#47478,#47479,#47480,#47481,#47482,#47483,#47484,#47485,#47486,
#47487,#47488,#47489,#47490,#47491,#47492,#47493,#47494,#47495,#47496,#47497,
#47498,#47499),.UNSPECIFIED.,.F.,.F.,(4,3,3,3,3,3,3,3,3,3,3,3,3,3,3,3,3,
3,3,3,3,3,3,3,3,3,3,3,3,3,3,3,3,3,3,4),(0.,0.040424976116911,0.081552621191953,
0.123116379418818,0.164484386952486,0.177258002125512,0.182429040513286,
0.224585211732574,0.229750939065668,0.271485437391992,0.313663426362065,
0.351832391899687,0.358992185792409,0.364434825962351,0.407093430609824,
0.45008484068709,0.466339288512555,0.509174339674324,0.534227886997736,
0.545013114142881,0.550666578456316,0.593964513128218,0.637614398405316,
0.68114810979745,0.709602718261623,0.725600523556765,0.736529828545389,
0.743509911151027,0.78723345430323,0.830193673824424,0.848440235266336,
0.858098500020291,0.902703209392534,0.947246712359152,0.959074332388006,
0.970006587573436),.UNSPECIFIED.);
#906=B_SPLINE_CURVE_WITH_KNOTS('',3,(#47500,#47501,#47502,#47503,#47504,
#47505,#47506,#47507,#47508,#47509,#47510,#47511,#47512,#47513,#47514,#47515,
#47516,#47517,#47518,#47519,#47520,#47521,#47522,#47523,#47524,#47525,#47526,
#47527,#47528,#47529,#47530,#47531,#47532,#47533,#47534,#47535,#47536,#47537,
#47538,#47539,#47540,#47541,#47542),.UNSPECIFIED.,.F.,.F.,(4,3,3,3,3,3,
3,3,3,3,3,3,3,3,4),(-10.1321597128207,-9.97416586773239,-9.47545757434577,
-8.97674928095915,-8.47804098757253,-7.97933269418591,-7.48062440079929,
-6.98191610741267,-6.48320781402605,-5.98449952063943,-5.48579122725281,
-4.98708293386619,-4.48837464047957,-3.98966634709295,-3.84897440564115),
 .UNSPECIFIED.);
#907=B_SPLINE_CURVE_WITH_KNOTS('',3,(#49531,#49532,#49533,#49534,#49535,
#49536,#49537,#49538,#49539,#49540,#49541,#49542,#49543,#49544,#49545,#49546,
#49547,#49548,#49549,#49550,#49551,#49552,#49553,#49554,#49555,#49556,#49557,
#49558,#49559,#49560,#49561,#49562,#49563,#49564,#49565,#49566,#49567,#49568,
#49569,#49570),.UNSPECIFIED.,.F.,.F.,(4,3,3,3,3,3,3,3,3,3,3,3,3,4),(7.59220430834772,
7.97933269418591,8.47804098757253,8.97674928095915,9.47545757434577,9.97416586773239,
10.472874161119,10.9715824545056,11.4702907478922,11.9689990412789,12.4677073346655,
12.9664156280521,13.4651239214387,13.8753896155273),.UNSPECIFIED.);
#908=B_SPLINE_CURVE_WITH_KNOTS('',3,(#49571,#49572,#49573,#49574,#49575,
#49576,#49577,#49578,#49579,#49580,#49581,#49582,#49583,#49584,#49585,#49586,
#49587,#49588,#49589,#49590,#49591,#49592,#49593,#49594,#49595,#49596,#49597,
#49598,#49599,#49600,#49601,#49602,#49603,#49604,#49605,#49606,#49607,#49608,
#49609,#49610,#49611,#49612,#49613,#49614,#49615,#49616,#49617,#49618,#49619,
#49620,#49621,#49622,#49623,#49624,#49625,#49626,#49627,#49628,#49629,#49630,
#49631,#49632,#49633,#49634,#49635,#49636,#49637,#49638,#49639,#49640,#49641,
#49642,#49643,#49644,#49645,#49646,#49647,#49648,#49649,#49650,#49651,#49652,
#49653,#49654,#49655,#49656,#49657,#49658,#49659,#49660,#49661,#49662,#49663,
#49664,#49665,#49666,#49667,#49668,#49669,#49670,#49671,#49672,#49673,#49674,
#49675,#49676),.UNSPECIFIED.,.F.,.F.,(4,3,3,3,3,3,3,3,3,3,3,3,3,3,3,3,3,
3,3,3,3,3,3,3,3,3,3,3,3,3,3,3,3,3,3,4),(0.,0.0441576970943254,0.088758491595093,
0.133154322886181,0.177017836347152,0.193697049021019,0.19965188566726,
0.243475277581627,0.250795014009384,0.294669452308725,0.338569619728244,
0.37767568962022,0.38721824859893,0.393275053464473,0.436458598855563,0.479377262352089,
0.494993899296151,0.538189921814499,0.562468636762688,0.572092716170009,
0.579226787127647,0.621711263641225,0.664154373258728,0.70594102510778,
0.732419641400012,0.748330061688134,0.757222465646011,0.763401818269173,
0.80529293424602,0.844615778238015,0.861173358979439,0.871344162504664,
0.912748133225373,0.953576775379504,0.962584310214001,0.972375876542313),
 .UNSPECIFIED.);
#909=B_SPLINE_CURVE_WITH_KNOTS('',3,(#49682,#49683,#49684,#49685,#49686,
#49687,#49688,#49689,#49690,#49691,#49692,#49693,#49694,#49695,#49696,#49697,
#49698,#49699,#49700,#49701,#49702,#49703,#49704,#49705,#49706,#49707,#49708,
#49709,#49710,#49711,#49712,#49713,#49714,#49715,#49716,#49717,#49718,#49719,
#49720,#49721,#49722,#49723,#49724,#49725,#49726,#49727,#49728,#49729,#49730,
#49731,#49732,#49733,#49734,#49735,#49736,#49737,#49738,#49739,#49740,#49741,
#49742,#49743,#49744,#49745,#49746,#49747,#49748,#49749,#49750,#49751,#49752,
#49753,#49754,#49755,#49756,#49757,#49758,#49759,#49760,#49761,#49762,#49763,
#49764,#49765,#49766,#49767,#49768,#49769,#49770,#49771,#49772,#49773,#49774,
#49775,#49776,#49777,#49778,#49779,#49780,#49781,#49782,#49783,#49784),
 .UNSPECIFIED.,.F.,.F.,(4,3,3,3,3,3,3,3,3,3,3,3,3,3,3,3,3,3,3,3,3,3,3,3,
3,3,3,3,3,3,3,3,3,3,4),(-0.972375876542414,-0.931565253728255,-0.890231005347033,
-0.869571408761885,-0.861266125665987,-0.819404433385386,-0.781321836236662,
-0.759040374121689,-0.752934683192443,-0.743239239087938,-0.701695078724687,
-0.659497058703992,-0.617009387497169,-0.589480672868744,-0.57644702705794,
-0.5714452780933,-0.528325351620324,-0.506894528983471,-0.464054318866617,
-0.420876860304666,-0.401240281040809,-0.388666227231065,-0.383537192824514,
-0.339939758883143,-0.295998103578765,-0.263784226193809,-0.219954566467475,
-0.204809517925579,-0.197308554950036,-0.192241015625869,-0.147699202975487,
-0.103111401264591,-0.0585925831444644,-0.0140737650243382,0.),
 .UNSPECIFIED.);
#910=B_SPLINE_CURVE_WITH_KNOTS('',3,(#49785,#49786,#49787,#49788,#49789,
#49790,#49791,#49792,#49793,#49794,#49795,#49796,#49797,#49798,#49799,#49800,
#49801,#49802,#49803,#49804,#49805,#49806,#49807,#49808,#49809,#49810,#49811,
#49812,#49813,#49814,#49815,#49816,#49817,#49818,#49819,#49820,#49821,#49822,
#49823,#49824,#49825,#49826,#49827,#49828,#49829,#49830,#49831,#49832,#49833,
#49834,#49835,#49836,#49837,#49838,#49839,#49840,#49841,#49842,#49843,#49844,
#49845,#49846,#49847,#49848,#49849,#49850,#49851,#49852,#49853,#49854,#49855,
#49856,#49857,#49858,#49859,#49860,#49861,#49862,#49863,#49864,#49865,#49866,
#49867,#49868,#49869,#49870,#49871,#49872,#49873,#49874,#49875,#49876,#49877,
#49878,#49879,#49880,#49881,#49882,#49883,#49884,#49885,#49886,#49887),
 .UNSPECIFIED.,.F.,.F.,(4,3,3,3,3,3,3,3,3,3,3,3,3,3,3,3,3,3,3,3,3,3,3,3,
3,3,3,3,3,3,3,3,3,3,4),(-0.97000658757332,-0.925493326456513,-0.880835987444213,
-0.86024842639854,-0.852333874766883,-0.808142692209155,-0.764580356539862,
-0.742334794451242,-0.733010188832428,-0.721018020870569,-0.677646574841948,
-0.633950360266973,-0.590648734368262,-0.562539792613221,-0.550153753024242,
-0.542978093928587,-0.50009796533363,-0.478212967348099,-0.435235450336473,
-0.392367497022972,-0.373572235159268,-0.361228651726056,-0.355614322341834,
-0.313378921971217,-0.271427075980555,-0.242005402113342,-0.199831951142943,
-0.186315085816715,-0.179649707786883,-0.174232916759018,-0.132703725702247,
-0.0912075908119877,-0.0504161836307489,-0.0125558726020182,0.),
 .UNSPECIFIED.);
#911=B_SPLINE_CURVE_WITH_KNOTS('',3,(#49889,#49890,#49891,#49892,#49893,
#49894,#49895,#49896,#49897,#49898,#49899,#49900,#49901,#49902,#49903,#49904,
#49905),.UNSPECIFIED.,.F.,.F.,(4,1,1,1,1,1,1,1,1,1,1,1,1,1,4),(15.707963267949,
15.8363896981257,16.3335648026029,16.8307399070801,17.3279150115573,17.8250901160345,
18.3222652205117,18.8194403249889,19.3166154294662,19.8137905339434,20.3109656384206,
20.8081407428978,21.305315847375,21.8024909518522,21.9911485751286),
 .UNSPECIFIED.);
#912=B_SPLINE_CURVE_WITH_KNOTS('',3,(#49906,#49907,#49908,#49909,#49910,
#49911,#49912,#49913,#49914,#49915,#49916,#49917,#49918,#49919,#49920,#49921,
#49922),.UNSPECIFIED.,.F.,.F.,(4,1,1,1,1,1,1,1,1,1,1,1,1,1,4),(15.707963267949,
15.8904695802126,16.3876446846898,16.884819789167,17.3819948936443,17.8791699981215,
18.3763451025987,18.8735202070759,19.3706953115531,19.8678704160303,20.3650455205075,
20.8622206249848,21.359395729462,21.8565708339392,21.9911485751286),
 .UNSPECIFIED.);
#913=B_SPLINE_CURVE_WITH_KNOTS('',3,(#51215,#51216,#51217,#51218,#51219,
#51220,#51221,#51222,#51223,#51224,#51225,#51226,#51227,#51228,#51229,#51230,
#51231,#51232,#51233,#51234,#51235,#51236,#51237,#51238,#51239,#51240,#51241,
#51242,#51243,#51244,#51245,#51246,#51247,#51248,#51249,#51250,#51251,#51252,
#51253,#51254,#51255,#51256,#51257,#51258,#51259,#51260,#51261,#51262,#51263,
#51264,#51265,#51266,#51267,#51268,#51269,#51270,#51271,#51272,#51273,#51274,
#51275,#51276,#51277,#51278,#51279,#51280,#51281,#51282,#51283,#51284,#51285,
#51286,#51287,#51288,#51289,#51290,#51291,#51292,#51293,#51294,#51295,#51296,
#51297,#51298,#51299,#51300,#51301,#51302,#51303,#51304,#51305,#51306,#51307,
#51308,#51309,#51310,#51311,#51312,#51313,#51314,#51315,#51316,#51317,#51318,
#51319,#51320),.UNSPECIFIED.,.F.,.F.,(4,3,3,3,3,3,3,3,3,3,3,3,3,3,3,3,3,
3,3,3,3,3,3,3,3,3,3,3,3,3,3,3,3,3,3,4),(0.,0.0404156030320338,0.0815364170314856,
0.123099442202208,0.164471164259153,0.177417333177223,0.182894508577368,
0.225046885757466,0.229033692090525,0.270767557602402,0.312945697761686,
0.350924838148176,0.357993918766748,0.363846074008531,0.406502560546029,
0.449493818503337,0.464862259307647,0.507689818261392,0.532644888553053,
0.54674918267878,0.552366866895522,0.595682545020243,0.639338821245014,
0.682868010841828,0.707330380594682,0.725816624679753,0.736955855775304,
0.74358314378864,0.787317407834192,0.829479796072424,0.846856648451819,
0.854114186312316,0.898699022066203,0.94326334774114,0.955966960787121,
0.97000658757331),.UNSPECIFIED.);
#914=B_SPLINE_CURVE_WITH_KNOTS('',3,(#51321,#51322,#51323,#51324,#51325,
#51326,#51327,#51328,#51329,#51330,#51331,#51332,#51333,#51334,#51335,#51336,
#51337,#51338,#51339,#51340,#51341,#51342,#51343,#51344,#51345,#51346,#51347,
#51348,#51349,#51350,#51351,#51352,#51353,#51354,#51355,#51356,#51357,#51358,
#51359,#51360,#51361,#51362,#51363),.UNSPECIFIED.,.F.,.F.,(4,3,3,3,3,3,
3,3,3,3,3,3,3,3,4),(-10.1321597128207,-9.94350208954429,-9.44632698506708,
-8.94915188058987,-8.45197677611265,-7.95480167163544,-7.45762656715822,
-6.96045146268101,-6.46327635820379,-5.96610125372657,-5.46892614924936,
-4.97175104477214,-4.47457594029493,-3.97740083581771,-3.848974405641),
 .UNSPECIFIED.);
#915=B_SPLINE_CURVE_WITH_KNOTS('',3,(#52656,#52657,#52658,#52659,#52660,
#52661,#52662,#52663,#52664,#52665,#52666,#52667,#52668,#52669,#52670,#52671,
#52672,#52673,#52674,#52675,#52676,#52677,#52678,#52679,#52680,#52681,#52682,
#52683,#52684,#52685,#52686,#52687,#52688,#52689,#52690,#52691,#52692,#52693,
#52694,#52695),.UNSPECIFIED.,.F.,.F.,(4,3,3,3,3,3,3,3,3,3,3,3,3,4),(7.59220430834767,
7.95480167163543,8.45197677611264,8.94915188058986,9.44632698506707,9.94350208954429,
10.4406771940215,10.9378522984987,11.4350274029759,11.9322025074531,12.4293776119304,
12.9265527164076,13.4237278208848,13.8753896155273),.UNSPECIFIED.);
#916=B_SPLINE_CURVE_WITH_KNOTS('',3,(#52696,#52697,#52698,#52699,#52700,
#52701,#52702,#52703,#52704,#52705,#52706,#52707,#52708,#52709,#52710,#52711,
#52712,#52713,#52714,#52715,#52716,#52717,#52718,#52719,#52720,#52721,#52722,
#52723,#52724,#52725,#52726,#52727,#52728,#52729,#52730,#52731,#52732,#52733,
#52734,#52735,#52736,#52737,#52738,#52739,#52740,#52741,#52742,#52743,#52744,
#52745,#52746,#52747,#52748,#52749,#52750,#52751,#52752,#52753,#52754,#52755,
#52756,#52757,#52758,#52759,#52760,#52761,#52762,#52763,#52764,#52765,#52766,
#52767,#52768,#52769,#52770,#52771,#52772,#52773,#52774,#52775,#52776,#52777,
#52778,#52779,#52780,#52781,#52782,#52783,#52784,#52785,#52786,#52787,#52788,
#52789,#52790,#52791,#52792,#52793,#52794,#52795,#52796,#52797,#52798,#52799,
#52800,#52801),.UNSPECIFIED.,.F.,.F.,(4,3,3,3,3,3,3,3,3,3,3,3,3,3,3,3,3,
3,3,3,3,3,3,3,3,3,3,3,3,3,3,3,3,3,3,4),(0.,0.044150773052086,0.0887487507111273,
0.133148741969068,0.177019043965151,0.193023436662248,0.199907412815446,
0.24373234733986,0.250033573379215,0.293906609053928,0.337808296166161,
0.376734021006827,0.385567082155686,0.391401994113249,0.434581851246655,
0.477513379513922,0.493511195528826,0.53671130462677,0.560905212030567,
0.574207000071321,0.579201605029167,0.62168463125547,0.664125603281933,
0.705919109414855,0.730262563857148,0.748325604460628,0.757394747707568,
0.762943677116111,0.804834492856293,0.843575066915537,0.859283154994003,
0.866889043776386,0.908311110283104,0.949189929713081,0.959796789093269,
0.972375876542504),.UNSPECIFIED.);
#2217=SHAPE_REPRESENTATION_RELATIONSHIP('SRR','None',#97611,#2236);
#2236=ADVANCED_BREP_SHAPE_REPRESENTATION('',(#2274),#97461);
#2255=STYLED_ITEM('',(#97718),#2274);
#2274=MANIFOLD_SOLID_BREP('Aluminum slotted profile',#21816);
#2316=FACE_BOUND('',#4035,.T.);
#2317=FACE_BOUND('',#4042,.T.);
#2318=FACE_BOUND('',#4046,.T.);
#2319=FACE_BOUND('',#4047,.T.);
#2320=FACE_BOUND('',#4048,.T.);
#2321=FACE_BOUND('',#4049,.T.);
#2322=FACE_BOUND('',#4050,.T.);
#2323=FACE_BOUND('',#4127,.T.);
#2324=FACE_BOUND('',#4128,.T.);
#2325=FACE_BOUND('',#4129,.T.);
#2326=FACE_BOUND('',#4130,.T.);
#2327=FACE_BOUND('',#4131,.T.);
#2417=PLANE('',#22440);
#2418=PLANE('',#22443);
#2419=PLANE('',#22445);
#2420=PLANE('',#22448);
#2421=PLANE('',#22453);
#2422=PLANE('',#22454);
#2423=PLANE('',#22496);
#2424=PLANE('',#22499);
#2425=PLANE('',#22502);
#2426=PLANE('',#22505);
#2427=PLANE('',#22510);
#2428=PLANE('',#22515);
#2429=PLANE('',#22520);
#2430=PLANE('',#22523);
#2431=PLANE('',#22526);
#2432=PLANE('',#22529);
#2433=PLANE('',#22534);
#2434=PLANE('',#22539);
#2435=PLANE('',#22544);
#2436=PLANE('',#22547);
#2437=PLANE('',#22550);
#2438=PLANE('',#22553);
#2439=PLANE('',#22558);
#2440=PLANE('',#22563);
#2441=PLANE('',#22568);
#2442=PLANE('',#22571);
#2443=PLANE('',#22574);
#2444=PLANE('',#22577);
#2445=PLANE('',#22582);
#2446=PLANE('',#22596);
#2447=PLANE('',#22597);
#2448=PLANE('',#22598);
#2449=PLANE('',#22599);
#2450=PLANE('',#22600);
#2451=PLANE('',#22601);
#2452=PLANE('',#22602);
#2453=PLANE('',#22603);
#2454=PLANE('',#22604);
#2455=PLANE('',#22605);
#2456=PLANE('',#22606);
#2457=PLANE('',#22607);
#2458=PLANE('',#22608);
#2717=FACE_OUTER_BOUND('',#3899,.T.);
#2718=FACE_OUTER_BOUND('',#3900,.T.);
#2719=FACE_OUTER_BOUND('',#3901,.T.);
#2720=FACE_OUTER_BOUND('',#3902,.T.);
#2721=FACE_OUTER_BOUND('',#3903,.T.);
#2722=FACE_OUTER_BOUND('',#3904,.T.);
#2723=FACE_OUTER_BOUND('',#3905,.T.);
#2724=FACE_OUTER_BOUND('',#3906,.T.);
#2725=FACE_OUTER_BOUND('',#3907,.T.);
#2726=FACE_OUTER_BOUND('',#3908,.T.);
#2727=FACE_OUTER_BOUND('',#3909,.T.);
#2728=FACE_OUTER_BOUND('',#3910,.T.);
#2729=FACE_OUTER_BOUND('',#3911,.T.);
#2730=FACE_OUTER_BOUND('',#3912,.T.);
#2731=FACE_OUTER_BOUND('',#3913,.T.);
#2732=FACE_OUTER_BOUND('',#3914,.T.);
#2733=FACE_OUTER_BOUND('',#3915,.T.);
#2734=FACE_OUTER_BOUND('',#3916,.T.);
#2735=FACE_OUTER_BOUND('',#3917,.T.);
#2736=FACE_OUTER_BOUND('',#3918,.T.);
#2737=FACE_OUTER_BOUND('',#3919,.T.);
#2738=FACE_OUTER_BOUND('',#3920,.T.);
#2739=FACE_OUTER_BOUND('',#3921,.T.);
#2740=FACE_OUTER_BOUND('',#3922,.T.);
#2741=FACE_OUTER_BOUND('',#3923,.T.);
#2742=FACE_OUTER_BOUND('',#3924,.T.);
#2743=FACE_OUTER_BOUND('',#3925,.T.);
#2744=FACE_OUTER_BOUND('',#3926,.T.);
#2745=FACE_OUTER_BOUND('',#3927,.T.);
#2746=FACE_OUTER_BOUND('',#3928,.T.);
#2747=FACE_OUTER_BOUND('',#3929,.T.);
#2748=FACE_OUTER_BOUND('',#3930,.T.);
#2749=FACE_OUTER_BOUND('',#3931,.T.);
#2750=FACE_OUTER_BOUND('',#3932,.T.);
#2751=FACE_OUTER_BOUND('',#3933,.T.);
#2752=FACE_OUTER_BOUND('',#3934,.T.);
#2753=FACE_OUTER_BOUND('',#3935,.T.);
#2754=FACE_OUTER_BOUND('',#3936,.T.);
#2755=FACE_OUTER_BOUND('',#3937,.T.);
#2756=FACE_OUTER_BOUND('',#3938,.T.);
#2757=FACE_OUTER_BOUND('',#3939,.T.);
#2758=FACE_OUTER_BOUND('',#3940,.T.);
#2759=FACE_OUTER_BOUND('',#3941,.T.);
#2760=FACE_OUTER_BOUND('',#3942,.T.);
#2761=FACE_OUTER_BOUND('',#3943,.T.);
#2762=FACE_OUTER_BOUND('',#3944,.T.);
#2763=FACE_OUTER_BOUND('',#3945,.T.);
#2764=FACE_OUTER_BOUND('',#3946,.T.);
#2765=FACE_OUTER_BOUND('',#3947,.T.);
#2766=FACE_OUTER_BOUND('',#3948,.T.);
#2767=FACE_OUTER_BOUND('',#3949,.T.);
#2768=FACE_OUTER_BOUND('',#3950,.T.);
#2769=FACE_OUTER_BOUND('',#3951,.T.);
#2770=FACE_OUTER_BOUND('',#3952,.T.);
#2771=FACE_OUTER_BOUND('',#3953,.T.);
#2772=FACE_OUTER_BOUND('',#3954,.T.);
#2773=FACE_OUTER_BOUND('',#3955,.T.);
#2774=FACE_OUTER_BOUND('',#3956,.T.);
#2775=FACE_OUTER_BOUND('',#3957,.T.);
#2776=FACE_OUTER_BOUND('',#3958,.T.);
#2777=FACE_OUTER_BOUND('',#3959,.T.);
#2778=FACE_OUTER_BOUND('',#3960,.T.);
#2779=FACE_OUTER_BOUND('',#3961,.T.);
#2780=FACE_OUTER_BOUND('',#3962,.T.);
#2781=FACE_OUTER_BOUND('',#3963,.T.);
#2782=FACE_OUTER_BOUND('',#3964,.T.);
#2783=FACE_OUTER_BOUND('',#3965,.T.);
#2784=FACE_OUTER_BOUND('',#3966,.T.);
#2785=FACE_OUTER_BOUND('',#3967,.T.);
#2786=FACE_OUTER_BOUND('',#3968,.T.);
#2787=FACE_OUTER_BOUND('',#3969,.T.);
#2788=FACE_OUTER_BOUND('',#3970,.T.);
#2789=FACE_OUTER_BOUND('',#3971,.T.);
#2790=FACE_OUTER_BOUND('',#3972,.T.);
#2791=FACE_OUTER_BOUND('',#3973,.T.);
#2792=FACE_OUTER_BOUND('',#3974,.T.);
#2793=FACE_OUTER_BOUND('',#3975,.T.);
#2794=FACE_OUTER_BOUND('',#3976,.T.);
#2795=FACE_OUTER_BOUND('',#3977,.T.);
#2796=FACE_OUTER_BOUND('',#3978,.T.);
#2797=FACE_OUTER_BOUND('',#3979,.T.);
#2798=FACE_OUTER_BOUND('',#3980,.T.);
#2799=FACE_OUTER_BOUND('',#3981,.T.);
#2800=FACE_OUTER_BOUND('',#3982,.T.);
#2801=FACE_OUTER_BOUND('',#3983,.T.);
#2802=FACE_OUTER_BOUND('',#3984,.T.);
#2803=FACE_OUTER_BOUND('',#3985,.T.);
#2804=FACE_OUTER_BOUND('',#3986,.T.);
#2805=FACE_OUTER_BOUND('',#3987,.T.);
#2806=FACE_OUTER_BOUND('',#3988,.T.);
#2807=FACE_OUTER_BOUND('',#3989,.T.);
#2808=FACE_OUTER_BOUND('',#3990,.T.);
#2809=FACE_OUTER_BOUND('',#3991,.T.);
#2810=FACE_OUTER_BOUND('',#3992,.T.);
#2811=FACE_OUTER_BOUND('',#3993,.T.);
#2812=FACE_OUTER_BOUND('',#3994,.T.);
#2813=FACE_OUTER_BOUND('',#3995,.T.);
#2814=FACE_OUTER_BOUND('',#3996,.T.);
#2815=FACE_OUTER_BOUND('',#3997,.T.);
#2816=FACE_OUTER_BOUND('',#3998,.T.);
#2817=FACE_OUTER_BOUND('',#3999,.T.);
#2818=FACE_OUTER_BOUND('',#4000,.T.);
#2819=FACE_OUTER_BOUND('',#4001,.T.);
#2820=FACE_OUTER_BOUND('',#4002,.T.);
#2821=FACE_OUTER_BOUND('',#4003,.T.);
#2822=FACE_OUTER_BOUND('',#4004,.T.);
#2823=FACE_OUTER_BOUND('',#4005,.T.);
#2824=FACE_OUTER_BOUND('',#4006,.T.);
#2825=FACE_OUTER_BOUND('',#4007,.T.);
#2826=FACE_OUTER_BOUND('',#4008,.T.);
#2827=FACE_OUTER_BOUND('',#4009,.T.);
#2828=FACE_OUTER_BOUND('',#4010,.T.);
#2829=FACE_OUTER_BOUND('',#4011,.T.);
#2830=FACE_OUTER_BOUND('',#4012,.T.);
#2831=FACE_OUTER_BOUND('',#4013,.T.);
#2832=FACE_OUTER_BOUND('',#4014,.T.);
#2833=FACE_OUTER_BOUND('',#4015,.T.);
#2834=FACE_OUTER_BOUND('',#4016,.T.);
#2835=FACE_OUTER_BOUND('',#4017,.T.);
#2836=FACE_OUTER_BOUND('',#4018,.T.);
#2837=FACE_OUTER_BOUND('',#4019,.T.);
#2838=FACE_OUTER_BOUND('',#4020,.T.);
#2839=FACE_OUTER_BOUND('',#4021,.T.);
#2840=FACE_OUTER_BOUND('',#4022,.T.);
#2841=FACE_OUTER_BOUND('',#4023,.T.);
#2842=FACE_OUTER_BOUND('',#4024,.T.);
#2843=FACE_OUTER_BOUND('',#4025,.T.);
#2844=FACE_OUTER_BOUND('',#4026,.T.);
#2845=FACE_OUTER_BOUND('',#4027,.T.);
#2846=FACE_OUTER_BOUND('',#4028,.T.);
#2847=FACE_OUTER_BOUND('',#4029,.T.);
#2848=FACE_OUTER_BOUND('',#4030,.T.);
#2849=FACE_OUTER_BOUND('',#4031,.T.);
#2850=FACE_OUTER_BOUND('',#4032,.T.);
#2851=FACE_OUTER_BOUND('',#4033,.T.);
#2852=FACE_OUTER_BOUND('',#4034,.T.);
#2853=FACE_OUTER_BOUND('',#4036,.T.);
#2854=FACE_OUTER_BOUND('',#4037,.T.);
#2855=FACE_OUTER_BOUND('',#4038,.T.);
#2856=FACE_OUTER_BOUND('',#4039,.T.);
#2857=FACE_OUTER_BOUND('',#4040,.T.);
#2858=FACE_OUTER_BOUND('',#4041,.T.);
#2859=FACE_OUTER_BOUND('',#4043,.T.);
#2860=FACE_OUTER_BOUND('',#4044,.T.);
#2861=FACE_OUTER_BOUND('',#4045,.T.);
#2862=FACE_OUTER_BOUND('',#4051,.T.);
#2863=FACE_OUTER_BOUND('',#4052,.T.);
#2864=FACE_OUTER_BOUND('',#4053,.T.);
#2865=FACE_OUTER_BOUND('',#4054,.T.);
#2866=FACE_OUTER_BOUND('',#4055,.T.);
#2867=FACE_OUTER_BOUND('',#4056,.T.);
#2868=FACE_OUTER_BOUND('',#4057,.T.);
#2869=FACE_OUTER_BOUND('',#4058,.T.);
#2870=FACE_OUTER_BOUND('',#4059,.T.);
#2871=FACE_OUTER_BOUND('',#4060,.T.);
#2872=FACE_OUTER_BOUND('',#4061,.T.);
#2873=FACE_OUTER_BOUND('',#4062,.T.);
#2874=FACE_OUTER_BOUND('',#4063,.T.);
#2875=FACE_OUTER_BOUND('',#4064,.T.);
#2876=FACE_OUTER_BOUND('',#4065,.T.);
#2877=FACE_OUTER_BOUND('',#4066,.T.);
#2878=FACE_OUTER_BOUND('',#4067,.T.);
#2879=FACE_OUTER_BOUND('',#4068,.T.);
#2880=FACE_OUTER_BOUND('',#4069,.T.);
#2881=FACE_OUTER_BOUND('',#4070,.T.);
#2882=FACE_OUTER_BOUND('',#4071,.T.);
#2883=FACE_OUTER_BOUND('',#4072,.T.);
#2884=FACE_OUTER_BOUND('',#4073,.T.);
#2885=FACE_OUTER_BOUND('',#4074,.T.);
#2886=FACE_OUTER_BOUND('',#4075,.T.);
#2887=FACE_OUTER_BOUND('',#4076,.T.);
#2888=FACE_OUTER_BOUND('',#4077,.T.);
#2889=FACE_OUTER_BOUND('',#4078,.T.);
#2890=FACE_OUTER_BOUND('',#4079,.T.);
#2891=FACE_OUTER_BOUND('',#4080,.T.);
#2892=FACE_OUTER_BOUND('',#4081,.T.);
#2893=FACE_OUTER_BOUND('',#4082,.T.);
#2894=FACE_OUTER_BOUND('',#4083,.T.);
#2895=FACE_OUTER_BOUND('',#4084,.T.);
#2896=FACE_OUTER_BOUND('',#4085,.T.);
#2897=FACE_OUTER_BOUND('',#4086,.T.);
#2898=FACE_OUTER_BOUND('',#4087,.T.);
#2899=FACE_OUTER_BOUND('',#4088,.T.);
#2900=FACE_OUTER_BOUND('',#4089,.T.);
#2901=FACE_OUTER_BOUND('',#4090,.T.);
#2902=FACE_OUTER_BOUND('',#4091,.T.);
#2903=FACE_OUTER_BOUND('',#4092,.T.);
#2904=FACE_OUTER_BOUND('',#4093,.T.);
#2905=FACE_OUTER_BOUND('',#4094,.T.);
#2906=FACE_OUTER_BOUND('',#4095,.T.);
#2907=FACE_OUTER_BOUND('',#4096,.T.);
#2908=FACE_OUTER_BOUND('',#4097,.T.);
#2909=FACE_OUTER_BOUND('',#4098,.T.);
#2910=FACE_OUTER_BOUND('',#4099,.T.);
#2911=FACE_OUTER_BOUND('',#4100,.T.);
#2912=FACE_OUTER_BOUND('',#4101,.T.);
#2913=FACE_OUTER_BOUND('',#4102,.T.);
#2914=FACE_OUTER_BOUND('',#4103,.T.);
#2915=FACE_OUTER_BOUND('',#4104,.T.);
#2916=FACE_OUTER_BOUND('',#4105,.T.);
#2917=FACE_OUTER_BOUND('',#4106,.T.);
#2918=FACE_OUTER_BOUND('',#4107,.T.);
#2919=FACE_OUTER_BOUND('',#4108,.T.);
#2920=FACE_OUTER_BOUND('',#4109,.T.);
#2921=FACE_OUTER_BOUND('',#4110,.T.);
#2922=FACE_OUTER_BOUND('',#4111,.T.);
#2923=FACE_OUTER_BOUND('',#4112,.T.);
#2924=FACE_OUTER_BOUND('',#4113,.T.);
#2925=FACE_OUTER_BOUND('',#4114,.T.);
#2926=FACE_OUTER_BOUND('',#4115,.T.);
#2927=FACE_OUTER_BOUND('',#4116,.T.);
#2928=FACE_OUTER_BOUND('',#4117,.T.);
#2929=FACE_OUTER_BOUND('',#4118,.T.);
#2930=FACE_OUTER_BOUND('',#4119,.T.);
#2931=FACE_OUTER_BOUND('',#4120,.T.);
#2932=FACE_OUTER_BOUND('',#4121,.T.);
#2933=FACE_OUTER_BOUND('',#4122,.T.);
#2934=FACE_OUTER_BOUND('',#4123,.T.);
#2935=FACE_OUTER_BOUND('',#4124,.T.);
#2936=FACE_OUTER_BOUND('',#4125,.T.);
#2937=FACE_OUTER_BOUND('',#4126,.T.);
#3899=EDGE_LOOP('',(#14120,#14121,#14122,#14123,#14124,#14125,#14126,#14127));
#3900=EDGE_LOOP('',(#14128,#14129,#14130,#14131));
#3901=EDGE_LOOP('',(#14132,#14133,#14134,#14135));
#3902=EDGE_LOOP('',(#14136,#14137,#14138,#14139));
#3903=EDGE_LOOP('',(#14140,#14141,#14142,#14143));
#3904=EDGE_LOOP('',(#14144,#14145,#14146,#14147));
#3905=EDGE_LOOP('',(#14148,#14149,#14150,#14151));
#3906=EDGE_LOOP('',(#14152,#14153,#14154,#14155));
#3907=EDGE_LOOP('',(#14156,#14157,#14158,#14159));
#3908=EDGE_LOOP('',(#14160,#14161,#14162,#14163));
#3909=EDGE_LOOP('',(#14164,#14165,#14166,#14167));
#3910=EDGE_LOOP('',(#14168,#14169,#14170,#14171));
#3911=EDGE_LOOP('',(#14172,#14173,#14174,#14175));
#3912=EDGE_LOOP('',(#14176,#14177,#14178,#14179));
#3913=EDGE_LOOP('',(#14180,#14181,#14182,#14183));
#3914=EDGE_LOOP('',(#14184,#14185,#14186,#14187));
#3915=EDGE_LOOP('',(#14188,#14189,#14190,#14191));
#3916=EDGE_LOOP('',(#14192,#14193,#14194,#14195));
#3917=EDGE_LOOP('',(#14196,#14197,#14198,#14199));
#3918=EDGE_LOOP('',(#14200,#14201,#14202,#14203));
#3919=EDGE_LOOP('',(#14204,#14205,#14206,#14207));
#3920=EDGE_LOOP('',(#14208,#14209,#14210,#14211));
#3921=EDGE_LOOP('',(#14212,#14213,#14214,#14215));
#3922=EDGE_LOOP('',(#14216,#14217,#14218,#14219));
#3923=EDGE_LOOP('',(#14220,#14221,#14222,#14223));
#3924=EDGE_LOOP('',(#14224,#14225,#14226,#14227));
#3925=EDGE_LOOP('',(#14228,#14229,#14230,#14231));
#3926=EDGE_LOOP('',(#14232,#14233,#14234,#14235));
#3927=EDGE_LOOP('',(#14236,#14237,#14238,#14239));
#3928=EDGE_LOOP('',(#14240,#14241,#14242,#14243));
#3929=EDGE_LOOP('',(#14244,#14245,#14246,#14247));
#3930=EDGE_LOOP('',(#14248,#14249,#14250,#14251));
#3931=EDGE_LOOP('',(#14252,#14253,#14254,#14255));
#3932=EDGE_LOOP('',(#14256,#14257,#14258,#14259));
#3933=EDGE_LOOP('',(#14260,#14261,#14262,#14263));
#3934=EDGE_LOOP('',(#14264,#14265,#14266,#14267));
#3935=EDGE_LOOP('',(#14268,#14269,#14270,#14271));
#3936=EDGE_LOOP('',(#14272,#14273,#14274,#14275));
#3937=EDGE_LOOP('',(#14276,#14277,#14278,#14279));
#3938=EDGE_LOOP('',(#14280,#14281,#14282,#14283));
#3939=EDGE_LOOP('',(#14284,#14285,#14286,#14287));
#3940=EDGE_LOOP('',(#14288,#14289,#14290,#14291));
#3941=EDGE_LOOP('',(#14292,#14293,#14294,#14295));
#3942=EDGE_LOOP('',(#14296,#14297,#14298,#14299));
#3943=EDGE_LOOP('',(#14300,#14301,#14302,#14303));
#3944=EDGE_LOOP('',(#14304,#14305,#14306,#14307));
#3945=EDGE_LOOP('',(#14308,#14309,#14310,#14311));
#3946=EDGE_LOOP('',(#14312,#14313,#14314,#14315));
#3947=EDGE_LOOP('',(#14316,#14317,#14318,#14319));
#3948=EDGE_LOOP('',(#14320,#14321,#14322,#14323));
#3949=EDGE_LOOP('',(#14324,#14325,#14326,#14327,#14328,#14329,#14330,#14331));
#3950=EDGE_LOOP('',(#14332,#14333,#14334,#14335));
#3951=EDGE_LOOP('',(#14336,#14337,#14338,#14339));
#3952=EDGE_LOOP('',(#14340,#14341,#14342,#14343));
#3953=EDGE_LOOP('',(#14344,#14345,#14346,#14347));
#3954=EDGE_LOOP('',(#14348,#14349,#14350,#14351));
#3955=EDGE_LOOP('',(#14352,#14353,#14354,#14355));
#3956=EDGE_LOOP('',(#14356,#14357,#14358,#14359));
#3957=EDGE_LOOP('',(#14360,#14361,#14362,#14363));
#3958=EDGE_LOOP('',(#14364,#14365,#14366,#14367));
#3959=EDGE_LOOP('',(#14368,#14369,#14370,#14371));
#3960=EDGE_LOOP('',(#14372,#14373,#14374,#14375));
#3961=EDGE_LOOP('',(#14376,#14377,#14378,#14379));
#3962=EDGE_LOOP('',(#14380,#14381,#14382,#14383));
#3963=EDGE_LOOP('',(#14384,#14385,#14386,#14387));
#3964=EDGE_LOOP('',(#14388,#14389,#14390,#14391));
#3965=EDGE_LOOP('',(#14392,#14393,#14394,#14395));
#3966=EDGE_LOOP('',(#14396,#14397,#14398,#14399));
#3967=EDGE_LOOP('',(#14400,#14401,#14402,#14403));
#3968=EDGE_LOOP('',(#14404,#14405,#14406,#14407));
#3969=EDGE_LOOP('',(#14408,#14409,#14410,#14411));
#3970=EDGE_LOOP('',(#14412,#14413,#14414,#14415));
#3971=EDGE_LOOP('',(#14416,#14417,#14418,#14419));
#3972=EDGE_LOOP('',(#14420,#14421,#14422,#14423));
#3973=EDGE_LOOP('',(#14424,#14425,#14426,#14427));
#3974=EDGE_LOOP('',(#14428,#14429,#14430,#14431));
#3975=EDGE_LOOP('',(#14432,#14433,#14434,#14435));
#3976=EDGE_LOOP('',(#14436,#14437,#14438,#14439));
#3977=EDGE_LOOP('',(#14440,#14441,#14442,#14443));
#3978=EDGE_LOOP('',(#14444,#14445,#14446,#14447));
#3979=EDGE_LOOP('',(#14448,#14449,#14450,#14451));
#3980=EDGE_LOOP('',(#14452,#14453,#14454,#14455));
#3981=EDGE_LOOP('',(#14456,#14457,#14458,#14459));
#3982=EDGE_LOOP('',(#14460,#14461,#14462,#14463));
#3983=EDGE_LOOP('',(#14464,#14465,#14466,#14467));
#3984=EDGE_LOOP('',(#14468,#14469,#14470,#14471));
#3985=EDGE_LOOP('',(#14472,#14473,#14474,#14475));
#3986=EDGE_LOOP('',(#14476,#14477,#14478,#14479));
#3987=EDGE_LOOP('',(#14480,#14481,#14482,#14483));
#3988=EDGE_LOOP('',(#14484,#14485,#14486,#14487));
#3989=EDGE_LOOP('',(#14488,#14489,#14490,#14491));
#3990=EDGE_LOOP('',(#14492,#14493,#14494,#14495));
#3991=EDGE_LOOP('',(#14496,#14497,#14498,#14499));
#3992=EDGE_LOOP('',(#14500,#14501,#14502,#14503));
#3993=EDGE_LOOP('',(#14504,#14505,#14506,#14507));
#3994=EDGE_LOOP('',(#14508,#14509,#14510,#14511));
#3995=EDGE_LOOP('',(#14512,#14513,#14514,#14515));
#3996=EDGE_LOOP('',(#14516,#14517,#14518,#14519));
#3997=EDGE_LOOP('',(#14520,#14521,#14522,#14523));
#3998=EDGE_LOOP('',(#14524,#14525,#14526,#14527));
#3999=EDGE_LOOP('',(#14528,#14529,#14530,#14531));
#4000=EDGE_LOOP('',(#14532,#14533,#14534,#14535));
#4001=EDGE_LOOP('',(#14536,#14537,#14538,#14539));
#4002=EDGE_LOOP('',(#14540,#14541,#14542,#14543));
#4003=EDGE_LOOP('',(#14544,#14545,#14546,#14547));
#4004=EDGE_LOOP('',(#14548,#14549,#14550,#14551));
#4005=EDGE_LOOP('',(#14552,#14553,#14554,#14555));
#4006=EDGE_LOOP('',(#14556,#14557,#14558,#14559));
#4007=EDGE_LOOP('',(#14560,#14561,#14562,#14563));
#4008=EDGE_LOOP('',(#14564,#14565,#14566,#14567));
#4009=EDGE_LOOP('',(#14568,#14569,#14570,#14571));
#4010=EDGE_LOOP('',(#14572,#14573,#14574,#14575));
#4011=EDGE_LOOP('',(#14576,#14577,#14578,#14579));
#4012=EDGE_LOOP('',(#14580,#14581,#14582,#14583));
#4013=EDGE_LOOP('',(#14584,#14585,#14586,#14587));
#4014=EDGE_LOOP('',(#14588,#14589,#14590,#14591));
#4015=EDGE_LOOP('',(#14592,#14593,#14594,#14595));
#4016=EDGE_LOOP('',(#14596,#14597,#14598,#14599));
#4017=EDGE_LOOP('',(#14600,#14601,#14602,#14603));
#4018=EDGE_LOOP('',(#14604,#14605,#14606,#14607));
#4019=EDGE_LOOP('',(#14608,#14609,#14610,#14611));
#4020=EDGE_LOOP('',(#14612,#14613,#14614,#14615));
#4021=EDGE_LOOP('',(#14616,#14617,#14618,#14619));
#4022=EDGE_LOOP('',(#14620,#14621,#14622,#14623));
#4023=EDGE_LOOP('',(#14624,#14625,#14626,#14627));
#4024=EDGE_LOOP('',(#14628,#14629,#14630,#14631));
#4025=EDGE_LOOP('',(#14632,#14633,#14634,#14635));
#4026=EDGE_LOOP('',(#14636,#14637,#14638,#14639));
#4027=EDGE_LOOP('',(#14640,#14641,#14642,#14643));
#4028=EDGE_LOOP('',(#14644,#14645,#14646,#14647));
#4029=EDGE_LOOP('',(#14648,#14649,#14650,#14651,#14652));
#4030=EDGE_LOOP('',(#14653,#14654,#14655,#14656));
#4031=EDGE_LOOP('',(#14657,#14658,#14659,#14660,#14661,#14662,#14663,#14664,
#14665,#14666,#14667,#14668,#14669,#14670,#14671,#14672,#14673,#14674,#14675,
#14676,#14677,#14678,#14679,#14680,#14681,#14682,#14683,#14684,#14685,#14686,
#14687,#14688,#14689,#14690,#14691,#14692,#14693,#14694,#14695,#14696,#14697,
#14698,#14699,#14700,#14701,#14702,#14703,#14704,#14705,#14706,#14707,#14708,
#14709,#14710,#14711,#14712,#14713,#14714,#14715,#14716,#14717,#14718,#14719,
#14720,#14721,#14722,#14723,#14724,#14725,#14726,#14727,#14728,#14729,#14730,
#14731,#14732,#14733,#14734,#14735,#14736,#14737,#14738,#14739,#14740));
#4032=EDGE_LOOP('',(#14741,#14742,#14743,#14744,#14745,#14746,#14747,#14748,
#14749,#14750,#14751,#14752,#14753,#14754,#14755,#14756,#14757,#14758,#14759,
#14760,#14761,#14762,#14763,#14764,#14765,#14766,#14767,#14768,#14769,#14770,
#14771,#14772,#14773,#14774,#14775,#14776,#14777,#14778,#14779,#14780,#14781,
#14782,#14783,#14784,#14785,#14786,#14787,#14788,#14789,#14790,#14791,#14792,
#14793,#14794,#14795,#14796,#14797,#14798,#14799,#14800,#14801,#14802,#14803,
#14804,#14805,#14806,#14807,#14808,#14809,#14810,#14811,#14812,#14813,#14814,
#14815,#14816,#14817,#14818,#14819,#14820,#14821,#14822,#14823,#14824));
#4033=EDGE_LOOP('',(#14825,#14826,#14827,#14828));
#4034=EDGE_LOOP('',(#14829));
#4035=EDGE_LOOP('',(#14830));
#4036=EDGE_LOOP('',(#14831,#14832,#14833,#14834,#14835));
#4037=EDGE_LOOP('',(#14836,#14837,#14838,#14839));
#4038=EDGE_LOOP('',(#14840,#14841,#14842,#14843,#14844,#14845,#14846,#14847,
#14848,#14849,#14850,#14851,#14852,#14853,#14854,#14855,#14856,#14857,#14858,
#14859,#14860,#14861,#14862,#14863,#14864,#14865,#14866,#14867,#14868,#14869,
#14870,#14871,#14872,#14873,#14874,#14875,#14876,#14877,#14878,#14879,#14880,
#14881,#14882,#14883,#14884,#14885,#14886,#14887,#14888,#14889,#14890,#14891,
#14892,#14893));
#4039=EDGE_LOOP('',(#14894,#14895,#14896,#14897,#14898,#14899,#14900,#14901,
#14902,#14903,#14904,#14905,#14906,#14907,#14908,#14909,#14910,#14911,#14912,
#14913,#14914,#14915,#14916,#14917,#14918,#14919,#14920,#14921,#14922,#14923,
#14924,#14925,#14926,#14927,#14928,#14929,#14930,#14931,#14932,#14933,#14934,
#14935,#14936,#14937,#14938,#14939,#14940,#14941,#14942,#14943,#14944,#14945,
#14946,#14947));
#4040=EDGE_LOOP('',(#14948,#14949,#14950,#14951));
#4041=EDGE_LOOP('',(#14952));
#4042=EDGE_LOOP('',(#14953));
#4043=EDGE_LOOP('',(#14954,#14955,#14956,#14957));
#4044=EDGE_LOOP('',(#14958,#14959,#14960,#14961));
#4045=EDGE_LOOP('',(#14962,#14963,#14964,#14965,#14966,#14967,#14968,#14969,
#14970,#14971,#14972,#14973,#14974,#14975,#14976,#14977,#14978,#14979,#14980,
#14981,#14982,#14983,#14984,#14985,#14986,#14987,#14988,#14989,#14990,#14991,
#14992,#14993,#14994,#14995,#14996,#14997,#14998,#14999,#15000,#15001,#15002,
#15003,#15004,#15005,#15006,#15007,#15008,#15009,#15010,#15011,#15012,#15013,
#15014,#15015,#15016,#15017,#15018,#15019,#15020,#15021,#15022,#15023,#15024,
#15025,#15026,#15027,#15028,#15029,#15030,#15031,#15032,#15033));
#4046=EDGE_LOOP('',(#15034,#15035,#15036,#15037));
#4047=EDGE_LOOP('',(#15038));
#4048=EDGE_LOOP('',(#15039));
#4049=EDGE_LOOP('',(#15040));
#4050=EDGE_LOOP('',(#15041));
#4051=EDGE_LOOP('',(#15042,#15043,#15044,#15045));
#4052=EDGE_LOOP('',(#15046,#15047,#15048,#15049));
#4053=EDGE_LOOP('',(#15050,#15051,#15052,#15053));
#4054=EDGE_LOOP('',(#15054,#15055,#15056,#15057));
#4055=EDGE_LOOP('',(#15058,#15059,#15060,#15061));
#4056=EDGE_LOOP('',(#15062,#15063,#15064,#15065));
#4057=EDGE_LOOP('',(#15066,#15067,#15068,#15069));
#4058=EDGE_LOOP('',(#15070,#15071,#15072,#15073));
#4059=EDGE_LOOP('',(#15074,#15075,#15076,#15077));
#4060=EDGE_LOOP('',(#15078,#15079,#15080,#15081));
#4061=EDGE_LOOP('',(#15082,#15083,#15084,#15085));
#4062=EDGE_LOOP('',(#15086,#15087,#15088,#15089));
#4063=EDGE_LOOP('',(#15090,#15091,#15092,#15093));
#4064=EDGE_LOOP('',(#15094,#15095,#15096,#15097));
#4065=EDGE_LOOP('',(#15098,#15099,#15100,#15101));
#4066=EDGE_LOOP('',(#15102,#15103,#15104,#15105));
#4067=EDGE_LOOP('',(#15106,#15107,#15108,#15109));
#4068=EDGE_LOOP('',(#15110,#15111,#15112,#15113));
#4069=EDGE_LOOP('',(#15114,#15115,#15116,#15117));
#4070=EDGE_LOOP('',(#15118,#15119,#15120,#15121));
#4071=EDGE_LOOP('',(#15122,#15123,#15124,#15125));
#4072=EDGE_LOOP('',(#15126,#15127,#15128,#15129));
#4073=EDGE_LOOP('',(#15130,#15131,#15132,#15133));
#4074=EDGE_LOOP('',(#15134,#15135,#15136,#15137));
#4075=EDGE_LOOP('',(#15138,#15139,#15140,#15141));
#4076=EDGE_LOOP('',(#15142,#15143,#15144,#15145));
#4077=EDGE_LOOP('',(#15146,#15147,#15148,#15149));
#4078=EDGE_LOOP('',(#15150,#15151,#15152,#15153));
#4079=EDGE_LOOP('',(#15154,#15155,#15156,#15157));
#4080=EDGE_LOOP('',(#15158,#15159,#15160,#15161));
#4081=EDGE_LOOP('',(#15162,#15163,#15164,#15165));
#4082=EDGE_LOOP('',(#15166,#15167,#15168,#15169));
#4083=EDGE_LOOP('',(#15170,#15171,#15172,#15173));
#4084=EDGE_LOOP('',(#15174,#15175,#15176,#15177));
#4085=EDGE_LOOP('',(#15178,#15179,#15180,#15181));
#4086=EDGE_LOOP('',(#15182,#15183,#15184,#15185));
#4087=EDGE_LOOP('',(#15186,#15187,#15188,#15189));
#4088=EDGE_LOOP('',(#15190,#15191,#15192,#15193));
#4089=EDGE_LOOP('',(#15194,#15195,#15196,#15197));
#4090=EDGE_LOOP('',(#15198,#15199,#15200,#15201));
#4091=EDGE_LOOP('',(#15202,#15203,#15204,#15205));
#4092=EDGE_LOOP('',(#15206,#15207,#15208,#15209));
#4093=EDGE_LOOP('',(#15210,#15211,#15212,#15213));
#4094=EDGE_LOOP('',(#15214,#15215,#15216,#15217));
#4095=EDGE_LOOP('',(#15218,#15219,#15220,#15221));
#4096=EDGE_LOOP('',(#15222,#15223,#15224,#15225));
#4097=EDGE_LOOP('',(#15226,#15227,#15228,#15229));
#4098=EDGE_LOOP('',(#15230,#15231,#15232,#15233));
#4099=EDGE_LOOP('',(#15234,#15235,#15236,#15237));
#4100=EDGE_LOOP('',(#15238,#15239,#15240,#15241));
#4101=EDGE_LOOP('',(#15242,#15243,#15244,#15245));
#4102=EDGE_LOOP('',(#15246,#15247,#15248,#15249));
#4103=EDGE_LOOP('',(#15250,#15251,#15252,#15253));
#4104=EDGE_LOOP('',(#15254,#15255,#15256,#15257));
#4105=EDGE_LOOP('',(#15258,#15259,#15260,#15261));
#4106=EDGE_LOOP('',(#15262,#15263,#15264,#15265));
#4107=EDGE_LOOP('',(#15266,#15267,#15268,#15269));
#4108=EDGE_LOOP('',(#15270,#15271,#15272,#15273));
#4109=EDGE_LOOP('',(#15274,#15275,#15276,#15277));
#4110=EDGE_LOOP('',(#15278,#15279,#15280,#15281));
#4111=EDGE_LOOP('',(#15282,#15283,#15284,#15285));
#4112=EDGE_LOOP('',(#15286,#15287,#15288,#15289));
#4113=EDGE_LOOP('',(#15290,#15291,#15292,#15293));
#4114=EDGE_LOOP('',(#15294,#15295,#15296,#15297));
#4115=EDGE_LOOP('',(#15298,#15299,#15300,#15301));
#4116=EDGE_LOOP('',(#15302,#15303,#15304,#15305));
#4117=EDGE_LOOP('',(#15306,#15307,#15308,#15309));
#4118=EDGE_LOOP('',(#15310,#15311,#15312,#15313));
#4119=EDGE_LOOP('',(#15314,#15315,#15316,#15317));
#4120=EDGE_LOOP('',(#15318,#15319,#15320,#15321));
#4121=EDGE_LOOP('',(#15322,#15323,#15324,#15325));
#4122=EDGE_LOOP('',(#15326,#15327,#15328,#15329));
#4123=EDGE_LOOP('',(#15330,#15331,#15332,#15333));
#4124=EDGE_LOOP('',(#15334,#15335,#15336,#15337));
#4125=EDGE_LOOP('',(#15338,#15339,#15340,#15341));
#4126=EDGE_LOOP('',(#15342,#15343,#15344,#15345,#15346,#15347,#15348,#15349,
#15350,#15351,#15352,#15353,#15354,#15355,#15356,#15357,#15358,#15359,#15360,
#15361,#15362,#15363,#15364,#15365,#15366,#15367,#15368,#15369,#15370,#15371,
#15372,#15373,#15374,#15375,#15376,#15377,#15378,#15379,#15380,#15381,#15382,
#15383,#15384,#15385,#15386,#15387,#15388,#15389,#15390,#15391,#15392,#15393,
#15394,#15395,#15396,#15397,#15398,#15399,#15400,#15401,#15402,#15403,#15404,
#15405,#15406,#15407,#15408,#15409,#15410,#15411,#15412,#15413));
#4127=EDGE_LOOP('',(#15414,#15415,#15416,#15417));
#4128=EDGE_LOOP('',(#15418));
#4129=EDGE_LOOP('',(#15419));
#4130=EDGE_LOOP('',(#15420));
#4131=EDGE_LOOP('',(#15421));
#5136=LINE('',#37343,#6350);
#5137=LINE('',#37355,#6351);
#5138=LINE('',#37378,#6352);
#5139=LINE('',#37468,#6353);
#5140=LINE('',#37555,#6354);
#5141=LINE('',#37642,#6355);
#5142=LINE('',#37729,#6356);
#5143=LINE('',#37819,#6357);
#5144=LINE('',#37906,#6358);
#5145=LINE('',#37993,#6359);
#5146=LINE('',#38083,#6360);
#5147=LINE('',#38170,#6361);
#5148=LINE('',#38257,#6362);
#5149=LINE('',#38344,#6363);
#5150=LINE('',#38434,#6364);
#5151=LINE('',#38521,#6365);
#5152=LINE('',#38608,#6366);
#5153=LINE('',#38695,#6367);
#5154=LINE('',#38785,#6368);
#5155=LINE('',#38872,#6369);
#5156=LINE('',#38959,#6370);
#5157=LINE('',#39049,#6371);
#5158=LINE('',#39136,#6372);
#5159=LINE('',#39223,#6373);
#5160=LINE('',#39310,#6374);
#5161=LINE('',#39400,#6375);
#5162=LINE('',#39469,#6376);
#5163=LINE('',#39502,#6377);
#5164=LINE('',#39539,#6378);
#5165=LINE('',#39577,#6379);
#5166=LINE('',#39613,#6380);
#5167=LINE('',#39651,#6381);
#5168=LINE('',#39689,#6382);
#5169=LINE('',#39725,#6383);
#5170=LINE('',#39763,#6384);
#5171=LINE('',#39801,#6385);
#5172=LINE('',#39837,#6386);
#5173=LINE('',#39875,#6387);
#5174=LINE('',#39912,#6388);
#5175=LINE('',#39949,#6389);
#5176=LINE('',#39987,#6390);
#5177=LINE('',#40023,#6391);
#5178=LINE('',#40061,#6392);
#5179=LINE('',#40099,#6393);
#5180=LINE('',#40135,#6394);
#5181=LINE('',#40173,#6395);
#5182=LINE('',#40211,#6396);
#5183=LINE('',#40247,#6397);
#5184=LINE('',#40285,#6398);
#5185=LINE('',#40322,#6399);
#5186=LINE('',#40359,#6400);
#5187=LINE('',#40379,#6401);
#5188=LINE('',#40391,#6402);
#5189=LINE('',#40414,#6403);
#5190=LINE('',#40504,#6404);
#5191=LINE('',#40591,#6405);
#5192=LINE('',#40678,#6406);
#5193=LINE('',#40765,#6407);
#5194=LINE('',#40852,#6408);
#5195=LINE('',#40942,#6409);
#5196=LINE('',#41029,#6410);
#5197=LINE('',#41116,#6411);
#5198=LINE('',#41203,#6412);
#5199=LINE('',#41290,#6413);
#5200=LINE('',#41380,#6414);
#5201=LINE('',#41467,#6415);
#5202=LINE('',#41554,#6416);
#5203=LINE('',#41641,#6417);
#5204=LINE('',#41728,#6418);
#5205=LINE('',#41815,#6419);
#5206=LINE('',#41902,#6420);
#5207=LINE('',#41989,#6421);
#5208=LINE('',#42064,#6422);
#5209=LINE('',#42112,#6423);
#5210=LINE('',#42169,#6424);
#5211=LINE('',#42256,#6425);
#5212=LINE('',#42343,#6426);
#5213=LINE('',#42430,#6427);
#5214=LINE('',#42517,#6428);
#5215=LINE('',#42604,#6429);
#5216=LINE('',#42694,#6430);
#5217=LINE('',#42781,#6431);
#5218=LINE('',#42868,#6432);
#5219=LINE('',#42955,#6433);
#5220=LINE('',#43042,#6434);
#5221=LINE('',#43132,#6435);
#5222=LINE('',#43219,#6436);
#5223=LINE('',#43306,#6437);
#5224=LINE('',#43393,#6438);
#5225=LINE('',#43480,#6439);
#5226=LINE('',#43570,#6440);
#5227=LINE('',#43657,#6441);
#5228=LINE('',#43726,#6442);
#5229=LINE('',#43759,#6443);
#5230=LINE('',#43796,#6444);
#5231=LINE('',#43834,#6445);
#5232=LINE('',#43870,#6446);
#5233=LINE('',#43908,#6447);
#5234=LINE('',#43945,#6448);
#5235=LINE('',#43982,#6449);
#5236=LINE('',#44020,#6450);
#5237=LINE('',#44056,#6451);
#5238=LINE('',#44094,#6452);
#5239=LINE('',#44131,#6453);
#5240=LINE('',#44168,#6454);
#5241=LINE('',#44206,#6455);
#5242=LINE('',#44242,#6456);
#5243=LINE('',#44280,#6457);
#5244=LINE('',#44317,#6458);
#5245=LINE('',#44354,#6459);
#5246=LINE('',#44392,#6460);
#5247=LINE('',#44428,#6461);
#5248=LINE('',#44455,#6462);
#5249=LINE('',#44479,#6463);
#5250=LINE('',#44512,#6464);
#5251=LINE('',#44550,#6465);
#5252=LINE('',#44586,#6466);
#5253=LINE('',#44624,#6467);
#5254=LINE('',#44660,#6468);
#5255=LINE('',#44698,#6469);
#5256=LINE('',#44736,#6470);
#5257=LINE('',#44772,#6471);
#5258=LINE('',#44810,#6472);
#5259=LINE('',#44846,#6473);
#5260=LINE('',#44884,#6474);
#5261=LINE('',#44922,#6475);
#5262=LINE('',#44958,#6476);
#5263=LINE('',#44996,#6477);
#5264=LINE('',#45032,#6478);
#5265=LINE('',#45070,#6479);
#5266=LINE('',#45108,#6480);
#5267=LINE('',#45144,#6481);
#5268=LINE('',#52811,#6482);
#5269=LINE('',#52814,#6483);
#5270=LINE('',#52817,#6484);
#5271=LINE('',#52819,#6485);
#5272=LINE('',#52820,#6486);
#5273=LINE('',#52823,#6487);
#5274=LINE('',#52827,#6488);
#5275=LINE('',#52831,#6489);
#5276=LINE('',#52835,#6490);
#5277=LINE('',#52839,#6491);
#5278=LINE('',#52843,#6492);
#5279=LINE('',#52847,#6493);
#5280=LINE('',#52851,#6494);
#5281=LINE('',#52855,#6495);
#5282=LINE('',#52859,#6496);
#5283=LINE('',#52863,#6497);
#5284=LINE('',#52867,#6498);
#5285=LINE('',#52871,#6499);
#5286=LINE('',#52875,#6500);
#5287=LINE('',#52879,#6501);
#5288=LINE('',#52883,#6502);
#5289=LINE('',#52887,#6503);
#5290=LINE('',#52891,#6504);
#5291=LINE('',#52895,#6505);
#5292=LINE('',#52899,#6506);
#5293=LINE('',#52903,#6507);
#5294=LINE('',#52907,#6508);
#5295=LINE('',#52911,#6509);
#5296=LINE('',#52915,#6510);
#5297=LINE('',#52919,#6511);
#5298=LINE('',#52923,#6512);
#5299=LINE('',#52927,#6513);
#5300=LINE('',#52931,#6514);
#5301=LINE('',#52935,#6515);
#5302=LINE('',#52939,#6516);
#5303=LINE('',#52943,#6517);
#5304=LINE('',#52947,#6518);
#5305=LINE('',#52951,#6519);
#5306=LINE('',#52955,#6520);
#5307=LINE('',#52959,#6521);
#5308=LINE('',#52973,#6522);
#5309=LINE('',#52974,#6523);
#5310=LINE('',#52977,#6524);
#5311=LINE('',#52978,#6525);
#5312=LINE('',#52982,#6526);
#5313=LINE('',#52985,#6527);
#5314=LINE('',#52986,#6528);
#5315=LINE('',#52990,#6529);
#5316=LINE('',#52993,#6530);
#5317=LINE('',#52994,#6531);
#5318=LINE('',#52998,#6532);
#5319=LINE('',#53001,#6533);
#5320=LINE('',#53002,#6534);
#5321=LINE('',#53006,#6535);
#5322=LINE('',#53009,#6536);
#5323=LINE('',#53012,#6537);
#5324=LINE('',#53015,#6538);
#5325=LINE('',#53016,#6539);
#5326=LINE('',#53020,#6540);
#5327=LINE('',#53023,#6541);
#5328=LINE('',#53026,#6542);
#5329=LINE('',#53029,#6543);
#5330=LINE('',#53030,#6544);
#5331=LINE('',#53034,#6545);
#5332=LINE('',#53039,#6546);
#5333=LINE('',#53040,#6547);
#5334=LINE('',#53043,#6548);
#5335=LINE('',#53044,#6549);
#5336=LINE('',#53048,#6550);
#5337=LINE('',#53051,#6551);
#5338=LINE('',#53052,#6552);
#5339=LINE('',#53056,#6553);
#5340=LINE('',#53059,#6554);
#5341=LINE('',#53060,#6555);
#5342=LINE('',#53064,#6556);
#5343=LINE('',#53067,#6557);
#5344=LINE('',#53068,#6558);
#5345=LINE('',#53072,#6559);
#5346=LINE('',#53075,#6560);
#5347=LINE('',#53078,#6561);
#5348=LINE('',#53081,#6562);
#5349=LINE('',#53082,#6563);
#5350=LINE('',#53086,#6564);
#5351=LINE('',#53089,#6565);
#5352=LINE('',#53092,#6566);
#5353=LINE('',#53095,#6567);
#5354=LINE('',#53096,#6568);
#5355=LINE('',#53100,#6569);
#5356=LINE('',#53105,#6570);
#5357=LINE('',#53106,#6571);
#5358=LINE('',#53109,#6572);
#5359=LINE('',#53110,#6573);
#5360=LINE('',#53114,#6574);
#5361=LINE('',#53117,#6575);
#5362=LINE('',#53118,#6576);
#5363=LINE('',#53122,#6577);
#5364=LINE('',#53125,#6578);
#5365=LINE('',#53126,#6579);
#5366=LINE('',#53130,#6580);
#5367=LINE('',#53133,#6581);
#5368=LINE('',#53134,#6582);
#5369=LINE('',#53138,#6583);
#5370=LINE('',#53141,#6584);
#5371=LINE('',#53144,#6585);
#5372=LINE('',#53147,#6586);
#5373=LINE('',#53148,#6587);
#5374=LINE('',#53152,#6588);
#5375=LINE('',#53155,#6589);
#5376=LINE('',#53158,#6590);
#5377=LINE('',#53161,#6591);
#5378=LINE('',#53162,#6592);
#5379=LINE('',#53166,#6593);
#5380=LINE('',#53171,#6594);
#5381=LINE('',#53172,#6595);
#5382=LINE('',#53175,#6596);
#5383=LINE('',#53176,#6597);
#5384=LINE('',#53180,#6598);
#5385=LINE('',#53183,#6599);
#5386=LINE('',#53184,#6600);
#5387=LINE('',#53188,#6601);
#5388=LINE('',#53191,#6602);
#5389=LINE('',#53192,#6603);
#5390=LINE('',#53196,#6604);
#5391=LINE('',#53199,#6605);
#5392=LINE('',#53200,#6606);
#5393=LINE('',#53204,#6607);
#5394=LINE('',#53207,#6608);
#5395=LINE('',#53210,#6609);
#5396=LINE('',#53213,#6610);
#5397=LINE('',#53214,#6611);
#5398=LINE('',#53218,#6612);
#5399=LINE('',#53221,#6613);
#5400=LINE('',#53225,#6614);
#5401=LINE('',#53229,#6615);
#5402=LINE('',#53232,#6616);
#5403=LINE('',#53235,#6617);
#5404=LINE('',#53239,#6618);
#5405=LINE('',#53242,#6619);
#5406=LINE('',#53244,#6620);
#5407=LINE('',#53246,#6621);
#5408=LINE('',#53248,#6622);
#5409=LINE('',#53250,#6623);
#5410=LINE('',#53252,#6624);
#5411=LINE('',#53254,#6625);
#5412=LINE('',#53256,#6626);
#5413=LINE('',#53258,#6627);
#5414=LINE('',#53260,#6628);
#5415=LINE('',#53262,#6629);
#5416=LINE('',#53264,#6630);
#6350=VECTOR('',#24220,5.);
#6351=VECTOR('',#24223,5.);
#6352=VECTOR('',#24230,5.);
#6353=VECTOR('',#24233,5.);
#6354=VECTOR('',#24236,5.);
#6355=VECTOR('',#24239,5.);
#6356=VECTOR('',#24242,5.);
#6357=VECTOR('',#24245,5.);
#6358=VECTOR('',#24248,5.);
#6359=VECTOR('',#24251,5.);
#6360=VECTOR('',#24254,5.);
#6361=VECTOR('',#24257,5.);
#6362=VECTOR('',#24260,5.);
#6363=VECTOR('',#24263,5.);
#6364=VECTOR('',#24266,5.);
#6365=VECTOR('',#24269,5.);
#6366=VECTOR('',#24272,5.);
#6367=VECTOR('',#24275,5.);
#6368=VECTOR('',#24278,5.);
#6369=VECTOR('',#24281,5.);
#6370=VECTOR('',#24284,5.);
#6371=VECTOR('',#24287,5.);
#6372=VECTOR('',#24290,5.);
#6373=VECTOR('',#24293,5.);
#6374=VECTOR('',#24296,5.);
#6375=VECTOR('',#24299,5.);
#6376=VECTOR('',#24304,5.0736);
#6377=VECTOR('',#24309,5.0736);
#6378=VECTOR('',#24312,5.0736);
#6379=VECTOR('',#24315,5.0736);
#6380=VECTOR('',#24318,5.0736);
#6381=VECTOR('',#24321,5.0736);
#6382=VECTOR('',#24324,5.0736);
#6383=VECTOR('',#24327,5.0736);
#6384=VECTOR('',#24330,5.0736);
#6385=VECTOR('',#24333,5.0736);
#6386=VECTOR('',#24336,5.0736);
#6387=VECTOR('',#24339,5.0736);
#6388=VECTOR('',#24342,5.0736);
#6389=VECTOR('',#24345,5.0736);
#6390=VECTOR('',#24348,5.0736);
#6391=VECTOR('',#24351,5.0736);
#6392=VECTOR('',#24354,5.0736);
#6393=VECTOR('',#24357,5.0736);
#6394=VECTOR('',#24360,5.0736);
#6395=VECTOR('',#24363,5.0736);
#6396=VECTOR('',#24366,5.0736);
#6397=VECTOR('',#24369,5.0736);
#6398=VECTOR('',#24372,5.0736);
#6399=VECTOR('',#24375,5.0736);
#6400=VECTOR('',#24378,5.0736);
#6401=VECTOR('',#24383,5.);
#6402=VECTOR('',#24386,5.);
#6403=VECTOR('',#24393,5.);
#6404=VECTOR('',#24396,5.);
#6405=VECTOR('',#24399,5.);
#6406=VECTOR('',#24402,5.);
#6407=VECTOR('',#24405,5.);
#6408=VECTOR('',#24408,5.);
#6409=VECTOR('',#24411,5.);
#6410=VECTOR('',#24414,5.);
#6411=VECTOR('',#24417,5.);
#6412=VECTOR('',#24420,5.);
#6413=VECTOR('',#24423,5.);
#6414=VECTOR('',#24426,5.);
#6415=VECTOR('',#24429,5.);
#6416=VECTOR('',#24432,5.);
#6417=VECTOR('',#24435,5.);
#6418=VECTOR('',#24438,5.);
#6419=VECTOR('',#24441,5.);
#6420=VECTOR('',#24444,5.);
#6421=VECTOR('',#24447,5.);
#6422=VECTOR('',#24450,5.);
#6423=VECTOR('',#24453,5.);
#6424=VECTOR('',#24456,5.);
#6425=VECTOR('',#24459,5.);
#6426=VECTOR('',#24462,5.);
#6427=VECTOR('',#24465,5.);
#6428=VECTOR('',#24468,5.);
#6429=VECTOR('',#24471,5.);
#6430=VECTOR('',#24474,5.);
#6431=VECTOR('',#24477,5.);
#6432=VECTOR('',#24480,5.);
#6433=VECTOR('',#24483,5.);
#6434=VECTOR('',#24486,5.);
#6435=VECTOR('',#24489,5.);
#6436=VECTOR('',#24492,5.);
#6437=VECTOR('',#24495,5.);
#6438=VECTOR('',#24498,5.);
#6439=VECTOR('',#24501,5.);
#6440=VECTOR('',#24504,5.);
#6441=VECTOR('',#24507,5.);
#6442=VECTOR('',#24512,5.0736);
#6443=VECTOR('',#24517,5.0736);
#6444=VECTOR('',#24520,5.0736);
#6445=VECTOR('',#24523,5.0736);
#6446=VECTOR('',#24526,5.0736);
#6447=VECTOR('',#24529,5.0736);
#6448=VECTOR('',#24532,5.0736);
#6449=VECTOR('',#24535,5.0736);
#6450=VECTOR('',#24538,5.0736);
#6451=VECTOR('',#24541,5.0736);
#6452=VECTOR('',#24544,5.0736);
#6453=VECTOR('',#24547,5.0736);
#6454=VECTOR('',#24550,5.0736);
#6455=VECTOR('',#24553,5.0736);
#6456=VECTOR('',#24556,5.0736);
#6457=VECTOR('',#24559,5.0736);
#6458=VECTOR('',#24562,5.0736);
#6459=VECTOR('',#24565,5.0736);
#6460=VECTOR('',#24568,5.0736);
#6461=VECTOR('',#24571,5.0736);
#6462=VECTOR('',#24574,5.0736);
#6463=VECTOR('',#24577,5.0736);
#6464=VECTOR('',#24580,5.0736);
#6465=VECTOR('',#24583,5.0736);
#6466=VECTOR('',#24586,5.0736);
#6467=VECTOR('',#24589,5.0736);
#6468=VECTOR('',#24592,5.0736);
#6469=VECTOR('',#24595,5.0736);
#6470=VECTOR('',#24598,5.0736);
#6471=VECTOR('',#24601,5.0736);
#6472=VECTOR('',#24604,5.0736);
#6473=VECTOR('',#24607,5.0736);
#6474=VECTOR('',#24610,5.0736);
#6475=VECTOR('',#24613,5.0736);
#6476=VECTOR('',#24616,5.0736);
#6477=VECTOR('',#24619,5.0736);
#6478=VECTOR('',#24622,5.0736);
#6479=VECTOR('',#24625,5.0736);
#6480=VECTOR('',#24628,5.0736);
#6481=VECTOR('',#24631,5.0736);
#6482=VECTOR('',#24658,10.);
#6483=VECTOR('',#24661,10.);
#6484=VECTOR('',#24664,10.);
#6485=VECTOR('',#24665,10.);
#6486=VECTOR('',#24666,10.);
#6487=VECTOR('',#24669,10.);
#6488=VECTOR('',#24672,10.);
#6489=VECTOR('',#24675,10.);
#6490=VECTOR('',#24678,10.);
#6491=VECTOR('',#24681,10.);
#6492=VECTOR('',#24684,10.);
#6493=VECTOR('',#24687,10.);
#6494=VECTOR('',#24690,10.);
#6495=VECTOR('',#24693,10.);
#6496=VECTOR('',#24696,10.);
#6497=VECTOR('',#24699,10.);
#6498=VECTOR('',#24702,10.);
#6499=VECTOR('',#24705,10.);
#6500=VECTOR('',#24708,10.);
#6501=VECTOR('',#24711,10.);
#6502=VECTOR('',#24714,10.);
#6503=VECTOR('',#24717,10.);
#6504=VECTOR('',#24720,10.);
#6505=VECTOR('',#24723,10.);
#6506=VECTOR('',#24726,10.);
#6507=VECTOR('',#24729,10.);
#6508=VECTOR('',#24732,10.);
#6509=VECTOR('',#24735,10.);
#6510=VECTOR('',#24738,10.);
#6511=VECTOR('',#24741,10.);
#6512=VECTOR('',#24744,10.);
#6513=VECTOR('',#24747,10.);
#6514=VECTOR('',#24750,10.);
#6515=VECTOR('',#24753,10.);
#6516=VECTOR('',#24756,10.);
#6517=VECTOR('',#24759,10.);
#6518=VECTOR('',#24762,10.);
#6519=VECTOR('',#24765,10.);
#6520=VECTOR('',#24768,10.);
#6521=VECTOR('',#24771,10.);
#6522=VECTOR('',#24786,10.);
#6523=VECTOR('',#24787,10.);
#6524=VECTOR('',#24790,10.);
#6525=VECTOR('',#24791,10.);
#6526=VECTOR('',#24796,10.);
#6527=VECTOR('',#24799,10.);
#6528=VECTOR('',#24800,10.);
#6529=VECTOR('',#24805,10.);
#6530=VECTOR('',#24808,10.);
#6531=VECTOR('',#24809,10.);
#6532=VECTOR('',#24814,10.);
#6533=VECTOR('',#24817,10.);
#6534=VECTOR('',#24818,10.);
#6535=VECTOR('',#24823,10.);
#6536=VECTOR('',#24826,10.);
#6537=VECTOR('',#24829,10.);
#6538=VECTOR('',#24832,10.);
#6539=VECTOR('',#24833,10.);
#6540=VECTOR('',#24838,10.);
#6541=VECTOR('',#24841,10.);
#6542=VECTOR('',#24844,10.);
#6543=VECTOR('',#24847,10.);
#6544=VECTOR('',#24848,10.);
#6545=VECTOR('',#24853,10.);
#6546=VECTOR('',#24858,10.);
#6547=VECTOR('',#24859,10.);
#6548=VECTOR('',#24862,10.);
#6549=VECTOR('',#24863,10.);
#6550=VECTOR('',#24868,10.);
#6551=VECTOR('',#24871,10.);
#6552=VECTOR('',#24872,10.);
#6553=VECTOR('',#24877,10.);
#6554=VECTOR('',#24880,10.);
#6555=VECTOR('',#24881,10.);
#6556=VECTOR('',#24886,10.);
#6557=VECTOR('',#24889,10.);
#6558=VECTOR('',#24890,10.);
#6559=VECTOR('',#24895,10.);
#6560=VECTOR('',#24898,10.);
#6561=VECTOR('',#24901,10.);
#6562=VECTOR('',#24904,10.);
#6563=VECTOR('',#24905,10.);
#6564=VECTOR('',#24910,10.);
#6565=VECTOR('',#24913,10.);
#6566=VECTOR('',#24916,10.);
#6567=VECTOR('',#24919,10.);
#6568=VECTOR('',#24920,10.);
#6569=VECTOR('',#24925,10.);
#6570=VECTOR('',#24930,10.);
#6571=VECTOR('',#24931,10.);
#6572=VECTOR('',#24934,10.);
#6573=VECTOR('',#24935,10.);
#6574=VECTOR('',#24940,10.);
#6575=VECTOR('',#24943,10.);
#6576=VECTOR('',#24944,10.);
#6577=VECTOR('',#24949,10.);
#6578=VECTOR('',#24952,10.);
#6579=VECTOR('',#24953,10.);
#6580=VECTOR('',#24958,10.);
#6581=VECTOR('',#24961,10.);
#6582=VECTOR('',#24962,10.);
#6583=VECTOR('',#24967,10.);
#6584=VECTOR('',#24970,10.);
#6585=VECTOR('',#24973,10.);
#6586=VECTOR('',#24976,10.);
#6587=VECTOR('',#24977,10.);
#6588=VECTOR('',#24982,10.);
#6589=VECTOR('',#24985,10.);
#6590=VECTOR('',#24988,10.);
#6591=VECTOR('',#24991,10.);
#6592=VECTOR('',#24992,10.);
#6593=VECTOR('',#24997,10.);
#6594=VECTOR('',#25002,10.);
#6595=VECTOR('',#25003,10.);
#6596=VECTOR('',#25006,10.);
#6597=VECTOR('',#25007,10.);
#6598=VECTOR('',#25012,10.);
#6599=VECTOR('',#25015,10.);
#6600=VECTOR('',#25016,10.);
#6601=VECTOR('',#25021,10.);
#6602=VECTOR('',#25024,10.);
#6603=VECTOR('',#25025,10.);
#6604=VECTOR('',#25030,10.);
#6605=VECTOR('',#25033,10.);
#6606=VECTOR('',#25034,10.);
#6607=VECTOR('',#25039,10.);
#6608=VECTOR('',#25042,10.);
#6609=VECTOR('',#25045,10.);
#6610=VECTOR('',#25048,10.);
#6611=VECTOR('',#25049,10.);
#6612=VECTOR('',#25054,10.);
#6613=VECTOR('',#25057,10.);
#6614=VECTOR('',#25062,3.);
#6615=VECTOR('',#25067,3.);
#6616=VECTOR('',#25072,4.);
#6617=VECTOR('',#25075,3.);
#6618=VECTOR('',#25080,3.);
#6619=VECTOR('',#25085,10.);
#6620=VECTOR('',#25088,10.);
#6621=VECTOR('',#25091,10.);
#6622=VECTOR('',#25094,10.);
#6623=VECTOR('',#25097,10.);
#6624=VECTOR('',#25100,10.);
#6625=VECTOR('',#25103,10.);
#6626=VECTOR('',#25106,10.);
#6627=VECTOR('',#25109,10.);
#6628=VECTOR('',#25112,10.);
#6629=VECTOR('',#25115,10.);
#6630=VECTOR('',#25118,10.);
#7403=CIRCLE('',#22299,4.51775);
#7404=CIRCLE('',#22300,4.51775);
#7405=CIRCLE('',#22301,4.51775);
#7406=CIRCLE('',#22326,4.51775);
#7407=CIRCLE('',#22328,5.0736);
#7408=CIRCLE('',#22353,5.0736);
#7409=CIRCLE('',#22355,4.51775);
#7410=CIRCLE('',#22356,4.51775);
#7411=CIRCLE('',#22357,4.51775);
#7412=CIRCLE('',#22397,4.51775);
#7413=CIRCLE('',#22399,5.07359999999999);
#7414=CIRCLE('',#22439,5.0736);
#7415=CIRCLE('',#22444,4.);
#7416=CIRCLE('',#22449,4.);
#7417=CIRCLE('',#22451,1.);
#7418=CIRCLE('',#22452,1.);
#7419=CIRCLE('',#22455,1.);
#7420=CIRCLE('',#22456,1.);
#7421=CIRCLE('',#22457,1.);
#7422=CIRCLE('',#22458,1.);
#7423=CIRCLE('',#22459,1.);
#7424=CIRCLE('',#22460,1.);
#7425=CIRCLE('',#22461,1.);
#7426=CIRCLE('',#22462,1.);
#7427=CIRCLE('',#22463,1.);
#7428=CIRCLE('',#22464,1.);
#7429=CIRCLE('',#22465,1.);
#7430=CIRCLE('',#22466,1.);
#7431=CIRCLE('',#22467,1.);
#7432=CIRCLE('',#22468,1.);
#7433=CIRCLE('',#22469,1.);
#7434=CIRCLE('',#22470,1.);
#7435=CIRCLE('',#22471,1.);
#7436=CIRCLE('',#22472,1.);
#7437=CIRCLE('',#22473,1.);
#7438=CIRCLE('',#22474,1.);
#7439=CIRCLE('',#22475,1.);
#7440=CIRCLE('',#22476,1.);
#7441=CIRCLE('',#22477,1.);
#7442=CIRCLE('',#22478,1.);
#7443=CIRCLE('',#22479,1.);
#7444=CIRCLE('',#22480,1.);
#7445=CIRCLE('',#22481,1.);
#7446=CIRCLE('',#22482,1.);
#7447=CIRCLE('',#22483,1.);
#7448=CIRCLE('',#22484,1.);
#7449=CIRCLE('',#22485,1.);
#7450=CIRCLE('',#22486,1.);
#7451=CIRCLE('',#22487,1.);
#7452=CIRCLE('',#22488,1.);
#7453=CIRCLE('',#22489,1.);
#7454=CIRCLE('',#22490,3.);
#7455=CIRCLE('',#22491,3.);
#7456=CIRCLE('',#22492,3.);
#7457=CIRCLE('',#22493,3.);
#7458=CIRCLE('',#22495,1.);
#7459=CIRCLE('',#22498,1.);
#7460=CIRCLE('',#22501,1.);
#7461=CIRCLE('',#22504,1.);
#7462=CIRCLE('',#22507,1.);
#7463=CIRCLE('',#22509,1.);
#7464=CIRCLE('',#22512,1.);
#7465=CIRCLE('',#22514,1.);
#7466=CIRCLE('',#22517,1.);
#7467=CIRCLE('',#22519,1.);
#7468=CIRCLE('',#22522,1.);
#7469=CIRCLE('',#22525,1.);
#7470=CIRCLE('',#22528,1.);
#7471=CIRCLE('',#22531,1.);
#7472=CIRCLE('',#22533,1.);
#7473=CIRCLE('',#22536,1.);
#7474=CIRCLE('',#22538,1.);
#7475=CIRCLE('',#22541,1.);
#7476=CIRCLE('',#22543,1.);
#7477=CIRCLE('',#22546,1.);
#7478=CIRCLE('',#22549,1.);
#7479=CIRCLE('',#22552,1.);
#7480=CIRCLE('',#22555,1.);
#7481=CIRCLE('',#22557,1.);
#7482=CIRCLE('',#22560,1.);
#7483=CIRCLE('',#22562,1.);
#7484=CIRCLE('',#22565,1.);
#7485=CIRCLE('',#22567,1.);
#7486=CIRCLE('',#22570,1.);
#7487=CIRCLE('',#22573,1.);
#7488=CIRCLE('',#22576,1.);
#7489=CIRCLE('',#22579,1.);
#7490=CIRCLE('',#22581,1.);
#7491=CIRCLE('',#22584,1.);
#7492=CIRCLE('',#22586,1.);
#7493=CIRCLE('',#22588,3.);
#7494=CIRCLE('',#22590,3.);
#7495=CIRCLE('',#22593,3.);
#7496=CIRCLE('',#22595,3.);
#7949=VERTEX_POINT('',#37341);
#7950=VERTEX_POINT('',#37342);
#7951=VERTEX_POINT('',#37344);
#7952=VERTEX_POINT('',#37352);
#7953=VERTEX_POINT('',#37354);
#7954=VERTEX_POINT('',#37357);
#7955=VERTEX_POINT('',#37376);
#7956=VERTEX_POINT('',#37377);
#7957=VERTEX_POINT('',#37466);
#7958=VERTEX_POINT('',#37467);
#7959=VERTEX_POINT('',#37553);
#7960=VERTEX_POINT('',#37554);
#7961=VERTEX_POINT('',#37640);
#7962=VERTEX_POINT('',#37641);
#7963=VERTEX_POINT('',#37727);
#7964=VERTEX_POINT('',#37728);
#7965=VERTEX_POINT('',#37817);
#7966=VERTEX_POINT('',#37818);
#7967=VERTEX_POINT('',#37904);
#7968=VERTEX_POINT('',#37905);
#7969=VERTEX_POINT('',#37991);
#7970=VERTEX_POINT('',#37992);
#7971=VERTEX_POINT('',#38081);
#7972=VERTEX_POINT('',#38082);
#7973=VERTEX_POINT('',#38168);
#7974=VERTEX_POINT('',#38169);
#7975=VERTEX_POINT('',#38255);
#7976=VERTEX_POINT('',#38256);
#7977=VERTEX_POINT('',#38342);
#7978=VERTEX_POINT('',#38343);
#7979=VERTEX_POINT('',#38432);
#7980=VERTEX_POINT('',#38433);
#7981=VERTEX_POINT('',#38519);
#7982=VERTEX_POINT('',#38520);
#7983=VERTEX_POINT('',#38606);
#7984=VERTEX_POINT('',#38607);
#7985=VERTEX_POINT('',#38693);
#7986=VERTEX_POINT('',#38694);
#7987=VERTEX_POINT('',#38783);
#7988=VERTEX_POINT('',#38784);
#7989=VERTEX_POINT('',#38870);
#7990=VERTEX_POINT('',#38871);
#7991=VERTEX_POINT('',#38957);
#7992=VERTEX_POINT('',#38958);
#7993=VERTEX_POINT('',#39047);
#7994=VERTEX_POINT('',#39048);
#7995=VERTEX_POINT('',#39134);
#7996=VERTEX_POINT('',#39135);
#7997=VERTEX_POINT('',#39221);
#7998=VERTEX_POINT('',#39222);
#7999=VERTEX_POINT('',#39308);
#8000=VERTEX_POINT('',#39309);
#8001=VERTEX_POINT('',#39398);
#8002=VERTEX_POINT('',#39399);
#8003=VERTEX_POINT('',#39401);
#8004=VERTEX_POINT('',#39427);
#8005=VERTEX_POINT('',#39467);
#8006=VERTEX_POINT('',#39468);
#8007=VERTEX_POINT('',#39470);
#8008=VERTEX_POINT('',#39483);
#8009=VERTEX_POINT('',#39500);
#8010=VERTEX_POINT('',#39501);
#8011=VERTEX_POINT('',#39537);
#8012=VERTEX_POINT('',#39538);
#8013=VERTEX_POINT('',#39575);
#8014=VERTEX_POINT('',#39576);
#8015=VERTEX_POINT('',#39611);
#8016=VERTEX_POINT('',#39612);
#8017=VERTEX_POINT('',#39649);
#8018=VERTEX_POINT('',#39650);
#8019=VERTEX_POINT('',#39687);
#8020=VERTEX_POINT('',#39688);
#8021=VERTEX_POINT('',#39723);
#8022=VERTEX_POINT('',#39724);
#8023=VERTEX_POINT('',#39761);
#8024=VERTEX_POINT('',#39762);
#8025=VERTEX_POINT('',#39799);
#8026=VERTEX_POINT('',#39800);
#8027=VERTEX_POINT('',#39835);
#8028=VERTEX_POINT('',#39836);
#8029=VERTEX_POINT('',#39873);
#8030=VERTEX_POINT('',#39874);
#8031=VERTEX_POINT('',#39910);
#8032=VERTEX_POINT('',#39911);
#8033=VERTEX_POINT('',#39947);
#8034=VERTEX_POINT('',#39948);
#8035=VERTEX_POINT('',#39985);
#8036=VERTEX_POINT('',#39986);
#8037=VERTEX_POINT('',#40021);
#8038=VERTEX_POINT('',#40022);
#8039=VERTEX_POINT('',#40059);
#8040=VERTEX_POINT('',#40060);
#8041=VERTEX_POINT('',#40097);
#8042=VERTEX_POINT('',#40098);
#8043=VERTEX_POINT('',#40133);
#8044=VERTEX_POINT('',#40134);
#8045=VERTEX_POINT('',#40171);
#8046=VERTEX_POINT('',#40172);
#8047=VERTEX_POINT('',#40209);
#8048=VERTEX_POINT('',#40210);
#8049=VERTEX_POINT('',#40245);
#8050=VERTEX_POINT('',#40246);
#8051=VERTEX_POINT('',#40283);
#8052=VERTEX_POINT('',#40284);
#8053=VERTEX_POINT('',#40320);
#8054=VERTEX_POINT('',#40321);
#8055=VERTEX_POINT('',#40357);
#8056=VERTEX_POINT('',#40358);
#8057=VERTEX_POINT('',#40360);
#8058=VERTEX_POINT('',#40367);
#8059=VERTEX_POINT('',#40377);
#8060=VERTEX_POINT('',#40378);
#8061=VERTEX_POINT('',#40380);
#8062=VERTEX_POINT('',#40388);
#8063=VERTEX_POINT('',#40390);
#8064=VERTEX_POINT('',#40393);
#8065=VERTEX_POINT('',#40412);
#8066=VERTEX_POINT('',#40413);
#8067=VERTEX_POINT('',#40502);
#8068=VERTEX_POINT('',#40503);
#8069=VERTEX_POINT('',#40589);
#8070=VERTEX_POINT('',#40590);
#8071=VERTEX_POINT('',#40676);
#8072=VERTEX_POINT('',#40677);
#8073=VERTEX_POINT('',#40763);
#8074=VERTEX_POINT('',#40764);
#8075=VERTEX_POINT('',#40850);
#8076=VERTEX_POINT('',#40851);
#8077=VERTEX_POINT('',#40940);
#8078=VERTEX_POINT('',#40941);
#8079=VERTEX_POINT('',#41027);
#8080=VERTEX_POINT('',#41028);
#8081=VERTEX_POINT('',#41114);
#8082=VERTEX_POINT('',#41115);
#8083=VERTEX_POINT('',#41201);
#8084=VERTEX_POINT('',#41202);
#8085=VERTEX_POINT('',#41288);
#8086=VERTEX_POINT('',#41289);
#8087=VERTEX_POINT('',#41378);
#8088=VERTEX_POINT('',#41379);
#8089=VERTEX_POINT('',#41465);
#8090=VERTEX_POINT('',#41466);
#8091=VERTEX_POINT('',#41552);
#8092=VERTEX_POINT('',#41553);
#8093=VERTEX_POINT('',#41639);
#8094=VERTEX_POINT('',#41640);
#8095=VERTEX_POINT('',#41726);
#8096=VERTEX_POINT('',#41727);
#8097=VERTEX_POINT('',#41813);
#8098=VERTEX_POINT('',#41814);
#8099=VERTEX_POINT('',#41900);
#8100=VERTEX_POINT('',#41901);
#8101=VERTEX_POINT('',#41987);
#8102=VERTEX_POINT('',#41988);
#8103=VERTEX_POINT('',#42062);
#8104=VERTEX_POINT('',#42063);
#8105=VERTEX_POINT('',#42110);
#8106=VERTEX_POINT('',#42111);
#8107=VERTEX_POINT('',#42167);
#8108=VERTEX_POINT('',#42168);
#8109=VERTEX_POINT('',#42254);
#8110=VERTEX_POINT('',#42255);
#8111=VERTEX_POINT('',#42341);
#8112=VERTEX_POINT('',#42342);
#8113=VERTEX_POINT('',#42428);
#8114=VERTEX_POINT('',#42429);
#8115=VERTEX_POINT('',#42515);
#8116=VERTEX_POINT('',#42516);
#8117=VERTEX_POINT('',#42602);
#8118=VERTEX_POINT('',#42603);
#8119=VERTEX_POINT('',#42692);
#8120=VERTEX_POINT('',#42693);
#8121=VERTEX_POINT('',#42779);
#8122=VERTEX_POINT('',#42780);
#8123=VERTEX_POINT('',#42866);
#8124=VERTEX_POINT('',#42867);
#8125=VERTEX_POINT('',#42953);
#8126=VERTEX_POINT('',#42954);
#8127=VERTEX_POINT('',#43040);
#8128=VERTEX_POINT('',#43041);
#8129=VERTEX_POINT('',#43130);
#8130=VERTEX_POINT('',#43131);
#8131=VERTEX_POINT('',#43217);
#8132=VERTEX_POINT('',#43218);
#8133=VERTEX_POINT('',#43304);
#8134=VERTEX_POINT('',#43305);
#8135=VERTEX_POINT('',#43391);
#8136=VERTEX_POINT('',#43392);
#8137=VERTEX_POINT('',#43478);
#8138=VERTEX_POINT('',#43479);
#8139=VERTEX_POINT('',#43568);
#8140=VERTEX_POINT('',#43569);
#8141=VERTEX_POINT('',#43655);
#8142=VERTEX_POINT('',#43656);
#8143=VERTEX_POINT('',#43658);
#8144=VERTEX_POINT('',#43684);
#8145=VERTEX_POINT('',#43724);
#8146=VERTEX_POINT('',#43725);
#8147=VERTEX_POINT('',#43727);
#8148=VERTEX_POINT('',#43740);
#8149=VERTEX_POINT('',#43757);
#8150=VERTEX_POINT('',#43758);
#8151=VERTEX_POINT('',#43794);
#8152=VERTEX_POINT('',#43795);
#8153=VERTEX_POINT('',#43832);
#8154=VERTEX_POINT('',#43833);
#8155=VERTEX_POINT('',#43868);
#8156=VERTEX_POINT('',#43869);
#8157=VERTEX_POINT('',#43906);
#8158=VERTEX_POINT('',#43907);
#8159=VERTEX_POINT('',#43943);
#8160=VERTEX_POINT('',#43944);
#8161=VERTEX_POINT('',#43980);
#8162=VERTEX_POINT('',#43981);
#8163=VERTEX_POINT('',#44018);
#8164=VERTEX_POINT('',#44019);
#8165=VERTEX_POINT('',#44054);
#8166=VERTEX_POINT('',#44055);
#8167=VERTEX_POINT('',#44092);
#8168=VERTEX_POINT('',#44093);
#8169=VERTEX_POINT('',#44129);
#8170=VERTEX_POINT('',#44130);
#8171=VERTEX_POINT('',#44166);
#8172=VERTEX_POINT('',#44167);
#8173=VERTEX_POINT('',#44204);
#8174=VERTEX_POINT('',#44205);
#8175=VERTEX_POINT('',#44240);
#8176=VERTEX_POINT('',#44241);
#8177=VERTEX_POINT('',#44278);
#8178=VERTEX_POINT('',#44279);
#8179=VERTEX_POINT('',#44315);
#8180=VERTEX_POINT('',#44316);
#8181=VERTEX_POINT('',#44352);
#8182=VERTEX_POINT('',#44353);
#8183=VERTEX_POINT('',#44390);
#8184=VERTEX_POINT('',#44391);
#8185=VERTEX_POINT('',#44426);
#8186=VERTEX_POINT('',#44427);
#8187=VERTEX_POINT('',#44453);
#8188=VERTEX_POINT('',#44454);
#8189=VERTEX_POINT('',#44477);
#8190=VERTEX_POINT('',#44478);
#8191=VERTEX_POINT('',#44510);
#8192=VERTEX_POINT('',#44511);
#8193=VERTEX_POINT('',#44548);
#8194=VERTEX_POINT('',#44549);
#8195=VERTEX_POINT('',#44584);
#8196=VERTEX_POINT('',#44585);
#8197=VERTEX_POINT('',#44622);
#8198=VERTEX_POINT('',#44623);
#8199=VERTEX_POINT('',#44658);
#8200=VERTEX_POINT('',#44659);
#8201=VERTEX_POINT('',#44696);
#8202=VERTEX_POINT('',#44697);
#8203=VERTEX_POINT('',#44734);
#8204=VERTEX_POINT('',#44735);
#8205=VERTEX_POINT('',#44770);
#8206=VERTEX_POINT('',#44771);
#8207=VERTEX_POINT('',#44808);
#8208=VERTEX_POINT('',#44809);
#8209=VERTEX_POINT('',#44844);
#8210=VERTEX_POINT('',#44845);
#8211=VERTEX_POINT('',#44882);
#8212=VERTEX_POINT('',#44883);
#8213=VERTEX_POINT('',#44920);
#8214=VERTEX_POINT('',#44921);
#8215=VERTEX_POINT('',#44956);
#8216=VERTEX_POINT('',#44957);
#8217=VERTEX_POINT('',#44994);
#8218=VERTEX_POINT('',#44995);
#8219=VERTEX_POINT('',#45030);
#8220=VERTEX_POINT('',#45031);
#8221=VERTEX_POINT('',#45068);
#8222=VERTEX_POINT('',#45069);
#8223=VERTEX_POINT('',#45106);
#8224=VERTEX_POINT('',#45107);
#8225=VERTEX_POINT('',#45142);
#8226=VERTEX_POINT('',#45143);
#8227=VERTEX_POINT('',#45145);
#8228=VERTEX_POINT('',#45152);
#8229=VERTEX_POINT('',#49679);
#8230=VERTEX_POINT('',#52804);
#8231=VERTEX_POINT('',#52807);
#8232=VERTEX_POINT('',#52808);
#8233=VERTEX_POINT('',#52810);
#8234=VERTEX_POINT('',#52812);
#8235=VERTEX_POINT('',#52816);
#8236=VERTEX_POINT('',#52818);
#8237=VERTEX_POINT('',#52822);
#8238=VERTEX_POINT('',#52824);
#8239=VERTEX_POINT('',#52826);
#8240=VERTEX_POINT('',#52828);
#8241=VERTEX_POINT('',#52830);
#8242=VERTEX_POINT('',#52832);
#8243=VERTEX_POINT('',#52834);
#8244=VERTEX_POINT('',#52836);
#8245=VERTEX_POINT('',#52838);
#8246=VERTEX_POINT('',#52840);
#8247=VERTEX_POINT('',#52842);
#8248=VERTEX_POINT('',#52844);
#8249=VERTEX_POINT('',#52846);
#8250=VERTEX_POINT('',#52848);
#8251=VERTEX_POINT('',#52850);
#8252=VERTEX_POINT('',#52852);
#8253=VERTEX_POINT('',#52854);
#8254=VERTEX_POINT('',#52856);
#8255=VERTEX_POINT('',#52858);
#8256=VERTEX_POINT('',#52860);
#8257=VERTEX_POINT('',#52862);
#8258=VERTEX_POINT('',#52864);
#8259=VERTEX_POINT('',#52866);
#8260=VERTEX_POINT('',#52868);
#8261=VERTEX_POINT('',#52870);
#8262=VERTEX_POINT('',#52872);
#8263=VERTEX_POINT('',#52874);
#8264=VERTEX_POINT('',#52876);
#8265=VERTEX_POINT('',#52878);
#8266=VERTEX_POINT('',#52880);
#8267=VERTEX_POINT('',#52882);
#8268=VERTEX_POINT('',#52884);
#8269=VERTEX_POINT('',#52886);
#8270=VERTEX_POINT('',#52888);
#8271=VERTEX_POINT('',#52890);
#8272=VERTEX_POINT('',#52892);
#8273=VERTEX_POINT('',#52894);
#8274=VERTEX_POINT('',#52896);
#8275=VERTEX_POINT('',#52898);
#8276=VERTEX_POINT('',#52900);
#8277=VERTEX_POINT('',#52902);
#8278=VERTEX_POINT('',#52904);
#8279=VERTEX_POINT('',#52906);
#8280=VERTEX_POINT('',#52908);
#8281=VERTEX_POINT('',#52910);
#8282=VERTEX_POINT('',#52912);
#8283=VERTEX_POINT('',#52914);
#8284=VERTEX_POINT('',#52916);
#8285=VERTEX_POINT('',#52918);
#8286=VERTEX_POINT('',#52920);
#8287=VERTEX_POINT('',#52922);
#8288=VERTEX_POINT('',#52924);
#8289=VERTEX_POINT('',#52926);
#8290=VERTEX_POINT('',#52928);
#8291=VERTEX_POINT('',#52930);
#8292=VERTEX_POINT('',#52932);
#8293=VERTEX_POINT('',#52934);
#8294=VERTEX_POINT('',#52936);
#8295=VERTEX_POINT('',#52938);
#8296=VERTEX_POINT('',#52940);
#8297=VERTEX_POINT('',#52942);
#8298=VERTEX_POINT('',#52944);
#8299=VERTEX_POINT('',#52946);
#8300=VERTEX_POINT('',#52948);
#8301=VERTEX_POINT('',#52950);
#8302=VERTEX_POINT('',#52952);
#8303=VERTEX_POINT('',#52954);
#8304=VERTEX_POINT('',#52956);
#8305=VERTEX_POINT('',#52958);
#8306=VERTEX_POINT('',#52961);
#8307=VERTEX_POINT('',#52963);
#8308=VERTEX_POINT('',#52965);
#8309=VERTEX_POINT('',#52967);
#8310=VERTEX_POINT('',#52970);
#8311=VERTEX_POINT('',#52971);
#8312=VERTEX_POINT('',#52976);
#8313=VERTEX_POINT('',#52980);
#8314=VERTEX_POINT('',#52984);
#8315=VERTEX_POINT('',#52988);
#8316=VERTEX_POINT('',#52992);
#8317=VERTEX_POINT('',#52996);
#8318=VERTEX_POINT('',#53000);
#8319=VERTEX_POINT('',#53004);
#8320=VERTEX_POINT('',#53008);
#8321=VERTEX_POINT('',#53010);
#8322=VERTEX_POINT('',#53014);
#8323=VERTEX_POINT('',#53018);
#8324=VERTEX_POINT('',#53022);
#8325=VERTEX_POINT('',#53024);
#8326=VERTEX_POINT('',#53028);
#8327=VERTEX_POINT('',#53032);
#8328=VERTEX_POINT('',#53036);
#8329=VERTEX_POINT('',#53037);
#8330=VERTEX_POINT('',#53042);
#8331=VERTEX_POINT('',#53046);
#8332=VERTEX_POINT('',#53050);
#8333=VERTEX_POINT('',#53054);
#8334=VERTEX_POINT('',#53058);
#8335=VERTEX_POINT('',#53062);
#8336=VERTEX_POINT('',#53066);
#8337=VERTEX_POINT('',#53070);
#8338=VERTEX_POINT('',#53074);
#8339=VERTEX_POINT('',#53076);
#8340=VERTEX_POINT('',#53080);
#8341=VERTEX_POINT('',#53084);
#8342=VERTEX_POINT('',#53088);
#8343=VERTEX_POINT('',#53090);
#8344=VERTEX_POINT('',#53094);
#8345=VERTEX_POINT('',#53098);
#8346=VERTEX_POINT('',#53102);
#8347=VERTEX_POINT('',#53103);
#8348=VERTEX_POINT('',#53108);
#8349=VERTEX_POINT('',#53112);
#8350=VERTEX_POINT('',#53116);
#8351=VERTEX_POINT('',#53120);
#8352=VERTEX_POINT('',#53124);
#8353=VERTEX_POINT('',#53128);
#8354=VERTEX_POINT('',#53132);
#8355=VERTEX_POINT('',#53136);
#8356=VERTEX_POINT('',#53140);
#8357=VERTEX_POINT('',#53142);
#8358=VERTEX_POINT('',#53146);
#8359=VERTEX_POINT('',#53150);
#8360=VERTEX_POINT('',#53154);
#8361=VERTEX_POINT('',#53156);
#8362=VERTEX_POINT('',#53160);
#8363=VERTEX_POINT('',#53164);
#8364=VERTEX_POINT('',#53168);
#8365=VERTEX_POINT('',#53169);
#8366=VERTEX_POINT('',#53174);
#8367=VERTEX_POINT('',#53178);
#8368=VERTEX_POINT('',#53182);
#8369=VERTEX_POINT('',#53186);
#8370=VERTEX_POINT('',#53190);
#8371=VERTEX_POINT('',#53194);
#8372=VERTEX_POINT('',#53198);
#8373=VERTEX_POINT('',#53202);
#8374=VERTEX_POINT('',#53206);
#8375=VERTEX_POINT('',#53208);
#8376=VERTEX_POINT('',#53212);
#8377=VERTEX_POINT('',#53216);
#8378=VERTEX_POINT('',#53220);
#8379=VERTEX_POINT('',#53224);
#8380=VERTEX_POINT('',#53228);
#8381=VERTEX_POINT('',#53234);
#8382=VERTEX_POINT('',#53238);
#10317=EDGE_CURVE('',#7949,#7950,#5136,.T.);
#10318=EDGE_CURVE('',#7950,#7951,#641,.T.);
#10319=EDGE_CURVE('',#7951,#7952,#7403,.T.);
#10320=EDGE_CURVE('',#7952,#7953,#5137,.T.);
#10321=EDGE_CURVE('',#7953,#7953,#7404,.F.);
#10322=EDGE_CURVE('',#7952,#7954,#7405,.T.);
#10323=EDGE_CURVE('',#7954,#7949,#642,.T.);
#10324=EDGE_CURVE('',#7955,#7956,#5138,.T.);
#10325=EDGE_CURVE('',#7956,#7950,#643,.T.);
#10326=EDGE_CURVE('',#7949,#7955,#644,.T.);
#10327=EDGE_CURVE('',#7957,#7958,#5139,.T.);
#10328=EDGE_CURVE('',#7958,#7956,#645,.T.);
#10329=EDGE_CURVE('',#7955,#7957,#646,.T.);
#10330=EDGE_CURVE('',#7959,#7960,#5140,.T.);
#10331=EDGE_CURVE('',#7960,#7958,#647,.T.);
#10332=EDGE_CURVE('',#7957,#7959,#648,.T.);
#10333=EDGE_CURVE('',#7961,#7962,#5141,.T.);
#10334=EDGE_CURVE('',#7962,#7960,#649,.T.);
#10335=EDGE_CURVE('',#7959,#7961,#650,.T.);
#10336=EDGE_CURVE('',#7963,#7964,#5142,.T.);
#10337=EDGE_CURVE('',#7964,#7962,#651,.T.);
#10338=EDGE_CURVE('',#7961,#7963,#652,.T.);
#10339=EDGE_CURVE('',#7965,#7966,#5143,.T.);
#10340=EDGE_CURVE('',#7966,#7964,#653,.T.);
#10341=EDGE_CURVE('',#7963,#7965,#654,.T.);
#10342=EDGE_CURVE('',#7967,#7968,#5144,.T.);
#10343=EDGE_CURVE('',#7968,#7966,#655,.T.);
#10344=EDGE_CURVE('',#7965,#7967,#656,.T.);
#10345=EDGE_CURVE('',#7969,#7970,#5145,.T.);
#10346=EDGE_CURVE('',#7970,#7968,#657,.T.);
#10347=EDGE_CURVE('',#7967,#7969,#658,.T.);
#10348=EDGE_CURVE('',#7971,#7972,#5146,.T.);
#10349=EDGE_CURVE('',#7972,#7970,#659,.T.);
#10350=EDGE_CURVE('',#7969,#7971,#660,.T.);
#10351=EDGE_CURVE('',#7973,#7974,#5147,.T.);
#10352=EDGE_CURVE('',#7974,#7972,#661,.T.);
#10353=EDGE_CURVE('',#7971,#7973,#662,.T.);
#10354=EDGE_CURVE('',#7975,#7976,#5148,.T.);
#10355=EDGE_CURVE('',#7976,#7974,#663,.T.);
#10356=EDGE_CURVE('',#7973,#7975,#664,.T.);
#10357=EDGE_CURVE('',#7977,#7978,#5149,.T.);
#10358=EDGE_CURVE('',#7978,#7976,#665,.T.);
#10359=EDGE_CURVE('',#7975,#7977,#666,.T.);
#10360=EDGE_CURVE('',#7979,#7980,#5150,.T.);
#10361=EDGE_CURVE('',#7980,#7978,#667,.T.);
#10362=EDGE_CURVE('',#7977,#7979,#668,.T.);
#10363=EDGE_CURVE('',#7981,#7982,#5151,.T.);
#10364=EDGE_CURVE('',#7982,#7980,#669,.T.);
#10365=EDGE_CURVE('',#7979,#7981,#670,.T.);
#10366=EDGE_CURVE('',#7983,#7984,#5152,.T.);
#10367=EDGE_CURVE('',#7984,#7982,#671,.T.);
#10368=EDGE_CURVE('',#7981,#7983,#672,.T.);
#10369=EDGE_CURVE('',#7985,#7986,#5153,.T.);
#10370=EDGE_CURVE('',#7986,#7984,#673,.T.);
#10371=EDGE_CURVE('',#7983,#7985,#674,.T.);
#10372=EDGE_CURVE('',#7987,#7988,#5154,.T.);
#10373=EDGE_CURVE('',#7988,#7986,#675,.T.);
#10374=EDGE_CURVE('',#7985,#7987,#676,.T.);
#10375=EDGE_CURVE('',#7989,#7990,#5155,.T.);
#10376=EDGE_CURVE('',#7990,#7988,#677,.T.);
#10377=EDGE_CURVE('',#7987,#7989,#678,.T.);
#10378=EDGE_CURVE('',#7991,#7992,#5156,.T.);
#10379=EDGE_CURVE('',#7992,#7990,#679,.T.);
#10380=EDGE_CURVE('',#7989,#7991,#680,.T.);
#10381=EDGE_CURVE('',#7993,#7994,#5157,.T.);
#10382=EDGE_CURVE('',#7994,#7992,#681,.T.);
#10383=EDGE_CURVE('',#7991,#7993,#682,.T.);
#10384=EDGE_CURVE('',#7995,#7996,#5158,.T.);
#10385=EDGE_CURVE('',#7996,#7994,#683,.T.);
#10386=EDGE_CURVE('',#7993,#7995,#684,.T.);
#10387=EDGE_CURVE('',#7997,#7998,#5159,.T.);
#10388=EDGE_CURVE('',#7998,#7996,#685,.T.);
#10389=EDGE_CURVE('',#7995,#7997,#686,.T.);
#10390=EDGE_CURVE('',#7999,#8000,#5160,.T.);
#10391=EDGE_CURVE('',#8000,#7998,#687,.T.);
#10392=EDGE_CURVE('',#7997,#7999,#688,.T.);
#10393=EDGE_CURVE('',#8001,#8002,#5161,.T.);
#10394=EDGE_CURVE('',#8001,#8003,#689,.T.);
#10395=EDGE_CURVE('',#8004,#8003,#7406,.T.);
#10396=EDGE_CURVE('',#8004,#8002,#690,.T.);
#10397=EDGE_CURVE('',#8005,#8006,#5162,.T.);
#10398=EDGE_CURVE('',#8006,#8007,#691,.T.);
#10399=EDGE_CURVE('',#8008,#8007,#7407,.T.);
#10400=EDGE_CURVE('',#8005,#8008,#692,.T.);
#10401=EDGE_CURVE('',#8009,#8010,#5163,.T.);
#10402=EDGE_CURVE('',#8010,#8006,#693,.T.);
#10403=EDGE_CURVE('',#8009,#8005,#694,.T.);
#10404=EDGE_CURVE('',#8011,#8012,#5164,.T.);
#10405=EDGE_CURVE('',#8012,#8010,#695,.T.);
#10406=EDGE_CURVE('',#8011,#8009,#696,.T.);
#10407=EDGE_CURVE('',#8013,#8014,#5165,.T.);
#10408=EDGE_CURVE('',#8014,#8012,#697,.T.);
#10409=EDGE_CURVE('',#8013,#8011,#698,.T.);
#10410=EDGE_CURVE('',#8015,#8016,#5166,.T.);
#10411=EDGE_CURVE('',#8016,#8014,#699,.T.);
#10412=EDGE_CURVE('',#8015,#8013,#700,.T.);
#10413=EDGE_CURVE('',#8017,#8018,#5167,.T.);
#10414=EDGE_CURVE('',#8018,#8016,#701,.T.);
#10415=EDGE_CURVE('',#8017,#8015,#702,.T.);
#10416=EDGE_CURVE('',#8019,#8020,#5168,.T.);
#10417=EDGE_CURVE('',#8020,#8018,#703,.T.);
#10418=EDGE_CURVE('',#8019,#8017,#704,.T.);
#10419=EDGE_CURVE('',#8021,#8022,#5169,.T.);
#10420=EDGE_CURVE('',#8022,#8020,#705,.T.);
#10421=EDGE_CURVE('',#8021,#8019,#706,.T.);
#10422=EDGE_CURVE('',#8023,#8024,#5170,.T.);
#10423=EDGE_CURVE('',#8024,#8022,#707,.T.);
#10424=EDGE_CURVE('',#8023,#8021,#708,.T.);
#10425=EDGE_CURVE('',#8025,#8026,#5171,.T.);
#10426=EDGE_CURVE('',#8026,#8024,#709,.T.);
#10427=EDGE_CURVE('',#8025,#8023,#710,.T.);
#10428=EDGE_CURVE('',#8027,#8028,#5172,.T.);
#10429=EDGE_CURVE('',#8028,#8026,#711,.T.);
#10430=EDGE_CURVE('',#8027,#8025,#712,.T.);
#10431=EDGE_CURVE('',#8029,#8030,#5173,.T.);
#10432=EDGE_CURVE('',#8030,#8028,#713,.T.);
#10433=EDGE_CURVE('',#8029,#8027,#714,.T.);
#10434=EDGE_CURVE('',#8031,#8032,#5174,.T.);
#10435=EDGE_CURVE('',#8032,#8030,#715,.T.);
#10436=EDGE_CURVE('',#8031,#8029,#716,.T.);
#10437=EDGE_CURVE('',#8033,#8034,#5175,.T.);
#10438=EDGE_CURVE('',#8034,#8032,#717,.T.);
#10439=EDGE_CURVE('',#8033,#8031,#718,.T.);
#10440=EDGE_CURVE('',#8035,#8036,#5176,.T.);
#10441=EDGE_CURVE('',#8036,#8034,#719,.T.);
#10442=EDGE_CURVE('',#8035,#8033,#720,.T.);
#10443=EDGE_CURVE('',#8037,#8038,#5177,.T.);
#10444=EDGE_CURVE('',#8038,#8036,#721,.T.);
#10445=EDGE_CURVE('',#8037,#8035,#722,.T.);
#10446=EDGE_CURVE('',#8039,#8040,#5178,.T.);
#10447=EDGE_CURVE('',#8040,#8038,#723,.T.);
#10448=EDGE_CURVE('',#8039,#8037,#724,.T.);
#10449=EDGE_CURVE('',#8041,#8042,#5179,.T.);
#10450=EDGE_CURVE('',#8042,#8040,#725,.T.);
#10451=EDGE_CURVE('',#8041,#8039,#726,.T.);
#10452=EDGE_CURVE('',#8043,#8044,#5180,.T.);
#10453=EDGE_CURVE('',#8044,#8042,#727,.T.);
#10454=EDGE_CURVE('',#8043,#8041,#728,.T.);
#10455=EDGE_CURVE('',#8045,#8046,#5181,.T.);
#10456=EDGE_CURVE('',#8046,#8044,#729,.T.);
#10457=EDGE_CURVE('',#8045,#8043,#730,.T.);
#10458=EDGE_CURVE('',#8047,#8048,#5182,.T.);
#10459=EDGE_CURVE('',#8048,#8046,#731,.T.);
#10460=EDGE_CURVE('',#8047,#8045,#732,.T.);
#10461=EDGE_CURVE('',#8049,#8050,#5183,.T.);
#10462=EDGE_CURVE('',#8050,#8048,#733,.T.);
#10463=EDGE_CURVE('',#8049,#8047,#734,.T.);
#10464=EDGE_CURVE('',#8051,#8052,#5184,.T.);
#10465=EDGE_CURVE('',#8052,#8050,#735,.T.);
#10466=EDGE_CURVE('',#8051,#8049,#736,.T.);
#10467=EDGE_CURVE('',#8053,#8054,#5185,.T.);
#10468=EDGE_CURVE('',#8054,#8052,#737,.T.);
#10469=EDGE_CURVE('',#8053,#8051,#738,.T.);
#10470=EDGE_CURVE('',#8055,#8056,#5186,.T.);
#10471=EDGE_CURVE('',#8057,#8055,#739,.T.);
#10472=EDGE_CURVE('',#8058,#8057,#7408,.T.);
#10473=EDGE_CURVE('',#8058,#8056,#740,.T.);
#10474=EDGE_CURVE('',#8059,#8060,#5187,.T.);
#10475=EDGE_CURVE('',#8060,#8061,#741,.T.);
#10476=EDGE_CURVE('',#8061,#8062,#7409,.T.);
#10477=EDGE_CURVE('',#8062,#8063,#5188,.T.);
#10478=EDGE_CURVE('',#8063,#8063,#7410,.F.);
#10479=EDGE_CURVE('',#8062,#8064,#7411,.T.);
#10480=EDGE_CURVE('',#8064,#8059,#742,.T.);
#10481=EDGE_CURVE('',#8065,#8066,#5189,.T.);
#10482=EDGE_CURVE('',#8066,#8060,#743,.T.);
#10483=EDGE_CURVE('',#8059,#8065,#744,.T.);
#10484=EDGE_CURVE('',#8067,#8068,#5190,.T.);
#10485=EDGE_CURVE('',#8068,#8066,#745,.T.);
#10486=EDGE_CURVE('',#8065,#8067,#746,.T.);
#10487=EDGE_CURVE('',#8069,#8070,#5191,.T.);
#10488=EDGE_CURVE('',#8070,#8068,#747,.T.);
#10489=EDGE_CURVE('',#8067,#8069,#748,.T.);
#10490=EDGE_CURVE('',#8071,#8072,#5192,.T.);
#10491=EDGE_CURVE('',#8072,#8070,#749,.T.);
#10492=EDGE_CURVE('',#8069,#8071,#750,.T.);
#10493=EDGE_CURVE('',#8073,#8074,#5193,.T.);
#10494=EDGE_CURVE('',#8074,#8072,#751,.T.);
#10495=EDGE_CURVE('',#8071,#8073,#752,.T.);
#10496=EDGE_CURVE('',#8075,#8076,#5194,.T.);
#10497=EDGE_CURVE('',#8076,#8074,#753,.T.);
#10498=EDGE_CURVE('',#8073,#8075,#754,.T.);
#10499=EDGE_CURVE('',#8077,#8078,#5195,.T.);
#10500=EDGE_CURVE('',#8078,#8076,#755,.T.);
#10501=EDGE_CURVE('',#8075,#8077,#756,.T.);
#10502=EDGE_CURVE('',#8079,#8080,#5196,.T.);
#10503=EDGE_CURVE('',#8080,#8078,#757,.T.);
#10504=EDGE_CURVE('',#8077,#8079,#758,.T.);
#10505=EDGE_CURVE('',#8081,#8082,#5197,.T.);
#10506=EDGE_CURVE('',#8082,#8080,#759,.T.);
#10507=EDGE_CURVE('',#8079,#8081,#760,.T.);
#10508=EDGE_CURVE('',#8083,#8084,#5198,.T.);
#10509=EDGE_CURVE('',#8084,#8082,#761,.T.);
#10510=EDGE_CURVE('',#8081,#8083,#762,.T.);
#10511=EDGE_CURVE('',#8085,#8086,#5199,.T.);
#10512=EDGE_CURVE('',#8086,#8084,#763,.T.);
#10513=EDGE_CURVE('',#8083,#8085,#764,.T.);
#10514=EDGE_CURVE('',#8087,#8088,#5200,.T.);
#10515=EDGE_CURVE('',#8088,#8086,#765,.T.);
#10516=EDGE_CURVE('',#8085,#8087,#766,.T.);
#10517=EDGE_CURVE('',#8089,#8090,#5201,.T.);
#10518=EDGE_CURVE('',#8090,#8088,#767,.T.);
#10519=EDGE_CURVE('',#8087,#8089,#768,.T.);
#10520=EDGE_CURVE('',#8091,#8092,#5202,.T.);
#10521=EDGE_CURVE('',#8092,#8090,#769,.T.);
#10522=EDGE_CURVE('',#8089,#8091,#770,.T.);
#10523=EDGE_CURVE('',#8093,#8094,#5203,.T.);
#10524=EDGE_CURVE('',#8094,#8092,#771,.T.);
#10525=EDGE_CURVE('',#8091,#8093,#772,.T.);
#10526=EDGE_CURVE('',#8095,#8096,#5204,.T.);
#10527=EDGE_CURVE('',#8096,#8094,#773,.T.);
#10528=EDGE_CURVE('',#8093,#8095,#774,.T.);
#10529=EDGE_CURVE('',#8097,#8098,#5205,.T.);
#10530=EDGE_CURVE('',#8098,#8096,#775,.T.);
#10531=EDGE_CURVE('',#8095,#8097,#776,.T.);
#10532=EDGE_CURVE('',#8099,#8100,#5206,.T.);
#10533=EDGE_CURVE('',#8100,#8098,#777,.T.);
#10534=EDGE_CURVE('',#8097,#8099,#778,.T.);
#10535=EDGE_CURVE('',#8101,#8102,#5207,.T.);
#10536=EDGE_CURVE('',#8102,#8100,#779,.T.);
#10537=EDGE_CURVE('',#8099,#8101,#780,.T.);
#10538=EDGE_CURVE('',#8103,#8104,#5208,.T.);
#10539=EDGE_CURVE('',#8104,#8102,#781,.T.);
#10540=EDGE_CURVE('',#8101,#8103,#782,.T.);
#10541=EDGE_CURVE('',#8105,#8106,#5209,.T.);
#10542=EDGE_CURVE('',#8106,#8104,#783,.T.);
#10543=EDGE_CURVE('',#8103,#8105,#784,.T.);
#10544=EDGE_CURVE('',#8107,#8108,#5210,.T.);
#10545=EDGE_CURVE('',#8108,#8106,#785,.T.);
#10546=EDGE_CURVE('',#8105,#8107,#786,.T.);
#10547=EDGE_CURVE('',#8109,#8110,#5211,.T.);
#10548=EDGE_CURVE('',#8110,#8108,#787,.T.);
#10549=EDGE_CURVE('',#8107,#8109,#788,.T.);
#10550=EDGE_CURVE('',#8111,#8112,#5212,.T.);
#10551=EDGE_CURVE('',#8112,#8110,#789,.T.);
#10552=EDGE_CURVE('',#8109,#8111,#790,.T.);
#10553=EDGE_CURVE('',#8113,#8114,#5213,.T.);
#10554=EDGE_CURVE('',#8114,#8112,#791,.T.);
#10555=EDGE_CURVE('',#8111,#8113,#792,.T.);
#10556=EDGE_CURVE('',#8115,#8116,#5214,.T.);
#10557=EDGE_CURVE('',#8116,#8114,#793,.T.);
#10558=EDGE_CURVE('',#8113,#8115,#794,.T.);
#10559=EDGE_CURVE('',#8117,#8118,#5215,.T.);
#10560=EDGE_CURVE('',#8118,#8116,#795,.T.);
#10561=EDGE_CURVE('',#8115,#8117,#796,.T.);
#10562=EDGE_CURVE('',#8119,#8120,#5216,.T.);
#10563=EDGE_CURVE('',#8120,#8118,#797,.T.);
#10564=EDGE_CURVE('',#8117,#8119,#798,.T.);
#10565=EDGE_CURVE('',#8121,#8122,#5217,.T.);
#10566=EDGE_CURVE('',#8122,#8120,#799,.T.);
#10567=EDGE_CURVE('',#8119,#8121,#800,.T.);
#10568=EDGE_CURVE('',#8123,#8124,#5218,.T.);
#10569=EDGE_CURVE('',#8124,#8122,#801,.T.);
#10570=EDGE_CURVE('',#8121,#8123,#802,.T.);
#10571=EDGE_CURVE('',#8125,#8126,#5219,.T.);
#10572=EDGE_CURVE('',#8126,#8124,#803,.T.);
#10573=EDGE_CURVE('',#8123,#8125,#804,.T.);
#10574=EDGE_CURVE('',#8127,#8128,#5220,.T.);
#10575=EDGE_CURVE('',#8128,#8126,#805,.T.);
#10576=EDGE_CURVE('',#8125,#8127,#806,.T.);
#10577=EDGE_CURVE('',#8129,#8130,#5221,.T.);
#10578=EDGE_CURVE('',#8130,#8128,#807,.T.);
#10579=EDGE_CURVE('',#8127,#8129,#808,.T.);
#10580=EDGE_CURVE('',#8131,#8132,#5222,.T.);
#10581=EDGE_CURVE('',#8132,#8130,#809,.T.);
#10582=EDGE_CURVE('',#8129,#8131,#810,.T.);
#10583=EDGE_CURVE('',#8133,#8134,#5223,.T.);
#10584=EDGE_CURVE('',#8134,#8132,#811,.T.);
#10585=EDGE_CURVE('',#8131,#8133,#812,.T.);
#10586=EDGE_CURVE('',#8135,#8136,#5224,.T.);
#10587=EDGE_CURVE('',#8136,#8134,#813,.T.);
#10588=EDGE_CURVE('',#8133,#8135,#814,.T.);
#10589=EDGE_CURVE('',#8137,#8138,#5225,.T.);
#10590=EDGE_CURVE('',#8138,#8136,#815,.T.);
#10591=EDGE_CURVE('',#8135,#8137,#816,.T.);
#10592=EDGE_CURVE('',#8139,#8140,#5226,.T.);
#10593=EDGE_CURVE('',#8140,#8138,#817,.T.);
#10594=EDGE_CURVE('',#8137,#8139,#818,.T.);
#10595=EDGE_CURVE('',#8141,#8142,#5227,.T.);
#10596=EDGE_CURVE('',#8141,#8143,#819,.T.);
#10597=EDGE_CURVE('',#8144,#8143,#7412,.F.);
#10598=EDGE_CURVE('',#8144,#8142,#820,.T.);
#10599=EDGE_CURVE('',#8145,#8146,#5228,.T.);
#10600=EDGE_CURVE('',#8146,#8147,#821,.T.);
#10601=EDGE_CURVE('',#8148,#8147,#7413,.T.);
#10602=EDGE_CURVE('',#8145,#8148,#822,.T.);
#10603=EDGE_CURVE('',#8149,#8150,#5229,.T.);
#10604=EDGE_CURVE('',#8150,#8146,#823,.T.);
#10605=EDGE_CURVE('',#8149,#8145,#824,.T.);
#10606=EDGE_CURVE('',#8151,#8152,#5230,.T.);
#10607=EDGE_CURVE('',#8152,#8150,#825,.T.);
#10608=EDGE_CURVE('',#8151,#8149,#826,.T.);
#10609=EDGE_CURVE('',#8153,#8154,#5231,.T.);
#10610=EDGE_CURVE('',#8154,#8152,#827,.T.);
#10611=EDGE_CURVE('',#8153,#8151,#828,.T.);
#10612=EDGE_CURVE('',#8155,#8156,#5232,.T.);
#10613=EDGE_CURVE('',#8156,#8154,#829,.T.);
#10614=EDGE_CURVE('',#8155,#8153,#830,.T.);
#10615=EDGE_CURVE('',#8157,#8158,#5233,.T.);
#10616=EDGE_CURVE('',#8158,#8156,#831,.T.);
#10617=EDGE_CURVE('',#8157,#8155,#832,.T.);
#10618=EDGE_CURVE('',#8159,#8160,#5234,.T.);
#10619=EDGE_CURVE('',#8160,#8158,#833,.T.);
#10620=EDGE_CURVE('',#8159,#8157,#834,.T.);
#10621=EDGE_CURVE('',#8161,#8162,#5235,.T.);
#10622=EDGE_CURVE('',#8162,#8160,#835,.T.);
#10623=EDGE_CURVE('',#8161,#8159,#836,.T.);
#10624=EDGE_CURVE('',#8163,#8164,#5236,.T.);
#10625=EDGE_CURVE('',#8164,#8162,#837,.T.);
#10626=EDGE_CURVE('',#8163,#8161,#838,.T.);
#10627=EDGE_CURVE('',#8165,#8166,#5237,.T.);
#10628=EDGE_CURVE('',#8166,#8164,#839,.T.);
#10629=EDGE_CURVE('',#8165,#8163,#840,.T.);
#10630=EDGE_CURVE('',#8167,#8168,#5238,.T.);
#10631=EDGE_CURVE('',#8168,#8166,#841,.T.);
#10632=EDGE_CURVE('',#8167,#8165,#842,.T.);
#10633=EDGE_CURVE('',#8169,#8170,#5239,.T.);
#10634=EDGE_CURVE('',#8170,#8168,#843,.T.);
#10635=EDGE_CURVE('',#8169,#8167,#844,.T.);
#10636=EDGE_CURVE('',#8171,#8172,#5240,.T.);
#10637=EDGE_CURVE('',#8172,#8170,#845,.T.);
#10638=EDGE_CURVE('',#8171,#8169,#846,.T.);
#10639=EDGE_CURVE('',#8173,#8174,#5241,.T.);
#10640=EDGE_CURVE('',#8174,#8172,#847,.T.);
#10641=EDGE_CURVE('',#8173,#8171,#848,.T.);
#10642=EDGE_CURVE('',#8175,#8176,#5242,.T.);
#10643=EDGE_CURVE('',#8176,#8174,#849,.T.);
#10644=EDGE_CURVE('',#8175,#8173,#850,.T.);
#10645=EDGE_CURVE('',#8177,#8178,#5243,.T.);
#10646=EDGE_CURVE('',#8178,#8176,#851,.T.);
#10647=EDGE_CURVE('',#8177,#8175,#852,.T.);
#10648=EDGE_CURVE('',#8179,#8180,#5244,.T.);
#10649=EDGE_CURVE('',#8180,#8178,#853,.T.);
#10650=EDGE_CURVE('',#8179,#8177,#854,.T.);
#10651=EDGE_CURVE('',#8181,#8182,#5245,.T.);
#10652=EDGE_CURVE('',#8182,#8180,#855,.T.);
#10653=EDGE_CURVE('',#8181,#8179,#856,.T.);
#10654=EDGE_CURVE('',#8183,#8184,#5246,.T.);
#10655=EDGE_CURVE('',#8184,#8182,#857,.T.);
#10656=EDGE_CURVE('',#8183,#8181,#858,.T.);
#10657=EDGE_CURVE('',#8185,#8186,#5247,.T.);
#10658=EDGE_CURVE('',#8186,#8184,#859,.T.);
#10659=EDGE_CURVE('',#8185,#8183,#860,.T.);
#10660=EDGE_CURVE('',#8187,#8188,#5248,.T.);
#10661=EDGE_CURVE('',#8188,#8186,#861,.T.);
#10662=EDGE_CURVE('',#8187,#8185,#862,.T.);
#10663=EDGE_CURVE('',#8189,#8190,#5249,.T.);
#10664=EDGE_CURVE('',#8190,#8188,#863,.T.);
#10665=EDGE_CURVE('',#8189,#8187,#864,.T.);
#10666=EDGE_CURVE('',#8191,#8192,#5250,.T.);
#10667=EDGE_CURVE('',#8192,#8190,#865,.T.);
#10668=EDGE_CURVE('',#8191,#8189,#866,.T.);
#10669=EDGE_CURVE('',#8193,#8194,#5251,.T.);
#10670=EDGE_CURVE('',#8194,#8192,#867,.T.);
#10671=EDGE_CURVE('',#8193,#8191,#868,.T.);
#10672=EDGE_CURVE('',#8195,#8196,#5252,.T.);
#10673=EDGE_CURVE('',#8196,#8194,#869,.T.);
#10674=EDGE_CURVE('',#8195,#8193,#870,.T.);
#10675=EDGE_CURVE('',#8197,#8198,#5253,.T.);
#10676=EDGE_CURVE('',#8198,#8196,#871,.T.);
#10677=EDGE_CURVE('',#8197,#8195,#872,.T.);
#10678=EDGE_CURVE('',#8199,#8200,#5254,.T.);
#10679=EDGE_CURVE('',#8200,#8198,#873,.T.);
#10680=EDGE_CURVE('',#8199,#8197,#874,.T.);
#10681=EDGE_CURVE('',#8201,#8202,#5255,.T.);
#10682=EDGE_CURVE('',#8202,#8200,#875,.T.);
#10683=EDGE_CURVE('',#8201,#8199,#876,.T.);
#10684=EDGE_CURVE('',#8203,#8204,#5256,.T.);
#10685=EDGE_CURVE('',#8204,#8202,#877,.T.);
#10686=EDGE_CURVE('',#8203,#8201,#878,.T.);
#10687=EDGE_CURVE('',#8205,#8206,#5257,.T.);
#10688=EDGE_CURVE('',#8206,#8204,#879,.T.);
#10689=EDGE_CURVE('',#8205,#8203,#880,.T.);
#10690=EDGE_CURVE('',#8207,#8208,#5258,.T.);
#10691=EDGE_CURVE('',#8208,#8206,#881,.T.);
#10692=EDGE_CURVE('',#8207,#8205,#882,.T.);
#10693=EDGE_CURVE('',#8209,#8210,#5259,.T.);
#10694=EDGE_CURVE('',#8210,#8208,#883,.T.);
#10695=EDGE_CURVE('',#8209,#8207,#884,.T.);
#10696=EDGE_CURVE('',#8211,#8212,#5260,.T.);
#10697=EDGE_CURVE('',#8212,#8210,#885,.T.);
#10698=EDGE_CURVE('',#8211,#8209,#886,.T.);
#10699=EDGE_CURVE('',#8213,#8214,#5261,.T.);
#10700=EDGE_CURVE('',#8214,#8212,#887,.T.);
#10701=EDGE_CURVE('',#8213,#8211,#888,.T.);
#10702=EDGE_CURVE('',#8215,#8216,#5262,.T.);
#10703=EDGE_CURVE('',#8216,#8214,#889,.T.);
#10704=EDGE_CURVE('',#8215,#8213,#890,.T.);
#10705=EDGE_CURVE('',#8217,#8218,#5263,.T.);
#10706=EDGE_CURVE('',#8218,#8216,#891,.T.);
#10707=EDGE_CURVE('',#8217,#8215,#892,.T.);
#10708=EDGE_CURVE('',#8219,#8220,#5264,.T.);
#10709=EDGE_CURVE('',#8220,#8218,#893,.T.);
#10710=EDGE_CURVE('',#8219,#8217,#894,.T.);
#10711=EDGE_CURVE('',#8221,#8222,#5265,.T.);
#10712=EDGE_CURVE('',#8222,#8220,#895,.T.);
#10713=EDGE_CURVE('',#8221,#8219,#896,.T.);
#10714=EDGE_CURVE('',#8223,#8224,#5266,.T.);
#10715=EDGE_CURVE('',#8224,#8222,#897,.T.);
#10716=EDGE_CURVE('',#8223,#8221,#898,.T.);
#10717=EDGE_CURVE('',#8225,#8226,#5267,.T.);
#10718=EDGE_CURVE('',#8227,#8225,#899,.T.);
#10719=EDGE_CURVE('',#8228,#8227,#7414,.T.);
#10720=EDGE_CURVE('',#8228,#8226,#900,.T.);
#10721=EDGE_CURVE('',#8061,#8148,#901,.T.);
#10722=EDGE_CURVE('',#8147,#8064,#902,.T.);
#10723=EDGE_CURVE('',#8226,#8224,#903,.T.);
#10724=EDGE_CURVE('',#8225,#8223,#904,.T.);
#10725=EDGE_CURVE('',#8143,#8228,#905,.T.);
#10726=EDGE_CURVE('',#8139,#8141,#906,.T.);
#10727=EDGE_CURVE('',#8142,#8140,#907,.T.);
#10728=EDGE_CURVE('',#8227,#8144,#908,.T.);
#10729=EDGE_CURVE('',#8229,#8229,#7415,.T.);
#10730=EDGE_CURVE('',#7951,#8008,#909,.T.);
#10731=EDGE_CURVE('',#8007,#7954,#910,.T.);
#10732=EDGE_CURVE('',#8056,#8054,#911,.T.);
#10733=EDGE_CURVE('',#8055,#8053,#912,.T.);
#10734=EDGE_CURVE('',#8003,#8058,#913,.T.);
#10735=EDGE_CURVE('',#7999,#8001,#914,.T.);
#10736=EDGE_CURVE('',#8002,#8000,#915,.T.);
#10737=EDGE_CURVE('',#8057,#8004,#916,.T.);
#10738=EDGE_CURVE('',#8230,#8230,#7416,.T.);
#10739=EDGE_CURVE('',#8231,#8232,#7417,.T.);
#10740=EDGE_CURVE('',#8232,#8233,#5268,.T.);
#10741=EDGE_CURVE('',#8233,#8234,#7418,.T.);
#10742=EDGE_CURVE('',#8234,#8231,#5269,.T.);
#10743=EDGE_CURVE('',#8235,#8232,#5270,.T.);
#10744=EDGE_CURVE('',#8236,#8235,#5271,.T.);
#10745=EDGE_CURVE('',#8233,#8236,#5272,.T.);
#10746=EDGE_CURVE('',#8231,#8237,#5273,.T.);
#10747=EDGE_CURVE('',#8238,#8237,#7419,.T.);
#10748=EDGE_CURVE('',#8238,#8239,#5274,.T.);
#10749=EDGE_CURVE('',#8240,#8239,#7420,.T.);
#10750=EDGE_CURVE('',#8240,#8241,#5275,.T.);
#10751=EDGE_CURVE('',#8242,#8241,#7421,.T.);
#10752=EDGE_CURVE('',#8242,#8243,#5276,.T.);
#10753=EDGE_CURVE('',#8244,#8243,#7422,.T.);
#10754=EDGE_CURVE('',#8244,#8245,#5277,.T.);
#10755=EDGE_CURVE('',#8246,#8245,#7423,.T.);
#10756=EDGE_CURVE('',#8246,#8247,#5278,.T.);
#10757=EDGE_CURVE('',#8248,#8247,#7424,.T.);
#10758=EDGE_CURVE('',#8248,#8249,#5279,.T.);
#10759=EDGE_CURVE('',#8250,#8249,#7425,.T.);
#10760=EDGE_CURVE('',#8250,#8251,#5280,.T.);
#10761=EDGE_CURVE('',#8252,#8251,#7426,.T.);
#10762=EDGE_CURVE('',#8252,#8253,#5281,.T.);
#10763=EDGE_CURVE('',#8254,#8253,#7427,.T.);
#10764=EDGE_CURVE('',#8254,#8255,#5282,.T.);
#10765=EDGE_CURVE('',#8256,#8255,#7428,.T.);
#10766=EDGE_CURVE('',#8256,#8257,#5283,.T.);
#10767=EDGE_CURVE('',#8258,#8257,#7429,.T.);
#10768=EDGE_CURVE('',#8258,#8259,#5284,.T.);
#10769=EDGE_CURVE('',#8260,#8259,#7430,.T.);
#10770=EDGE_CURVE('',#8260,#8261,#5285,.T.);
#10771=EDGE_CURVE('',#8262,#8261,#7431,.T.);
#10772=EDGE_CURVE('',#8262,#8263,#5286,.T.);
#10773=EDGE_CURVE('',#8264,#8263,#7432,.T.);
#10774=EDGE_CURVE('',#8264,#8265,#5287,.T.);
#10775=EDGE_CURVE('',#8266,#8265,#7433,.T.);
#10776=EDGE_CURVE('',#8266,#8267,#5288,.T.);
#10777=EDGE_CURVE('',#8268,#8267,#7434,.T.);
#10778=EDGE_CURVE('',#8268,#8269,#5289,.T.);
#10779=EDGE_CURVE('',#8270,#8269,#7435,.T.);
#10780=EDGE_CURVE('',#8270,#8271,#5290,.T.);
#10781=EDGE_CURVE('',#8272,#8271,#7436,.T.);
#10782=EDGE_CURVE('',#8272,#8273,#5291,.T.);
#10783=EDGE_CURVE('',#8274,#8273,#7437,.T.);
#10784=EDGE_CURVE('',#8274,#8275,#5292,.T.);
#10785=EDGE_CURVE('',#8276,#8275,#7438,.T.);
#10786=EDGE_CURVE('',#8276,#8277,#5293,.T.);
#10787=EDGE_CURVE('',#8278,#8277,#7439,.T.);
#10788=EDGE_CURVE('',#8278,#8279,#5294,.T.);
#10789=EDGE_CURVE('',#8280,#8279,#7440,.T.);
#10790=EDGE_CURVE('',#8280,#8281,#5295,.T.);
#10791=EDGE_CURVE('',#8282,#8281,#7441,.T.);
#10792=EDGE_CURVE('',#8282,#8283,#5296,.T.);
#10793=EDGE_CURVE('',#8284,#8283,#7442,.T.);
#10794=EDGE_CURVE('',#8284,#8285,#5297,.T.);
#10795=EDGE_CURVE('',#8286,#8285,#7443,.T.);
#10796=EDGE_CURVE('',#8286,#8287,#5298,.T.);
#10797=EDGE_CURVE('',#8288,#8287,#7444,.T.);
#10798=EDGE_CURVE('',#8288,#8289,#5299,.T.);
#10799=EDGE_CURVE('',#8290,#8289,#7445,.T.);
#10800=EDGE_CURVE('',#8290,#8291,#5300,.T.);
#10801=EDGE_CURVE('',#8292,#8291,#7446,.T.);
#10802=EDGE_CURVE('',#8292,#8293,#5301,.T.);
#10803=EDGE_CURVE('',#8294,#8293,#7447,.T.);
#10804=EDGE_CURVE('',#8294,#8295,#5302,.T.);
#10805=EDGE_CURVE('',#8296,#8295,#7448,.T.);
#10806=EDGE_CURVE('',#8296,#8297,#5303,.T.);
#10807=EDGE_CURVE('',#8298,#8297,#7449,.T.);
#10808=EDGE_CURVE('',#8298,#8299,#5304,.T.);
#10809=EDGE_CURVE('',#8300,#8299,#7450,.T.);
#10810=EDGE_CURVE('',#8300,#8301,#5305,.T.);
#10811=EDGE_CURVE('',#8302,#8301,#7451,.T.);
#10812=EDGE_CURVE('',#8302,#8303,#5306,.T.);
#10813=EDGE_CURVE('',#8304,#8303,#7452,.T.);
#10814=EDGE_CURVE('',#8304,#8305,#5307,.T.);
#10815=EDGE_CURVE('',#8235,#8305,#7453,.T.);
#10816=EDGE_CURVE('',#8306,#8306,#7454,.T.);
#10817=EDGE_CURVE('',#8307,#8307,#7455,.T.);
#10818=EDGE_CURVE('',#8308,#8308,#7456,.T.);
#10819=EDGE_CURVE('',#8309,#8309,#7457,.T.);
#10820=EDGE_CURVE('',#8310,#8311,#7458,.T.);
#10821=EDGE_CURVE('',#8311,#8238,#5308,.T.);
#10822=EDGE_CURVE('',#8237,#8310,#5309,.T.);
#10823=EDGE_CURVE('',#8312,#8311,#5310,.T.);
#10824=EDGE_CURVE('',#8239,#8312,#5311,.T.);
#10825=EDGE_CURVE('',#8312,#8313,#7459,.T.);
#10826=EDGE_CURVE('',#8313,#8240,#5312,.T.);
#10827=EDGE_CURVE('',#8314,#8313,#5313,.T.);
#10828=EDGE_CURVE('',#8241,#8314,#5314,.T.);
#10829=EDGE_CURVE('',#8314,#8315,#7460,.T.);
#10830=EDGE_CURVE('',#8315,#8242,#5315,.T.);
#10831=EDGE_CURVE('',#8316,#8315,#5316,.T.);
#10832=EDGE_CURVE('',#8243,#8316,#5317,.T.);
#10833=EDGE_CURVE('',#8316,#8317,#7461,.T.);
#10834=EDGE_CURVE('',#8317,#8244,#5318,.T.);
#10835=EDGE_CURVE('',#8318,#8317,#5319,.T.);
#10836=EDGE_CURVE('',#8245,#8318,#5320,.T.);
#10837=EDGE_CURVE('',#8318,#8319,#7462,.T.);
#10838=EDGE_CURVE('',#8319,#8246,#5321,.T.);
#10839=EDGE_CURVE('',#8247,#8320,#5322,.T.);
#10840=EDGE_CURVE('',#8320,#8321,#7463,.T.);
#10841=EDGE_CURVE('',#8321,#8248,#5323,.T.);
#10842=EDGE_CURVE('',#8322,#8321,#5324,.T.);
#10843=EDGE_CURVE('',#8249,#8322,#5325,.T.);
#10844=EDGE_CURVE('',#8322,#8323,#7464,.T.);
#10845=EDGE_CURVE('',#8323,#8250,#5326,.T.);
#10846=EDGE_CURVE('',#8251,#8324,#5327,.T.);
#10847=EDGE_CURVE('',#8324,#8325,#7465,.T.);
#10848=EDGE_CURVE('',#8325,#8252,#5328,.T.);
#10849=EDGE_CURVE('',#8326,#8325,#5329,.T.);
#10850=EDGE_CURVE('',#8253,#8326,#5330,.T.);
#10851=EDGE_CURVE('',#8326,#8327,#7466,.T.);
#10852=EDGE_CURVE('',#8327,#8254,#5331,.T.);
#10853=EDGE_CURVE('',#8328,#8329,#7467,.T.);
#10854=EDGE_CURVE('',#8329,#8256,#5332,.T.);
#10855=EDGE_CURVE('',#8255,#8328,#5333,.T.);
#10856=EDGE_CURVE('',#8330,#8329,#5334,.T.);
#10857=EDGE_CURVE('',#8257,#8330,#5335,.T.);
#10858=EDGE_CURVE('',#8330,#8331,#7468,.T.);
#10859=EDGE_CURVE('',#8331,#8258,#5336,.T.);
#10860=EDGE_CURVE('',#8332,#8331,#5337,.T.);
#10861=EDGE_CURVE('',#8259,#8332,#5338,.T.);
#10862=EDGE_CURVE('',#8332,#8333,#7469,.T.);
#10863=EDGE_CURVE('',#8333,#8260,#5339,.T.);
#10864=EDGE_CURVE('',#8334,#8333,#5340,.T.);
#10865=EDGE_CURVE('',#8261,#8334,#5341,.T.);
#10866=EDGE_CURVE('',#8334,#8335,#7470,.T.);
#10867=EDGE_CURVE('',#8335,#8262,#5342,.T.);
#10868=EDGE_CURVE('',#8336,#8335,#5343,.T.);
#10869=EDGE_CURVE('',#8263,#8336,#5344,.T.);
#10870=EDGE_CURVE('',#8336,#8337,#7471,.T.);
#10871=EDGE_CURVE('',#8337,#8264,#5345,.T.);
#10872=EDGE_CURVE('',#8265,#8338,#5346,.T.);
#10873=EDGE_CURVE('',#8338,#8339,#7472,.T.);
#10874=EDGE_CURVE('',#8339,#8266,#5347,.T.);
#10875=EDGE_CURVE('',#8340,#8339,#5348,.T.);
#10876=EDGE_CURVE('',#8267,#8340,#5349,.T.);
#10877=EDGE_CURVE('',#8340,#8341,#7473,.T.);
#10878=EDGE_CURVE('',#8341,#8268,#5350,.T.);
#10879=EDGE_CURVE('',#8269,#8342,#5351,.T.);
#10880=EDGE_CURVE('',#8342,#8343,#7474,.T.);
#10881=EDGE_CURVE('',#8343,#8270,#5352,.T.);
#10882=EDGE_CURVE('',#8344,#8343,#5353,.T.);
#10883=EDGE_CURVE('',#8271,#8344,#5354,.T.);
#10884=EDGE_CURVE('',#8344,#8345,#7475,.T.);
#10885=EDGE_CURVE('',#8345,#8272,#5355,.T.);
#10886=EDGE_CURVE('',#8346,#8347,#7476,.T.);
#10887=EDGE_CURVE('',#8347,#8274,#5356,.T.);
#10888=EDGE_CURVE('',#8273,#8346,#5357,.T.);
#10889=EDGE_CURVE('',#8348,#8347,#5358,.T.);
#10890=EDGE_CURVE('',#8275,#8348,#5359,.T.);
#10891=EDGE_CURVE('',#8348,#8349,#7477,.T.);
#10892=EDGE_CURVE('',#8349,#8276,#5360,.T.);
#10893=EDGE_CURVE('',#8350,#8349,#5361,.T.);
#10894=EDGE_CURVE('',#8277,#8350,#5362,.T.);
#10895=EDGE_CURVE('',#8350,#8351,#7478,.T.);
#10896=EDGE_CURVE('',#8351,#8278,#5363,.T.);
#10897=EDGE_CURVE('',#8352,#8351,#5364,.T.);
#10898=EDGE_CURVE('',#8279,#8352,#5365,.T.);
#10899=EDGE_CURVE('',#8352,#8353,#7479,.T.);
#10900=EDGE_CURVE('',#8353,#8280,#5366,.T.);
#10901=EDGE_CURVE('',#8354,#8353,#5367,.T.);
#10902=EDGE_CURVE('',#8281,#8354,#5368,.T.);
#10903=EDGE_CURVE('',#8354,#8355,#7480,.T.);
#10904=EDGE_CURVE('',#8355,#8282,#5369,.T.);
#10905=EDGE_CURVE('',#8283,#8356,#5370,.T.);
#10906=EDGE_CURVE('',#8356,#8357,#7481,.T.);
#10907=EDGE_CURVE('',#8357,#8284,#5371,.T.);
#10908=EDGE_CURVE('',#8358,#8357,#5372,.T.);
#10909=EDGE_CURVE('',#8285,#8358,#5373,.T.);
#10910=EDGE_CURVE('',#8358,#8359,#7482,.T.);
#10911=EDGE_CURVE('',#8359,#8286,#5374,.T.);
#10912=EDGE_CURVE('',#8287,#8360,#5375,.T.);
#10913=EDGE_CURVE('',#8360,#8361,#7483,.T.);
#10914=EDGE_CURVE('',#8361,#8288,#5376,.T.);
#10915=EDGE_CURVE('',#8362,#8361,#5377,.T.);
#10916=EDGE_CURVE('',#8289,#8362,#5378,.T.);
#10917=EDGE_CURVE('',#8362,#8363,#7484,.T.);
#10918=EDGE_CURVE('',#8363,#8290,#5379,.T.);
#10919=EDGE_CURVE('',#8364,#8365,#7485,.T.);
#10920=EDGE_CURVE('',#8365,#8292,#5380,.T.);
#10921=EDGE_CURVE('',#8291,#8364,#5381,.T.);
#10922=EDGE_CURVE('',#8366,#8365,#5382,.T.);
#10923=EDGE_CURVE('',#8293,#8366,#5383,.T.);
#10924=EDGE_CURVE('',#8366,#8367,#7486,.T.);
#10925=EDGE_CURVE('',#8367,#8294,#5384,.T.);
#10926=EDGE_CURVE('',#8368,#8367,#5385,.T.);
#10927=EDGE_CURVE('',#8295,#8368,#5386,.T.);
#10928=EDGE_CURVE('',#8368,#8369,#7487,.T.);
#10929=EDGE_CURVE('',#8369,#8296,#5387,.T.);
#10930=EDGE_CURVE('',#8370,#8369,#5388,.T.);
#10931=EDGE_CURVE('',#8297,#8370,#5389,.T.);
#10932=EDGE_CURVE('',#8370,#8371,#7488,.T.);
#10933=EDGE_CURVE('',#8371,#8298,#5390,.T.);
#10934=EDGE_CURVE('',#8372,#8371,#5391,.T.);
#10935=EDGE_CURVE('',#8299,#8372,#5392,.T.);
#10936=EDGE_CURVE('',#8372,#8373,#7489,.T.);
#10937=EDGE_CURVE('',#8373,#8300,#5393,.T.);
#10938=EDGE_CURVE('',#8301,#8374,#5394,.T.);
#10939=EDGE_CURVE('',#8374,#8375,#7490,.T.);
#10940=EDGE_CURVE('',#8375,#8302,#5395,.T.);
#10941=EDGE_CURVE('',#8376,#8375,#5396,.T.);
#10942=EDGE_CURVE('',#8303,#8376,#5397,.T.);
#10943=EDGE_CURVE('',#8376,#8377,#7491,.T.);
#10944=EDGE_CURVE('',#8377,#8304,#5398,.T.);
#10945=EDGE_CURVE('',#8305,#8378,#5399,.T.);
#10946=EDGE_CURVE('',#8378,#8236,#7492,.T.);
#10947=EDGE_CURVE('',#8309,#8379,#5400,.T.);
#10948=EDGE_CURVE('',#8379,#8379,#7493,.T.);
#10949=EDGE_CURVE('',#8308,#8380,#5401,.T.);
#10950=EDGE_CURVE('',#8380,#8380,#7494,.T.);
#10951=EDGE_CURVE('',#8230,#8229,#5402,.T.);
#10952=EDGE_CURVE('',#8307,#8381,#5403,.T.);
#10953=EDGE_CURVE('',#8381,#8381,#7495,.T.);
#10954=EDGE_CURVE('',#8306,#8382,#5404,.T.);
#10955=EDGE_CURVE('',#8382,#8382,#7496,.T.);
#10956=EDGE_CURVE('',#8378,#8377,#5405,.T.);
#10957=EDGE_CURVE('',#8374,#8373,#5406,.T.);
#10958=EDGE_CURVE('',#8364,#8363,#5407,.T.);
#10959=EDGE_CURVE('',#8360,#8359,#5408,.T.);
#10960=EDGE_CURVE('',#8356,#8355,#5409,.T.);
#10961=EDGE_CURVE('',#8346,#8345,#5410,.T.);
#10962=EDGE_CURVE('',#8342,#8341,#5411,.T.);
#10963=EDGE_CURVE('',#8338,#8337,#5412,.T.);
#10964=EDGE_CURVE('',#8328,#8327,#5413,.T.);
#10965=EDGE_CURVE('',#8324,#8323,#5414,.T.);
#10966=EDGE_CURVE('',#8320,#8319,#5415,.T.);
#10967=EDGE_CURVE('',#8310,#8234,#5416,.T.);
#14120=ORIENTED_EDGE('',*,*,#10317,.T.);
#14121=ORIENTED_EDGE('',*,*,#10318,.T.);
#14122=ORIENTED_EDGE('',*,*,#10319,.T.);
#14123=ORIENTED_EDGE('',*,*,#10320,.T.);
#14124=ORIENTED_EDGE('',*,*,#10321,.T.);
#14125=ORIENTED_EDGE('',*,*,#10320,.F.);
#14126=ORIENTED_EDGE('',*,*,#10322,.T.);
#14127=ORIENTED_EDGE('',*,*,#10323,.T.);
#14128=ORIENTED_EDGE('',*,*,#10324,.T.);
#14129=ORIENTED_EDGE('',*,*,#10325,.T.);
#14130=ORIENTED_EDGE('',*,*,#10317,.F.);
#14131=ORIENTED_EDGE('',*,*,#10326,.T.);
#14132=ORIENTED_EDGE('',*,*,#10327,.T.);
#14133=ORIENTED_EDGE('',*,*,#10328,.T.);
#14134=ORIENTED_EDGE('',*,*,#10324,.F.);
#14135=ORIENTED_EDGE('',*,*,#10329,.T.);
#14136=ORIENTED_EDGE('',*,*,#10330,.T.);
#14137=ORIENTED_EDGE('',*,*,#10331,.T.);
#14138=ORIENTED_EDGE('',*,*,#10327,.F.);
#14139=ORIENTED_EDGE('',*,*,#10332,.T.);
#14140=ORIENTED_EDGE('',*,*,#10333,.T.);
#14141=ORIENTED_EDGE('',*,*,#10334,.T.);
#14142=ORIENTED_EDGE('',*,*,#10330,.F.);
#14143=ORIENTED_EDGE('',*,*,#10335,.T.);
#14144=ORIENTED_EDGE('',*,*,#10336,.T.);
#14145=ORIENTED_EDGE('',*,*,#10337,.T.);
#14146=ORIENTED_EDGE('',*,*,#10333,.F.);
#14147=ORIENTED_EDGE('',*,*,#10338,.T.);
#14148=ORIENTED_EDGE('',*,*,#10339,.T.);
#14149=ORIENTED_EDGE('',*,*,#10340,.T.);
#14150=ORIENTED_EDGE('',*,*,#10336,.F.);
#14151=ORIENTED_EDGE('',*,*,#10341,.T.);
#14152=ORIENTED_EDGE('',*,*,#10342,.T.);
#14153=ORIENTED_EDGE('',*,*,#10343,.T.);
#14154=ORIENTED_EDGE('',*,*,#10339,.F.);
#14155=ORIENTED_EDGE('',*,*,#10344,.T.);
#14156=ORIENTED_EDGE('',*,*,#10345,.T.);
#14157=ORIENTED_EDGE('',*,*,#10346,.T.);
#14158=ORIENTED_EDGE('',*,*,#10342,.F.);
#14159=ORIENTED_EDGE('',*,*,#10347,.T.);
#14160=ORIENTED_EDGE('',*,*,#10348,.T.);
#14161=ORIENTED_EDGE('',*,*,#10349,.T.);
#14162=ORIENTED_EDGE('',*,*,#10345,.F.);
#14163=ORIENTED_EDGE('',*,*,#10350,.T.);
#14164=ORIENTED_EDGE('',*,*,#10351,.T.);
#14165=ORIENTED_EDGE('',*,*,#10352,.T.);
#14166=ORIENTED_EDGE('',*,*,#10348,.F.);
#14167=ORIENTED_EDGE('',*,*,#10353,.T.);
#14168=ORIENTED_EDGE('',*,*,#10354,.T.);
#14169=ORIENTED_EDGE('',*,*,#10355,.T.);
#14170=ORIENTED_EDGE('',*,*,#10351,.F.);
#14171=ORIENTED_EDGE('',*,*,#10356,.T.);
#14172=ORIENTED_EDGE('',*,*,#10357,.T.);
#14173=ORIENTED_EDGE('',*,*,#10358,.T.);
#14174=ORIENTED_EDGE('',*,*,#10354,.F.);
#14175=ORIENTED_EDGE('',*,*,#10359,.T.);
#14176=ORIENTED_EDGE('',*,*,#10360,.T.);
#14177=ORIENTED_EDGE('',*,*,#10361,.T.);
#14178=ORIENTED_EDGE('',*,*,#10357,.F.);
#14179=ORIENTED_EDGE('',*,*,#10362,.T.);
#14180=ORIENTED_EDGE('',*,*,#10363,.T.);
#14181=ORIENTED_EDGE('',*,*,#10364,.T.);
#14182=ORIENTED_EDGE('',*,*,#10360,.F.);
#14183=ORIENTED_EDGE('',*,*,#10365,.T.);
#14184=ORIENTED_EDGE('',*,*,#10366,.T.);
#14185=ORIENTED_EDGE('',*,*,#10367,.T.);
#14186=ORIENTED_EDGE('',*,*,#10363,.F.);
#14187=ORIENTED_EDGE('',*,*,#10368,.T.);
#14188=ORIENTED_EDGE('',*,*,#10369,.T.);
#14189=ORIENTED_EDGE('',*,*,#10370,.T.);
#14190=ORIENTED_EDGE('',*,*,#10366,.F.);
#14191=ORIENTED_EDGE('',*,*,#10371,.T.);
#14192=ORIENTED_EDGE('',*,*,#10372,.T.);
#14193=ORIENTED_EDGE('',*,*,#10373,.T.);
#14194=ORIENTED_EDGE('',*,*,#10369,.F.);
#14195=ORIENTED_EDGE('',*,*,#10374,.T.);
#14196=ORIENTED_EDGE('',*,*,#10375,.T.);
#14197=ORIENTED_EDGE('',*,*,#10376,.T.);
#14198=ORIENTED_EDGE('',*,*,#10372,.F.);
#14199=ORIENTED_EDGE('',*,*,#10377,.T.);
#14200=ORIENTED_EDGE('',*,*,#10378,.T.);
#14201=ORIENTED_EDGE('',*,*,#10379,.T.);
#14202=ORIENTED_EDGE('',*,*,#10375,.F.);
#14203=ORIENTED_EDGE('',*,*,#10380,.T.);
#14204=ORIENTED_EDGE('',*,*,#10381,.T.);
#14205=ORIENTED_EDGE('',*,*,#10382,.T.);
#14206=ORIENTED_EDGE('',*,*,#10378,.F.);
#14207=ORIENTED_EDGE('',*,*,#10383,.T.);
#14208=ORIENTED_EDGE('',*,*,#10384,.T.);
#14209=ORIENTED_EDGE('',*,*,#10385,.T.);
#14210=ORIENTED_EDGE('',*,*,#10381,.F.);
#14211=ORIENTED_EDGE('',*,*,#10386,.T.);
#14212=ORIENTED_EDGE('',*,*,#10387,.T.);
#14213=ORIENTED_EDGE('',*,*,#10388,.T.);
#14214=ORIENTED_EDGE('',*,*,#10384,.F.);
#14215=ORIENTED_EDGE('',*,*,#10389,.T.);
#14216=ORIENTED_EDGE('',*,*,#10390,.T.);
#14217=ORIENTED_EDGE('',*,*,#10391,.T.);
#14218=ORIENTED_EDGE('',*,*,#10387,.F.);
#14219=ORIENTED_EDGE('',*,*,#10392,.T.);
#14220=ORIENTED_EDGE('',*,*,#10393,.F.);
#14221=ORIENTED_EDGE('',*,*,#10394,.T.);
#14222=ORIENTED_EDGE('',*,*,#10395,.F.);
#14223=ORIENTED_EDGE('',*,*,#10396,.T.);
#14224=ORIENTED_EDGE('',*,*,#10397,.T.);
#14225=ORIENTED_EDGE('',*,*,#10398,.T.);
#14226=ORIENTED_EDGE('',*,*,#10399,.F.);
#14227=ORIENTED_EDGE('',*,*,#10400,.F.);
#14228=ORIENTED_EDGE('',*,*,#10401,.T.);
#14229=ORIENTED_EDGE('',*,*,#10402,.T.);
#14230=ORIENTED_EDGE('',*,*,#10397,.F.);
#14231=ORIENTED_EDGE('',*,*,#10403,.F.);
#14232=ORIENTED_EDGE('',*,*,#10404,.T.);
#14233=ORIENTED_EDGE('',*,*,#10405,.T.);
#14234=ORIENTED_EDGE('',*,*,#10401,.F.);
#14235=ORIENTED_EDGE('',*,*,#10406,.F.);
#14236=ORIENTED_EDGE('',*,*,#10407,.T.);
#14237=ORIENTED_EDGE('',*,*,#10408,.T.);
#14238=ORIENTED_EDGE('',*,*,#10404,.F.);
#14239=ORIENTED_EDGE('',*,*,#10409,.F.);
#14240=ORIENTED_EDGE('',*,*,#10410,.T.);
#14241=ORIENTED_EDGE('',*,*,#10411,.T.);
#14242=ORIENTED_EDGE('',*,*,#10407,.F.);
#14243=ORIENTED_EDGE('',*,*,#10412,.F.);
#14244=ORIENTED_EDGE('',*,*,#10413,.T.);
#14245=ORIENTED_EDGE('',*,*,#10414,.T.);
#14246=ORIENTED_EDGE('',*,*,#10410,.F.);
#14247=ORIENTED_EDGE('',*,*,#10415,.F.);
#14248=ORIENTED_EDGE('',*,*,#10416,.T.);
#14249=ORIENTED_EDGE('',*,*,#10417,.T.);
#14250=ORIENTED_EDGE('',*,*,#10413,.F.);
#14251=ORIENTED_EDGE('',*,*,#10418,.F.);
#14252=ORIENTED_EDGE('',*,*,#10419,.T.);
#14253=ORIENTED_EDGE('',*,*,#10420,.T.);
#14254=ORIENTED_EDGE('',*,*,#10416,.F.);
#14255=ORIENTED_EDGE('',*,*,#10421,.F.);
#14256=ORIENTED_EDGE('',*,*,#10422,.T.);
#14257=ORIENTED_EDGE('',*,*,#10423,.T.);
#14258=ORIENTED_EDGE('',*,*,#10419,.F.);
#14259=ORIENTED_EDGE('',*,*,#10424,.F.);
#14260=ORIENTED_EDGE('',*,*,#10425,.T.);
#14261=ORIENTED_EDGE('',*,*,#10426,.T.);
#14262=ORIENTED_EDGE('',*,*,#10422,.F.);
#14263=ORIENTED_EDGE('',*,*,#10427,.F.);
#14264=ORIENTED_EDGE('',*,*,#10428,.T.);
#14265=ORIENTED_EDGE('',*,*,#10429,.T.);
#14266=ORIENTED_EDGE('',*,*,#10425,.F.);
#14267=ORIENTED_EDGE('',*,*,#10430,.F.);
#14268=ORIENTED_EDGE('',*,*,#10431,.T.);
#14269=ORIENTED_EDGE('',*,*,#10432,.T.);
#14270=ORIENTED_EDGE('',*,*,#10428,.F.);
#14271=ORIENTED_EDGE('',*,*,#10433,.F.);
#14272=ORIENTED_EDGE('',*,*,#10434,.T.);
#14273=ORIENTED_EDGE('',*,*,#10435,.T.);
#14274=ORIENTED_EDGE('',*,*,#10431,.F.);
#14275=ORIENTED_EDGE('',*,*,#10436,.F.);
#14276=ORIENTED_EDGE('',*,*,#10437,.T.);
#14277=ORIENTED_EDGE('',*,*,#10438,.T.);
#14278=ORIENTED_EDGE('',*,*,#10434,.F.);
#14279=ORIENTED_EDGE('',*,*,#10439,.F.);
#14280=ORIENTED_EDGE('',*,*,#10440,.T.);
#14281=ORIENTED_EDGE('',*,*,#10441,.T.);
#14282=ORIENTED_EDGE('',*,*,#10437,.F.);
#14283=ORIENTED_EDGE('',*,*,#10442,.F.);
#14284=ORIENTED_EDGE('',*,*,#10443,.T.);
#14285=ORIENTED_EDGE('',*,*,#10444,.T.);
#14286=ORIENTED_EDGE('',*,*,#10440,.F.);
#14287=ORIENTED_EDGE('',*,*,#10445,.F.);
#14288=ORIENTED_EDGE('',*,*,#10446,.T.);
#14289=ORIENTED_EDGE('',*,*,#10447,.T.);
#14290=ORIENTED_EDGE('',*,*,#10443,.F.);
#14291=ORIENTED_EDGE('',*,*,#10448,.F.);
#14292=ORIENTED_EDGE('',*,*,#10449,.T.);
#14293=ORIENTED_EDGE('',*,*,#10450,.T.);
#14294=ORIENTED_EDGE('',*,*,#10446,.F.);
#14295=ORIENTED_EDGE('',*,*,#10451,.F.);
#14296=ORIENTED_EDGE('',*,*,#10452,.T.);
#14297=ORIENTED_EDGE('',*,*,#10453,.T.);
#14298=ORIENTED_EDGE('',*,*,#10449,.F.);
#14299=ORIENTED_EDGE('',*,*,#10454,.F.);
#14300=ORIENTED_EDGE('',*,*,#10455,.T.);
#14301=ORIENTED_EDGE('',*,*,#10456,.T.);
#14302=ORIENTED_EDGE('',*,*,#10452,.F.);
#14303=ORIENTED_EDGE('',*,*,#10457,.F.);
#14304=ORIENTED_EDGE('',*,*,#10458,.T.);
#14305=ORIENTED_EDGE('',*,*,#10459,.T.);
#14306=ORIENTED_EDGE('',*,*,#10455,.F.);
#14307=ORIENTED_EDGE('',*,*,#10460,.F.);
#14308=ORIENTED_EDGE('',*,*,#10461,.T.);
#14309=ORIENTED_EDGE('',*,*,#10462,.T.);
#14310=ORIENTED_EDGE('',*,*,#10458,.F.);
#14311=ORIENTED_EDGE('',*,*,#10463,.F.);
#14312=ORIENTED_EDGE('',*,*,#10464,.T.);
#14313=ORIENTED_EDGE('',*,*,#10465,.T.);
#14314=ORIENTED_EDGE('',*,*,#10461,.F.);
#14315=ORIENTED_EDGE('',*,*,#10466,.F.);
#14316=ORIENTED_EDGE('',*,*,#10467,.T.);
#14317=ORIENTED_EDGE('',*,*,#10468,.T.);
#14318=ORIENTED_EDGE('',*,*,#10464,.F.);
#14319=ORIENTED_EDGE('',*,*,#10469,.F.);
#14320=ORIENTED_EDGE('',*,*,#10470,.F.);
#14321=ORIENTED_EDGE('',*,*,#10471,.F.);
#14322=ORIENTED_EDGE('',*,*,#10472,.F.);
#14323=ORIENTED_EDGE('',*,*,#10473,.T.);
#14324=ORIENTED_EDGE('',*,*,#10474,.T.);
#14325=ORIENTED_EDGE('',*,*,#10475,.T.);
#14326=ORIENTED_EDGE('',*,*,#10476,.T.);
#14327=ORIENTED_EDGE('',*,*,#10477,.T.);
#14328=ORIENTED_EDGE('',*,*,#10478,.T.);
#14329=ORIENTED_EDGE('',*,*,#10477,.F.);
#14330=ORIENTED_EDGE('',*,*,#10479,.T.);
#14331=ORIENTED_EDGE('',*,*,#10480,.T.);
#14332=ORIENTED_EDGE('',*,*,#10481,.T.);
#14333=ORIENTED_EDGE('',*,*,#10482,.T.);
#14334=ORIENTED_EDGE('',*,*,#10474,.F.);
#14335=ORIENTED_EDGE('',*,*,#10483,.T.);
#14336=ORIENTED_EDGE('',*,*,#10484,.T.);
#14337=ORIENTED_EDGE('',*,*,#10485,.T.);
#14338=ORIENTED_EDGE('',*,*,#10481,.F.);
#14339=ORIENTED_EDGE('',*,*,#10486,.T.);
#14340=ORIENTED_EDGE('',*,*,#10487,.T.);
#14341=ORIENTED_EDGE('',*,*,#10488,.T.);
#14342=ORIENTED_EDGE('',*,*,#10484,.F.);
#14343=ORIENTED_EDGE('',*,*,#10489,.T.);
#14344=ORIENTED_EDGE('',*,*,#10490,.T.);
#14345=ORIENTED_EDGE('',*,*,#10491,.T.);
#14346=ORIENTED_EDGE('',*,*,#10487,.F.);
#14347=ORIENTED_EDGE('',*,*,#10492,.T.);
#14348=ORIENTED_EDGE('',*,*,#10493,.T.);
#14349=ORIENTED_EDGE('',*,*,#10494,.T.);
#14350=ORIENTED_EDGE('',*,*,#10490,.F.);
#14351=ORIENTED_EDGE('',*,*,#10495,.T.);
#14352=ORIENTED_EDGE('',*,*,#10496,.T.);
#14353=ORIENTED_EDGE('',*,*,#10497,.T.);
#14354=ORIENTED_EDGE('',*,*,#10493,.F.);
#14355=ORIENTED_EDGE('',*,*,#10498,.T.);
#14356=ORIENTED_EDGE('',*,*,#10499,.T.);
#14357=ORIENTED_EDGE('',*,*,#10500,.T.);
#14358=ORIENTED_EDGE('',*,*,#10496,.F.);
#14359=ORIENTED_EDGE('',*,*,#10501,.T.);
#14360=ORIENTED_EDGE('',*,*,#10502,.T.);
#14361=ORIENTED_EDGE('',*,*,#10503,.T.);
#14362=ORIENTED_EDGE('',*,*,#10499,.F.);
#14363=ORIENTED_EDGE('',*,*,#10504,.T.);
#14364=ORIENTED_EDGE('',*,*,#10505,.T.);
#14365=ORIENTED_EDGE('',*,*,#10506,.T.);
#14366=ORIENTED_EDGE('',*,*,#10502,.F.);
#14367=ORIENTED_EDGE('',*,*,#10507,.T.);
#14368=ORIENTED_EDGE('',*,*,#10508,.T.);
#14369=ORIENTED_EDGE('',*,*,#10509,.T.);
#14370=ORIENTED_EDGE('',*,*,#10505,.F.);
#14371=ORIENTED_EDGE('',*,*,#10510,.T.);
#14372=ORIENTED_EDGE('',*,*,#10511,.T.);
#14373=ORIENTED_EDGE('',*,*,#10512,.T.);
#14374=ORIENTED_EDGE('',*,*,#10508,.F.);
#14375=ORIENTED_EDGE('',*,*,#10513,.T.);
#14376=ORIENTED_EDGE('',*,*,#10514,.T.);
#14377=ORIENTED_EDGE('',*,*,#10515,.T.);
#14378=ORIENTED_EDGE('',*,*,#10511,.F.);
#14379=ORIENTED_EDGE('',*,*,#10516,.T.);
#14380=ORIENTED_EDGE('',*,*,#10517,.T.);
#14381=ORIENTED_EDGE('',*,*,#10518,.T.);
#14382=ORIENTED_EDGE('',*,*,#10514,.F.);
#14383=ORIENTED_EDGE('',*,*,#10519,.T.);
#14384=ORIENTED_EDGE('',*,*,#10520,.T.);
#14385=ORIENTED_EDGE('',*,*,#10521,.T.);
#14386=ORIENTED_EDGE('',*,*,#10517,.F.);
#14387=ORIENTED_EDGE('',*,*,#10522,.T.);
#14388=ORIENTED_EDGE('',*,*,#10523,.T.);
#14389=ORIENTED_EDGE('',*,*,#10524,.T.);
#14390=ORIENTED_EDGE('',*,*,#10520,.F.);
#14391=ORIENTED_EDGE('',*,*,#10525,.T.);
#14392=ORIENTED_EDGE('',*,*,#10526,.T.);
#14393=ORIENTED_EDGE('',*,*,#10527,.T.);
#14394=ORIENTED_EDGE('',*,*,#10523,.F.);
#14395=ORIENTED_EDGE('',*,*,#10528,.T.);
#14396=ORIENTED_EDGE('',*,*,#10529,.T.);
#14397=ORIENTED_EDGE('',*,*,#10530,.T.);
#14398=ORIENTED_EDGE('',*,*,#10526,.F.);
#14399=ORIENTED_EDGE('',*,*,#10531,.T.);
#14400=ORIENTED_EDGE('',*,*,#10532,.T.);
#14401=ORIENTED_EDGE('',*,*,#10533,.T.);
#14402=ORIENTED_EDGE('',*,*,#10529,.F.);
#14403=ORIENTED_EDGE('',*,*,#10534,.T.);
#14404=ORIENTED_EDGE('',*,*,#10535,.T.);
#14405=ORIENTED_EDGE('',*,*,#10536,.T.);
#14406=ORIENTED_EDGE('',*,*,#10532,.F.);
#14407=ORIENTED_EDGE('',*,*,#10537,.T.);
#14408=ORIENTED_EDGE('',*,*,#10538,.T.);
#14409=ORIENTED_EDGE('',*,*,#10539,.T.);
#14410=ORIENTED_EDGE('',*,*,#10535,.F.);
#14411=ORIENTED_EDGE('',*,*,#10540,.T.);
#14412=ORIENTED_EDGE('',*,*,#10541,.T.);
#14413=ORIENTED_EDGE('',*,*,#10542,.T.);
#14414=ORIENTED_EDGE('',*,*,#10538,.F.);
#14415=ORIENTED_EDGE('',*,*,#10543,.T.);
#14416=ORIENTED_EDGE('',*,*,#10544,.T.);
#14417=ORIENTED_EDGE('',*,*,#10545,.T.);
#14418=ORIENTED_EDGE('',*,*,#10541,.F.);
#14419=ORIENTED_EDGE('',*,*,#10546,.T.);
#14420=ORIENTED_EDGE('',*,*,#10547,.T.);
#14421=ORIENTED_EDGE('',*,*,#10548,.T.);
#14422=ORIENTED_EDGE('',*,*,#10544,.F.);
#14423=ORIENTED_EDGE('',*,*,#10549,.T.);
#14424=ORIENTED_EDGE('',*,*,#10550,.T.);
#14425=ORIENTED_EDGE('',*,*,#10551,.T.);
#14426=ORIENTED_EDGE('',*,*,#10547,.F.);
#14427=ORIENTED_EDGE('',*,*,#10552,.T.);
#14428=ORIENTED_EDGE('',*,*,#10553,.T.);
#14429=ORIENTED_EDGE('',*,*,#10554,.T.);
#14430=ORIENTED_EDGE('',*,*,#10550,.F.);
#14431=ORIENTED_EDGE('',*,*,#10555,.T.);
#14432=ORIENTED_EDGE('',*,*,#10556,.T.);
#14433=ORIENTED_EDGE('',*,*,#10557,.T.);
#14434=ORIENTED_EDGE('',*,*,#10553,.F.);
#14435=ORIENTED_EDGE('',*,*,#10558,.T.);
#14436=ORIENTED_EDGE('',*,*,#10559,.T.);
#14437=ORIENTED_EDGE('',*,*,#10560,.T.);
#14438=ORIENTED_EDGE('',*,*,#10556,.F.);
#14439=ORIENTED_EDGE('',*,*,#10561,.T.);
#14440=ORIENTED_EDGE('',*,*,#10562,.T.);
#14441=ORIENTED_EDGE('',*,*,#10563,.T.);
#14442=ORIENTED_EDGE('',*,*,#10559,.F.);
#14443=ORIENTED_EDGE('',*,*,#10564,.T.);
#14444=ORIENTED_EDGE('',*,*,#10565,.T.);
#14445=ORIENTED_EDGE('',*,*,#10566,.T.);
#14446=ORIENTED_EDGE('',*,*,#10562,.F.);
#14447=ORIENTED_EDGE('',*,*,#10567,.T.);
#14448=ORIENTED_EDGE('',*,*,#10568,.T.);
#14449=ORIENTED_EDGE('',*,*,#10569,.T.);
#14450=ORIENTED_EDGE('',*,*,#10565,.F.);
#14451=ORIENTED_EDGE('',*,*,#10570,.T.);
#14452=ORIENTED_EDGE('',*,*,#10571,.T.);
#14453=ORIENTED_EDGE('',*,*,#10572,.T.);
#14454=ORIENTED_EDGE('',*,*,#10568,.F.);
#14455=ORIENTED_EDGE('',*,*,#10573,.T.);
#14456=ORIENTED_EDGE('',*,*,#10574,.T.);
#14457=ORIENTED_EDGE('',*,*,#10575,.T.);
#14458=ORIENTED_EDGE('',*,*,#10571,.F.);
#14459=ORIENTED_EDGE('',*,*,#10576,.T.);
#14460=ORIENTED_EDGE('',*,*,#10577,.T.);
#14461=ORIENTED_EDGE('',*,*,#10578,.T.);
#14462=ORIENTED_EDGE('',*,*,#10574,.F.);
#14463=ORIENTED_EDGE('',*,*,#10579,.T.);
#14464=ORIENTED_EDGE('',*,*,#10580,.T.);
#14465=ORIENTED_EDGE('',*,*,#10581,.T.);
#14466=ORIENTED_EDGE('',*,*,#10577,.F.);
#14467=ORIENTED_EDGE('',*,*,#10582,.T.);
#14468=ORIENTED_EDGE('',*,*,#10583,.T.);
#14469=ORIENTED_EDGE('',*,*,#10584,.T.);
#14470=ORIENTED_EDGE('',*,*,#10580,.F.);
#14471=ORIENTED_EDGE('',*,*,#10585,.T.);
#14472=ORIENTED_EDGE('',*,*,#10586,.T.);
#14473=ORIENTED_EDGE('',*,*,#10587,.T.);
#14474=ORIENTED_EDGE('',*,*,#10583,.F.);
#14475=ORIENTED_EDGE('',*,*,#10588,.T.);
#14476=ORIENTED_EDGE('',*,*,#10589,.T.);
#14477=ORIENTED_EDGE('',*,*,#10590,.T.);
#14478=ORIENTED_EDGE('',*,*,#10586,.F.);
#14479=ORIENTED_EDGE('',*,*,#10591,.T.);
#14480=ORIENTED_EDGE('',*,*,#10592,.T.);
#14481=ORIENTED_EDGE('',*,*,#10593,.T.);
#14482=ORIENTED_EDGE('',*,*,#10589,.F.);
#14483=ORIENTED_EDGE('',*,*,#10594,.T.);
#14484=ORIENTED_EDGE('',*,*,#10595,.F.);
#14485=ORIENTED_EDGE('',*,*,#10596,.T.);
#14486=ORIENTED_EDGE('',*,*,#10597,.F.);
#14487=ORIENTED_EDGE('',*,*,#10598,.T.);
#14488=ORIENTED_EDGE('',*,*,#10599,.T.);
#14489=ORIENTED_EDGE('',*,*,#10600,.T.);
#14490=ORIENTED_EDGE('',*,*,#10601,.F.);
#14491=ORIENTED_EDGE('',*,*,#10602,.F.);
#14492=ORIENTED_EDGE('',*,*,#10603,.T.);
#14493=ORIENTED_EDGE('',*,*,#10604,.T.);
#14494=ORIENTED_EDGE('',*,*,#10599,.F.);
#14495=ORIENTED_EDGE('',*,*,#10605,.F.);
#14496=ORIENTED_EDGE('',*,*,#10606,.T.);
#14497=ORIENTED_EDGE('',*,*,#10607,.T.);
#14498=ORIENTED_EDGE('',*,*,#10603,.F.);
#14499=ORIENTED_EDGE('',*,*,#10608,.F.);
#14500=ORIENTED_EDGE('',*,*,#10609,.T.);
#14501=ORIENTED_EDGE('',*,*,#10610,.T.);
#14502=ORIENTED_EDGE('',*,*,#10606,.F.);
#14503=ORIENTED_EDGE('',*,*,#10611,.F.);
#14504=ORIENTED_EDGE('',*,*,#10612,.T.);
#14505=ORIENTED_EDGE('',*,*,#10613,.T.);
#14506=ORIENTED_EDGE('',*,*,#10609,.F.);
#14507=ORIENTED_EDGE('',*,*,#10614,.F.);
#14508=ORIENTED_EDGE('',*,*,#10615,.T.);
#14509=ORIENTED_EDGE('',*,*,#10616,.T.);
#14510=ORIENTED_EDGE('',*,*,#10612,.F.);
#14511=ORIENTED_EDGE('',*,*,#10617,.F.);
#14512=ORIENTED_EDGE('',*,*,#10618,.T.);
#14513=ORIENTED_EDGE('',*,*,#10619,.T.);
#14514=ORIENTED_EDGE('',*,*,#10615,.F.);
#14515=ORIENTED_EDGE('',*,*,#10620,.F.);
#14516=ORIENTED_EDGE('',*,*,#10621,.T.);
#14517=ORIENTED_EDGE('',*,*,#10622,.T.);
#14518=ORIENTED_EDGE('',*,*,#10618,.F.);
#14519=ORIENTED_EDGE('',*,*,#10623,.F.);
#14520=ORIENTED_EDGE('',*,*,#10624,.T.);
#14521=ORIENTED_EDGE('',*,*,#10625,.T.);
#14522=ORIENTED_EDGE('',*,*,#10621,.F.);
#14523=ORIENTED_EDGE('',*,*,#10626,.F.);
#14524=ORIENTED_EDGE('',*,*,#10627,.T.);
#14525=ORIENTED_EDGE('',*,*,#10628,.T.);
#14526=ORIENTED_EDGE('',*,*,#10624,.F.);
#14527=ORIENTED_EDGE('',*,*,#10629,.F.);
#14528=ORIENTED_EDGE('',*,*,#10630,.T.);
#14529=ORIENTED_EDGE('',*,*,#10631,.T.);
#14530=ORIENTED_EDGE('',*,*,#10627,.F.);
#14531=ORIENTED_EDGE('',*,*,#10632,.F.);
#14532=ORIENTED_EDGE('',*,*,#10633,.T.);
#14533=ORIENTED_EDGE('',*,*,#10634,.T.);
#14534=ORIENTED_EDGE('',*,*,#10630,.F.);
#14535=ORIENTED_EDGE('',*,*,#10635,.F.);
#14536=ORIENTED_EDGE('',*,*,#10636,.T.);
#14537=ORIENTED_EDGE('',*,*,#10637,.T.);
#14538=ORIENTED_EDGE('',*,*,#10633,.F.);
#14539=ORIENTED_EDGE('',*,*,#10638,.F.);
#14540=ORIENTED_EDGE('',*,*,#10639,.T.);
#14541=ORIENTED_EDGE('',*,*,#10640,.T.);
#14542=ORIENTED_EDGE('',*,*,#10636,.F.);
#14543=ORIENTED_EDGE('',*,*,#10641,.F.);
#14544=ORIENTED_EDGE('',*,*,#10642,.T.);
#14545=ORIENTED_EDGE('',*,*,#10643,.T.);
#14546=ORIENTED_EDGE('',*,*,#10639,.F.);
#14547=ORIENTED_EDGE('',*,*,#10644,.F.);
#14548=ORIENTED_EDGE('',*,*,#10645,.T.);
#14549=ORIENTED_EDGE('',*,*,#10646,.T.);
#14550=ORIENTED_EDGE('',*,*,#10642,.F.);
#14551=ORIENTED_EDGE('',*,*,#10647,.F.);
#14552=ORIENTED_EDGE('',*,*,#10648,.T.);
#14553=ORIENTED_EDGE('',*,*,#10649,.T.);
#14554=ORIENTED_EDGE('',*,*,#10645,.F.);
#14555=ORIENTED_EDGE('',*,*,#10650,.F.);
#14556=ORIENTED_EDGE('',*,*,#10651,.T.);
#14557=ORIENTED_EDGE('',*,*,#10652,.T.);
#14558=ORIENTED_EDGE('',*,*,#10648,.F.);
#14559=ORIENTED_EDGE('',*,*,#10653,.F.);
#14560=ORIENTED_EDGE('',*,*,#10654,.T.);
#14561=ORIENTED_EDGE('',*,*,#10655,.T.);
#14562=ORIENTED_EDGE('',*,*,#10651,.F.);
#14563=ORIENTED_EDGE('',*,*,#10656,.F.);
#14564=ORIENTED_EDGE('',*,*,#10657,.T.);
#14565=ORIENTED_EDGE('',*,*,#10658,.T.);
#14566=ORIENTED_EDGE('',*,*,#10654,.F.);
#14567=ORIENTED_EDGE('',*,*,#10659,.F.);
#14568=ORIENTED_EDGE('',*,*,#10660,.T.);
#14569=ORIENTED_EDGE('',*,*,#10661,.T.);
#14570=ORIENTED_EDGE('',*,*,#10657,.F.);
#14571=ORIENTED_EDGE('',*,*,#10662,.F.);
#14572=ORIENTED_EDGE('',*,*,#10663,.T.);
#14573=ORIENTED_EDGE('',*,*,#10664,.T.);
#14574=ORIENTED_EDGE('',*,*,#10660,.F.);
#14575=ORIENTED_EDGE('',*,*,#10665,.F.);
#14576=ORIENTED_EDGE('',*,*,#10666,.T.);
#14577=ORIENTED_EDGE('',*,*,#10667,.T.);
#14578=ORIENTED_EDGE('',*,*,#10663,.F.);
#14579=ORIENTED_EDGE('',*,*,#10668,.F.);
#14580=ORIENTED_EDGE('',*,*,#10669,.T.);
#14581=ORIENTED_EDGE('',*,*,#10670,.T.);
#14582=ORIENTED_EDGE('',*,*,#10666,.F.);
#14583=ORIENTED_EDGE('',*,*,#10671,.F.);
#14584=ORIENTED_EDGE('',*,*,#10672,.T.);
#14585=ORIENTED_EDGE('',*,*,#10673,.T.);
#14586=ORIENTED_EDGE('',*,*,#10669,.F.);
#14587=ORIENTED_EDGE('',*,*,#10674,.F.);
#14588=ORIENTED_EDGE('',*,*,#10675,.T.);
#14589=ORIENTED_EDGE('',*,*,#10676,.T.);
#14590=ORIENTED_EDGE('',*,*,#10672,.F.);
#14591=ORIENTED_EDGE('',*,*,#10677,.F.);
#14592=ORIENTED_EDGE('',*,*,#10678,.T.);
#14593=ORIENTED_EDGE('',*,*,#10679,.T.);
#14594=ORIENTED_EDGE('',*,*,#10675,.F.);
#14595=ORIENTED_EDGE('',*,*,#10680,.F.);
#14596=ORIENTED_EDGE('',*,*,#10681,.T.);
#14597=ORIENTED_EDGE('',*,*,#10682,.T.);
#14598=ORIENTED_EDGE('',*,*,#10678,.F.);
#14599=ORIENTED_EDGE('',*,*,#10683,.F.);
#14600=ORIENTED_EDGE('',*,*,#10684,.T.);
#14601=ORIENTED_EDGE('',*,*,#10685,.T.);
#14602=ORIENTED_EDGE('',*,*,#10681,.F.);
#14603=ORIENTED_EDGE('',*,*,#10686,.F.);
#14604=ORIENTED_EDGE('',*,*,#10687,.T.);
#14605=ORIENTED_EDGE('',*,*,#10688,.T.);
#14606=ORIENTED_EDGE('',*,*,#10684,.F.);
#14607=ORIENTED_EDGE('',*,*,#10689,.F.);
#14608=ORIENTED_EDGE('',*,*,#10690,.T.);
#14609=ORIENTED_EDGE('',*,*,#10691,.T.);
#14610=ORIENTED_EDGE('',*,*,#10687,.F.);
#14611=ORIENTED_EDGE('',*,*,#10692,.F.);
#14612=ORIENTED_EDGE('',*,*,#10693,.T.);
#14613=ORIENTED_EDGE('',*,*,#10694,.T.);
#14614=ORIENTED_EDGE('',*,*,#10690,.F.);
#14615=ORIENTED_EDGE('',*,*,#10695,.F.);
#14616=ORIENTED_EDGE('',*,*,#10696,.T.);
#14617=ORIENTED_EDGE('',*,*,#10697,.T.);
#14618=ORIENTED_EDGE('',*,*,#10693,.F.);
#14619=ORIENTED_EDGE('',*,*,#10698,.F.);
#14620=ORIENTED_EDGE('',*,*,#10699,.T.);
#14621=ORIENTED_EDGE('',*,*,#10700,.T.);
#14622=ORIENTED_EDGE('',*,*,#10696,.F.);
#14623=ORIENTED_EDGE('',*,*,#10701,.F.);
#14624=ORIENTED_EDGE('',*,*,#10702,.T.);
#14625=ORIENTED_EDGE('',*,*,#10703,.T.);
#14626=ORIENTED_EDGE('',*,*,#10699,.F.);
#14627=ORIENTED_EDGE('',*,*,#10704,.F.);
#14628=ORIENTED_EDGE('',*,*,#10705,.T.);
#14629=ORIENTED_EDGE('',*,*,#10706,.T.);
#14630=ORIENTED_EDGE('',*,*,#10702,.F.);
#14631=ORIENTED_EDGE('',*,*,#10707,.F.);
#14632=ORIENTED_EDGE('',*,*,#10708,.T.);
#14633=ORIENTED_EDGE('',*,*,#10709,.T.);
#14634=ORIENTED_EDGE('',*,*,#10705,.F.);
#14635=ORIENTED_EDGE('',*,*,#10710,.F.);
#14636=ORIENTED_EDGE('',*,*,#10711,.T.);
#14637=ORIENTED_EDGE('',*,*,#10712,.T.);
#14638=ORIENTED_EDGE('',*,*,#10708,.F.);
#14639=ORIENTED_EDGE('',*,*,#10713,.F.);
#14640=ORIENTED_EDGE('',*,*,#10714,.T.);
#14641=ORIENTED_EDGE('',*,*,#10715,.T.);
#14642=ORIENTED_EDGE('',*,*,#10711,.F.);
#14643=ORIENTED_EDGE('',*,*,#10716,.F.);
#14644=ORIENTED_EDGE('',*,*,#10717,.F.);
#14645=ORIENTED_EDGE('',*,*,#10718,.F.);
#14646=ORIENTED_EDGE('',*,*,#10719,.F.);
#14647=ORIENTED_EDGE('',*,*,#10720,.T.);
#14648=ORIENTED_EDGE('',*,*,#10476,.F.);
#14649=ORIENTED_EDGE('',*,*,#10721,.T.);
#14650=ORIENTED_EDGE('',*,*,#10601,.T.);
#14651=ORIENTED_EDGE('',*,*,#10722,.T.);
#14652=ORIENTED_EDGE('',*,*,#10479,.F.);
#14653=ORIENTED_EDGE('',*,*,#10717,.T.);
#14654=ORIENTED_EDGE('',*,*,#10723,.T.);
#14655=ORIENTED_EDGE('',*,*,#10714,.F.);
#14656=ORIENTED_EDGE('',*,*,#10724,.F.);
#14657=ORIENTED_EDGE('',*,*,#10722,.F.);
#14658=ORIENTED_EDGE('',*,*,#10600,.F.);
#14659=ORIENTED_EDGE('',*,*,#10604,.F.);
#14660=ORIENTED_EDGE('',*,*,#10607,.F.);
#14661=ORIENTED_EDGE('',*,*,#10610,.F.);
#14662=ORIENTED_EDGE('',*,*,#10613,.F.);
#14663=ORIENTED_EDGE('',*,*,#10616,.F.);
#14664=ORIENTED_EDGE('',*,*,#10619,.F.);
#14665=ORIENTED_EDGE('',*,*,#10622,.F.);
#14666=ORIENTED_EDGE('',*,*,#10625,.F.);
#14667=ORIENTED_EDGE('',*,*,#10628,.F.);
#14668=ORIENTED_EDGE('',*,*,#10631,.F.);
#14669=ORIENTED_EDGE('',*,*,#10634,.F.);
#14670=ORIENTED_EDGE('',*,*,#10637,.F.);
#14671=ORIENTED_EDGE('',*,*,#10640,.F.);
#14672=ORIENTED_EDGE('',*,*,#10643,.F.);
#14673=ORIENTED_EDGE('',*,*,#10646,.F.);
#14674=ORIENTED_EDGE('',*,*,#10649,.F.);
#14675=ORIENTED_EDGE('',*,*,#10652,.F.);
#14676=ORIENTED_EDGE('',*,*,#10655,.F.);
#14677=ORIENTED_EDGE('',*,*,#10658,.F.);
#14678=ORIENTED_EDGE('',*,*,#10661,.F.);
#14679=ORIENTED_EDGE('',*,*,#10664,.F.);
#14680=ORIENTED_EDGE('',*,*,#10667,.F.);
#14681=ORIENTED_EDGE('',*,*,#10670,.F.);
#14682=ORIENTED_EDGE('',*,*,#10673,.F.);
#14683=ORIENTED_EDGE('',*,*,#10676,.F.);
#14684=ORIENTED_EDGE('',*,*,#10679,.F.);
#14685=ORIENTED_EDGE('',*,*,#10682,.F.);
#14686=ORIENTED_EDGE('',*,*,#10685,.F.);
#14687=ORIENTED_EDGE('',*,*,#10688,.F.);
#14688=ORIENTED_EDGE('',*,*,#10691,.F.);
#14689=ORIENTED_EDGE('',*,*,#10694,.F.);
#14690=ORIENTED_EDGE('',*,*,#10697,.F.);
#14691=ORIENTED_EDGE('',*,*,#10700,.F.);
#14692=ORIENTED_EDGE('',*,*,#10703,.F.);
#14693=ORIENTED_EDGE('',*,*,#10706,.F.);
#14694=ORIENTED_EDGE('',*,*,#10709,.F.);
#14695=ORIENTED_EDGE('',*,*,#10712,.F.);
#14696=ORIENTED_EDGE('',*,*,#10715,.F.);
#14697=ORIENTED_EDGE('',*,*,#10723,.F.);
#14698=ORIENTED_EDGE('',*,*,#10720,.F.);
#14699=ORIENTED_EDGE('',*,*,#10725,.F.);
#14700=ORIENTED_EDGE('',*,*,#10596,.F.);
#14701=ORIENTED_EDGE('',*,*,#10726,.F.);
#14702=ORIENTED_EDGE('',*,*,#10594,.F.);
#14703=ORIENTED_EDGE('',*,*,#10591,.F.);
#14704=ORIENTED_EDGE('',*,*,#10588,.F.);
#14705=ORIENTED_EDGE('',*,*,#10585,.F.);
#14706=ORIENTED_EDGE('',*,*,#10582,.F.);
#14707=ORIENTED_EDGE('',*,*,#10579,.F.);
#14708=ORIENTED_EDGE('',*,*,#10576,.F.);
#14709=ORIENTED_EDGE('',*,*,#10573,.F.);
#14710=ORIENTED_EDGE('',*,*,#10570,.F.);
#14711=ORIENTED_EDGE('',*,*,#10567,.F.);
#14712=ORIENTED_EDGE('',*,*,#10564,.F.);
#14713=ORIENTED_EDGE('',*,*,#10561,.F.);
#14714=ORIENTED_EDGE('',*,*,#10558,.F.);
#14715=ORIENTED_EDGE('',*,*,#10555,.F.);
#14716=ORIENTED_EDGE('',*,*,#10552,.F.);
#14717=ORIENTED_EDGE('',*,*,#10549,.F.);
#14718=ORIENTED_EDGE('',*,*,#10546,.F.);
#14719=ORIENTED_EDGE('',*,*,#10543,.F.);
#14720=ORIENTED_EDGE('',*,*,#10540,.F.);
#14721=ORIENTED_EDGE('',*,*,#10537,.F.);
#14722=ORIENTED_EDGE('',*,*,#10534,.F.);
#14723=ORIENTED_EDGE('',*,*,#10531,.F.);
#14724=ORIENTED_EDGE('',*,*,#10528,.F.);
#14725=ORIENTED_EDGE('',*,*,#10525,.F.);
#14726=ORIENTED_EDGE('',*,*,#10522,.F.);
#14727=ORIENTED_EDGE('',*,*,#10519,.F.);
#14728=ORIENTED_EDGE('',*,*,#10516,.F.);
#14729=ORIENTED_EDGE('',*,*,#10513,.F.);
#14730=ORIENTED_EDGE('',*,*,#10510,.F.);
#14731=ORIENTED_EDGE('',*,*,#10507,.F.);
#14732=ORIENTED_EDGE('',*,*,#10504,.F.);
#14733=ORIENTED_EDGE('',*,*,#10501,.F.);
#14734=ORIENTED_EDGE('',*,*,#10498,.F.);
#14735=ORIENTED_EDGE('',*,*,#10495,.F.);
#14736=ORIENTED_EDGE('',*,*,#10492,.F.);
#14737=ORIENTED_EDGE('',*,*,#10489,.F.);
#14738=ORIENTED_EDGE('',*,*,#10486,.F.);
#14739=ORIENTED_EDGE('',*,*,#10483,.F.);
#14740=ORIENTED_EDGE('',*,*,#10480,.F.);
#14741=ORIENTED_EDGE('',*,*,#10721,.F.);
#14742=ORIENTED_EDGE('',*,*,#10475,.F.);
#14743=ORIENTED_EDGE('',*,*,#10482,.F.);
#14744=ORIENTED_EDGE('',*,*,#10485,.F.);
#14745=ORIENTED_EDGE('',*,*,#10488,.F.);
#14746=ORIENTED_EDGE('',*,*,#10491,.F.);
#14747=ORIENTED_EDGE('',*,*,#10494,.F.);
#14748=ORIENTED_EDGE('',*,*,#10497,.F.);
#14749=ORIENTED_EDGE('',*,*,#10500,.F.);
#14750=ORIENTED_EDGE('',*,*,#10503,.F.);
#14751=ORIENTED_EDGE('',*,*,#10506,.F.);
#14752=ORIENTED_EDGE('',*,*,#10509,.F.);
#14753=ORIENTED_EDGE('',*,*,#10512,.F.);
#14754=ORIENTED_EDGE('',*,*,#10515,.F.);
#14755=ORIENTED_EDGE('',*,*,#10518,.F.);
#14756=ORIENTED_EDGE('',*,*,#10521,.F.);
#14757=ORIENTED_EDGE('',*,*,#10524,.F.);
#14758=ORIENTED_EDGE('',*,*,#10527,.F.);
#14759=ORIENTED_EDGE('',*,*,#10530,.F.);
#14760=ORIENTED_EDGE('',*,*,#10533,.F.);
#14761=ORIENTED_EDGE('',*,*,#10536,.F.);
#14762=ORIENTED_EDGE('',*,*,#10539,.F.);
#14763=ORIENTED_EDGE('',*,*,#10542,.F.);
#14764=ORIENTED_EDGE('',*,*,#10545,.F.);
#14765=ORIENTED_EDGE('',*,*,#10548,.F.);
#14766=ORIENTED_EDGE('',*,*,#10551,.F.);
#14767=ORIENTED_EDGE('',*,*,#10554,.F.);
#14768=ORIENTED_EDGE('',*,*,#10557,.F.);
#14769=ORIENTED_EDGE('',*,*,#10560,.F.);
#14770=ORIENTED_EDGE('',*,*,#10563,.F.);
#14771=ORIENTED_EDGE('',*,*,#10566,.F.);
#14772=ORIENTED_EDGE('',*,*,#10569,.F.);
#14773=ORIENTED_EDGE('',*,*,#10572,.F.);
#14774=ORIENTED_EDGE('',*,*,#10575,.F.);
#14775=ORIENTED_EDGE('',*,*,#10578,.F.);
#14776=ORIENTED_EDGE('',*,*,#10581,.F.);
#14777=ORIENTED_EDGE('',*,*,#10584,.F.);
#14778=ORIENTED_EDGE('',*,*,#10587,.F.);
#14779=ORIENTED_EDGE('',*,*,#10590,.F.);
#14780=ORIENTED_EDGE('',*,*,#10593,.F.);
#14781=ORIENTED_EDGE('',*,*,#10727,.F.);
#14782=ORIENTED_EDGE('',*,*,#10598,.F.);
#14783=ORIENTED_EDGE('',*,*,#10728,.F.);
#14784=ORIENTED_EDGE('',*,*,#10718,.T.);
#14785=ORIENTED_EDGE('',*,*,#10724,.T.);
#14786=ORIENTED_EDGE('',*,*,#10716,.T.);
#14787=ORIENTED_EDGE('',*,*,#10713,.T.);
#14788=ORIENTED_EDGE('',*,*,#10710,.T.);
#14789=ORIENTED_EDGE('',*,*,#10707,.T.);
#14790=ORIENTED_EDGE('',*,*,#10704,.T.);
#14791=ORIENTED_EDGE('',*,*,#10701,.T.);
#14792=ORIENTED_EDGE('',*,*,#10698,.T.);
#14793=ORIENTED_EDGE('',*,*,#10695,.T.);
#14794=ORIENTED_EDGE('',*,*,#10692,.T.);
#14795=ORIENTED_EDGE('',*,*,#10689,.T.);
#14796=ORIENTED_EDGE('',*,*,#10686,.T.);
#14797=ORIENTED_EDGE('',*,*,#10683,.T.);
#14798=ORIENTED_EDGE('',*,*,#10680,.T.);
#14799=ORIENTED_EDGE('',*,*,#10677,.T.);
#14800=ORIENTED_EDGE('',*,*,#10674,.T.);
#14801=ORIENTED_EDGE('',*,*,#10671,.T.);
#14802=ORIENTED_EDGE('',*,*,#10668,.T.);
#14803=ORIENTED_EDGE('',*,*,#10665,.T.);
#14804=ORIENTED_EDGE('',*,*,#10662,.T.);
#14805=ORIENTED_EDGE('',*,*,#10659,.T.);
#14806=ORIENTED_EDGE('',*,*,#10656,.T.);
#14807=ORIENTED_EDGE('',*,*,#10653,.T.);
#14808=ORIENTED_EDGE('',*,*,#10650,.T.);
#14809=ORIENTED_EDGE('',*,*,#10647,.T.);
#14810=ORIENTED_EDGE('',*,*,#10644,.T.);
#14811=ORIENTED_EDGE('',*,*,#10641,.T.);
#14812=ORIENTED_EDGE('',*,*,#10638,.T.);
#14813=ORIENTED_EDGE('',*,*,#10635,.T.);
#14814=ORIENTED_EDGE('',*,*,#10632,.T.);
#14815=ORIENTED_EDGE('',*,*,#10629,.T.);
#14816=ORIENTED_EDGE('',*,*,#10626,.T.);
#14817=ORIENTED_EDGE('',*,*,#10623,.T.);
#14818=ORIENTED_EDGE('',*,*,#10620,.T.);
#14819=ORIENTED_EDGE('',*,*,#10617,.T.);
#14820=ORIENTED_EDGE('',*,*,#10614,.T.);
#14821=ORIENTED_EDGE('',*,*,#10611,.T.);
#14822=ORIENTED_EDGE('',*,*,#10608,.T.);
#14823=ORIENTED_EDGE('',*,*,#10605,.T.);
#14824=ORIENTED_EDGE('',*,*,#10602,.T.);
#14825=ORIENTED_EDGE('',*,*,#10595,.T.);
#14826=ORIENTED_EDGE('',*,*,#10727,.T.);
#14827=ORIENTED_EDGE('',*,*,#10592,.F.);
#14828=ORIENTED_EDGE('',*,*,#10726,.T.);
#14829=ORIENTED_EDGE('',*,*,#10478,.F.);
#14830=ORIENTED_EDGE('',*,*,#10729,.F.);
#14831=ORIENTED_EDGE('',*,*,#10319,.F.);
#14832=ORIENTED_EDGE('',*,*,#10730,.T.);
#14833=ORIENTED_EDGE('',*,*,#10399,.T.);
#14834=ORIENTED_EDGE('',*,*,#10731,.T.);
#14835=ORIENTED_EDGE('',*,*,#10322,.F.);
#14836=ORIENTED_EDGE('',*,*,#10470,.T.);
#14837=ORIENTED_EDGE('',*,*,#10732,.T.);
#14838=ORIENTED_EDGE('',*,*,#10467,.F.);
#14839=ORIENTED_EDGE('',*,*,#10733,.F.);
#14840=ORIENTED_EDGE('',*,*,#10731,.F.);
#14841=ORIENTED_EDGE('',*,*,#10398,.F.);
#14842=ORIENTED_EDGE('',*,*,#10402,.F.);
#14843=ORIENTED_EDGE('',*,*,#10405,.F.);
#14844=ORIENTED_EDGE('',*,*,#10408,.F.);
#14845=ORIENTED_EDGE('',*,*,#10411,.F.);
#14846=ORIENTED_EDGE('',*,*,#10414,.F.);
#14847=ORIENTED_EDGE('',*,*,#10417,.F.);
#14848=ORIENTED_EDGE('',*,*,#10420,.F.);
#14849=ORIENTED_EDGE('',*,*,#10423,.F.);
#14850=ORIENTED_EDGE('',*,*,#10426,.F.);
#14851=ORIENTED_EDGE('',*,*,#10429,.F.);
#14852=ORIENTED_EDGE('',*,*,#10432,.F.);
#14853=ORIENTED_EDGE('',*,*,#10435,.F.);
#14854=ORIENTED_EDGE('',*,*,#10438,.F.);
#14855=ORIENTED_EDGE('',*,*,#10441,.F.);
#14856=ORIENTED_EDGE('',*,*,#10444,.F.);
#14857=ORIENTED_EDGE('',*,*,#10447,.F.);
#14858=ORIENTED_EDGE('',*,*,#10450,.F.);
#14859=ORIENTED_EDGE('',*,*,#10453,.F.);
#14860=ORIENTED_EDGE('',*,*,#10456,.F.);
#14861=ORIENTED_EDGE('',*,*,#10459,.F.);
#14862=ORIENTED_EDGE('',*,*,#10462,.F.);
#14863=ORIENTED_EDGE('',*,*,#10465,.F.);
#14864=ORIENTED_EDGE('',*,*,#10468,.F.);
#14865=ORIENTED_EDGE('',*,*,#10732,.F.);
#14866=ORIENTED_EDGE('',*,*,#10473,.F.);
#14867=ORIENTED_EDGE('',*,*,#10734,.F.);
#14868=ORIENTED_EDGE('',*,*,#10394,.F.);
#14869=ORIENTED_EDGE('',*,*,#10735,.F.);
#14870=ORIENTED_EDGE('',*,*,#10392,.F.);
#14871=ORIENTED_EDGE('',*,*,#10389,.F.);
#14872=ORIENTED_EDGE('',*,*,#10386,.F.);
#14873=ORIENTED_EDGE('',*,*,#10383,.F.);
#14874=ORIENTED_EDGE('',*,*,#10380,.F.);
#14875=ORIENTED_EDGE('',*,*,#10377,.F.);
#14876=ORIENTED_EDGE('',*,*,#10374,.F.);
#14877=ORIENTED_EDGE('',*,*,#10371,.F.);
#14878=ORIENTED_EDGE('',*,*,#10368,.F.);
#14879=ORIENTED_EDGE('',*,*,#10365,.F.);
#14880=ORIENTED_EDGE('',*,*,#10362,.F.);
#14881=ORIENTED_EDGE('',*,*,#10359,.F.);
#14882=ORIENTED_EDGE('',*,*,#10356,.F.);
#14883=ORIENTED_EDGE('',*,*,#10353,.F.);
#14884=ORIENTED_EDGE('',*,*,#10350,.F.);
#14885=ORIENTED_EDGE('',*,*,#10347,.F.);
#14886=ORIENTED_EDGE('',*,*,#10344,.F.);
#14887=ORIENTED_EDGE('',*,*,#10341,.F.);
#14888=ORIENTED_EDGE('',*,*,#10338,.F.);
#14889=ORIENTED_EDGE('',*,*,#10335,.F.);
#14890=ORIENTED_EDGE('',*,*,#10332,.F.);
#14891=ORIENTED_EDGE('',*,*,#10329,.F.);
#14892=ORIENTED_EDGE('',*,*,#10326,.F.);
#14893=ORIENTED_EDGE('',*,*,#10323,.F.);
#14894=ORIENTED_EDGE('',*,*,#10730,.F.);
#14895=ORIENTED_EDGE('',*,*,#10318,.F.);
#14896=ORIENTED_EDGE('',*,*,#10325,.F.);
#14897=ORIENTED_EDGE('',*,*,#10328,.F.);
#14898=ORIENTED_EDGE('',*,*,#10331,.F.);
#14899=ORIENTED_EDGE('',*,*,#10334,.F.);
#14900=ORIENTED_EDGE('',*,*,#10337,.F.);
#14901=ORIENTED_EDGE('',*,*,#10340,.F.);
#14902=ORIENTED_EDGE('',*,*,#10343,.F.);
#14903=ORIENTED_EDGE('',*,*,#10346,.F.);
#14904=ORIENTED_EDGE('',*,*,#10349,.F.);
#14905=ORIENTED_EDGE('',*,*,#10352,.F.);
#14906=ORIENTED_EDGE('',*,*,#10355,.F.);
#14907=ORIENTED_EDGE('',*,*,#10358,.F.);
#14908=ORIENTED_EDGE('',*,*,#10361,.F.);
#14909=ORIENTED_EDGE('',*,*,#10364,.F.);
#14910=ORIENTED_EDGE('',*,*,#10367,.F.);
#14911=ORIENTED_EDGE('',*,*,#10370,.F.);
#14912=ORIENTED_EDGE('',*,*,#10373,.F.);
#14913=ORIENTED_EDGE('',*,*,#10376,.F.);
#14914=ORIENTED_EDGE('',*,*,#10379,.F.);
#14915=ORIENTED_EDGE('',*,*,#10382,.F.);
#14916=ORIENTED_EDGE('',*,*,#10385,.F.);
#14917=ORIENTED_EDGE('',*,*,#10388,.F.);
#14918=ORIENTED_EDGE('',*,*,#10391,.F.);
#14919=ORIENTED_EDGE('',*,*,#10736,.F.);
#14920=ORIENTED_EDGE('',*,*,#10396,.F.);
#14921=ORIENTED_EDGE('',*,*,#10737,.F.);
#14922=ORIENTED_EDGE('',*,*,#10471,.T.);
#14923=ORIENTED_EDGE('',*,*,#10733,.T.);
#14924=ORIENTED_EDGE('',*,*,#10469,.T.);
#14925=ORIENTED_EDGE('',*,*,#10466,.T.);
#14926=ORIENTED_EDGE('',*,*,#10463,.T.);
#14927=ORIENTED_EDGE('',*,*,#10460,.T.);
#14928=ORIENTED_EDGE('',*,*,#10457,.T.);
#14929=ORIENTED_EDGE('',*,*,#10454,.T.);
#14930=ORIENTED_EDGE('',*,*,#10451,.T.);
#14931=ORIENTED_EDGE('',*,*,#10448,.T.);
#14932=ORIENTED_EDGE('',*,*,#10445,.T.);
#14933=ORIENTED_EDGE('',*,*,#10442,.T.);
#14934=ORIENTED_EDGE('',*,*,#10439,.T.);
#14935=ORIENTED_EDGE('',*,*,#10436,.T.);
#14936=ORIENTED_EDGE('',*,*,#10433,.T.);
#14937=ORIENTED_EDGE('',*,*,#10430,.T.);
#14938=ORIENTED_EDGE('',*,*,#10427,.T.);
#14939=ORIENTED_EDGE('',*,*,#10424,.T.);
#14940=ORIENTED_EDGE('',*,*,#10421,.T.);
#14941=ORIENTED_EDGE('',*,*,#10418,.T.);
#14942=ORIENTED_EDGE('',*,*,#10415,.T.);
#14943=ORIENTED_EDGE('',*,*,#10412,.T.);
#14944=ORIENTED_EDGE('',*,*,#10409,.T.);
#14945=ORIENTED_EDGE('',*,*,#10406,.T.);
#14946=ORIENTED_EDGE('',*,*,#10403,.T.);
#14947=ORIENTED_EDGE('',*,*,#10400,.T.);
#14948=ORIENTED_EDGE('',*,*,#10393,.T.);
#14949=ORIENTED_EDGE('',*,*,#10736,.T.);
#14950=ORIENTED_EDGE('',*,*,#10390,.F.);
#14951=ORIENTED_EDGE('',*,*,#10735,.T.);
#14952=ORIENTED_EDGE('',*,*,#10321,.F.);
#14953=ORIENTED_EDGE('',*,*,#10738,.F.);
#14954=ORIENTED_EDGE('',*,*,#10739,.T.);
#14955=ORIENTED_EDGE('',*,*,#10740,.T.);
#14956=ORIENTED_EDGE('',*,*,#10741,.T.);
#14957=ORIENTED_EDGE('',*,*,#10742,.T.);
#14958=ORIENTED_EDGE('',*,*,#10740,.F.);
#14959=ORIENTED_EDGE('',*,*,#10743,.F.);
#14960=ORIENTED_EDGE('',*,*,#10744,.F.);
#14961=ORIENTED_EDGE('',*,*,#10745,.F.);
#14962=ORIENTED_EDGE('',*,*,#10739,.F.);
#14963=ORIENTED_EDGE('',*,*,#10746,.T.);
#14964=ORIENTED_EDGE('',*,*,#10747,.F.);
#14965=ORIENTED_EDGE('',*,*,#10748,.T.);
#14966=ORIENTED_EDGE('',*,*,#10749,.F.);
#14967=ORIENTED_EDGE('',*,*,#10750,.T.);
#14968=ORIENTED_EDGE('',*,*,#10751,.F.);
#14969=ORIENTED_EDGE('',*,*,#10752,.T.);
#14970=ORIENTED_EDGE('',*,*,#10753,.F.);
#14971=ORIENTED_EDGE('',*,*,#10754,.T.);
#14972=ORIENTED_EDGE('',*,*,#10755,.F.);
#14973=ORIENTED_EDGE('',*,*,#10756,.T.);
#14974=ORIENTED_EDGE('',*,*,#10757,.F.);
#14975=ORIENTED_EDGE('',*,*,#10758,.T.);
#14976=ORIENTED_EDGE('',*,*,#10759,.F.);
#14977=ORIENTED_EDGE('',*,*,#10760,.T.);
#14978=ORIENTED_EDGE('',*,*,#10761,.F.);
#14979=ORIENTED_EDGE('',*,*,#10762,.T.);
#14980=ORIENTED_EDGE('',*,*,#10763,.F.);
#14981=ORIENTED_EDGE('',*,*,#10764,.T.);
#14982=ORIENTED_EDGE('',*,*,#10765,.F.);
#14983=ORIENTED_EDGE('',*,*,#10766,.T.);
#14984=ORIENTED_EDGE('',*,*,#10767,.F.);
#14985=ORIENTED_EDGE('',*,*,#10768,.T.);
#14986=ORIENTED_EDGE('',*,*,#10769,.F.);
#14987=ORIENTED_EDGE('',*,*,#10770,.T.);
#14988=ORIENTED_EDGE('',*,*,#10771,.F.);
#14989=ORIENTED_EDGE('',*,*,#10772,.T.);
#14990=ORIENTED_EDGE('',*,*,#10773,.F.);
#14991=ORIENTED_EDGE('',*,*,#10774,.T.);
#14992=ORIENTED_EDGE('',*,*,#10775,.F.);
#14993=ORIENTED_EDGE('',*,*,#10776,.T.);
#14994=ORIENTED_EDGE('',*,*,#10777,.F.);
#14995=ORIENTED_EDGE('',*,*,#10778,.T.);
#14996=ORIENTED_EDGE('',*,*,#10779,.F.);
#14997=ORIENTED_EDGE('',*,*,#10780,.T.);
#14998=ORIENTED_EDGE('',*,*,#10781,.F.);
#14999=ORIENTED_EDGE('',*,*,#10782,.T.);
#15000=ORIENTED_EDGE('',*,*,#10783,.F.);
#15001=ORIENTED_EDGE('',*,*,#10784,.T.);
#15002=ORIENTED_EDGE('',*,*,#10785,.F.);
#15003=ORIENTED_EDGE('',*,*,#10786,.T.);
#15004=ORIENTED_EDGE('',*,*,#10787,.F.);
#15005=ORIENTED_EDGE('',*,*,#10788,.T.);
#15006=ORIENTED_EDGE('',*,*,#10789,.F.);
#15007=ORIENTED_EDGE('',*,*,#10790,.T.);
#15008=ORIENTED_EDGE('',*,*,#10791,.F.);
#15009=ORIENTED_EDGE('',*,*,#10792,.T.);
#15010=ORIENTED_EDGE('',*,*,#10793,.F.);
#15011=ORIENTED_EDGE('',*,*,#10794,.T.);
#15012=ORIENTED_EDGE('',*,*,#10795,.F.);
#15013=ORIENTED_EDGE('',*,*,#10796,.T.);
#15014=ORIENTED_EDGE('',*,*,#10797,.F.);
#15015=ORIENTED_EDGE('',*,*,#10798,.T.);
#15016=ORIENTED_EDGE('',*,*,#10799,.F.);
#15017=ORIENTED_EDGE('',*,*,#10800,.T.);
#15018=ORIENTED_EDGE('',*,*,#10801,.F.);
#15019=ORIENTED_EDGE('',*,*,#10802,.T.);
#15020=ORIENTED_EDGE('',*,*,#10803,.F.);
#15021=ORIENTED_EDGE('',*,*,#10804,.T.);
#15022=ORIENTED_EDGE('',*,*,#10805,.F.);
#15023=ORIENTED_EDGE('',*,*,#10806,.T.);
#15024=ORIENTED_EDGE('',*,*,#10807,.F.);
#15025=ORIENTED_EDGE('',*,*,#10808,.T.);
#15026=ORIENTED_EDGE('',*,*,#10809,.F.);
#15027=ORIENTED_EDGE('',*,*,#10810,.T.);
#15028=ORIENTED_EDGE('',*,*,#10811,.F.);
#15029=ORIENTED_EDGE('',*,*,#10812,.T.);
#15030=ORIENTED_EDGE('',*,*,#10813,.F.);
#15031=ORIENTED_EDGE('',*,*,#10814,.T.);
#15032=ORIENTED_EDGE('',*,*,#10815,.F.);
#15033=ORIENTED_EDGE('',*,*,#10743,.T.);
#15034=ORIENTED_EDGE('',*,*,#10737,.T.);
#15035=ORIENTED_EDGE('',*,*,#10395,.T.);
#15036=ORIENTED_EDGE('',*,*,#10734,.T.);
#15037=ORIENTED_EDGE('',*,*,#10472,.T.);
#15038=ORIENTED_EDGE('',*,*,#10816,.T.);
#15039=ORIENTED_EDGE('',*,*,#10817,.T.);
#15040=ORIENTED_EDGE('',*,*,#10818,.T.);
#15041=ORIENTED_EDGE('',*,*,#10819,.T.);
#15042=ORIENTED_EDGE('',*,*,#10820,.T.);
#15043=ORIENTED_EDGE('',*,*,#10821,.T.);
#15044=ORIENTED_EDGE('',*,*,#10747,.T.);
#15045=ORIENTED_EDGE('',*,*,#10822,.T.);
#15046=ORIENTED_EDGE('',*,*,#10821,.F.);
#15047=ORIENTED_EDGE('',*,*,#10823,.F.);
#15048=ORIENTED_EDGE('',*,*,#10824,.F.);
#15049=ORIENTED_EDGE('',*,*,#10748,.F.);
#15050=ORIENTED_EDGE('',*,*,#10825,.T.);
#15051=ORIENTED_EDGE('',*,*,#10826,.T.);
#15052=ORIENTED_EDGE('',*,*,#10749,.T.);
#15053=ORIENTED_EDGE('',*,*,#10824,.T.);
#15054=ORIENTED_EDGE('',*,*,#10826,.F.);
#15055=ORIENTED_EDGE('',*,*,#10827,.F.);
#15056=ORIENTED_EDGE('',*,*,#10828,.F.);
#15057=ORIENTED_EDGE('',*,*,#10750,.F.);
#15058=ORIENTED_EDGE('',*,*,#10829,.T.);
#15059=ORIENTED_EDGE('',*,*,#10830,.T.);
#15060=ORIENTED_EDGE('',*,*,#10751,.T.);
#15061=ORIENTED_EDGE('',*,*,#10828,.T.);
#15062=ORIENTED_EDGE('',*,*,#10830,.F.);
#15063=ORIENTED_EDGE('',*,*,#10831,.F.);
#15064=ORIENTED_EDGE('',*,*,#10832,.F.);
#15065=ORIENTED_EDGE('',*,*,#10752,.F.);
#15066=ORIENTED_EDGE('',*,*,#10833,.T.);
#15067=ORIENTED_EDGE('',*,*,#10834,.T.);
#15068=ORIENTED_EDGE('',*,*,#10753,.T.);
#15069=ORIENTED_EDGE('',*,*,#10832,.T.);
#15070=ORIENTED_EDGE('',*,*,#10834,.F.);
#15071=ORIENTED_EDGE('',*,*,#10835,.F.);
#15072=ORIENTED_EDGE('',*,*,#10836,.F.);
#15073=ORIENTED_EDGE('',*,*,#10754,.F.);
#15074=ORIENTED_EDGE('',*,*,#10755,.T.);
#15075=ORIENTED_EDGE('',*,*,#10836,.T.);
#15076=ORIENTED_EDGE('',*,*,#10837,.T.);
#15077=ORIENTED_EDGE('',*,*,#10838,.T.);
#15078=ORIENTED_EDGE('',*,*,#10757,.T.);
#15079=ORIENTED_EDGE('',*,*,#10839,.T.);
#15080=ORIENTED_EDGE('',*,*,#10840,.T.);
#15081=ORIENTED_EDGE('',*,*,#10841,.T.);
#15082=ORIENTED_EDGE('',*,*,#10841,.F.);
#15083=ORIENTED_EDGE('',*,*,#10842,.F.);
#15084=ORIENTED_EDGE('',*,*,#10843,.F.);
#15085=ORIENTED_EDGE('',*,*,#10758,.F.);
#15086=ORIENTED_EDGE('',*,*,#10759,.T.);
#15087=ORIENTED_EDGE('',*,*,#10843,.T.);
#15088=ORIENTED_EDGE('',*,*,#10844,.T.);
#15089=ORIENTED_EDGE('',*,*,#10845,.T.);
#15090=ORIENTED_EDGE('',*,*,#10761,.T.);
#15091=ORIENTED_EDGE('',*,*,#10846,.T.);
#15092=ORIENTED_EDGE('',*,*,#10847,.T.);
#15093=ORIENTED_EDGE('',*,*,#10848,.T.);
#15094=ORIENTED_EDGE('',*,*,#10848,.F.);
#15095=ORIENTED_EDGE('',*,*,#10849,.F.);
#15096=ORIENTED_EDGE('',*,*,#10850,.F.);
#15097=ORIENTED_EDGE('',*,*,#10762,.F.);
#15098=ORIENTED_EDGE('',*,*,#10763,.T.);
#15099=ORIENTED_EDGE('',*,*,#10850,.T.);
#15100=ORIENTED_EDGE('',*,*,#10851,.T.);
#15101=ORIENTED_EDGE('',*,*,#10852,.T.);
#15102=ORIENTED_EDGE('',*,*,#10853,.T.);
#15103=ORIENTED_EDGE('',*,*,#10854,.T.);
#15104=ORIENTED_EDGE('',*,*,#10765,.T.);
#15105=ORIENTED_EDGE('',*,*,#10855,.T.);
#15106=ORIENTED_EDGE('',*,*,#10854,.F.);
#15107=ORIENTED_EDGE('',*,*,#10856,.F.);
#15108=ORIENTED_EDGE('',*,*,#10857,.F.);
#15109=ORIENTED_EDGE('',*,*,#10766,.F.);
#15110=ORIENTED_EDGE('',*,*,#10858,.T.);
#15111=ORIENTED_EDGE('',*,*,#10859,.T.);
#15112=ORIENTED_EDGE('',*,*,#10767,.T.);
#15113=ORIENTED_EDGE('',*,*,#10857,.T.);
#15114=ORIENTED_EDGE('',*,*,#10859,.F.);
#15115=ORIENTED_EDGE('',*,*,#10860,.F.);
#15116=ORIENTED_EDGE('',*,*,#10861,.F.);
#15117=ORIENTED_EDGE('',*,*,#10768,.F.);
#15118=ORIENTED_EDGE('',*,*,#10862,.T.);
#15119=ORIENTED_EDGE('',*,*,#10863,.T.);
#15120=ORIENTED_EDGE('',*,*,#10769,.T.);
#15121=ORIENTED_EDGE('',*,*,#10861,.T.);
#15122=ORIENTED_EDGE('',*,*,#10863,.F.);
#15123=ORIENTED_EDGE('',*,*,#10864,.F.);
#15124=ORIENTED_EDGE('',*,*,#10865,.F.);
#15125=ORIENTED_EDGE('',*,*,#10770,.F.);
#15126=ORIENTED_EDGE('',*,*,#10866,.T.);
#15127=ORIENTED_EDGE('',*,*,#10867,.T.);
#15128=ORIENTED_EDGE('',*,*,#10771,.T.);
#15129=ORIENTED_EDGE('',*,*,#10865,.T.);
#15130=ORIENTED_EDGE('',*,*,#10867,.F.);
#15131=ORIENTED_EDGE('',*,*,#10868,.F.);
#15132=ORIENTED_EDGE('',*,*,#10869,.F.);
#15133=ORIENTED_EDGE('',*,*,#10772,.F.);
#15134=ORIENTED_EDGE('',*,*,#10773,.T.);
#15135=ORIENTED_EDGE('',*,*,#10869,.T.);
#15136=ORIENTED_EDGE('',*,*,#10870,.T.);
#15137=ORIENTED_EDGE('',*,*,#10871,.T.);
#15138=ORIENTED_EDGE('',*,*,#10775,.T.);
#15139=ORIENTED_EDGE('',*,*,#10872,.T.);
#15140=ORIENTED_EDGE('',*,*,#10873,.T.);
#15141=ORIENTED_EDGE('',*,*,#10874,.T.);
#15142=ORIENTED_EDGE('',*,*,#10874,.F.);
#15143=ORIENTED_EDGE('',*,*,#10875,.F.);
#15144=ORIENTED_EDGE('',*,*,#10876,.F.);
#15145=ORIENTED_EDGE('',*,*,#10776,.F.);
#15146=ORIENTED_EDGE('',*,*,#10777,.T.);
#15147=ORIENTED_EDGE('',*,*,#10876,.T.);
#15148=ORIENTED_EDGE('',*,*,#10877,.T.);
#15149=ORIENTED_EDGE('',*,*,#10878,.T.);
#15150=ORIENTED_EDGE('',*,*,#10779,.T.);
#15151=ORIENTED_EDGE('',*,*,#10879,.T.);
#15152=ORIENTED_EDGE('',*,*,#10880,.T.);
#15153=ORIENTED_EDGE('',*,*,#10881,.T.);
#15154=ORIENTED_EDGE('',*,*,#10881,.F.);
#15155=ORIENTED_EDGE('',*,*,#10882,.F.);
#15156=ORIENTED_EDGE('',*,*,#10883,.F.);
#15157=ORIENTED_EDGE('',*,*,#10780,.F.);
#15158=ORIENTED_EDGE('',*,*,#10781,.T.);
#15159=ORIENTED_EDGE('',*,*,#10883,.T.);
#15160=ORIENTED_EDGE('',*,*,#10884,.T.);
#15161=ORIENTED_EDGE('',*,*,#10885,.T.);
#15162=ORIENTED_EDGE('',*,*,#10886,.T.);
#15163=ORIENTED_EDGE('',*,*,#10887,.T.);
#15164=ORIENTED_EDGE('',*,*,#10783,.T.);
#15165=ORIENTED_EDGE('',*,*,#10888,.T.);
#15166=ORIENTED_EDGE('',*,*,#10887,.F.);
#15167=ORIENTED_EDGE('',*,*,#10889,.F.);
#15168=ORIENTED_EDGE('',*,*,#10890,.F.);
#15169=ORIENTED_EDGE('',*,*,#10784,.F.);
#15170=ORIENTED_EDGE('',*,*,#10891,.T.);
#15171=ORIENTED_EDGE('',*,*,#10892,.T.);
#15172=ORIENTED_EDGE('',*,*,#10785,.T.);
#15173=ORIENTED_EDGE('',*,*,#10890,.T.);
#15174=ORIENTED_EDGE('',*,*,#10892,.F.);
#15175=ORIENTED_EDGE('',*,*,#10893,.F.);
#15176=ORIENTED_EDGE('',*,*,#10894,.F.);
#15177=ORIENTED_EDGE('',*,*,#10786,.F.);
#15178=ORIENTED_EDGE('',*,*,#10895,.T.);
#15179=ORIENTED_EDGE('',*,*,#10896,.T.);
#15180=ORIENTED_EDGE('',*,*,#10787,.T.);
#15181=ORIENTED_EDGE('',*,*,#10894,.T.);
#15182=ORIENTED_EDGE('',*,*,#10896,.F.);
#15183=ORIENTED_EDGE('',*,*,#10897,.F.);
#15184=ORIENTED_EDGE('',*,*,#10898,.F.);
#15185=ORIENTED_EDGE('',*,*,#10788,.F.);
#15186=ORIENTED_EDGE('',*,*,#10899,.T.);
#15187=ORIENTED_EDGE('',*,*,#10900,.T.);
#15188=ORIENTED_EDGE('',*,*,#10789,.T.);
#15189=ORIENTED_EDGE('',*,*,#10898,.T.);
#15190=ORIENTED_EDGE('',*,*,#10900,.F.);
#15191=ORIENTED_EDGE('',*,*,#10901,.F.);
#15192=ORIENTED_EDGE('',*,*,#10902,.F.);
#15193=ORIENTED_EDGE('',*,*,#10790,.F.);
#15194=ORIENTED_EDGE('',*,*,#10791,.T.);
#15195=ORIENTED_EDGE('',*,*,#10902,.T.);
#15196=ORIENTED_EDGE('',*,*,#10903,.T.);
#15197=ORIENTED_EDGE('',*,*,#10904,.T.);
#15198=ORIENTED_EDGE('',*,*,#10793,.T.);
#15199=ORIENTED_EDGE('',*,*,#10905,.T.);
#15200=ORIENTED_EDGE('',*,*,#10906,.T.);
#15201=ORIENTED_EDGE('',*,*,#10907,.T.);
#15202=ORIENTED_EDGE('',*,*,#10907,.F.);
#15203=ORIENTED_EDGE('',*,*,#10908,.F.);
#15204=ORIENTED_EDGE('',*,*,#10909,.F.);
#15205=ORIENTED_EDGE('',*,*,#10794,.F.);
#15206=ORIENTED_EDGE('',*,*,#10795,.T.);
#15207=ORIENTED_EDGE('',*,*,#10909,.T.);
#15208=ORIENTED_EDGE('',*,*,#10910,.T.);
#15209=ORIENTED_EDGE('',*,*,#10911,.T.);
#15210=ORIENTED_EDGE('',*,*,#10797,.T.);
#15211=ORIENTED_EDGE('',*,*,#10912,.T.);
#15212=ORIENTED_EDGE('',*,*,#10913,.T.);
#15213=ORIENTED_EDGE('',*,*,#10914,.T.);
#15214=ORIENTED_EDGE('',*,*,#10914,.F.);
#15215=ORIENTED_EDGE('',*,*,#10915,.F.);
#15216=ORIENTED_EDGE('',*,*,#10916,.F.);
#15217=ORIENTED_EDGE('',*,*,#10798,.F.);
#15218=ORIENTED_EDGE('',*,*,#10799,.T.);
#15219=ORIENTED_EDGE('',*,*,#10916,.T.);
#15220=ORIENTED_EDGE('',*,*,#10917,.T.);
#15221=ORIENTED_EDGE('',*,*,#10918,.T.);
#15222=ORIENTED_EDGE('',*,*,#10919,.T.);
#15223=ORIENTED_EDGE('',*,*,#10920,.T.);
#15224=ORIENTED_EDGE('',*,*,#10801,.T.);
#15225=ORIENTED_EDGE('',*,*,#10921,.T.);
#15226=ORIENTED_EDGE('',*,*,#10920,.F.);
#15227=ORIENTED_EDGE('',*,*,#10922,.F.);
#15228=ORIENTED_EDGE('',*,*,#10923,.F.);
#15229=ORIENTED_EDGE('',*,*,#10802,.F.);
#15230=ORIENTED_EDGE('',*,*,#10924,.T.);
#15231=ORIENTED_EDGE('',*,*,#10925,.T.);
#15232=ORIENTED_EDGE('',*,*,#10803,.T.);
#15233=ORIENTED_EDGE('',*,*,#10923,.T.);
#15234=ORIENTED_EDGE('',*,*,#10925,.F.);
#15235=ORIENTED_EDGE('',*,*,#10926,.F.);
#15236=ORIENTED_EDGE('',*,*,#10927,.F.);
#15237=ORIENTED_EDGE('',*,*,#10804,.F.);
#15238=ORIENTED_EDGE('',*,*,#10928,.T.);
#15239=ORIENTED_EDGE('',*,*,#10929,.T.);
#15240=ORIENTED_EDGE('',*,*,#10805,.T.);
#15241=ORIENTED_EDGE('',*,*,#10927,.T.);
#15242=ORIENTED_EDGE('',*,*,#10929,.F.);
#15243=ORIENTED_EDGE('',*,*,#10930,.F.);
#15244=ORIENTED_EDGE('',*,*,#10931,.F.);
#15245=ORIENTED_EDGE('',*,*,#10806,.F.);
#15246=ORIENTED_EDGE('',*,*,#10932,.T.);
#15247=ORIENTED_EDGE('',*,*,#10933,.T.);
#15248=ORIENTED_EDGE('',*,*,#10807,.T.);
#15249=ORIENTED_EDGE('',*,*,#10931,.T.);
#15250=ORIENTED_EDGE('',*,*,#10933,.F.);
#15251=ORIENTED_EDGE('',*,*,#10934,.F.);
#15252=ORIENTED_EDGE('',*,*,#10935,.F.);
#15253=ORIENTED_EDGE('',*,*,#10808,.F.);
#15254=ORIENTED_EDGE('',*,*,#10809,.T.);
#15255=ORIENTED_EDGE('',*,*,#10935,.T.);
#15256=ORIENTED_EDGE('',*,*,#10936,.T.);
#15257=ORIENTED_EDGE('',*,*,#10937,.T.);
#15258=ORIENTED_EDGE('',*,*,#10811,.T.);
#15259=ORIENTED_EDGE('',*,*,#10938,.T.);
#15260=ORIENTED_EDGE('',*,*,#10939,.T.);
#15261=ORIENTED_EDGE('',*,*,#10940,.T.);
#15262=ORIENTED_EDGE('',*,*,#10940,.F.);
#15263=ORIENTED_EDGE('',*,*,#10941,.F.);
#15264=ORIENTED_EDGE('',*,*,#10942,.F.);
#15265=ORIENTED_EDGE('',*,*,#10812,.F.);
#15266=ORIENTED_EDGE('',*,*,#10813,.T.);
#15267=ORIENTED_EDGE('',*,*,#10942,.T.);
#15268=ORIENTED_EDGE('',*,*,#10943,.T.);
#15269=ORIENTED_EDGE('',*,*,#10944,.T.);
#15270=ORIENTED_EDGE('',*,*,#10815,.T.);
#15271=ORIENTED_EDGE('',*,*,#10945,.T.);
#15272=ORIENTED_EDGE('',*,*,#10946,.T.);
#15273=ORIENTED_EDGE('',*,*,#10744,.T.);
#15274=ORIENTED_EDGE('',*,*,#10819,.F.);
#15275=ORIENTED_EDGE('',*,*,#10947,.T.);
#15276=ORIENTED_EDGE('',*,*,#10948,.T.);
#15277=ORIENTED_EDGE('',*,*,#10947,.F.);
#15278=ORIENTED_EDGE('',*,*,#10818,.F.);
#15279=ORIENTED_EDGE('',*,*,#10949,.T.);
#15280=ORIENTED_EDGE('',*,*,#10950,.T.);
#15281=ORIENTED_EDGE('',*,*,#10949,.F.);
#15282=ORIENTED_EDGE('',*,*,#10738,.T.);
#15283=ORIENTED_EDGE('',*,*,#10951,.T.);
#15284=ORIENTED_EDGE('',*,*,#10729,.T.);
#15285=ORIENTED_EDGE('',*,*,#10951,.F.);
#15286=ORIENTED_EDGE('',*,*,#10817,.F.);
#15287=ORIENTED_EDGE('',*,*,#10952,.T.);
#15288=ORIENTED_EDGE('',*,*,#10953,.T.);
#15289=ORIENTED_EDGE('',*,*,#10952,.F.);
#15290=ORIENTED_EDGE('',*,*,#10816,.F.);
#15291=ORIENTED_EDGE('',*,*,#10954,.T.);
#15292=ORIENTED_EDGE('',*,*,#10955,.T.);
#15293=ORIENTED_EDGE('',*,*,#10954,.F.);
#15294=ORIENTED_EDGE('',*,*,#10944,.F.);
#15295=ORIENTED_EDGE('',*,*,#10956,.F.);
#15296=ORIENTED_EDGE('',*,*,#10945,.F.);
#15297=ORIENTED_EDGE('',*,*,#10814,.F.);
#15298=ORIENTED_EDGE('',*,*,#10937,.F.);
#15299=ORIENTED_EDGE('',*,*,#10957,.F.);
#15300=ORIENTED_EDGE('',*,*,#10938,.F.);
#15301=ORIENTED_EDGE('',*,*,#10810,.F.);
#15302=ORIENTED_EDGE('',*,*,#10918,.F.);
#15303=ORIENTED_EDGE('',*,*,#10958,.F.);
#15304=ORIENTED_EDGE('',*,*,#10921,.F.);
#15305=ORIENTED_EDGE('',*,*,#10800,.F.);
#15306=ORIENTED_EDGE('',*,*,#10911,.F.);
#15307=ORIENTED_EDGE('',*,*,#10959,.F.);
#15308=ORIENTED_EDGE('',*,*,#10912,.F.);
#15309=ORIENTED_EDGE('',*,*,#10796,.F.);
#15310=ORIENTED_EDGE('',*,*,#10904,.F.);
#15311=ORIENTED_EDGE('',*,*,#10960,.F.);
#15312=ORIENTED_EDGE('',*,*,#10905,.F.);
#15313=ORIENTED_EDGE('',*,*,#10792,.F.);
#15314=ORIENTED_EDGE('',*,*,#10885,.F.);
#15315=ORIENTED_EDGE('',*,*,#10961,.F.);
#15316=ORIENTED_EDGE('',*,*,#10888,.F.);
#15317=ORIENTED_EDGE('',*,*,#10782,.F.);
#15318=ORIENTED_EDGE('',*,*,#10878,.F.);
#15319=ORIENTED_EDGE('',*,*,#10962,.F.);
#15320=ORIENTED_EDGE('',*,*,#10879,.F.);
#15321=ORIENTED_EDGE('',*,*,#10778,.F.);
#15322=ORIENTED_EDGE('',*,*,#10871,.F.);
#15323=ORIENTED_EDGE('',*,*,#10963,.F.);
#15324=ORIENTED_EDGE('',*,*,#10872,.F.);
#15325=ORIENTED_EDGE('',*,*,#10774,.F.);
#15326=ORIENTED_EDGE('',*,*,#10852,.F.);
#15327=ORIENTED_EDGE('',*,*,#10964,.F.);
#15328=ORIENTED_EDGE('',*,*,#10855,.F.);
#15329=ORIENTED_EDGE('',*,*,#10764,.F.);
#15330=ORIENTED_EDGE('',*,*,#10845,.F.);
#15331=ORIENTED_EDGE('',*,*,#10965,.F.);
#15332=ORIENTED_EDGE('',*,*,#10846,.F.);
#15333=ORIENTED_EDGE('',*,*,#10760,.F.);
#15334=ORIENTED_EDGE('',*,*,#10838,.F.);
#15335=ORIENTED_EDGE('',*,*,#10966,.F.);
#15336=ORIENTED_EDGE('',*,*,#10839,.F.);
#15337=ORIENTED_EDGE('',*,*,#10756,.F.);
#15338=ORIENTED_EDGE('',*,*,#10742,.F.);
#15339=ORIENTED_EDGE('',*,*,#10967,.F.);
#15340=ORIENTED_EDGE('',*,*,#10822,.F.);
#15341=ORIENTED_EDGE('',*,*,#10746,.F.);
#15342=ORIENTED_EDGE('',*,*,#10741,.F.);
#15343=ORIENTED_EDGE('',*,*,#10745,.T.);
#15344=ORIENTED_EDGE('',*,*,#10946,.F.);
#15345=ORIENTED_EDGE('',*,*,#10956,.T.);
#15346=ORIENTED_EDGE('',*,*,#10943,.F.);
#15347=ORIENTED_EDGE('',*,*,#10941,.T.);
#15348=ORIENTED_EDGE('',*,*,#10939,.F.);
#15349=ORIENTED_EDGE('',*,*,#10957,.T.);
#15350=ORIENTED_EDGE('',*,*,#10936,.F.);
#15351=ORIENTED_EDGE('',*,*,#10934,.T.);
#15352=ORIENTED_EDGE('',*,*,#10932,.F.);
#15353=ORIENTED_EDGE('',*,*,#10930,.T.);
#15354=ORIENTED_EDGE('',*,*,#10928,.F.);
#15355=ORIENTED_EDGE('',*,*,#10926,.T.);
#15356=ORIENTED_EDGE('',*,*,#10924,.F.);
#15357=ORIENTED_EDGE('',*,*,#10922,.T.);
#15358=ORIENTED_EDGE('',*,*,#10919,.F.);
#15359=ORIENTED_EDGE('',*,*,#10958,.T.);
#15360=ORIENTED_EDGE('',*,*,#10917,.F.);
#15361=ORIENTED_EDGE('',*,*,#10915,.T.);
#15362=ORIENTED_EDGE('',*,*,#10913,.F.);
#15363=ORIENTED_EDGE('',*,*,#10959,.T.);
#15364=ORIENTED_EDGE('',*,*,#10910,.F.);
#15365=ORIENTED_EDGE('',*,*,#10908,.T.);
#15366=ORIENTED_EDGE('',*,*,#10906,.F.);
#15367=ORIENTED_EDGE('',*,*,#10960,.T.);
#15368=ORIENTED_EDGE('',*,*,#10903,.F.);
#15369=ORIENTED_EDGE('',*,*,#10901,.T.);
#15370=ORIENTED_EDGE('',*,*,#10899,.F.);
#15371=ORIENTED_EDGE('',*,*,#10897,.T.);
#15372=ORIENTED_EDGE('',*,*,#10895,.F.);
#15373=ORIENTED_EDGE('',*,*,#10893,.T.);
#15374=ORIENTED_EDGE('',*,*,#10891,.F.);
#15375=ORIENTED_EDGE('',*,*,#10889,.T.);
#15376=ORIENTED_EDGE('',*,*,#10886,.F.);
#15377=ORIENTED_EDGE('',*,*,#10961,.T.);
#15378=ORIENTED_EDGE('',*,*,#10884,.F.);
#15379=ORIENTED_EDGE('',*,*,#10882,.T.);
#15380=ORIENTED_EDGE('',*,*,#10880,.F.);
#15381=ORIENTED_EDGE('',*,*,#10962,.T.);
#15382=ORIENTED_EDGE('',*,*,#10877,.F.);
#15383=ORIENTED_EDGE('',*,*,#10875,.T.);
#15384=ORIENTED_EDGE('',*,*,#10873,.F.);
#15385=ORIENTED_EDGE('',*,*,#10963,.T.);
#15386=ORIENTED_EDGE('',*,*,#10870,.F.);
#15387=ORIENTED_EDGE('',*,*,#10868,.T.);
#15388=ORIENTED_EDGE('',*,*,#10866,.F.);
#15389=ORIENTED_EDGE('',*,*,#10864,.T.);
#15390=ORIENTED_EDGE('',*,*,#10862,.F.);
#15391=ORIENTED_EDGE('',*,*,#10860,.T.);
#15392=ORIENTED_EDGE('',*,*,#10858,.F.);
#15393=ORIENTED_EDGE('',*,*,#10856,.T.);
#15394=ORIENTED_EDGE('',*,*,#10853,.F.);
#15395=ORIENTED_EDGE('',*,*,#10964,.T.);
#15396=ORIENTED_EDGE('',*,*,#10851,.F.);
#15397=ORIENTED_EDGE('',*,*,#10849,.T.);
#15398=ORIENTED_EDGE('',*,*,#10847,.F.);
#15399=ORIENTED_EDGE('',*,*,#10965,.T.);
#15400=ORIENTED_EDGE('',*,*,#10844,.F.);
#15401=ORIENTED_EDGE('',*,*,#10842,.T.);
#15402=ORIENTED_EDGE('',*,*,#10840,.F.);
#15403=ORIENTED_EDGE('',*,*,#10966,.T.);
#15404=ORIENTED_EDGE('',*,*,#10837,.F.);
#15405=ORIENTED_EDGE('',*,*,#10835,.T.);
#15406=ORIENTED_EDGE('',*,*,#10833,.F.);
#15407=ORIENTED_EDGE('',*,*,#10831,.T.);
#15408=ORIENTED_EDGE('',*,*,#10829,.F.);
#15409=ORIENTED_EDGE('',*,*,#10827,.T.);
#15410=ORIENTED_EDGE('',*,*,#10825,.F.);
#15411=ORIENTED_EDGE('',*,*,#10823,.T.);
#15412=ORIENTED_EDGE('',*,*,#10820,.F.);
#15413=ORIENTED_EDGE('',*,*,#10967,.T.);
#15414=ORIENTED_EDGE('',*,*,#10728,.T.);
#15415=ORIENTED_EDGE('',*,*,#10597,.T.);
#15416=ORIENTED_EDGE('',*,*,#10725,.T.);
#15417=ORIENTED_EDGE('',*,*,#10719,.T.);
#15418=ORIENTED_EDGE('',*,*,#10955,.F.);
#15419=ORIENTED_EDGE('',*,*,#10953,.F.);
#15420=ORIENTED_EDGE('',*,*,#10950,.F.);
#15421=ORIENTED_EDGE('',*,*,#10948,.F.);
#19841=CYLINDRICAL_SURFACE('',#22298,4.51775);
#19842=CYLINDRICAL_SURFACE('',#22302,4.51775);
#19843=CYLINDRICAL_SURFACE('',#22303,4.51775);
#19844=CYLINDRICAL_SURFACE('',#22304,4.51775);
#19845=CYLINDRICAL_SURFACE('',#22305,4.51775);
#19846=CYLINDRICAL_SURFACE('',#22306,4.51775);
#19847=CYLINDRICAL_SURFACE('',#22307,4.51775);
#19848=CYLINDRICAL_SURFACE('',#22308,4.51775);
#19849=CYLINDRICAL_SURFACE('',#22309,4.51775);
#19850=CYLINDRICAL_SURFACE('',#22310,4.51775);
#19851=CYLINDRICAL_SURFACE('',#22311,4.51775);
#19852=CYLINDRICAL_SURFACE('',#22312,4.51775);
#19853=CYLINDRICAL_SURFACE('',#22313,4.51775);
#19854=CYLINDRICAL_SURFACE('',#22314,4.51775);
#19855=CYLINDRICAL_SURFACE('',#22315,4.51775);
#19856=CYLINDRICAL_SURFACE('',#22316,4.51775);
#19857=CYLINDRICAL_SURFACE('',#22317,4.51775);
#19858=CYLINDRICAL_SURFACE('',#22318,4.51775);
#19859=CYLINDRICAL_SURFACE('',#22319,4.51775);
#19860=CYLINDRICAL_SURFACE('',#22320,4.51775);
#19861=CYLINDRICAL_SURFACE('',#22321,4.51775);
#19862=CYLINDRICAL_SURFACE('',#22322,4.51775);
#19863=CYLINDRICAL_SURFACE('',#22323,4.51775);
#19864=CYLINDRICAL_SURFACE('',#22324,4.51775);
#19865=CYLINDRICAL_SURFACE('',#22325,4.51775);
#19866=CYLINDRICAL_SURFACE('',#22327,5.0736);
#19867=CYLINDRICAL_SURFACE('',#22329,5.0736);
#19868=CYLINDRICAL_SURFACE('',#22330,5.0736);
#19869=CYLINDRICAL_SURFACE('',#22331,5.0736);
#19870=CYLINDRICAL_SURFACE('',#22332,5.0736);
#19871=CYLINDRICAL_SURFACE('',#22333,5.0736);
#19872=CYLINDRICAL_SURFACE('',#22334,5.0736);
#19873=CYLINDRICAL_SURFACE('',#22335,5.0736);
#19874=CYLINDRICAL_SURFACE('',#22336,5.0736);
#19875=CYLINDRICAL_SURFACE('',#22337,5.0736);
#19876=CYLINDRICAL_SURFACE('',#22338,5.0736);
#19877=CYLINDRICAL_SURFACE('',#22339,5.0736);
#19878=CYLINDRICAL_SURFACE('',#22340,5.0736);
#19879=CYLINDRICAL_SURFACE('',#22341,5.0736);
#19880=CYLINDRICAL_SURFACE('',#22342,5.0736);
#19881=CYLINDRICAL_SURFACE('',#22343,5.0736);
#19882=CYLINDRICAL_SURFACE('',#22344,5.0736);
#19883=CYLINDRICAL_SURFACE('',#22345,5.0736);
#19884=CYLINDRICAL_SURFACE('',#22346,5.0736);
#19885=CYLINDRICAL_SURFACE('',#22347,5.0736);
#19886=CYLINDRICAL_SURFACE('',#22348,5.0736);
#19887=CYLINDRICAL_SURFACE('',#22349,5.0736);
#19888=CYLINDRICAL_SURFACE('',#22350,5.0736);
#19889=CYLINDRICAL_SURFACE('',#22351,5.0736);
#19890=CYLINDRICAL_SURFACE('',#22352,5.0736);
#19891=CYLINDRICAL_SURFACE('',#22354,4.51775);
#19892=CYLINDRICAL_SURFACE('',#22358,4.51775);
#19893=CYLINDRICAL_SURFACE('',#22359,4.51775);
#19894=CYLINDRICAL_SURFACE('',#22360,4.51775);
#19895=CYLINDRICAL_SURFACE('',#22361,4.51775);
#19896=CYLINDRICAL_SURFACE('',#22362,4.51775);
#19897=CYLINDRICAL_SURFACE('',#22363,4.51775);
#19898=CYLINDRICAL_SURFACE('',#22364,4.51775);
#19899=CYLINDRICAL_SURFACE('',#22365,4.51775);
#19900=CYLINDRICAL_SURFACE('',#22366,4.51775);
#19901=CYLINDRICAL_SURFACE('',#22367,4.51775);
#19902=CYLINDRICAL_SURFACE('',#22368,4.51775);
#19903=CYLINDRICAL_SURFACE('',#22369,4.51775);
#19904=CYLINDRICAL_SURFACE('',#22370,4.51775);
#19905=CYLINDRICAL_SURFACE('',#22371,4.51775);
#19906=CYLINDRICAL_SURFACE('',#22372,4.51775);
#19907=CYLINDRICAL_SURFACE('',#22373,4.51775);
#19908=CYLINDRICAL_SURFACE('',#22374,4.51775);
#19909=CYLINDRICAL_SURFACE('',#22375,4.51775);
#19910=CYLINDRICAL_SURFACE('',#22376,4.51775);
#19911=CYLINDRICAL_SURFACE('',#22377,4.51775);
#19912=CYLINDRICAL_SURFACE('',#22378,4.51775);
#19913=CYLINDRICAL_SURFACE('',#22379,4.51775);
#19914=CYLINDRICAL_SURFACE('',#22380,4.51775);
#19915=CYLINDRICAL_SURFACE('',#22381,4.51775);
#19916=CYLINDRICAL_SURFACE('',#22382,4.51775);
#19917=CYLINDRICAL_SURFACE('',#22383,4.51775);
#19918=CYLINDRICAL_SURFACE('',#22384,4.51775);
#19919=CYLINDRICAL_SURFACE('',#22385,4.51775);
#19920=CYLINDRICAL_SURFACE('',#22386,4.51775);
#19921=CYLINDRICAL_SURFACE('',#22387,4.51775);
#19922=CYLINDRICAL_SURFACE('',#22388,4.51775);
#19923=CYLINDRICAL_SURFACE('',#22389,4.51775);
#19924=CYLINDRICAL_SURFACE('',#22390,4.51775);
#19925=CYLINDRICAL_SURFACE('',#22391,4.51775);
#19926=CYLINDRICAL_SURFACE('',#22392,4.51775);
#19927=CYLINDRICAL_SURFACE('',#22393,4.51775);
#19928=CYLINDRICAL_SURFACE('',#22394,4.51775);
#19929=CYLINDRICAL_SURFACE('',#22395,4.51775);
#19930=CYLINDRICAL_SURFACE('',#22396,4.51775);
#19931=CYLINDRICAL_SURFACE('',#22398,5.0736);
#19932=CYLINDRICAL_SURFACE('',#22400,5.0736);
#19933=CYLINDRICAL_SURFACE('',#22401,5.0736);
#19934=CYLINDRICAL_SURFACE('',#22402,5.0736);
#19935=CYLINDRICAL_SURFACE('',#22403,5.0736);
#19936=CYLINDRICAL_SURFACE('',#22404,5.0736);
#19937=CYLINDRICAL_SURFACE('',#22405,5.0736);
#19938=CYLINDRICAL_SURFACE('',#22406,5.0736);
#19939=CYLINDRICAL_SURFACE('',#22407,5.0736);
#19940=CYLINDRICAL_SURFACE('',#22408,5.0736);
#19941=CYLINDRICAL_SURFACE('',#22409,5.0736);
#19942=CYLINDRICAL_SURFACE('',#22410,5.0736);
#19943=CYLINDRICAL_SURFACE('',#22411,5.0736);
#19944=CYLINDRICAL_SURFACE('',#22412,5.0736);
#19945=CYLINDRICAL_SURFACE('',#22413,5.0736);
#19946=CYLINDRICAL_SURFACE('',#22414,5.0736);
#19947=CYLINDRICAL_SURFACE('',#22415,5.0736);
#19948=CYLINDRICAL_SURFACE('',#22416,5.0736);
#19949=CYLINDRICAL_SURFACE('',#22417,5.0736);
#19950=CYLINDRICAL_SURFACE('',#22418,5.0736);
#19951=CYLINDRICAL_SURFACE('',#22419,5.0736);
#19952=CYLINDRICAL_SURFACE('',#22420,5.0736);
#19953=CYLINDRICAL_SURFACE('',#22421,5.0736);
#19954=CYLINDRICAL_SURFACE('',#22422,5.0736);
#19955=CYLINDRICAL_SURFACE('',#22423,5.0736);
#19956=CYLINDRICAL_SURFACE('',#22424,5.0736);
#19957=CYLINDRICAL_SURFACE('',#22425,5.0736);
#19958=CYLINDRICAL_SURFACE('',#22426,5.0736);
#19959=CYLINDRICAL_SURFACE('',#22427,5.0736);
#19960=CYLINDRICAL_SURFACE('',#22428,5.0736);
#19961=CYLINDRICAL_SURFACE('',#22429,5.0736);
#19962=CYLINDRICAL_SURFACE('',#22430,5.0736);
#19963=CYLINDRICAL_SURFACE('',#22431,5.0736);
#19964=CYLINDRICAL_SURFACE('',#22432,5.0736);
#19965=CYLINDRICAL_SURFACE('',#22433,5.0736);
#19966=CYLINDRICAL_SURFACE('',#22434,5.0736);
#19967=CYLINDRICAL_SURFACE('',#22435,5.0736);
#19968=CYLINDRICAL_SURFACE('',#22436,5.0736);
#19969=CYLINDRICAL_SURFACE('',#22437,5.0736);
#19970=CYLINDRICAL_SURFACE('',#22438,5.0736);
#19971=CYLINDRICAL_SURFACE('',#22441,5.0736);
#19972=CYLINDRICAL_SURFACE('',#22442,4.51775);
#19973=CYLINDRICAL_SURFACE('',#22446,5.0736);
#19974=CYLINDRICAL_SURFACE('',#22447,4.51775);
#19975=CYLINDRICAL_SURFACE('',#22450,1.);
#19976=CYLINDRICAL_SURFACE('',#22494,1.);
#19977=CYLINDRICAL_SURFACE('',#22497,1.);
#19978=CYLINDRICAL_SURFACE('',#22500,1.);
#19979=CYLINDRICAL_SURFACE('',#22503,1.);
#19980=CYLINDRICAL_SURFACE('',#22506,1.);
#19981=CYLINDRICAL_SURFACE('',#22508,1.);
#19982=CYLINDRICAL_SURFACE('',#22511,1.);
#19983=CYLINDRICAL_SURFACE('',#22513,1.);
#19984=CYLINDRICAL_SURFACE('',#22516,1.);
#19985=CYLINDRICAL_SURFACE('',#22518,1.);
#19986=CYLINDRICAL_SURFACE('',#22521,1.);
#19987=CYLINDRICAL_SURFACE('',#22524,1.);
#19988=CYLINDRICAL_SURFACE('',#22527,1.);
#19989=CYLINDRICAL_SURFACE('',#22530,1.);
#19990=CYLINDRICAL_SURFACE('',#22532,1.);
#19991=CYLINDRICAL_SURFACE('',#22535,1.);
#19992=CYLINDRICAL_SURFACE('',#22537,1.);
#19993=CYLINDRICAL_SURFACE('',#22540,1.);
#19994=CYLINDRICAL_SURFACE('',#22542,1.);
#19995=CYLINDRICAL_SURFACE('',#22545,1.);
#19996=CYLINDRICAL_SURFACE('',#22548,1.);
#19997=CYLINDRICAL_SURFACE('',#22551,1.);
#19998=CYLINDRICAL_SURFACE('',#22554,1.);
#19999=CYLINDRICAL_SURFACE('',#22556,1.);
#20000=CYLINDRICAL_SURFACE('',#22559,1.);
#20001=CYLINDRICAL_SURFACE('',#22561,1.);
#20002=CYLINDRICAL_SURFACE('',#22564,1.);
#20003=CYLINDRICAL_SURFACE('',#22566,1.);
#20004=CYLINDRICAL_SURFACE('',#22569,1.);
#20005=CYLINDRICAL_SURFACE('',#22572,1.);
#20006=CYLINDRICAL_SURFACE('',#22575,1.);
#20007=CYLINDRICAL_SURFACE('',#22578,1.);
#20008=CYLINDRICAL_SURFACE('',#22580,1.);
#20009=CYLINDRICAL_SURFACE('',#22583,1.);
#20010=CYLINDRICAL_SURFACE('',#22585,1.);
#20011=CYLINDRICAL_SURFACE('',#22587,3.);
#20012=CYLINDRICAL_SURFACE('',#22589,3.);
#20013=CYLINDRICAL_SURFACE('',#22591,4.);
#20014=CYLINDRICAL_SURFACE('',#22592,3.);
#20015=CYLINDRICAL_SURFACE('',#22594,3.);
#20837=ADVANCED_FACE('',(#2717),#19841,.F.);
#20838=ADVANCED_FACE('',(#2718),#19842,.F.);
#20839=ADVANCED_FACE('',(#2719),#19843,.F.);
#20840=ADVANCED_FACE('',(#2720),#19844,.F.);
#20841=ADVANCED_FACE('',(#2721),#19845,.F.);
#20842=ADVANCED_FACE('',(#2722),#19846,.F.);
#20843=ADVANCED_FACE('',(#2723),#19847,.F.);
#20844=ADVANCED_FACE('',(#2724),#19848,.F.);
#20845=ADVANCED_FACE('',(#2725),#19849,.F.);
#20846=ADVANCED_FACE('',(#2726),#19850,.F.);
#20847=ADVANCED_FACE('',(#2727),#19851,.F.);
#20848=ADVANCED_FACE('',(#2728),#19852,.F.);
#20849=ADVANCED_FACE('',(#2729),#19853,.F.);
#20850=ADVANCED_FACE('',(#2730),#19854,.F.);
#20851=ADVANCED_FACE('',(#2731),#19855,.F.);
#20852=ADVANCED_FACE('',(#2732),#19856,.F.);
#20853=ADVANCED_FACE('',(#2733),#19857,.F.);
#20854=ADVANCED_FACE('',(#2734),#19858,.F.);
#20855=ADVANCED_FACE('',(#2735),#19859,.F.);
#20856=ADVANCED_FACE('',(#2736),#19860,.F.);
#20857=ADVANCED_FACE('',(#2737),#19861,.F.);
#20858=ADVANCED_FACE('',(#2738),#19862,.F.);
#20859=ADVANCED_FACE('',(#2739),#19863,.F.);
#20860=ADVANCED_FACE('',(#2740),#19864,.F.);
#20861=ADVANCED_FACE('',(#2741),#19865,.F.);
#20862=ADVANCED_FACE('',(#2742),#19866,.F.);
#20863=ADVANCED_FACE('',(#2743),#19867,.F.);
#20864=ADVANCED_FACE('',(#2744),#19868,.F.);
#20865=ADVANCED_FACE('',(#2745),#19869,.F.);
#20866=ADVANCED_FACE('',(#2746),#19870,.F.);
#20867=ADVANCED_FACE('',(#2747),#19871,.F.);
#20868=ADVANCED_FACE('',(#2748),#19872,.F.);
#20869=ADVANCED_FACE('',(#2749),#19873,.F.);
#20870=ADVANCED_FACE('',(#2750),#19874,.F.);
#20871=ADVANCED_FACE('',(#2751),#19875,.F.);
#20872=ADVANCED_FACE('',(#2752),#19876,.F.);
#20873=ADVANCED_FACE('',(#2753),#19877,.F.);
#20874=ADVANCED_FACE('',(#2754),#19878,.F.);
#20875=ADVANCED_FACE('',(#2755),#19879,.F.);
#20876=ADVANCED_FACE('',(#2756),#19880,.F.);
#20877=ADVANCED_FACE('',(#2757),#19881,.F.);
#20878=ADVANCED_FACE('',(#2758),#19882,.F.);
#20879=ADVANCED_FACE('',(#2759),#19883,.F.);
#20880=ADVANCED_FACE('',(#2760),#19884,.F.);
#20881=ADVANCED_FACE('',(#2761),#19885,.F.);
#20882=ADVANCED_FACE('',(#2762),#19886,.F.);
#20883=ADVANCED_FACE('',(#2763),#19887,.F.);
#20884=ADVANCED_FACE('',(#2764),#19888,.F.);
#20885=ADVANCED_FACE('',(#2765),#19889,.F.);
#20886=ADVANCED_FACE('',(#2766),#19890,.F.);
#20887=ADVANCED_FACE('',(#2767),#19891,.F.);
#20888=ADVANCED_FACE('',(#2768),#19892,.F.);
#20889=ADVANCED_FACE('',(#2769),#19893,.F.);
#20890=ADVANCED_FACE('',(#2770),#19894,.F.);
#20891=ADVANCED_FACE('',(#2771),#19895,.F.);
#20892=ADVANCED_FACE('',(#2772),#19896,.F.);
#20893=ADVANCED_FACE('',(#2773),#19897,.F.);
#20894=ADVANCED_FACE('',(#2774),#19898,.F.);
#20895=ADVANCED_FACE('',(#2775),#19899,.F.);
#20896=ADVANCED_FACE('',(#2776),#19900,.F.);
#20897=ADVANCED_FACE('',(#2777),#19901,.F.);
#20898=ADVANCED_FACE('',(#2778),#19902,.F.);
#20899=ADVANCED_FACE('',(#2779),#19903,.F.);
#20900=ADVANCED_FACE('',(#2780),#19904,.F.);
#20901=ADVANCED_FACE('',(#2781),#19905,.F.);
#20902=ADVANCED_FACE('',(#2782),#19906,.F.);
#20903=ADVANCED_FACE('',(#2783),#19907,.F.);
#20904=ADVANCED_FACE('',(#2784),#19908,.F.);
#20905=ADVANCED_FACE('',(#2785),#19909,.F.);
#20906=ADVANCED_FACE('',(#2786),#19910,.F.);
#20907=ADVANCED_FACE('',(#2787),#19911,.F.);
#20908=ADVANCED_FACE('',(#2788),#19912,.F.);
#20909=ADVANCED_FACE('',(#2789),#19913,.F.);
#20910=ADVANCED_FACE('',(#2790),#19914,.F.);
#20911=ADVANCED_FACE('',(#2791),#19915,.F.);
#20912=ADVANCED_FACE('',(#2792),#19916,.F.);
#20913=ADVANCED_FACE('',(#2793),#19917,.F.);
#20914=ADVANCED_FACE('',(#2794),#19918,.F.);
#20915=ADVANCED_FACE('',(#2795),#19919,.F.);
#20916=ADVANCED_FACE('',(#2796),#19920,.F.);
#20917=ADVANCED_FACE('',(#2797),#19921,.F.);
#20918=ADVANCED_FACE('',(#2798),#19922,.F.);
#20919=ADVANCED_FACE('',(#2799),#19923,.F.);
#20920=ADVANCED_FACE('',(#2800),#19924,.F.);
#20921=ADVANCED_FACE('',(#2801),#19925,.F.);
#20922=ADVANCED_FACE('',(#2802),#19926,.F.);
#20923=ADVANCED_FACE('',(#2803),#19927,.F.);
#20924=ADVANCED_FACE('',(#2804),#19928,.F.);
#20925=ADVANCED_FACE('',(#2805),#19929,.F.);
#20926=ADVANCED_FACE('',(#2806),#19930,.F.);
#20927=ADVANCED_FACE('',(#2807),#19931,.F.);
#20928=ADVANCED_FACE('',(#2808),#19932,.F.);
#20929=ADVANCED_FACE('',(#2809),#19933,.F.);
#20930=ADVANCED_FACE('',(#2810),#19934,.F.);
#20931=ADVANCED_FACE('',(#2811),#19935,.F.);
#20932=ADVANCED_FACE('',(#2812),#19936,.F.);
#20933=ADVANCED_FACE('',(#2813),#19937,.F.);
#20934=ADVANCED_FACE('',(#2814),#19938,.F.);
#20935=ADVANCED_FACE('',(#2815),#19939,.F.);
#20936=ADVANCED_FACE('',(#2816),#19940,.F.);
#20937=ADVANCED_FACE('',(#2817),#19941,.F.);
#20938=ADVANCED_FACE('',(#2818),#19942,.F.);
#20939=ADVANCED_FACE('',(#2819),#19943,.F.);
#20940=ADVANCED_FACE('',(#2820),#19944,.F.);
#20941=ADVANCED_FACE('',(#2821),#19945,.F.);
#20942=ADVANCED_FACE('',(#2822),#19946,.F.);
#20943=ADVANCED_FACE('',(#2823),#19947,.F.);
#20944=ADVANCED_FACE('',(#2824),#19948,.F.);
#20945=ADVANCED_FACE('',(#2825),#19949,.F.);
#20946=ADVANCED_FACE('',(#2826),#19950,.F.);
#20947=ADVANCED_FACE('',(#2827),#19951,.F.);
#20948=ADVANCED_FACE('',(#2828),#19952,.F.);
#20949=ADVANCED_FACE('',(#2829),#19953,.F.);
#20950=ADVANCED_FACE('',(#2830),#19954,.F.);
#20951=ADVANCED_FACE('',(#2831),#19955,.F.);
#20952=ADVANCED_FACE('',(#2832),#19956,.F.);
#20953=ADVANCED_FACE('',(#2833),#19957,.F.);
#20954=ADVANCED_FACE('',(#2834),#19958,.F.);
#20955=ADVANCED_FACE('',(#2835),#19959,.F.);
#20956=ADVANCED_FACE('',(#2836),#19960,.F.);
#20957=ADVANCED_FACE('',(#2837),#19961,.F.);
#20958=ADVANCED_FACE('',(#2838),#19962,.F.);
#20959=ADVANCED_FACE('',(#2839),#19963,.F.);
#20960=ADVANCED_FACE('',(#2840),#19964,.F.);
#20961=ADVANCED_FACE('',(#2841),#19965,.F.);
#20962=ADVANCED_FACE('',(#2842),#19966,.F.);
#20963=ADVANCED_FACE('',(#2843),#19967,.F.);
#20964=ADVANCED_FACE('',(#2844),#19968,.F.);
#20965=ADVANCED_FACE('',(#2845),#19969,.F.);
#20966=ADVANCED_FACE('',(#2846),#19970,.F.);
#20967=ADVANCED_FACE('',(#2847),#2417,.F.);
#20968=ADVANCED_FACE('',(#2848),#19971,.F.);
#20969=ADVANCED_FACE('',(#2849),#344,.F.);
#20970=ADVANCED_FACE('',(#2850),#345,.F.);
#20971=ADVANCED_FACE('',(#2851),#19972,.F.);
#20972=ADVANCED_FACE('',(#2852,#2316),#2418,.F.);
#20973=ADVANCED_FACE('',(#2853),#2419,.T.);
#20974=ADVANCED_FACE('',(#2854),#19973,.F.);
#20975=ADVANCED_FACE('',(#2855),#346,.F.);
#20976=ADVANCED_FACE('',(#2856),#347,.F.);
#20977=ADVANCED_FACE('',(#2857),#19974,.F.);
#20978=ADVANCED_FACE('',(#2858,#2317),#2420,.F.);
#20979=ADVANCED_FACE('',(#2859),#19975,.T.);
#20980=ADVANCED_FACE('',(#2860),#2421,.T.);
#20981=ADVANCED_FACE('',(#2861,#2318,#2319,#2320,#2321,#2322),#2422,.T.);
#20982=ADVANCED_FACE('',(#2862),#19976,.F.);
#20983=ADVANCED_FACE('',(#2863),#2423,.T.);
#20984=ADVANCED_FACE('',(#2864),#19977,.F.);
#20985=ADVANCED_FACE('',(#2865),#2424,.T.);
#20986=ADVANCED_FACE('',(#2866),#19978,.F.);
#20987=ADVANCED_FACE('',(#2867),#2425,.T.);
#20988=ADVANCED_FACE('',(#2868),#19979,.F.);
#20989=ADVANCED_FACE('',(#2869),#2426,.T.);
#20990=ADVANCED_FACE('',(#2870),#19980,.T.);
#20991=ADVANCED_FACE('',(#2871),#19981,.T.);
#20992=ADVANCED_FACE('',(#2872),#2427,.T.);
#20993=ADVANCED_FACE('',(#2873),#19982,.T.);
#20994=ADVANCED_FACE('',(#2874),#19983,.T.);
#20995=ADVANCED_FACE('',(#2875),#2428,.T.);
#20996=ADVANCED_FACE('',(#2876),#19984,.T.);
#20997=ADVANCED_FACE('',(#2877),#19985,.F.);
#20998=ADVANCED_FACE('',(#2878),#2429,.T.);
#20999=ADVANCED_FACE('',(#2879),#19986,.F.);
#21000=ADVANCED_FACE('',(#2880),#2430,.T.);
#21001=ADVANCED_FACE('',(#2881),#19987,.F.);
#21002=ADVANCED_FACE('',(#2882),#2431,.T.);
#21003=ADVANCED_FACE('',(#2883),#19988,.F.);
#21004=ADVANCED_FACE('',(#2884),#2432,.T.);
#21005=ADVANCED_FACE('',(#2885),#19989,.T.);
#21006=ADVANCED_FACE('',(#2886),#19990,.T.);
#21007=ADVANCED_FACE('',(#2887),#2433,.T.);
#21008=ADVANCED_FACE('',(#2888),#19991,.T.);
#21009=ADVANCED_FACE('',(#2889),#19992,.T.);
#21010=ADVANCED_FACE('',(#2890),#2434,.T.);
#21011=ADVANCED_FACE('',(#2891),#19993,.T.);
#21012=ADVANCED_FACE('',(#2892),#19994,.F.);
#21013=ADVANCED_FACE('',(#2893),#2435,.T.);
#21014=ADVANCED_FACE('',(#2894),#19995,.F.);
#21015=ADVANCED_FACE('',(#2895),#2436,.T.);
#21016=ADVANCED_FACE('',(#2896),#19996,.F.);
#21017=ADVANCED_FACE('',(#2897),#2437,.T.);
#21018=ADVANCED_FACE('',(#2898),#19997,.F.);
#21019=ADVANCED_FACE('',(#2899),#2438,.T.);
#21020=ADVANCED_FACE('',(#2900),#19998,.T.);
#21021=ADVANCED_FACE('',(#2901),#19999,.T.);
#21022=ADVANCED_FACE('',(#2902),#2439,.T.);
#21023=ADVANCED_FACE('',(#2903),#20000,.T.);
#21024=ADVANCED_FACE('',(#2904),#20001,.T.);
#21025=ADVANCED_FACE('',(#2905),#2440,.T.);
#21026=ADVANCED_FACE('',(#2906),#20002,.T.);
#21027=ADVANCED_FACE('',(#2907),#20003,.F.);
#21028=ADVANCED_FACE('',(#2908),#2441,.T.);
#21029=ADVANCED_FACE('',(#2909),#20004,.F.);
#21030=ADVANCED_FACE('',(#2910),#2442,.T.);
#21031=ADVANCED_FACE('',(#2911),#20005,.F.);
#21032=ADVANCED_FACE('',(#2912),#2443,.T.);
#21033=ADVANCED_FACE('',(#2913),#20006,.F.);
#21034=ADVANCED_FACE('',(#2914),#2444,.T.);
#21035=ADVANCED_FACE('',(#2915),#20007,.T.);
#21036=ADVANCED_FACE('',(#2916),#20008,.T.);
#21037=ADVANCED_FACE('',(#2917),#2445,.T.);
#21038=ADVANCED_FACE('',(#2918),#20009,.T.);
#21039=ADVANCED_FACE('',(#2919),#20010,.T.);
#21040=ADVANCED_FACE('',(#2920),#20011,.F.);
#21041=ADVANCED_FACE('',(#2921),#20012,.F.);
#21042=ADVANCED_FACE('',(#2922),#20013,.F.);
#21043=ADVANCED_FACE('',(#2923),#20014,.F.);
#21044=ADVANCED_FACE('',(#2924),#20015,.F.);
#21045=ADVANCED_FACE('',(#2925),#2446,.T.);
#21046=ADVANCED_FACE('',(#2926),#2447,.T.);
#21047=ADVANCED_FACE('',(#2927),#2448,.T.);
#21048=ADVANCED_FACE('',(#2928),#2449,.T.);
#21049=ADVANCED_FACE('',(#2929),#2450,.T.);
#21050=ADVANCED_FACE('',(#2930),#2451,.T.);
#21051=ADVANCED_FACE('',(#2931),#2452,.T.);
#21052=ADVANCED_FACE('',(#2932),#2453,.T.);
#21053=ADVANCED_FACE('',(#2933),#2454,.T.);
#21054=ADVANCED_FACE('',(#2934),#2455,.T.);
#21055=ADVANCED_FACE('',(#2935),#2456,.T.);
#21056=ADVANCED_FACE('',(#2936),#2457,.T.);
#21057=ADVANCED_FACE('',(#2937,#2323,#2324,#2325,#2326,#2327),#2458,.F.);
#21816=CLOSED_SHELL('',(#20837,#20838,#20839,#20840,#20841,#20842,#20843,
#20844,#20845,#20846,#20847,#20848,#20849,#20850,#20851,#20852,#20853,#20854,
#20855,#20856,#20857,#20858,#20859,#20860,#20861,#20862,#20863,#20864,#20865,
#20866,#20867,#20868,#20869,#20870,#20871,#20872,#20873,#20874,#20875,#20876,
#20877,#20878,#20879,#20880,#20881,#20882,#20883,#20884,#20885,#20886,#20887,
#20888,#20889,#20890,#20891,#20892,#20893,#20894,#20895,#20896,#20897,#20898,
#20899,#20900,#20901,#20902,#20903,#20904,#20905,#20906,#20907,#20908,#20909,
#20910,#20911,#20912,#20913,#20914,#20915,#20916,#20917,#20918,#20919,#20920,
#20921,#20922,#20923,#20924,#20925,#20926,#20927,#20928,#20929,#20930,#20931,
#20932,#20933,#20934,#20935,#20936,#20937,#20938,#20939,#20940,#20941,#20942,
#20943,#20944,#20945,#20946,#20947,#20948,#20949,#20950,#20951,#20952,#20953,
#20954,#20955,#20956,#20957,#20958,#20959,#20960,#20961,#20962,#20963,#20964,
#20965,#20966,#20967,#20968,#20969,#20970,#20971,#20972,#20973,#20974,#20975,
#20976,#20977,#20978,#20979,#20980,#20981,#20982,#20983,#20984,#20985,#20986,
#20987,#20988,#20989,#20990,#20991,#20992,#20993,#20994,#20995,#20996,#20997,
#20998,#20999,#21000,#21001,#21002,#21003,#21004,#21005,#21006,#21007,#21008,
#21009,#21010,#21011,#21012,#21013,#21014,#21015,#21016,#21017,#21018,#21019,
#21020,#21021,#21022,#21023,#21024,#21025,#21026,#21027,#21028,#21029,#21030,
#21031,#21032,#21033,#21034,#21035,#21036,#21037,#21038,#21039,#21040,#21041,
#21042,#21043,#21044,#21045,#21046,#21047,#21048,#21049,#21050,#21051,#21052,
#21053,#21054,#21055,#21056,#21057));
#22297=AXIS2_PLACEMENT_3D('',#37339,#24216,#24217);
#22298=AXIS2_PLACEMENT_3D('',#37340,#24218,#24219);
#22299=AXIS2_PLACEMENT_3D('',#37353,#24221,#24222);
#22300=AXIS2_PLACEMENT_3D('',#37356,#24224,#24225);
#22301=AXIS2_PLACEMENT_3D('',#37358,#24226,#24227);
#22302=AXIS2_PLACEMENT_3D('',#37375,#24228,#24229);
#22303=AXIS2_PLACEMENT_3D('',#37465,#24231,#24232);
#22304=AXIS2_PLACEMENT_3D('',#37552,#24234,#24235);
#22305=AXIS2_PLACEMENT_3D('',#37639,#24237,#24238);
#22306=AXIS2_PLACEMENT_3D('',#37726,#24240,#24241);
#22307=AXIS2_PLACEMENT_3D('',#37816,#24243,#24244);
#22308=AXIS2_PLACEMENT_3D('',#37903,#24246,#24247);
#22309=AXIS2_PLACEMENT_3D('',#37990,#24249,#24250);
#22310=AXIS2_PLACEMENT_3D('',#38080,#24252,#24253);
#22311=AXIS2_PLACEMENT_3D('',#38167,#24255,#24256);
#22312=AXIS2_PLACEMENT_3D('',#38254,#24258,#24259);
#22313=AXIS2_PLACEMENT_3D('',#38341,#24261,#24262);
#22314=AXIS2_PLACEMENT_3D('',#38431,#24264,#24265);
#22315=AXIS2_PLACEMENT_3D('',#38518,#24267,#24268);
#22316=AXIS2_PLACEMENT_3D('',#38605,#24270,#24271);
#22317=AXIS2_PLACEMENT_3D('',#38692,#24273,#24274);
#22318=AXIS2_PLACEMENT_3D('',#38782,#24276,#24277);
#22319=AXIS2_PLACEMENT_3D('',#38869,#24279,#24280);
#22320=AXIS2_PLACEMENT_3D('',#38956,#24282,#24283);
#22321=AXIS2_PLACEMENT_3D('',#39046,#24285,#24286);
#22322=AXIS2_PLACEMENT_3D('',#39133,#24288,#24289);
#22323=AXIS2_PLACEMENT_3D('',#39220,#24291,#24292);
#22324=AXIS2_PLACEMENT_3D('',#39307,#24294,#24295);
#22325=AXIS2_PLACEMENT_3D('',#39397,#24297,#24298);
#22326=AXIS2_PLACEMENT_3D('',#39428,#24300,#24301);
#22327=AXIS2_PLACEMENT_3D('',#39466,#24302,#24303);
#22328=AXIS2_PLACEMENT_3D('',#39484,#24305,#24306);
#22329=AXIS2_PLACEMENT_3D('',#39499,#24307,#24308);
#22330=AXIS2_PLACEMENT_3D('',#39536,#24310,#24311);
#22331=AXIS2_PLACEMENT_3D('',#39574,#24313,#24314);
#22332=AXIS2_PLACEMENT_3D('',#39610,#24316,#24317);
#22333=AXIS2_PLACEMENT_3D('',#39648,#24319,#24320);
#22334=AXIS2_PLACEMENT_3D('',#39686,#24322,#24323);
#22335=AXIS2_PLACEMENT_3D('',#39722,#24325,#24326);
#22336=AXIS2_PLACEMENT_3D('',#39760,#24328,#24329);
#22337=AXIS2_PLACEMENT_3D('',#39798,#24331,#24332);
#22338=AXIS2_PLACEMENT_3D('',#39834,#24334,#24335);
#22339=AXIS2_PLACEMENT_3D('',#39872,#24337,#24338);
#22340=AXIS2_PLACEMENT_3D('',#39909,#24340,#24341);
#22341=AXIS2_PLACEMENT_3D('',#39946,#24343,#24344);
#22342=AXIS2_PLACEMENT_3D('',#39984,#24346,#24347);
#22343=AXIS2_PLACEMENT_3D('',#40020,#24349,#24350);
#22344=AXIS2_PLACEMENT_3D('',#40058,#24352,#24353);
#22345=AXIS2_PLACEMENT_3D('',#40096,#24355,#24356);
#22346=AXIS2_PLACEMENT_3D('',#40132,#24358,#24359);
#22347=AXIS2_PLACEMENT_3D('',#40170,#24361,#24362);
#22348=AXIS2_PLACEMENT_3D('',#40208,#24364,#24365);
#22349=AXIS2_PLACEMENT_3D('',#40244,#24367,#24368);
#22350=AXIS2_PLACEMENT_3D('',#40282,#24370,#24371);
#22351=AXIS2_PLACEMENT_3D('',#40319,#24373,#24374);
#22352=AXIS2_PLACEMENT_3D('',#40356,#24376,#24377);
#22353=AXIS2_PLACEMENT_3D('',#40368,#24379,#24380);
#22354=AXIS2_PLACEMENT_3D('',#40376,#24381,#24382);
#22355=AXIS2_PLACEMENT_3D('',#40389,#24384,#24385);
#22356=AXIS2_PLACEMENT_3D('',#40392,#24387,#24388);
#22357=AXIS2_PLACEMENT_3D('',#40394,#24389,#24390);
#22358=AXIS2_PLACEMENT_3D('',#40411,#24391,#24392);
#22359=AXIS2_PLACEMENT_3D('',#40501,#24394,#24395);
#22360=AXIS2_PLACEMENT_3D('',#40588,#24397,#24398);
#22361=AXIS2_PLACEMENT_3D('',#40675,#24400,#24401);
#22362=AXIS2_PLACEMENT_3D('',#40762,#24403,#24404);
#22363=AXIS2_PLACEMENT_3D('',#40849,#24406,#24407);
#22364=AXIS2_PLACEMENT_3D('',#40939,#24409,#24410);
#22365=AXIS2_PLACEMENT_3D('',#41026,#24412,#24413);
#22366=AXIS2_PLACEMENT_3D('',#41113,#24415,#24416);
#22367=AXIS2_PLACEMENT_3D('',#41200,#24418,#24419);
#22368=AXIS2_PLACEMENT_3D('',#41287,#24421,#24422);
#22369=AXIS2_PLACEMENT_3D('',#41377,#24424,#24425);
#22370=AXIS2_PLACEMENT_3D('',#41464,#24427,#24428);
#22371=AXIS2_PLACEMENT_3D('',#41551,#24430,#24431);
#22372=AXIS2_PLACEMENT_3D('',#41638,#24433,#24434);
#22373=AXIS2_PLACEMENT_3D('',#41725,#24436,#24437);
#22374=AXIS2_PLACEMENT_3D('',#41812,#24439,#24440);
#22375=AXIS2_PLACEMENT_3D('',#41899,#24442,#24443);
#22376=AXIS2_PLACEMENT_3D('',#41986,#24445,#24446);
#22377=AXIS2_PLACEMENT_3D('',#42061,#24448,#24449);
#22378=AXIS2_PLACEMENT_3D('',#42109,#24451,#24452);
#22379=AXIS2_PLACEMENT_3D('',#42166,#24454,#24455);
#22380=AXIS2_PLACEMENT_3D('',#42253,#24457,#24458);
#22381=AXIS2_PLACEMENT_3D('',#42340,#24460,#24461);
#22382=AXIS2_PLACEMENT_3D('',#42427,#24463,#24464);
#22383=AXIS2_PLACEMENT_3D('',#42514,#24466,#24467);
#22384=AXIS2_PLACEMENT_3D('',#42601,#24469,#24470);
#22385=AXIS2_PLACEMENT_3D('',#42691,#24472,#24473);
#22386=AXIS2_PLACEMENT_3D('',#42778,#24475,#24476);
#22387=AXIS2_PLACEMENT_3D('',#42865,#24478,#24479);
#22388=AXIS2_PLACEMENT_3D('',#42952,#24481,#24482);
#22389=AXIS2_PLACEMENT_3D('',#43039,#24484,#24485);
#22390=AXIS2_PLACEMENT_3D('',#43129,#24487,#24488);
#22391=AXIS2_PLACEMENT_3D('',#43216,#24490,#24491);
#22392=AXIS2_PLACEMENT_3D('',#43303,#24493,#24494);
#22393=AXIS2_PLACEMENT_3D('',#43390,#24496,#24497);
#22394=AXIS2_PLACEMENT_3D('',#43477,#24499,#24500);
#22395=AXIS2_PLACEMENT_3D('',#43567,#24502,#24503);
#22396=AXIS2_PLACEMENT_3D('',#43654,#24505,#24506);
#22397=AXIS2_PLACEMENT_3D('',#43685,#24508,#24509);
#22398=AXIS2_PLACEMENT_3D('',#43723,#24510,#24511);
#22399=AXIS2_PLACEMENT_3D('',#43741,#24513,#24514);
#22400=AXIS2_PLACEMENT_3D('',#43756,#24515,#24516);
#22401=AXIS2_PLACEMENT_3D('',#43793,#24518,#24519);
#22402=AXIS2_PLACEMENT_3D('',#43831,#24521,#24522);
#22403=AXIS2_PLACEMENT_3D('',#43867,#24524,#24525);
#22404=AXIS2_PLACEMENT_3D('',#43905,#24527,#24528);
#22405=AXIS2_PLACEMENT_3D('',#43942,#24530,#24531);
#22406=AXIS2_PLACEMENT_3D('',#43979,#24533,#24534);
#22407=AXIS2_PLACEMENT_3D('',#44017,#24536,#24537);
#22408=AXIS2_PLACEMENT_3D('',#44053,#24539,#24540);
#22409=AXIS2_PLACEMENT_3D('',#44091,#24542,#24543);
#22410=AXIS2_PLACEMENT_3D('',#44128,#24545,#24546);
#22411=AXIS2_PLACEMENT_3D('',#44165,#24548,#24549);
#22412=AXIS2_PLACEMENT_3D('',#44203,#24551,#24552);
#22413=AXIS2_PLACEMENT_3D('',#44239,#24554,#24555);
#22414=AXIS2_PLACEMENT_3D('',#44277,#24557,#24558);
#22415=AXIS2_PLACEMENT_3D('',#44314,#24560,#24561);
#22416=AXIS2_PLACEMENT_3D('',#44351,#24563,#24564);
#22417=AXIS2_PLACEMENT_3D('',#44389,#24566,#24567);
#22418=AXIS2_PLACEMENT_3D('',#44425,#24569,#24570);
#22419=AXIS2_PLACEMENT_3D('',#44452,#24572,#24573);
#22420=AXIS2_PLACEMENT_3D('',#44476,#24575,#24576);
#22421=AXIS2_PLACEMENT_3D('',#44509,#24578,#24579);
#22422=AXIS2_PLACEMENT_3D('',#44547,#24581,#24582);
#22423=AXIS2_PLACEMENT_3D('',#44583,#24584,#24585);
#22424=AXIS2_PLACEMENT_3D('',#44621,#24587,#24588);
#22425=AXIS2_PLACEMENT_3D('',#44657,#24590,#24591);
#22426=AXIS2_PLACEMENT_3D('',#44695,#24593,#24594);
#22427=AXIS2_PLACEMENT_3D('',#44733,#24596,#24597);
#22428=AXIS2_PLACEMENT_3D('',#44769,#24599,#24600);
#22429=AXIS2_PLACEMENT_3D('',#44807,#24602,#24603);
#22430=AXIS2_PLACEMENT_3D('',#44843,#24605,#24606);
#22431=AXIS2_PLACEMENT_3D('',#44881,#24608,#24609);
#22432=AXIS2_PLACEMENT_3D('',#44919,#24611,#24612);
#22433=AXIS2_PLACEMENT_3D('',#44955,#24614,#24615);
#22434=AXIS2_PLACEMENT_3D('',#44993,#24617,#24618);
#22435=AXIS2_PLACEMENT_3D('',#45029,#24620,#24621);
#22436=AXIS2_PLACEMENT_3D('',#45067,#24623,#24624);
#22437=AXIS2_PLACEMENT_3D('',#45105,#24626,#24627);
#22438=AXIS2_PLACEMENT_3D('',#45141,#24629,#24630);
#22439=AXIS2_PLACEMENT_3D('',#45153,#24632,#24633);
#22440=AXIS2_PLACEMENT_3D('',#45161,#24634,#24635);
#22441=AXIS2_PLACEMENT_3D('',#45371,#24636,#24637);
#22442=AXIS2_PLACEMENT_3D('',#49677,#24638,#24639);
#22443=AXIS2_PLACEMENT_3D('',#49678,#24640,#24641);
#22444=AXIS2_PLACEMENT_3D('',#49680,#24642,#24643);
#22445=AXIS2_PLACEMENT_3D('',#49681,#24644,#24645);
#22446=AXIS2_PLACEMENT_3D('',#49888,#24646,#24647);
#22447=AXIS2_PLACEMENT_3D('',#52802,#24648,#24649);
#22448=AXIS2_PLACEMENT_3D('',#52803,#24650,#24651);
#22449=AXIS2_PLACEMENT_3D('',#52805,#24652,#24653);
#22450=AXIS2_PLACEMENT_3D('',#52806,#24654,#24655);
#22451=AXIS2_PLACEMENT_3D('',#52809,#24656,#24657);
#22452=AXIS2_PLACEMENT_3D('',#52813,#24659,#24660);
#22453=AXIS2_PLACEMENT_3D('',#52815,#24662,#24663);
#22454=AXIS2_PLACEMENT_3D('',#52821,#24667,#24668);
#22455=AXIS2_PLACEMENT_3D('',#52825,#24670,#24671);
#22456=AXIS2_PLACEMENT_3D('',#52829,#24673,#24674);
#22457=AXIS2_PLACEMENT_3D('',#52833,#24676,#24677);
#22458=AXIS2_PLACEMENT_3D('',#52837,#24679,#24680);
#22459=AXIS2_PLACEMENT_3D('',#52841,#24682,#24683);
#22460=AXIS2_PLACEMENT_3D('',#52845,#24685,#24686);
#22461=AXIS2_PLACEMENT_3D('',#52849,#24688,#24689);
#22462=AXIS2_PLACEMENT_3D('',#52853,#24691,#24692);
#22463=AXIS2_PLACEMENT_3D('',#52857,#24694,#24695);
#22464=AXIS2_PLACEMENT_3D('',#52861,#24697,#24698);
#22465=AXIS2_PLACEMENT_3D('',#52865,#24700,#24701);
#22466=AXIS2_PLACEMENT_3D('',#52869,#24703,#24704);
#22467=AXIS2_PLACEMENT_3D('',#52873,#24706,#24707);
#22468=AXIS2_PLACEMENT_3D('',#52877,#24709,#24710);
#22469=AXIS2_PLACEMENT_3D('',#52881,#24712,#24713);
#22470=AXIS2_PLACEMENT_3D('',#52885,#24715,#24716);
#22471=AXIS2_PLACEMENT_3D('',#52889,#24718,#24719);
#22472=AXIS2_PLACEMENT_3D('',#52893,#24721,#24722);
#22473=AXIS2_PLACEMENT_3D('',#52897,#24724,#24725);
#22474=AXIS2_PLACEMENT_3D('',#52901,#24727,#24728);
#22475=AXIS2_PLACEMENT_3D('',#52905,#24730,#24731);
#22476=AXIS2_PLACEMENT_3D('',#52909,#24733,#24734);
#22477=AXIS2_PLACEMENT_3D('',#52913,#24736,#24737);
#22478=AXIS2_PLACEMENT_3D('',#52917,#24739,#24740);
#22479=AXIS2_PLACEMENT_3D('',#52921,#24742,#24743);
#22480=AXIS2_PLACEMENT_3D('',#52925,#24745,#24746);
#22481=AXIS2_PLACEMENT_3D('',#52929,#24748,#24749);
#22482=AXIS2_PLACEMENT_3D('',#52933,#24751,#24752);
#22483=AXIS2_PLACEMENT_3D('',#52937,#24754,#24755);
#22484=AXIS2_PLACEMENT_3D('',#52941,#24757,#24758);
#22485=AXIS2_PLACEMENT_3D('',#52945,#24760,#24761);
#22486=AXIS2_PLACEMENT_3D('',#52949,#24763,#24764);
#22487=AXIS2_PLACEMENT_3D('',#52953,#24766,#24767);
#22488=AXIS2_PLACEMENT_3D('',#52957,#24769,#24770);
#22489=AXIS2_PLACEMENT_3D('',#52960,#24772,#24773);
#22490=AXIS2_PLACEMENT_3D('',#52962,#24774,#24775);
#22491=AXIS2_PLACEMENT_3D('',#52964,#24776,#24777);
#22492=AXIS2_PLACEMENT_3D('',#52966,#24778,#24779);
#22493=AXIS2_PLACEMENT_3D('',#52968,#24780,#24781);
#22494=AXIS2_PLACEMENT_3D('',#52969,#24782,#24783);
#22495=AXIS2_PLACEMENT_3D('',#52972,#24784,#24785);
#22496=AXIS2_PLACEMENT_3D('',#52975,#24788,#24789);
#22497=AXIS2_PLACEMENT_3D('',#52979,#24792,#24793);
#22498=AXIS2_PLACEMENT_3D('',#52981,#24794,#24795);
#22499=AXIS2_PLACEMENT_3D('',#52983,#24797,#24798);
#22500=AXIS2_PLACEMENT_3D('',#52987,#24801,#24802);
#22501=AXIS2_PLACEMENT_3D('',#52989,#24803,#24804);
#22502=AXIS2_PLACEMENT_3D('',#52991,#24806,#24807);
#22503=AXIS2_PLACEMENT_3D('',#52995,#24810,#24811);
#22504=AXIS2_PLACEMENT_3D('',#52997,#24812,#24813);
#22505=AXIS2_PLACEMENT_3D('',#52999,#24815,#24816);
#22506=AXIS2_PLACEMENT_3D('',#53003,#24819,#24820);
#22507=AXIS2_PLACEMENT_3D('',#53005,#24821,#24822);
#22508=AXIS2_PLACEMENT_3D('',#53007,#24824,#24825);
#22509=AXIS2_PLACEMENT_3D('',#53011,#24827,#24828);
#22510=AXIS2_PLACEMENT_3D('',#53013,#24830,#24831);
#22511=AXIS2_PLACEMENT_3D('',#53017,#24834,#24835);
#22512=AXIS2_PLACEMENT_3D('',#53019,#24836,#24837);
#22513=AXIS2_PLACEMENT_3D('',#53021,#24839,#24840);
#22514=AXIS2_PLACEMENT_3D('',#53025,#24842,#24843);
#22515=AXIS2_PLACEMENT_3D('',#53027,#24845,#24846);
#22516=AXIS2_PLACEMENT_3D('',#53031,#24849,#24850);
#22517=AXIS2_PLACEMENT_3D('',#53033,#24851,#24852);
#22518=AXIS2_PLACEMENT_3D('',#53035,#24854,#24855);
#22519=AXIS2_PLACEMENT_3D('',#53038,#24856,#24857);
#22520=AXIS2_PLACEMENT_3D('',#53041,#24860,#24861);
#22521=AXIS2_PLACEMENT_3D('',#53045,#24864,#24865);
#22522=AXIS2_PLACEMENT_3D('',#53047,#24866,#24867);
#22523=AXIS2_PLACEMENT_3D('',#53049,#24869,#24870);
#22524=AXIS2_PLACEMENT_3D('',#53053,#24873,#24874);
#22525=AXIS2_PLACEMENT_3D('',#53055,#24875,#24876);
#22526=AXIS2_PLACEMENT_3D('',#53057,#24878,#24879);
#22527=AXIS2_PLACEMENT_3D('',#53061,#24882,#24883);
#22528=AXIS2_PLACEMENT_3D('',#53063,#24884,#24885);
#22529=AXIS2_PLACEMENT_3D('',#53065,#24887,#24888);
#22530=AXIS2_PLACEMENT_3D('',#53069,#24891,#24892);
#22531=AXIS2_PLACEMENT_3D('',#53071,#24893,#24894);
#22532=AXIS2_PLACEMENT_3D('',#53073,#24896,#24897);
#22533=AXIS2_PLACEMENT_3D('',#53077,#24899,#24900);
#22534=AXIS2_PLACEMENT_3D('',#53079,#24902,#24903);
#22535=AXIS2_PLACEMENT_3D('',#53083,#24906,#24907);
#22536=AXIS2_PLACEMENT_3D('',#53085,#24908,#24909);
#22537=AXIS2_PLACEMENT_3D('',#53087,#24911,#24912);
#22538=AXIS2_PLACEMENT_3D('',#53091,#24914,#24915);
#22539=AXIS2_PLACEMENT_3D('',#53093,#24917,#24918);
#22540=AXIS2_PLACEMENT_3D('',#53097,#24921,#24922);
#22541=AXIS2_PLACEMENT_3D('',#53099,#24923,#24924);
#22542=AXIS2_PLACEMENT_3D('',#53101,#24926,#24927);
#22543=AXIS2_PLACEMENT_3D('',#53104,#24928,#24929);
#22544=AXIS2_PLACEMENT_3D('',#53107,#24932,#24933);
#22545=AXIS2_PLACEMENT_3D('',#53111,#24936,#24937);
#22546=AXIS2_PLACEMENT_3D('',#53113,#24938,#24939);
#22547=AXIS2_PLACEMENT_3D('',#53115,#24941,#24942);
#22548=AXIS2_PLACEMENT_3D('',#53119,#24945,#24946);
#22549=AXIS2_PLACEMENT_3D('',#53121,#24947,#24948);
#22550=AXIS2_PLACEMENT_3D('',#53123,#24950,#24951);
#22551=AXIS2_PLACEMENT_3D('',#53127,#24954,#24955);
#22552=AXIS2_PLACEMENT_3D('',#53129,#24956,#24957);
#22553=AXIS2_PLACEMENT_3D('',#53131,#24959,#24960);
#22554=AXIS2_PLACEMENT_3D('',#53135,#24963,#24964);
#22555=AXIS2_PLACEMENT_3D('',#53137,#24965,#24966);
#22556=AXIS2_PLACEMENT_3D('',#53139,#24968,#24969);
#22557=AXIS2_PLACEMENT_3D('',#53143,#24971,#24972);
#22558=AXIS2_PLACEMENT_3D('',#53145,#24974,#24975);
#22559=AXIS2_PLACEMENT_3D('',#53149,#24978,#24979);
#22560=AXIS2_PLACEMENT_3D('',#53151,#24980,#24981);
#22561=AXIS2_PLACEMENT_3D('',#53153,#24983,#24984);
#22562=AXIS2_PLACEMENT_3D('',#53157,#24986,#24987);
#22563=AXIS2_PLACEMENT_3D('',#53159,#24989,#24990);
#22564=AXIS2_PLACEMENT_3D('',#53163,#24993,#24994);
#22565=AXIS2_PLACEMENT_3D('',#53165,#24995,#24996);
#22566=AXIS2_PLACEMENT_3D('',#53167,#24998,#24999);
#22567=AXIS2_PLACEMENT_3D('',#53170,#25000,#25001);
#22568=AXIS2_PLACEMENT_3D('',#53173,#25004,#25005);
#22569=AXIS2_PLACEMENT_3D('',#53177,#25008,#25009);
#22570=AXIS2_PLACEMENT_3D('',#53179,#25010,#25011);
#22571=AXIS2_PLACEMENT_3D('',#53181,#25013,#25014);
#22572=AXIS2_PLACEMENT_3D('',#53185,#25017,#25018);
#22573=AXIS2_PLACEMENT_3D('',#53187,#25019,#25020);
#22574=AXIS2_PLACEMENT_3D('',#53189,#25022,#25023);
#22575=AXIS2_PLACEMENT_3D('',#53193,#25026,#25027);
#22576=AXIS2_PLACEMENT_3D('',#53195,#25028,#25029);
#22577=AXIS2_PLACEMENT_3D('',#53197,#25031,#25032);
#22578=AXIS2_PLACEMENT_3D('',#53201,#25035,#25036);
#22579=AXIS2_PLACEMENT_3D('',#53203,#25037,#25038);
#22580=AXIS2_PLACEMENT_3D('',#53205,#25040,#25041);
#22581=AXIS2_PLACEMENT_3D('',#53209,#25043,#25044);
#22582=AXIS2_PLACEMENT_3D('',#53211,#25046,#25047);
#22583=AXIS2_PLACEMENT_3D('',#53215,#25050,#25051);
#22584=AXIS2_PLACEMENT_3D('',#53217,#25052,#25053);
#22585=AXIS2_PLACEMENT_3D('',#53219,#25055,#25056);
#22586=AXIS2_PLACEMENT_3D('',#53222,#25058,#25059);
#22587=AXIS2_PLACEMENT_3D('',#53223,#25060,#25061);
#22588=AXIS2_PLACEMENT_3D('',#53226,#25063,#25064);
#22589=AXIS2_PLACEMENT_3D('',#53227,#25065,#25066);
#22590=AXIS2_PLACEMENT_3D('',#53230,#25068,#25069);
#22591=AXIS2_PLACEMENT_3D('',#53231,#25070,#25071);
#22592=AXIS2_PLACEMENT_3D('',#53233,#25073,#25074);
#22593=AXIS2_PLACEMENT_3D('',#53236,#25076,#25077);
#22594=AXIS2_PLACEMENT_3D('',#53237,#25078,#25079);
#22595=AXIS2_PLACEMENT_3D('',#53240,#25081,#25082);
#22596=AXIS2_PLACEMENT_3D('',#53241,#25083,#25084);
#22597=AXIS2_PLACEMENT_3D('',#53243,#25086,#25087);
#22598=AXIS2_PLACEMENT_3D('',#53245,#25089,#25090);
#22599=AXIS2_PLACEMENT_3D('',#53247,#25092,#25093);
#22600=AXIS2_PLACEMENT_3D('',#53249,#25095,#25096);
#22601=AXIS2_PLACEMENT_3D('',#53251,#25098,#25099);
#22602=AXIS2_PLACEMENT_3D('',#53253,#25101,#25102);
#22603=AXIS2_PLACEMENT_3D('',#53255,#25104,#25105);
#22604=AXIS2_PLACEMENT_3D('',#53257,#25107,#25108);
#22605=AXIS2_PLACEMENT_3D('',#53259,#25110,#25111);
#22606=AXIS2_PLACEMENT_3D('',#53261,#25113,#25114);
#22607=AXIS2_PLACEMENT_3D('',#53263,#25116,#25117);
#22608=AXIS2_PLACEMENT_3D('',#53265,#25119,#25120);
#24216=DIRECTION('axis',(0.,0.,1.));
#24217=DIRECTION('refdir',(1.,0.,0.));
#24218=DIRECTION('center_axis',(0.,0.,-1.));
#24219=DIRECTION('ref_axis',(1.,0.,0.));
#24220=DIRECTION('',(0.,0.,-1.));
#24221=DIRECTION('center_axis',(0.,0.,1.));
#24222=DIRECTION('ref_axis',(1.,0.,0.));
#24223=DIRECTION('',(0.,0.,-1.));
#24224=DIRECTION('center_axis',(0.,0.,1.));
#24225=DIRECTION('ref_axis',(1.,0.,0.));
#24226=DIRECTION('center_axis',(0.,0.,1.));
#24227=DIRECTION('ref_axis',(1.,0.,0.));
#24228=DIRECTION('center_axis',(0.,0.,-1.));
#24229=DIRECTION('ref_axis',(1.,0.,0.));
#24230=DIRECTION('',(0.,0.,-1.));
#24231=DIRECTION('center_axis',(0.,0.,-1.));
#24232=DIRECTION('ref_axis',(1.,0.,0.));
#24233=DIRECTION('',(0.,0.,-1.));
#24234=DIRECTION('center_axis',(0.,0.,-1.));
#24235=DIRECTION('ref_axis',(1.,0.,0.));
#24236=DIRECTION('',(0.,0.,-1.));
#24237=DIRECTION('center_axis',(0.,0.,-1.));
#24238=DIRECTION('ref_axis',(1.,0.,0.));
#24239=DIRECTION('',(0.,0.,-1.));
#24240=DIRECTION('center_axis',(0.,0.,-1.));
#24241=DIRECTION('ref_axis',(1.,0.,0.));
#24242=DIRECTION('',(0.,0.,-1.));
#24243=DIRECTION('center_axis',(0.,0.,-1.));
#24244=DIRECTION('ref_axis',(1.,0.,0.));
#24245=DIRECTION('',(0.,0.,-1.));
#24246=DIRECTION('center_axis',(0.,0.,-1.));
#24247=DIRECTION('ref_axis',(1.,0.,0.));
#24248=DIRECTION('',(0.,0.,-1.));
#24249=DIRECTION('center_axis',(0.,0.,-1.));
#24250=DIRECTION('ref_axis',(1.,0.,0.));
#24251=DIRECTION('',(0.,0.,-1.));
#24252=DIRECTION('center_axis',(0.,0.,-1.));
#24253=DIRECTION('ref_axis',(1.,0.,0.));
#24254=DIRECTION('',(0.,0.,-1.));
#24255=DIRECTION('center_axis',(0.,0.,-1.));
#24256=DIRECTION('ref_axis',(1.,0.,0.));
#24257=DIRECTION('',(0.,0.,-1.));
#24258=DIRECTION('center_axis',(0.,0.,-1.));
#24259=DIRECTION('ref_axis',(1.,0.,0.));
#24260=DIRECTION('',(0.,0.,-1.));
#24261=DIRECTION('center_axis',(0.,0.,-1.));
#24262=DIRECTION('ref_axis',(1.,0.,0.));
#24263=DIRECTION('',(0.,0.,-1.));
#24264=DIRECTION('center_axis',(0.,0.,-1.));
#24265=DIRECTION('ref_axis',(1.,0.,0.));
#24266=DIRECTION('',(0.,0.,-1.));
#24267=DIRECTION('center_axis',(0.,0.,-1.));
#24268=DIRECTION('ref_axis',(1.,0.,0.));
#24269=DIRECTION('',(0.,0.,-1.));
#24270=DIRECTION('center_axis',(0.,0.,-1.));
#24271=DIRECTION('ref_axis',(1.,0.,0.));
#24272=DIRECTION('',(0.,0.,-1.));
#24273=DIRECTION('center_axis',(0.,0.,-1.));
#24274=DIRECTION('ref_axis',(1.,0.,0.));
#24275=DIRECTION('',(0.,0.,-1.));
#24276=DIRECTION('center_axis',(0.,0.,-1.));
#24277=DIRECTION('ref_axis',(1.,0.,0.));
#24278=DIRECTION('',(0.,0.,-1.));
#24279=DIRECTION('center_axis',(0.,0.,-1.));
#24280=DIRECTION('ref_axis',(1.,0.,0.));
#24281=DIRECTION('',(0.,0.,-1.));
#24282=DIRECTION('center_axis',(0.,0.,-1.));
#24283=DIRECTION('ref_axis',(1.,0.,0.));
#24284=DIRECTION('',(0.,0.,-1.));
#24285=DIRECTION('center_axis',(0.,0.,-1.));
#24286=DIRECTION('ref_axis',(1.,0.,0.));
#24287=DIRECTION('',(0.,0.,-1.));
#24288=DIRECTION('center_axis',(0.,0.,-1.));
#24289=DIRECTION('ref_axis',(1.,0.,0.));
#24290=DIRECTION('',(0.,0.,-1.));
#24291=DIRECTION('center_axis',(0.,0.,-1.));
#24292=DIRECTION('ref_axis',(1.,0.,0.));
#24293=DIRECTION('',(0.,0.,-1.));
#24294=DIRECTION('center_axis',(0.,0.,-1.));
#24295=DIRECTION('ref_axis',(1.,0.,0.));
#24296=DIRECTION('',(0.,0.,-1.));
#24297=DIRECTION('center_axis',(0.,0.,-1.));
#24298=DIRECTION('ref_axis',(0.938097899428847,-0.346370222575766,0.));
#24299=DIRECTION('',(0.,0.,-1.));
#24300=DIRECTION('center_axis',(0.,0.,-1.));
#24301=DIRECTION('ref_axis',(1.,0.,0.));
#24302=DIRECTION('center_axis',(0.,0.,-1.));
#24303=DIRECTION('ref_axis',(0.793346897669268,0.608769825105144,0.));
#24304=DIRECTION('',(1.22464679914735E-16,3.85574710022057E-30,-1.));
#24305=DIRECTION('center_axis',(0.,0.,1.));
#24306=DIRECTION('ref_axis',(1.,3.16070290694603E-14,0.));
#24307=DIRECTION('center_axis',(0.,0.,-1.));
#24308=DIRECTION('ref_axis',(1.,3.16070290694603E-14,0.));
#24309=DIRECTION('',(1.22464679914735E-16,3.85574710022057E-30,-1.));
#24310=DIRECTION('center_axis',(0.,0.,-1.));
#24311=DIRECTION('ref_axis',(1.,3.16070290694603E-14,0.));
#24312=DIRECTION('',(1.22464679914735E-16,3.85574710022057E-30,-1.));
#24313=DIRECTION('center_axis',(0.,0.,-1.));
#24314=DIRECTION('ref_axis',(1.,3.16070290694603E-14,0.));
#24315=DIRECTION('',(1.22464679914735E-16,3.85574710022057E-30,-1.));
#24316=DIRECTION('center_axis',(0.,0.,-1.));
#24317=DIRECTION('ref_axis',(1.,3.16070290694603E-14,0.));
#24318=DIRECTION('',(1.22464679914735E-16,3.85574710022057E-30,-1.));
#24319=DIRECTION('center_axis',(0.,0.,-1.));
#24320=DIRECTION('ref_axis',(1.,3.16070290694603E-14,0.));
#24321=DIRECTION('',(1.22464679914735E-16,3.85574710022057E-30,-1.));
#24322=DIRECTION('center_axis',(0.,0.,-1.));
#24323=DIRECTION('ref_axis',(1.,3.16070290694603E-14,0.));
#24324=DIRECTION('',(1.22464679914735E-16,3.85574710022057E-30,-1.));
#24325=DIRECTION('center_axis',(0.,0.,-1.));
#24326=DIRECTION('ref_axis',(1.,3.16070290694603E-14,0.));
#24327=DIRECTION('',(1.22464679914735E-16,3.85574710022057E-30,-1.));
#24328=DIRECTION('center_axis',(0.,0.,-1.));
#24329=DIRECTION('ref_axis',(1.,3.16070290694603E-14,0.));
#24330=DIRECTION('',(1.22464679914735E-16,3.85574710022057E-30,-1.));
#24331=DIRECTION('center_axis',(0.,0.,-1.));
#24332=DIRECTION('ref_axis',(1.,3.16070290694603E-14,0.));
#24333=DIRECTION('',(1.22464679914735E-16,3.85574710022057E-30,-1.));
#24334=DIRECTION('center_axis',(0.,0.,-1.));
#24335=DIRECTION('ref_axis',(1.,3.16070290694603E-14,0.));
#24336=DIRECTION('',(1.22464679914735E-16,3.85574710022057E-30,-1.));
#24337=DIRECTION('center_axis',(0.,0.,-1.));
#24338=DIRECTION('ref_axis',(1.,3.16070290694603E-14,0.));
#24339=DIRECTION('',(1.22464679914735E-16,3.85574710022057E-30,-1.));
#24340=DIRECTION('center_axis',(0.,0.,-1.));
#24341=DIRECTION('ref_axis',(1.,3.16070290694603E-14,0.));
#24342=DIRECTION('',(1.22464679914735E-16,3.85574710022057E-30,-1.));
#24343=DIRECTION('center_axis',(0.,0.,-1.));
#24344=DIRECTION('ref_axis',(1.,3.16070290694603E-14,0.));
#24345=DIRECTION('',(1.22464679914735E-16,3.85574710022057E-30,-1.));
#24346=DIRECTION('center_axis',(0.,0.,-1.));
#24347=DIRECTION('ref_axis',(1.,3.16070290694603E-14,0.));
#24348=DIRECTION('',(1.22464679914735E-16,3.85574710022057E-30,-1.));
#24349=DIRECTION('center_axis',(0.,0.,-1.));
#24350=DIRECTION('ref_axis',(1.,3.16070290694603E-14,0.));
#24351=DIRECTION('',(1.22464679914735E-16,3.85574710022057E-30,-1.));
#24352=DIRECTION('center_axis',(0.,0.,-1.));
#24353=DIRECTION('ref_axis',(1.,3.16070290694603E-14,0.));
#24354=DIRECTION('',(1.22464679914735E-16,3.85574710022057E-30,-1.));
#24355=DIRECTION('center_axis',(0.,0.,-1.));
#24356=DIRECTION('ref_axis',(1.,3.16070290694603E-14,0.));
#24357=DIRECTION('',(1.22464679914735E-16,3.85574710022057E-30,-1.));
#24358=DIRECTION('center_axis',(0.,0.,-1.));
#24359=DIRECTION('ref_axis',(1.,3.16070290694603E-14,0.));
#24360=DIRECTION('',(1.22464679914735E-16,3.85574710022057E-30,-1.));
#24361=DIRECTION('center_axis',(0.,0.,-1.));
#24362=DIRECTION('ref_axis',(1.,3.16070290694603E-14,0.));
#24363=DIRECTION('',(1.22464679914735E-16,3.85574710022057E-30,-1.));
#24364=DIRECTION('center_axis',(0.,0.,-1.));
#24365=DIRECTION('ref_axis',(1.,3.16070290694603E-14,0.));
#24366=DIRECTION('',(1.22464679914735E-16,3.85574710022057E-30,-1.));
#24367=DIRECTION('center_axis',(0.,0.,-1.));
#24368=DIRECTION('ref_axis',(1.,3.16070290694603E-14,0.));
#24369=DIRECTION('',(1.22464679914735E-16,3.85574710022057E-30,-1.));
#24370=DIRECTION('center_axis',(0.,0.,-1.));
#24371=DIRECTION('ref_axis',(1.,3.16070290694603E-14,0.));
#24372=DIRECTION('',(1.22464679914735E-16,3.85574710022057E-30,-1.));
#24373=DIRECTION('center_axis',(0.,0.,-1.));
#24374=DIRECTION('ref_axis',(1.,3.16070290694603E-14,0.));
#24375=DIRECTION('',(1.22464679914735E-16,3.85574710022057E-30,-1.));
#24376=DIRECTION('center_axis',(0.,0.,-1.));
#24377=DIRECTION('ref_axis',(-0.6087766502803,-0.793341660366766,0.));
#24378=DIRECTION('',(1.22464679914735E-16,3.85574710022057E-30,-1.));
#24379=DIRECTION('center_axis',(0.,0.,-1.));
#24380=DIRECTION('ref_axis',(1.,3.16070290694603E-14,0.));
#24381=DIRECTION('center_axis',(0.,0.,1.));
#24382=DIRECTION('ref_axis',(-1.,0.,0.));
#24383=DIRECTION('',(0.,0.,1.));
#24384=DIRECTION('center_axis',(0.,0.,-1.));
#24385=DIRECTION('ref_axis',(-1.,0.,0.));
#24386=DIRECTION('',(0.,0.,1.));
#24387=DIRECTION('center_axis',(0.,0.,-1.));
#24388=DIRECTION('ref_axis',(-1.,0.,0.));
#24389=DIRECTION('center_axis',(0.,0.,-1.));
#24390=DIRECTION('ref_axis',(-1.,0.,0.));
#24391=DIRECTION('center_axis',(0.,0.,1.));
#24392=DIRECTION('ref_axis',(-1.,0.,0.));
#24393=DIRECTION('',(0.,0.,1.));
#24394=DIRECTION('center_axis',(0.,0.,1.));
#24395=DIRECTION('ref_axis',(-1.,0.,0.));
#24396=DIRECTION('',(0.,0.,1.));
#24397=DIRECTION('center_axis',(0.,0.,1.));
#24398=DIRECTION('ref_axis',(-1.,0.,0.));
#24399=DIRECTION('',(0.,0.,1.));
#24400=DIRECTION('center_axis',(0.,0.,1.));
#24401=DIRECTION('ref_axis',(-1.,0.,0.));
#24402=DIRECTION('',(0.,0.,1.));
#24403=DIRECTION('center_axis',(0.,0.,1.));
#24404=DIRECTION('ref_axis',(-1.,0.,0.));
#24405=DIRECTION('',(0.,0.,1.));
#24406=DIRECTION('center_axis',(0.,0.,1.));
#24407=DIRECTION('ref_axis',(-1.,0.,0.));
#24408=DIRECTION('',(0.,0.,1.));
#24409=DIRECTION('center_axis',(0.,0.,1.));
#24410=DIRECTION('ref_axis',(-1.,0.,0.));
#24411=DIRECTION('',(0.,0.,1.));
#24412=DIRECTION('center_axis',(0.,0.,1.));
#24413=DIRECTION('ref_axis',(-1.,0.,0.));
#24414=DIRECTION('',(0.,0.,1.));
#24415=DIRECTION('center_axis',(0.,0.,1.));
#24416=DIRECTION('ref_axis',(-1.,0.,0.));
#24417=DIRECTION('',(0.,0.,1.));
#24418=DIRECTION('center_axis',(0.,0.,1.));
#24419=DIRECTION('ref_axis',(-1.,0.,0.));
#24420=DIRECTION('',(0.,0.,1.));
#24421=DIRECTION('center_axis',(0.,0.,1.));
#24422=DIRECTION('ref_axis',(-1.,0.,0.));
#24423=DIRECTION('',(0.,0.,1.));
#24424=DIRECTION('center_axis',(0.,0.,1.));
#24425=DIRECTION('ref_axis',(-1.,0.,0.));
#24426=DIRECTION('',(0.,0.,1.));
#24427=DIRECTION('center_axis',(0.,0.,1.));
#24428=DIRECTION('ref_axis',(-1.,0.,0.));
#24429=DIRECTION('',(0.,0.,1.));
#24430=DIRECTION('center_axis',(0.,0.,1.));
#24431=DIRECTION('ref_axis',(-1.,0.,0.));
#24432=DIRECTION('',(0.,0.,1.));
#24433=DIRECTION('center_axis',(0.,0.,1.));
#24434=DIRECTION('ref_axis',(-1.,0.,0.));
#24435=DIRECTION('',(0.,0.,1.));
#24436=DIRECTION('center_axis',(0.,0.,1.));
#24437=DIRECTION('ref_axis',(-1.,0.,0.));
#24438=DIRECTION('',(0.,0.,1.));
#24439=DIRECTION('center_axis',(0.,0.,1.));
#24440=DIRECTION('ref_axis',(-1.,0.,0.));
#24441=DIRECTION('',(0.,0.,1.));
#24442=DIRECTION('center_axis',(0.,0.,1.));
#24443=DIRECTION('ref_axis',(-1.,0.,0.));
#24444=DIRECTION('',(0.,0.,1.));
#24445=DIRECTION('center_axis',(0.,0.,1.));
#24446=DIRECTION('ref_axis',(-1.,0.,0.));
#24447=DIRECTION('',(0.,0.,1.));
#24448=DIRECTION('center_axis',(0.,0.,1.));
#24449=DIRECTION('ref_axis',(-1.,0.,0.));
#24450=DIRECTION('',(0.,0.,1.));
#24451=DIRECTION('center_axis',(0.,0.,1.));
#24452=DIRECTION('ref_axis',(-1.,0.,0.));
#24453=DIRECTION('',(0.,0.,1.));
#24454=DIRECTION('center_axis',(0.,0.,1.));
#24455=DIRECTION('ref_axis',(-1.,0.,0.));
#24456=DIRECTION('',(0.,0.,1.));
#24457=DIRECTION('center_axis',(0.,0.,1.));
#24458=DIRECTION('ref_axis',(-1.,0.,0.));
#24459=DIRECTION('',(0.,0.,1.));
#24460=DIRECTION('center_axis',(0.,0.,1.));
#24461=DIRECTION('ref_axis',(-1.,0.,0.));
#24462=DIRECTION('',(0.,0.,1.));
#24463=DIRECTION('center_axis',(0.,0.,1.));
#24464=DIRECTION('ref_axis',(-1.,0.,0.));
#24465=DIRECTION('',(0.,0.,1.));
#24466=DIRECTION('center_axis',(0.,0.,1.));
#24467=DIRECTION('ref_axis',(-1.,0.,0.));
#24468=DIRECTION('',(0.,0.,1.));
#24469=DIRECTION('center_axis',(0.,0.,1.));
#24470=DIRECTION('ref_axis',(-1.,0.,0.));
#24471=DIRECTION('',(0.,0.,1.));
#24472=DIRECTION('center_axis',(0.,0.,1.));
#24473=DIRECTION('ref_axis',(-1.,0.,0.));
#24474=DIRECTION('',(0.,0.,1.));
#24475=DIRECTION('center_axis',(0.,0.,1.));
#24476=DIRECTION('ref_axis',(-1.,0.,0.));
#24477=DIRECTION('',(0.,0.,1.));
#24478=DIRECTION('center_axis',(0.,0.,1.));
#24479=DIRECTION('ref_axis',(-1.,0.,0.));
#24480=DIRECTION('',(0.,0.,1.));
#24481=DIRECTION('center_axis',(0.,0.,1.));
#24482=DIRECTION('ref_axis',(-1.,0.,0.));
#24483=DIRECTION('',(0.,0.,1.));
#24484=DIRECTION('center_axis',(0.,0.,1.));
#24485=DIRECTION('ref_axis',(-1.,0.,0.));
#24486=DIRECTION('',(0.,0.,1.));
#24487=DIRECTION('center_axis',(0.,0.,1.));
#24488=DIRECTION('ref_axis',(-1.,0.,0.));
#24489=DIRECTION('',(0.,0.,1.));
#24490=DIRECTION('center_axis',(0.,0.,1.));
#24491=DIRECTION('ref_axis',(-1.,0.,0.));
#24492=DIRECTION('',(0.,0.,1.));
#24493=DIRECTION('center_axis',(0.,0.,1.));
#24494=DIRECTION('ref_axis',(-1.,0.,0.));
#24495=DIRECTION('',(0.,0.,1.));
#24496=DIRECTION('center_axis',(0.,0.,1.));
#24497=DIRECTION('ref_axis',(-1.,0.,0.));
#24498=DIRECTION('',(0.,0.,1.));
#24499=DIRECTION('center_axis',(0.,0.,1.));
#24500=DIRECTION('ref_axis',(-1.,0.,0.));
#24501=DIRECTION('',(0.,0.,1.));
#24502=DIRECTION('center_axis',(0.,0.,1.));
#24503=DIRECTION('ref_axis',(-1.,0.,0.));
#24504=DIRECTION('',(0.,0.,1.));
#24505=DIRECTION('center_axis',(0.,0.,1.));
#24506=DIRECTION('ref_axis',(-0.938097369934915,-0.346371656636617,0.));
#24507=DIRECTION('',(0.,0.,1.));
#24508=DIRECTION('center_axis',(0.,0.,-1.));
#24509=DIRECTION('ref_axis',(-1.,0.,0.));
#24510=DIRECTION('center_axis',(0.,0.,1.));
#24511=DIRECTION('ref_axis',(-0.793344496203991,0.608772954674266,0.));
#24512=DIRECTION('',(-1.22464679914735E-16,4.47534497895031E-29,1.));
#24513=DIRECTION('center_axis',(0.,0.,-1.));
#24514=DIRECTION('ref_axis',(-1.,3.65562114876707E-13,0.));
#24515=DIRECTION('center_axis',(0.,0.,1.));
#24516=DIRECTION('ref_axis',(-1.,3.65562114876707E-13,0.));
#24517=DIRECTION('',(-1.22464679914735E-16,4.47534497895031E-29,1.));
#24518=DIRECTION('center_axis',(0.,0.,1.));
#24519=DIRECTION('ref_axis',(-1.,3.65562114876707E-13,0.));
#24520=DIRECTION('',(-1.22464679914735E-16,4.47534497895031E-29,1.));
#24521=DIRECTION('center_axis',(0.,0.,1.));
#24522=DIRECTION('ref_axis',(-1.,3.65562114876707E-13,0.));
#24523=DIRECTION('',(-1.22464679914735E-16,4.47534497895031E-29,1.));
#24524=DIRECTION('center_axis',(0.,0.,1.));
#24525=DIRECTION('ref_axis',(-1.,3.65562114876707E-13,0.));
#24526=DIRECTION('',(-1.22464679914735E-16,4.47534497895031E-29,1.));
#24527=DIRECTION('center_axis',(0.,0.,1.));
#24528=DIRECTION('ref_axis',(-1.,3.65562114876707E-13,0.));
#24529=DIRECTION('',(-1.22464679914735E-16,4.47534497895031E-29,1.));
#24530=DIRECTION('center_axis',(0.,0.,1.));
#24531=DIRECTION('ref_axis',(-1.,3.65562114876707E-13,0.));
#24532=DIRECTION('',(-1.22464679914735E-16,4.47534497895031E-29,1.));
#24533=DIRECTION('center_axis',(0.,0.,1.));
#24534=DIRECTION('ref_axis',(-1.,3.65562114876707E-13,0.));
#24535=DIRECTION('',(-1.22464679914735E-16,4.47534497895031E-29,1.));
#24536=DIRECTION('center_axis',(0.,0.,1.));
#24537=DIRECTION('ref_axis',(-1.,3.65562114876707E-13,0.));
#24538=DIRECTION('',(-1.22464679914735E-16,4.47534497895031E-29,1.));
#24539=DIRECTION('center_axis',(0.,0.,1.));
#24540=DIRECTION('ref_axis',(-1.,3.65562114876707E-13,0.));
#24541=DIRECTION('',(-1.22464679914735E-16,4.47534497895031E-29,1.));
#24542=DIRECTION('center_axis',(0.,0.,1.));
#24543=DIRECTION('ref_axis',(-1.,3.65562114876707E-13,0.));
#24544=DIRECTION('',(-1.22464679914735E-16,4.47534497895031E-29,1.));
#24545=DIRECTION('center_axis',(0.,0.,1.));
#24546=DIRECTION('ref_axis',(-1.,3.65562114876707E-13,0.));
#24547=DIRECTION('',(-1.22464679914735E-16,4.47534497895031E-29,1.));
#24548=DIRECTION('center_axis',(0.,0.,1.));
#24549=DIRECTION('ref_axis',(-1.,3.65562114876707E-13,0.));
#24550=DIRECTION('',(-1.22464679914735E-16,4.47534497895031E-29,1.));
#24551=DIRECTION('center_axis',(0.,0.,1.));
#24552=DIRECTION('ref_axis',(-1.,3.65562114876707E-13,0.));
#24553=DIRECTION('',(-1.22464679914735E-16,4.47534497895031E-29,1.));
#24554=DIRECTION('center_axis',(0.,0.,1.));
#24555=DIRECTION('ref_axis',(-1.,3.65562114876707E-13,0.));
#24556=DIRECTION('',(-1.22464679914735E-16,4.47534497895031E-29,1.));
#24557=DIRECTION('center_axis',(0.,0.,1.));
#24558=DIRECTION('ref_axis',(-1.,3.65562114876707E-13,0.));
#24559=DIRECTION('',(-1.22464679914735E-16,4.47534497895031E-29,1.));
#24560=DIRECTION('center_axis',(0.,0.,1.));
#24561=DIRECTION('ref_axis',(-1.,3.65562114876707E-13,0.));
#24562=DIRECTION('',(-1.22464679914735E-16,4.47534497895031E-29,1.));
#24563=DIRECTION('center_axis',(0.,0.,1.));
#24564=DIRECTION('ref_axis',(-1.,3.65562114876707E-13,0.));
#24565=DIRECTION('',(-1.22464679914735E-16,4.47534497895031E-29,1.));
#24566=DIRECTION('center_axis',(0.,0.,1.));
#24567=DIRECTION('ref_axis',(-1.,3.65562114876707E-13,0.));
#24568=DIRECTION('',(-1.22464679914735E-16,4.47534497895031E-29,1.));
#24569=DIRECTION('center_axis',(0.,0.,1.));
#24570=DIRECTION('ref_axis',(-1.,3.65562114876707E-13,0.));
#24571=DIRECTION('',(-1.22464679914735E-16,4.47534497895031E-29,1.));
#24572=DIRECTION('center_axis',(0.,0.,1.));
#24573=DIRECTION('ref_axis',(-1.,3.65562114876707E-13,0.));
#24574=DIRECTION('',(-1.22464679914735E-16,4.47534497895031E-29,1.));
#24575=DIRECTION('center_axis',(0.,0.,1.));
#24576=DIRECTION('ref_axis',(-1.,3.65562114876707E-13,0.));
#24577=DIRECTION('',(-1.22464679914735E-16,4.47534497895031E-29,1.));
#24578=DIRECTION('center_axis',(0.,0.,1.));
#24579=DIRECTION('ref_axis',(-1.,3.65562114876707E-13,0.));
#24580=DIRECTION('',(-1.22464679914735E-16,4.47534497895031E-29,1.));
#24581=DIRECTION('center_axis',(0.,0.,1.));
#24582=DIRECTION('ref_axis',(-1.,3.65562114876707E-13,0.));
#24583=DIRECTION('',(-1.22464679914735E-16,4.47534497895031E-29,1.));
#24584=DIRECTION('center_axis',(0.,0.,1.));
#24585=DIRECTION('ref_axis',(-1.,3.65562114876707E-13,0.));
#24586=DIRECTION('',(-1.22464679914735E-16,4.47534497895031E-29,1.));
#24587=DIRECTION('center_axis',(0.,0.,1.));
#24588=DIRECTION('ref_axis',(-1.,3.65562114876707E-13,0.));
#24589=DIRECTION('',(-1.22464679914735E-16,4.47534497895031E-29,1.));
#24590=DIRECTION('center_axis',(0.,0.,1.));
#24591=DIRECTION('ref_axis',(-1.,3.65562114876707E-13,0.));
#24592=DIRECTION('',(-1.22464679914735E-16,4.47534497895031E-29,1.));
#24593=DIRECTION('center_axis',(0.,0.,1.));
#24594=DIRECTION('ref_axis',(-1.,3.65562114876707E-13,0.));
#24595=DIRECTION('',(-1.22464679914735E-16,4.47534497895031E-29,1.));
#24596=DIRECTION('center_axis',(0.,0.,1.));
#24597=DIRECTION('ref_axis',(-1.,3.65562114876707E-13,0.));
#24598=DIRECTION('',(-1.22464679914735E-16,4.47534497895031E-29,1.));
#24599=DIRECTION('center_axis',(0.,0.,1.));
#24600=DIRECTION('ref_axis',(-1.,3.65562114876707E-13,0.));
#24601=DIRECTION('',(-1.22464679914735E-16,4.47534497895031E-29,1.));
#24602=DIRECTION('center_axis',(0.,0.,1.));
#24603=DIRECTION('ref_axis',(-1.,3.65562114876707E-13,0.));
#24604=DIRECTION('',(-1.22464679914735E-16,4.47534497895031E-29,1.));
#24605=DIRECTION('center_axis',(0.,0.,1.));
#24606=DIRECTION('ref_axis',(-1.,3.65562114876707E-13,0.));
#24607=DIRECTION('',(-1.22464679914735E-16,4.47534497895031E-29,1.));
#24608=DIRECTION('center_axis',(0.,0.,1.));
#24609=DIRECTION('ref_axis',(-1.,3.65562114876707E-13,0.));
#24610=DIRECTION('',(-1.22464679914735E-16,4.47534497895031E-29,1.));
#24611=DIRECTION('center_axis',(0.,0.,1.));
#24612=DIRECTION('ref_axis',(-1.,3.65562114876707E-13,0.));
#24613=DIRECTION('',(-1.22464679914735E-16,4.47534497895031E-29,1.));
#24614=DIRECTION('center_axis',(0.,0.,1.));
#24615=DIRECTION('ref_axis',(-1.,3.65562114876707E-13,0.));
#24616=DIRECTION('',(-1.22464679914735E-16,4.47534497895031E-29,1.));
#24617=DIRECTION('center_axis',(0.,0.,1.));
#24618=DIRECTION('ref_axis',(-1.,3.65562114876707E-13,0.));
#24619=DIRECTION('',(-1.22464679914735E-16,4.47534497895031E-29,1.));
#24620=DIRECTION('center_axis',(0.,0.,1.));
#24621=DIRECTION('ref_axis',(-1.,3.65562114876707E-13,0.));
#24622=DIRECTION('',(-1.22464679914735E-16,4.47534497895031E-29,1.));
#24623=DIRECTION('center_axis',(0.,0.,1.));
#24624=DIRECTION('ref_axis',(-1.,3.65562114876707E-13,0.));
#24625=DIRECTION('',(-1.22464679914735E-16,4.47534497895031E-29,1.));
#24626=DIRECTION('center_axis',(0.,0.,1.));
#24627=DIRECTION('ref_axis',(-1.,3.65562114876707E-13,0.));
#24628=DIRECTION('',(-1.22464679914735E-16,4.47534497895031E-29,1.));
#24629=DIRECTION('center_axis',(0.,0.,1.));
#24630=DIRECTION('ref_axis',(0.608777863132373,-0.793340729674193,0.));
#24631=DIRECTION('',(-1.22464679914735E-16,4.47534497895031E-29,1.));
#24632=DIRECTION('center_axis',(0.,0.,1.));
#24633=DIRECTION('ref_axis',(-1.,3.65562114876707E-13,0.));
#24634=DIRECTION('center_axis',(0.,0.,1.));
#24635=DIRECTION('ref_axis',(1.,0.,0.));
#24636=DIRECTION('center_axis',(0.,0.,1.));
#24637=DIRECTION('ref_axis',(-1.,3.65562114876707E-13,0.));
#24638=DIRECTION('center_axis',(0.,0.,1.));
#24639=DIRECTION('ref_axis',(-1.,0.,0.));
#24640=DIRECTION('center_axis',(0.,0.,1.));
#24641=DIRECTION('ref_axis',(-1.,0.,0.));
#24642=DIRECTION('center_axis',(0.,0.,-1.));
#24643=DIRECTION('ref_axis',(1.,0.,0.));
#24644=DIRECTION('center_axis',(0.,0.,1.));
#24645=DIRECTION('ref_axis',(1.,0.,0.));
#24646=DIRECTION('center_axis',(0.,0.,-1.));
#24647=DIRECTION('ref_axis',(1.,3.16070290694603E-14,0.));
#24648=DIRECTION('center_axis',(0.,0.,-1.));
#24649=DIRECTION('ref_axis',(1.,0.,0.));
#24650=DIRECTION('center_axis',(0.,0.,-1.));
#24651=DIRECTION('ref_axis',(1.,0.,0.));
#24652=DIRECTION('center_axis',(0.,0.,1.));
#24653=DIRECTION('ref_axis',(1.,0.,0.));
#24654=DIRECTION('center_axis',(0.,0.,1.));
#24655=DIRECTION('ref_axis',(0.707106781186548,-0.707106781186547,0.));
#24656=DIRECTION('center_axis',(0.,0.,-1.));
#24657=DIRECTION('ref_axis',(0.707106781186548,-0.707106781186547,0.));
#24658=DIRECTION('',(0.,0.,-1.));
#24659=DIRECTION('center_axis',(0.,0.,1.));
#24660=DIRECTION('ref_axis',(0.707106781186548,-0.707106781186547,0.));
#24661=DIRECTION('',(0.,0.,1.));
#24662=DIRECTION('center_axis',(0.,-1.,0.));
#24663=DIRECTION('ref_axis',(1.,0.,0.));
#24664=DIRECTION('',(1.,0.,0.));
#24665=DIRECTION('',(0.,0.,1.));
#24666=DIRECTION('',(-1.,0.,0.));
#24667=DIRECTION('center_axis',(0.,0.,1.));
#24668=DIRECTION('ref_axis',(1.,0.,0.));
#24669=DIRECTION('',(0.,1.,0.));
#24670=DIRECTION('center_axis',(0.,0.,1.));
#24671=DIRECTION('ref_axis',(-0.707106781186548,0.707106781186547,0.));
#24672=DIRECTION('',(1.,0.,0.));
#24673=DIRECTION('center_axis',(0.,0.,1.));
#24674=DIRECTION('ref_axis',(0.707106781186547,0.707106781186548,0.));
#24675=DIRECTION('',(0.,-1.,0.));
#24676=DIRECTION('center_axis',(0.,0.,1.));
#24677=DIRECTION('ref_axis',(0.707106781186548,-0.707106781186548,0.));
#24678=DIRECTION('',(-1.,0.,0.));
#24679=DIRECTION('center_axis',(0.,0.,1.));
#24680=DIRECTION('ref_axis',(-0.707106781186548,-0.707106781186548,0.));
#24681=DIRECTION('',(0.,1.,0.));
#24682=DIRECTION('center_axis',(0.,0.,-1.));
#24683=DIRECTION('ref_axis',(0.707106781186548,0.707106781186547,0.));
#24684=DIRECTION('',(-1.,0.,0.));
#24685=DIRECTION('center_axis',(0.,0.,-1.));
#24686=DIRECTION('ref_axis',(-0.707106781186548,0.707106781186547,0.));
#24687=DIRECTION('',(0.,-1.,0.));
#24688=DIRECTION('center_axis',(0.,0.,-1.));
#24689=DIRECTION('ref_axis',(-0.707106781186548,-0.707106781186548,0.));
#24690=DIRECTION('',(1.,0.,0.));
#24691=DIRECTION('center_axis',(0.,0.,-1.));
#24692=DIRECTION('ref_axis',(0.707106781186547,-0.707106781186548,0.));
#24693=DIRECTION('',(0.,1.,0.));
#24694=DIRECTION('center_axis',(0.,0.,-1.));
#24695=DIRECTION('ref_axis',(0.707106781186547,0.707106781186548,0.));
#24696=DIRECTION('',(-1.,0.,0.));
#24697=DIRECTION('center_axis',(0.,0.,1.));
#24698=DIRECTION('ref_axis',(-0.707106781186547,-0.707106781186548,0.));
#24699=DIRECTION('',(0.,1.,0.));
#24700=DIRECTION('center_axis',(0.,0.,1.));
#24701=DIRECTION('ref_axis',(-0.707106781186548,0.707106781186547,0.));
#24702=DIRECTION('',(1.,0.,0.));
#24703=DIRECTION('center_axis',(0.,0.,1.));
#24704=DIRECTION('ref_axis',(0.707106781186548,0.707106781186548,0.));
#24705=DIRECTION('',(0.,-1.,0.));
#24706=DIRECTION('center_axis',(0.,0.,1.));
#24707=DIRECTION('ref_axis',(0.707106781186548,-0.707106781186548,0.));
#24708=DIRECTION('',(-1.,0.,0.));
#24709=DIRECTION('center_axis',(0.,0.,-1.));
#24710=DIRECTION('ref_axis',(-0.707106781186547,0.707106781186548,0.));
#24711=DIRECTION('',(0.,-1.,0.));
#24712=DIRECTION('center_axis',(0.,0.,-1.));
#24713=DIRECTION('ref_axis',(-0.707106781186547,-0.707106781186548,0.));
#24714=DIRECTION('',(1.,0.,0.));
#24715=DIRECTION('center_axis',(0.,0.,-1.));
#24716=DIRECTION('ref_axis',(0.707106781186548,-0.707106781186548,0.));
#24717=DIRECTION('',(0.,1.,0.));
#24718=DIRECTION('center_axis',(0.,0.,-1.));
#24719=DIRECTION('ref_axis',(0.707106781186548,0.707106781186547,0.));
#24720=DIRECTION('',(-1.,0.,0.));
#24721=DIRECTION('center_axis',(0.,0.,-1.));
#24722=DIRECTION('ref_axis',(-0.707106781186548,0.707106781186547,0.));
#24723=DIRECTION('',(0.,-1.,0.));
#24724=DIRECTION('center_axis',(0.,0.,1.));
#24725=DIRECTION('ref_axis',(0.707106781186548,-0.707106781186547,0.));
#24726=DIRECTION('',(-1.,0.,0.));
#24727=DIRECTION('center_axis',(0.,0.,1.));
#24728=DIRECTION('ref_axis',(-0.707106781186547,-0.707106781186548,0.));
#24729=DIRECTION('',(0.,1.,0.));
#24730=DIRECTION('center_axis',(0.,0.,1.));
#24731=DIRECTION('ref_axis',(-0.707106781186548,0.707106781186548,0.));
#24732=DIRECTION('',(1.,0.,0.));
#24733=DIRECTION('center_axis',(0.,0.,1.));
#24734=DIRECTION('ref_axis',(0.707106781186548,0.707106781186548,0.));
#24735=DIRECTION('',(0.,-1.,0.));
#24736=DIRECTION('center_axis',(0.,0.,-1.));
#24737=DIRECTION('ref_axis',(-0.707106781186548,-0.707106781186547,0.));
#24738=DIRECTION('',(1.,0.,0.));
#24739=DIRECTION('center_axis',(0.,0.,-1.));
#24740=DIRECTION('ref_axis',(0.707106781186548,-0.707106781186547,0.));
#24741=DIRECTION('',(0.,1.,0.));
#24742=DIRECTION('center_axis',(0.,0.,-1.));
#24743=DIRECTION('ref_axis',(0.707106781186548,0.707106781186548,0.));
#24744=DIRECTION('',(-1.,0.,0.));
#24745=DIRECTION('center_axis',(0.,0.,-1.));
#24746=DIRECTION('ref_axis',(-0.707106781186547,0.707106781186548,0.));
#24747=DIRECTION('',(0.,-1.,0.));
#24748=DIRECTION('center_axis',(0.,0.,-1.));
#24749=DIRECTION('ref_axis',(-0.707106781186547,-0.707106781186548,0.));
#24750=DIRECTION('',(1.,0.,0.));
#24751=DIRECTION('center_axis',(0.,0.,1.));
#24752=DIRECTION('ref_axis',(0.707106781186547,0.707106781186548,0.));
#24753=DIRECTION('',(0.,-1.,0.));
#24754=DIRECTION('center_axis',(0.,0.,1.));
#24755=DIRECTION('ref_axis',(0.707106781186548,-0.707106781186547,0.));
#24756=DIRECTION('',(-1.,0.,0.));
#24757=DIRECTION('center_axis',(0.,0.,1.));
#24758=DIRECTION('ref_axis',(-0.707106781186548,-0.707106781186548,0.));
#24759=DIRECTION('',(0.,1.,0.));
#24760=DIRECTION('center_axis',(0.,0.,1.));
#24761=DIRECTION('ref_axis',(-0.707106781186548,0.707106781186548,0.));
#24762=DIRECTION('',(1.,0.,0.));
#24763=DIRECTION('center_axis',(0.,0.,-1.));
#24764=DIRECTION('ref_axis',(0.707106781186547,-0.707106781186548,0.));
#24765=DIRECTION('',(0.,1.,0.));
#24766=DIRECTION('center_axis',(0.,0.,-1.));
#24767=DIRECTION('ref_axis',(0.707106781186547,0.707106781186548,0.));
#24768=DIRECTION('',(-1.,0.,0.));
#24769=DIRECTION('center_axis',(0.,0.,-1.));
#24770=DIRECTION('ref_axis',(-0.707106781186548,0.707106781186548,0.));
#24771=DIRECTION('',(0.,-1.,0.));
#24772=DIRECTION('center_axis',(0.,0.,-1.));
#24773=DIRECTION('ref_axis',(-0.707106781186548,-0.707106781186547,0.));
#24774=DIRECTION('center_axis',(0.,0.,-1.));
#24775=DIRECTION('ref_axis',(1.,0.,0.));
#24776=DIRECTION('center_axis',(0.,0.,-1.));
#24777=DIRECTION('ref_axis',(1.,0.,0.));
#24778=DIRECTION('center_axis',(0.,0.,-1.));
#24779=DIRECTION('ref_axis',(1.,0.,0.));
#24780=DIRECTION('center_axis',(0.,0.,-1.));
#24781=DIRECTION('ref_axis',(1.,0.,0.));
#24782=DIRECTION('center_axis',(0.,0.,1.));
#24783=DIRECTION('ref_axis',(-0.707106781186548,0.707106781186547,0.));
#24784=DIRECTION('center_axis',(0.,0.,-1.));
#24785=DIRECTION('ref_axis',(-0.707106781186548,0.707106781186547,0.));
#24786=DIRECTION('',(0.,0.,1.));
#24787=DIRECTION('',(0.,0.,-1.));
#24788=DIRECTION('center_axis',(0.,-1.,0.));
#24789=DIRECTION('ref_axis',(1.,0.,0.));
#24790=DIRECTION('',(-1.,0.,0.));
#24791=DIRECTION('',(0.,0.,-1.));
#24792=DIRECTION('center_axis',(0.,0.,1.));
#24793=DIRECTION('ref_axis',(0.707106781186547,0.707106781186548,0.));
#24794=DIRECTION('center_axis',(0.,0.,-1.));
#24795=DIRECTION('ref_axis',(0.707106781186547,0.707106781186548,0.));
#24796=DIRECTION('',(0.,0.,1.));
#24797=DIRECTION('center_axis',(-1.,0.,0.));
#24798=DIRECTION('ref_axis',(0.,-1.,0.));
#24799=DIRECTION('',(0.,1.,0.));
#24800=DIRECTION('',(0.,0.,-1.));
#24801=DIRECTION('center_axis',(0.,0.,1.));
#24802=DIRECTION('ref_axis',(0.707106781186548,-0.707106781186548,0.));
#24803=DIRECTION('center_axis',(0.,0.,-1.));
#24804=DIRECTION('ref_axis',(0.707106781186548,-0.707106781186548,0.));
#24805=DIRECTION('',(0.,0.,1.));
#24806=DIRECTION('center_axis',(0.,1.,0.));
#24807=DIRECTION('ref_axis',(-1.,0.,0.));
#24808=DIRECTION('',(1.,0.,0.));
#24809=DIRECTION('',(0.,0.,-1.));
#24810=DIRECTION('center_axis',(0.,0.,1.));
#24811=DIRECTION('ref_axis',(-0.707106781186548,-0.707106781186548,0.));
#24812=DIRECTION('center_axis',(0.,0.,-1.));
#24813=DIRECTION('ref_axis',(-0.707106781186548,-0.707106781186548,0.));
#24814=DIRECTION('',(0.,0.,1.));
#24815=DIRECTION('center_axis',(1.,0.,0.));
#24816=DIRECTION('ref_axis',(0.,1.,0.));
#24817=DIRECTION('',(0.,-1.,0.));
#24818=DIRECTION('',(0.,0.,-1.));
#24819=DIRECTION('center_axis',(0.,0.,1.));
#24820=DIRECTION('ref_axis',(0.707106781186548,0.707106781186547,0.));
#24821=DIRECTION('center_axis',(0.,0.,1.));
#24822=DIRECTION('ref_axis',(0.707106781186548,0.707106781186547,0.));
#24823=DIRECTION('',(0.,0.,1.));
#24824=DIRECTION('center_axis',(0.,0.,1.));
#24825=DIRECTION('ref_axis',(-0.707106781186548,0.707106781186547,0.));
#24826=DIRECTION('',(0.,0.,-1.));
#24827=DIRECTION('center_axis',(0.,0.,1.));
#24828=DIRECTION('ref_axis',(-0.707106781186548,0.707106781186547,0.));
#24829=DIRECTION('',(0.,0.,1.));
#24830=DIRECTION('center_axis',(-1.,0.,0.));
#24831=DIRECTION('ref_axis',(0.,-1.,0.));
#24832=DIRECTION('',(0.,1.,0.));
#24833=DIRECTION('',(0.,0.,-1.));
#24834=DIRECTION('center_axis',(0.,0.,1.));
#24835=DIRECTION('ref_axis',(-0.707106781186548,-0.707106781186548,0.));
#24836=DIRECTION('center_axis',(0.,0.,1.));
#24837=DIRECTION('ref_axis',(-0.707106781186548,-0.707106781186548,0.));
#24838=DIRECTION('',(0.,0.,1.));
#24839=DIRECTION('center_axis',(0.,0.,1.));
#24840=DIRECTION('ref_axis',(0.707106781186547,-0.707106781186548,0.));
#24841=DIRECTION('',(0.,0.,-1.));
#24842=DIRECTION('center_axis',(0.,0.,1.));
#24843=DIRECTION('ref_axis',(0.707106781186547,-0.707106781186548,0.));
#24844=DIRECTION('',(0.,0.,1.));
#24845=DIRECTION('center_axis',(1.,0.,0.));
#24846=DIRECTION('ref_axis',(0.,1.,0.));
#24847=DIRECTION('',(0.,-1.,0.));
#24848=DIRECTION('',(0.,0.,-1.));
#24849=DIRECTION('center_axis',(0.,0.,1.));
#24850=DIRECTION('ref_axis',(0.707106781186547,0.707106781186548,0.));
#24851=DIRECTION('center_axis',(0.,0.,1.));
#24852=DIRECTION('ref_axis',(0.707106781186547,0.707106781186548,0.));
#24853=DIRECTION('',(0.,0.,1.));
#24854=DIRECTION('center_axis',(0.,0.,1.));
#24855=DIRECTION('ref_axis',(-0.707106781186547,-0.707106781186548,0.));
#24856=DIRECTION('center_axis',(0.,0.,-1.));
#24857=DIRECTION('ref_axis',(-0.707106781186547,-0.707106781186548,0.));
#24858=DIRECTION('',(0.,0.,1.));
#24859=DIRECTION('',(0.,0.,-1.));
#24860=DIRECTION('center_axis',(1.,0.,0.));
#24861=DIRECTION('ref_axis',(0.,1.,0.));
#24862=DIRECTION('',(0.,-1.,0.));
#24863=DIRECTION('',(0.,0.,-1.));
#24864=DIRECTION('center_axis',(0.,0.,1.));
#24865=DIRECTION('ref_axis',(-0.707106781186548,0.707106781186547,0.));
#24866=DIRECTION('center_axis',(0.,0.,-1.));
#24867=DIRECTION('ref_axis',(-0.707106781186548,0.707106781186547,0.));
#24868=DIRECTION('',(0.,0.,1.));
#24869=DIRECTION('center_axis',(0.,-1.,0.));
#24870=DIRECTION('ref_axis',(1.,0.,0.));
#24871=DIRECTION('',(-1.,0.,0.));
#24872=DIRECTION('',(0.,0.,-1.));
#24873=DIRECTION('center_axis',(0.,0.,1.));
#24874=DIRECTION('ref_axis',(0.707106781186548,0.707106781186548,0.));
#24875=DIRECTION('center_axis',(0.,0.,-1.));
#24876=DIRECTION('ref_axis',(0.707106781186548,0.707106781186548,0.));
#24877=DIRECTION('',(0.,0.,1.));
#24878=DIRECTION('center_axis',(-1.,0.,0.));
#24879=DIRECTION('ref_axis',(0.,-1.,0.));
#24880=DIRECTION('',(0.,1.,0.));
#24881=DIRECTION('',(0.,0.,-1.));
#24882=DIRECTION('center_axis',(0.,0.,1.));
#24883=DIRECTION('ref_axis',(0.707106781186548,-0.707106781186548,0.));
#24884=DIRECTION('center_axis',(0.,0.,-1.));
#24885=DIRECTION('ref_axis',(0.707106781186548,-0.707106781186548,0.));
#24886=DIRECTION('',(0.,0.,1.));
#24887=DIRECTION('center_axis',(0.,1.,0.));
#24888=DIRECTION('ref_axis',(-1.,0.,0.));
#24889=DIRECTION('',(1.,0.,0.));
#24890=DIRECTION('',(0.,0.,-1.));
#24891=DIRECTION('center_axis',(0.,0.,1.));
#24892=DIRECTION('ref_axis',(-0.707106781186547,0.707106781186548,0.));
#24893=DIRECTION('center_axis',(0.,0.,1.));
#24894=DIRECTION('ref_axis',(-0.707106781186547,0.707106781186548,0.));
#24895=DIRECTION('',(0.,0.,1.));
#24896=DIRECTION('center_axis',(0.,0.,1.));
#24897=DIRECTION('ref_axis',(-0.707106781186547,-0.707106781186548,0.));
#24898=DIRECTION('',(0.,0.,-1.));
#24899=DIRECTION('center_axis',(0.,0.,1.));
#24900=DIRECTION('ref_axis',(-0.707106781186547,-0.707106781186548,0.));
#24901=DIRECTION('',(0.,0.,1.));
#24902=DIRECTION('center_axis',(0.,-1.,0.));
#24903=DIRECTION('ref_axis',(1.,0.,0.));
#24904=DIRECTION('',(-1.,0.,0.));
#24905=DIRECTION('',(0.,0.,-1.));
#24906=DIRECTION('center_axis',(0.,0.,1.));
#24907=DIRECTION('ref_axis',(0.707106781186548,-0.707106781186548,0.));
#24908=DIRECTION('center_axis',(0.,0.,1.));
#24909=DIRECTION('ref_axis',(0.707106781186548,-0.707106781186548,0.));
#24910=DIRECTION('',(0.,0.,1.));
#24911=DIRECTION('center_axis',(0.,0.,1.));
#24912=DIRECTION('ref_axis',(0.707106781186548,0.707106781186547,0.));
#24913=DIRECTION('',(0.,0.,-1.));
#24914=DIRECTION('center_axis',(0.,0.,1.));
#24915=DIRECTION('ref_axis',(0.707106781186548,0.707106781186547,0.));
#24916=DIRECTION('',(0.,0.,1.));
#24917=DIRECTION('center_axis',(0.,1.,0.));
#24918=DIRECTION('ref_axis',(-1.,0.,0.));
#24919=DIRECTION('',(1.,0.,0.));
#24920=DIRECTION('',(0.,0.,-1.));
#24921=DIRECTION('center_axis',(0.,0.,1.));
#24922=DIRECTION('ref_axis',(-0.707106781186548,0.707106781186547,0.));
#24923=DIRECTION('center_axis',(0.,0.,1.));
#24924=DIRECTION('ref_axis',(-0.707106781186548,0.707106781186547,0.));
#24925=DIRECTION('',(0.,0.,1.));
#24926=DIRECTION('center_axis',(0.,0.,1.));
#24927=DIRECTION('ref_axis',(0.707106781186548,-0.707106781186547,0.));
#24928=DIRECTION('center_axis',(0.,0.,-1.));
#24929=DIRECTION('ref_axis',(0.707106781186548,-0.707106781186547,0.));
#24930=DIRECTION('',(0.,0.,1.));
#24931=DIRECTION('',(0.,0.,-1.));
#24932=DIRECTION('center_axis',(0.,1.,0.));
#24933=DIRECTION('ref_axis',(-1.,0.,0.));
#24934=DIRECTION('',(1.,0.,0.));
#24935=DIRECTION('',(0.,0.,-1.));
#24936=DIRECTION('center_axis',(0.,0.,1.));
#24937=DIRECTION('ref_axis',(-0.707106781186547,-0.707106781186548,0.));
#24938=DIRECTION('center_axis',(0.,0.,-1.));
#24939=DIRECTION('ref_axis',(-0.707106781186547,-0.707106781186548,0.));
#24940=DIRECTION('',(0.,0.,1.));
#24941=DIRECTION('center_axis',(1.,0.,0.));
#24942=DIRECTION('ref_axis',(0.,1.,0.));
#24943=DIRECTION('',(0.,-1.,0.));
#24944=DIRECTION('',(0.,0.,-1.));
#24945=DIRECTION('center_axis',(0.,0.,1.));
#24946=DIRECTION('ref_axis',(-0.707106781186548,0.707106781186548,0.));
#24947=DIRECTION('center_axis',(0.,0.,-1.));
#24948=DIRECTION('ref_axis',(-0.707106781186548,0.707106781186548,0.));
#24949=DIRECTION('',(0.,0.,1.));
#24950=DIRECTION('center_axis',(0.,-1.,0.));
#24951=DIRECTION('ref_axis',(1.,0.,0.));
#24952=DIRECTION('',(-1.,0.,0.));
#24953=DIRECTION('',(0.,0.,-1.));
#24954=DIRECTION('center_axis',(0.,0.,1.));
#24955=DIRECTION('ref_axis',(0.707106781186548,0.707106781186548,0.));
#24956=DIRECTION('center_axis',(0.,0.,-1.));
#24957=DIRECTION('ref_axis',(0.707106781186548,0.707106781186548,0.));
#24958=DIRECTION('',(0.,0.,1.));
#24959=DIRECTION('center_axis',(-1.,0.,0.));
#24960=DIRECTION('ref_axis',(0.,-1.,0.));
#24961=DIRECTION('',(0.,1.,0.));
#24962=DIRECTION('',(0.,0.,-1.));
#24963=DIRECTION('center_axis',(0.,0.,1.));
#24964=DIRECTION('ref_axis',(-0.707106781186548,-0.707106781186547,0.));
#24965=DIRECTION('center_axis',(0.,0.,1.));
#24966=DIRECTION('ref_axis',(-0.707106781186548,-0.707106781186547,0.));
#24967=DIRECTION('',(0.,0.,1.));
#24968=DIRECTION('center_axis',(0.,0.,1.));
#24969=DIRECTION('ref_axis',(0.707106781186548,-0.707106781186547,0.));
#24970=DIRECTION('',(0.,0.,-1.));
#24971=DIRECTION('center_axis',(0.,0.,1.));
#24972=DIRECTION('ref_axis',(0.707106781186548,-0.707106781186547,0.));
#24973=DIRECTION('',(0.,0.,1.));
#24974=DIRECTION('center_axis',(1.,0.,0.));
#24975=DIRECTION('ref_axis',(0.,1.,0.));
#24976=DIRECTION('',(0.,-1.,0.));
#24977=DIRECTION('',(0.,0.,-1.));
#24978=DIRECTION('center_axis',(0.,0.,1.));
#24979=DIRECTION('ref_axis',(0.707106781186548,0.707106781186548,0.));
#24980=DIRECTION('center_axis',(0.,0.,1.));
#24981=DIRECTION('ref_axis',(0.707106781186548,0.707106781186548,0.));
#24982=DIRECTION('',(0.,0.,1.));
#24983=DIRECTION('center_axis',(0.,0.,1.));
#24984=DIRECTION('ref_axis',(-0.707106781186547,0.707106781186548,0.));
#24985=DIRECTION('',(0.,0.,-1.));
#24986=DIRECTION('center_axis',(0.,0.,1.));
#24987=DIRECTION('ref_axis',(-0.707106781186547,0.707106781186548,0.));
#24988=DIRECTION('',(0.,0.,1.));
#24989=DIRECTION('center_axis',(-1.,0.,0.));
#24990=DIRECTION('ref_axis',(0.,-1.,0.));
#24991=DIRECTION('',(0.,1.,0.));
#24992=DIRECTION('',(0.,0.,-1.));
#24993=DIRECTION('center_axis',(0.,0.,1.));
#24994=DIRECTION('ref_axis',(-0.707106781186547,-0.707106781186548,0.));
#24995=DIRECTION('center_axis',(0.,0.,1.));
#24996=DIRECTION('ref_axis',(-0.707106781186547,-0.707106781186548,0.));
#24997=DIRECTION('',(0.,0.,1.));
#24998=DIRECTION('center_axis',(0.,0.,1.));
#24999=DIRECTION('ref_axis',(0.707106781186547,0.707106781186548,0.));
#25000=DIRECTION('center_axis',(0.,0.,-1.));
#25001=DIRECTION('ref_axis',(0.707106781186547,0.707106781186548,0.));
#25002=DIRECTION('',(0.,0.,1.));
#25003=DIRECTION('',(0.,0.,-1.));
#25004=DIRECTION('center_axis',(-1.,0.,0.));
#25005=DIRECTION('ref_axis',(0.,-1.,0.));
#25006=DIRECTION('',(0.,1.,0.));
#25007=DIRECTION('',(0.,0.,-1.));
#25008=DIRECTION('center_axis',(0.,0.,1.));
#25009=DIRECTION('ref_axis',(0.707106781186548,-0.707106781186547,0.));
#25010=DIRECTION('center_axis',(0.,0.,-1.));
#25011=DIRECTION('ref_axis',(0.707106781186548,-0.707106781186547,0.));
#25012=DIRECTION('',(0.,0.,1.));
#25013=DIRECTION('center_axis',(0.,1.,0.));
#25014=DIRECTION('ref_axis',(-1.,0.,0.));
#25015=DIRECTION('',(1.,0.,0.));
#25016=DIRECTION('',(0.,0.,-1.));
#25017=DIRECTION('center_axis',(0.,0.,1.));
#25018=DIRECTION('ref_axis',(-0.707106781186548,-0.707106781186548,0.));
#25019=DIRECTION('center_axis',(0.,0.,-1.));
#25020=DIRECTION('ref_axis',(-0.707106781186548,-0.707106781186548,0.));
#25021=DIRECTION('',(0.,0.,1.));
#25022=DIRECTION('center_axis',(1.,0.,0.));
#25023=DIRECTION('ref_axis',(0.,1.,0.));
#25024=DIRECTION('',(0.,-1.,0.));
#25025=DIRECTION('',(0.,0.,-1.));
#25026=DIRECTION('center_axis',(0.,0.,1.));
#25027=DIRECTION('ref_axis',(-0.707106781186548,0.707106781186548,0.));
#25028=DIRECTION('center_axis',(0.,0.,-1.));
#25029=DIRECTION('ref_axis',(-0.707106781186548,0.707106781186548,0.));
#25030=DIRECTION('',(0.,0.,1.));
#25031=DIRECTION('center_axis',(0.,-1.,0.));
#25032=DIRECTION('ref_axis',(1.,0.,0.));
#25033=DIRECTION('',(-1.,0.,0.));
#25034=DIRECTION('',(0.,0.,-1.));
#25035=DIRECTION('center_axis',(0.,0.,1.));
#25036=DIRECTION('ref_axis',(0.707106781186547,-0.707106781186548,0.));
#25037=DIRECTION('center_axis',(0.,0.,1.));
#25038=DIRECTION('ref_axis',(0.707106781186547,-0.707106781186548,0.));
#25039=DIRECTION('',(0.,0.,1.));
#25040=DIRECTION('center_axis',(0.,0.,1.));
#25041=DIRECTION('ref_axis',(0.707106781186547,0.707106781186548,0.));
#25042=DIRECTION('',(0.,0.,-1.));
#25043=DIRECTION('center_axis',(0.,0.,1.));
#25044=DIRECTION('ref_axis',(0.707106781186547,0.707106781186548,0.));
#25045=DIRECTION('',(0.,0.,1.));
#25046=DIRECTION('center_axis',(0.,1.,0.));
#25047=DIRECTION('ref_axis',(-1.,0.,0.));
#25048=DIRECTION('',(1.,0.,0.));
#25049=DIRECTION('',(0.,0.,-1.));
#25050=DIRECTION('center_axis',(0.,0.,1.));
#25051=DIRECTION('ref_axis',(-0.707106781186548,0.707106781186548,0.));
#25052=DIRECTION('center_axis',(0.,0.,1.));
#25053=DIRECTION('ref_axis',(-0.707106781186548,0.707106781186548,0.));
#25054=DIRECTION('',(0.,0.,1.));
#25055=DIRECTION('center_axis',(0.,0.,1.));
#25056=DIRECTION('ref_axis',(-0.707106781186548,-0.707106781186547,0.));
#25057=DIRECTION('',(0.,0.,-1.));
#25058=DIRECTION('center_axis',(0.,0.,1.));
#25059=DIRECTION('ref_axis',(-0.707106781186548,-0.707106781186547,0.));
#25060=DIRECTION('center_axis',(0.,0.,1.));
#25061=DIRECTION('ref_axis',(1.,0.,0.));
#25062=DIRECTION('',(0.,0.,-1.));
#25063=DIRECTION('center_axis',(0.,0.,-1.));
#25064=DIRECTION('ref_axis',(1.,0.,0.));
#25065=DIRECTION('center_axis',(0.,0.,1.));
#25066=DIRECTION('ref_axis',(1.,0.,0.));
#25067=DIRECTION('',(0.,0.,-1.));
#25068=DIRECTION('center_axis',(0.,0.,-1.));
#25069=DIRECTION('ref_axis',(1.,0.,0.));
#25070=DIRECTION('center_axis',(0.,0.,1.));
#25071=DIRECTION('ref_axis',(1.,0.,0.));
#25072=DIRECTION('',(0.,0.,-1.));
#25073=DIRECTION('center_axis',(0.,0.,1.));
#25074=DIRECTION('ref_axis',(1.,0.,0.));
#25075=DIRECTION('',(0.,0.,-1.));
#25076=DIRECTION('center_axis',(0.,0.,-1.));
#25077=DIRECTION('ref_axis',(1.,0.,0.));
#25078=DIRECTION('center_axis',(0.,0.,1.));
#25079=DIRECTION('ref_axis',(1.,0.,0.));
#25080=DIRECTION('',(0.,0.,-1.));
#25081=DIRECTION('center_axis',(0.,0.,-1.));
#25082=DIRECTION('ref_axis',(1.,0.,0.));
#25083=DIRECTION('center_axis',(-1.,0.,0.));
#25084=DIRECTION('ref_axis',(0.,-1.,0.));
#25085=DIRECTION('',(0.,1.,0.));
#25086=DIRECTION('center_axis',(1.,0.,0.));
#25087=DIRECTION('ref_axis',(0.,1.,0.));
#25088=DIRECTION('',(0.,-1.,0.));
#25089=DIRECTION('center_axis',(0.,-1.,0.));
#25090=DIRECTION('ref_axis',(1.,0.,0.));
#25091=DIRECTION('',(-1.,0.,0.));
#25092=DIRECTION('center_axis',(0.,1.,0.));
#25093=DIRECTION('ref_axis',(-1.,0.,0.));
#25094=DIRECTION('',(1.,0.,0.));
#25095=DIRECTION('center_axis',(0.,-1.,0.));
#25096=DIRECTION('ref_axis',(1.,0.,0.));
#25097=DIRECTION('',(-1.,0.,0.));
#25098=DIRECTION('center_axis',(-1.,0.,0.));
#25099=DIRECTION('ref_axis',(0.,-1.,0.));
#25100=DIRECTION('',(0.,1.,0.));
#25101=DIRECTION('center_axis',(1.,0.,0.));
#25102=DIRECTION('ref_axis',(0.,1.,0.));
#25103=DIRECTION('',(0.,-1.,0.));
#25104=DIRECTION('center_axis',(-1.,0.,0.));
#25105=DIRECTION('ref_axis',(0.,-1.,0.));
#25106=DIRECTION('',(0.,1.,0.));
#25107=DIRECTION('center_axis',(0.,1.,0.));
#25108=DIRECTION('ref_axis',(-1.,0.,0.));
#25109=DIRECTION('',(1.,0.,0.));
#25110=DIRECTION('center_axis',(0.,-1.,0.));
#25111=DIRECTION('ref_axis',(1.,0.,0.));
#25112=DIRECTION('',(-1.,0.,0.));
#25113=DIRECTION('center_axis',(0.,1.,0.));
#25114=DIRECTION('ref_axis',(-1.,0.,0.));
#25115=DIRECTION('',(1.,0.,0.));
#25116=DIRECTION('center_axis',(1.,0.,0.));
#25117=DIRECTION('ref_axis',(0.,1.,0.));
#25118=DIRECTION('',(0.,-1.,0.));
#25119=DIRECTION('center_axis',(0.,0.,1.));
#25120=DIRECTION('ref_axis',(1.,0.,0.));
#37339=CARTESIAN_POINT('',(0.,0.,0.));
#37340=CARTESIAN_POINT('Origin',(0.,0.,387.));
#37341=CARTESIAN_POINT('',(-4.51811257745934,-3.71096681342671E-5,375.387416697508));
#37342=CARTESIAN_POINT('',(-4.51738402494857,7.56118822245166E-5,375.112583302492));
#37343=CARTESIAN_POINT('',(-4.51775,5.53264807684796E-16,387.));
#37344=CARTESIAN_POINT('',(-3.43378788736318,2.93584158412846,375.));
#37345=CARTESIAN_POINT('Ctrl Pts',(-4.51738402494857,7.56118822245166E-5,
375.112583302492));
#37346=CARTESIAN_POINT('Ctrl Pts',(-4.51750331650906,0.316697913039608,
375.101431493481));
#37347=CARTESIAN_POINT('Ctrl Pts',(-4.4846735281982,0.633280120229468,375.09027968447));
#37348=CARTESIAN_POINT('Ctrl Pts',(-4.41862189351514,0.942742403897512,
375.07912787546));
#37349=CARTESIAN_POINT('Ctrl Pts',(-4.26239834514751,1.67467426709133,375.052751916973));
#37350=CARTESIAN_POINT('Ctrl Pts',(-3.92033033613571,2.36677696691102,375.026375958487));
#37351=CARTESIAN_POINT('Ctrl Pts',(-3.43378788736318,2.93584158412846,375.));
#37352=CARTESIAN_POINT('',(-4.51775,5.53264807684796E-16,375.));
#37353=CARTESIAN_POINT('Origin',(0.,0.,375.));
#37354=CARTESIAN_POINT('',(-4.51775,-5.53264807684796E-16,374.));
#37355=CARTESIAN_POINT('',(-4.51775,5.53264807684796E-16,387.));
#37356=CARTESIAN_POINT('Origin',(0.,0.,374.));
#37357=CARTESIAN_POINT('',(3.43408816985915,2.93604417002329,375.));
#37358=CARTESIAN_POINT('Origin',(0.,0.,375.));
#37359=CARTESIAN_POINT('Ctrl Pts',(3.43408816985915,2.93604417002329,375.));
#37360=CARTESIAN_POINT('Ctrl Pts',(2.97450239048794,3.47304931219374,375.024906410057));
#37361=CARTESIAN_POINT('Ctrl Pts',(2.38685944123298,3.90077491345638,375.049812820113));
#37362=CARTESIAN_POINT('Ctrl Pts',(1.73419289985632,4.17206490566361,375.07471923017));
#37363=CARTESIAN_POINT('Ctrl Pts',(1.04301719200363,4.45936177245515,375.101095188656));
#37364=CARTESIAN_POINT('Ctrl Pts',(0.278918372660684,4.57121814160633,375.127471147143));
#37365=CARTESIAN_POINT('Ctrl Pts',(-0.465602633695269,4.49408396451439,
375.153847105629));
#37366=CARTESIAN_POINT('Ctrl Pts',(-1.21012364005122,4.41694978742245,375.180223064116));
#37367=CARTESIAN_POINT('Ctrl Pts',(-1.93506683342019,4.15082506408738,375.206599022603));
#37368=CARTESIAN_POINT('Ctrl Pts',(-2.55266299064051,3.7279323762134,375.232974981089));
#37369=CARTESIAN_POINT('Ctrl Pts',(-3.17025914786083,3.30503968833942,375.259350939576));
#37370=CARTESIAN_POINT('Ctrl Pts',(-3.68050826893252,2.72537903592653,375.285726898063));
#37371=CARTESIAN_POINT('Ctrl Pts',(-4.02163754569994,2.05912619262106,375.312102856549));
#37372=CARTESIAN_POINT('Ctrl Pts',(-4.346324085653,1.4249873333691,375.337207470202));
#37373=CARTESIAN_POINT('Ctrl Pts',(-4.51780131678173,0.712402743689628,
375.362312083855));
#37374=CARTESIAN_POINT('Ctrl Pts',(-4.51811257745934,-3.71096681342671E-5,
375.387416697508));
#37375=CARTESIAN_POINT('Origin',(0.,0.,387.));
#37376=CARTESIAN_POINT('',(-4.51742232703027,-5.89235854892012E-5,376.387416697508));
#37377=CARTESIAN_POINT('',(-4.51809885152616,4.59828434581654E-5,376.112583302492));
#37378=CARTESIAN_POINT('',(-4.51775,5.53264807684796E-16,387.));
#37379=CARTESIAN_POINT('Ctrl Pts',(-4.51809885152616,4.59828434581654E-5,
376.112583302492));
#37380=CARTESIAN_POINT('Ctrl Pts',(-4.51812276106344,0.0453867389231147,
376.110985620474));
#37381=CARTESIAN_POINT('Ctrl Pts',(-4.51745435602182,0.090726788718723,
376.109387938455));
#37382=CARTESIAN_POINT('Ctrl Pts',(-4.51608913278767,0.136045847103087,
376.107790256437));
#37383=CARTESIAN_POINT('Ctrl Pts',(-4.49355081105947,0.884213247670103,
376.08141429795));
#37384=CARTESIAN_POINT('Ctrl Pts',(-4.28109923000243,1.62665957583979,376.055038339464));
#37385=CARTESIAN_POINT('Ctrl Pts',(-3.90445518421615,2.27349934356334,376.028662380977));
#37386=CARTESIAN_POINT('Ctrl Pts',(-3.52781113842983,2.92033911128693,376.002286422491));
#37387=CARTESIAN_POINT('Ctrl Pts',(-2.98697462791424,3.47157231856439,375.975910464004));
#37388=CARTESIAN_POINT('Ctrl Pts',(-2.3474228959368,3.86046307951571,375.949534505517));
#37389=CARTESIAN_POINT('Ctrl Pts',(-1.70787116395944,4.24935384046699,375.923158547031));
#37390=CARTESIAN_POINT('Ctrl Pts',(-0.969604210520236,4.47590215509218,
375.896782588544));
#37391=CARTESIAN_POINT('Ctrl Pts',(-0.222001520476049,4.51268047531198,
375.870406630058));
#37392=CARTESIAN_POINT('Ctrl Pts',(0.525601169568224,4.54945879553177,375.844030671571));
#37393=CARTESIAN_POINT('Ctrl Pts',(1.28253959621751,4.39646712134613,375.817654713084));
#37394=CARTESIAN_POINT('Ctrl Pts',(1.95717379585807,4.07222787085974,375.791278754598));
#37395=CARTESIAN_POINT('Ctrl Pts',(2.63180799549863,3.74798862037335,375.764902796111));
#37396=CARTESIAN_POINT('Ctrl Pts',(3.2241379681305,3.25250179358621,375.738526837624));
#37397=CARTESIAN_POINT('Ctrl Pts',(3.66245231025333,2.64575380780901,375.712150879138));
#37398=CARTESIAN_POINT('Ctrl Pts',(4.10076665237614,2.03900582203184,375.685774920651));
#37399=CARTESIAN_POINT('Ctrl Pts',(4.38506536398996,1.3209966772646,375.659398962165));
#37400=CARTESIAN_POINT('Ctrl Pts',(4.48092940302618,0.578654357786939,375.633023003678));
#37401=CARTESIAN_POINT('Ctrl Pts',(4.57679344206242,-0.163687961690764,
375.606647045192));
#37402=CARTESIAN_POINT('Ctrl Pts',(4.48422280852107,-0.930363455878798,
375.580271086705));
#37403=CARTESIAN_POINT('Ctrl Pts',(4.21442463026058,-1.62855553605874,375.553895128218));
#37404=CARTESIAN_POINT('Ctrl Pts',(3.9446264520001,-2.32674761623864,375.527519169732));
#37405=CARTESIAN_POINT('Ctrl Pts',(3.49760072902049,-2.95645628241037,375.501143211245));
#37406=CARTESIAN_POINT('Ctrl Pts',(2.92746753425598,-3.44144014717816,375.474767252759));
#37407=CARTESIAN_POINT('Ctrl Pts',(2.35733433949146,-3.92642401194595,375.448391294272));
#37408=CARTESIAN_POINT('Ctrl Pts',(1.66409367294202,-4.26668307530983,375.422015335785));
#37409=CARTESIAN_POINT('Ctrl Pts',(0.931673460847324,-4.42103326145621,
375.395639377299));
#37410=CARTESIAN_POINT('Ctrl Pts',(0.199253248752631,-4.57538344760259,
375.369263418812));
#37411=CARTESIAN_POINT('Ctrl Pts',(-0.572346508887337,-4.54382475653147,
375.342887460326));
#37412=CARTESIAN_POINT('Ctrl Pts',(-1.28970997066769,-4.33015694226547,
375.316511501839));
#37413=CARTESIAN_POINT('Ctrl Pts',(-2.00707343244804,-4.11648912799948,
375.290135543353));
#37414=CARTESIAN_POINT('Ctrl Pts',(-2.67020059836879,-3.72071219053859,
375.263759584866));
#37415=CARTESIAN_POINT('Ctrl Pts',(-3.19881015683584,-3.19078643170059,
375.237383626379));
#37416=CARTESIAN_POINT('Ctrl Pts',(-3.72741971530293,-2.66086067286256,
375.211007667893));
#37417=CARTESIAN_POINT('Ctrl Pts',(-4.12151166631632,-1.99678609264739,
375.184631709406));
#37418=CARTESIAN_POINT('Ctrl Pts',(-4.33336809796127,-1.27886828925581,
375.158255750919));
#37419=CARTESIAN_POINT('Ctrl Pts',(-4.45565119847602,-0.864487596482785,
375.143031601444));
#37420=CARTESIAN_POINT('Ctrl Pts',(-4.51722117132128,-0.432168630785926,
375.127807451968));
#37421=CARTESIAN_POINT('Ctrl Pts',(-4.51738402494857,7.56118822245166E-5,
375.112583302492));
#37422=CARTESIAN_POINT('Ctrl Pts',(-4.51811257745934,-3.71096681342671E-5,
375.387416697508));
#37423=CARTESIAN_POINT('Ctrl Pts',(-4.51812834028524,-0.0361164032740072,
375.388688042342));
#37424=CARTESIAN_POINT('Ctrl Pts',(-4.51770513086054,-0.072195325689107,
375.389959387175));
#37425=CARTESIAN_POINT('Ctrl Pts',(-4.51684061704284,-0.108263669884894,
375.391230732009));
#37426=CARTESIAN_POINT('Ctrl Pts',(-4.49890497915514,-0.856555654887204,
375.417606690495));
#37427=CARTESIAN_POINT('Ctrl Pts',(-4.29102427091659,-1.60029459069377,
375.443982648982));
#37428=CARTESIAN_POINT('Ctrl Pts',(-3.91836620190419,-2.24943891961304,
375.470358607469));
#37429=CARTESIAN_POINT('Ctrl Pts',(-3.54570813289175,-2.89858324853235,
375.496734565955));
#37430=CARTESIAN_POINT('Ctrl Pts',(-3.00827270310544,-3.45313297056435,
375.523110524442));
#37431=CARTESIAN_POINT('Ctrl Pts',(-2.37112526060116,-3.84595044058964,
375.549486482929));
#37432=CARTESIAN_POINT('Ctrl Pts',(-1.73397781809692,-4.2387679106149,375.575862441415));
#37433=CARTESIAN_POINT('Ctrl Pts',(-0.997118362874728,-4.46985312863346,
375.602238399902));
#37434=CARTESIAN_POINT('Ctrl Pts',(-0.249756040595646,-4.5112294783827,
375.628614358388));
#37435=CARTESIAN_POINT('Ctrl Pts',(0.497606281683436,-4.55260582813195,
375.654990316875));
#37436=CARTESIAN_POINT('Ctrl Pts',(1.25547147101941,-4.40427330961188,375.681366275361));
#37437=CARTESIAN_POINT('Ctrl Pts',(1.93208738599618,-4.08418999671804,375.707742233848));
#37438=CARTESIAN_POINT('Ctrl Pts',(2.60870330097296,-3.76410668382419,375.734118192335));
#37439=CARTESIAN_POINT('Ctrl Pts',(3.20406994159053,-3.27227257655657,375.760494150821));
#37440=CARTESIAN_POINT('Ctrl Pts',(3.64610826956487,-2.66823238495421,375.786870109308));
#37441=CARTESIAN_POINT('Ctrl Pts',(4.0881465975392,-2.06419219335185,375.813246067794));
#37442=CARTESIAN_POINT('Ctrl Pts',(4.37685661287028,-1.34794591741475,375.839622026281));
#37443=CARTESIAN_POINT('Ctrl Pts',(4.47728517843054,-0.606207059497561,
375.865997984767));
#37444=CARTESIAN_POINT('Ctrl Pts',(4.57771374399081,0.135531798419669,375.892373943254));
#37445=CARTESIAN_POINT('Ctrl Pts',(4.48986085978024,0.902763238316989,375.918749901741));
#37446=CARTESIAN_POINT('Ctrl Pts',(4.22436257375966,1.6026011428634,375.945125860228));
#37447=CARTESIAN_POINT('Ctrl Pts',(3.95886428773907,2.30243904740981,375.971501818714));
#37448=CARTESIAN_POINT('Ctrl Pts',(3.51572059990846,2.93488341660531,375.9978777772));
#37449=CARTESIAN_POINT('Ctrl Pts',(2.9485814178138,3.42336635395337,376.024253735687));
#37450=CARTESIAN_POINT('Ctrl Pts',(2.38144223571922,3.91184929130138,376.050629694174));
#37451=CARTESIAN_POINT('Ctrl Pts',(1.69030755936062,4.25637079680199,376.07700565266));
#37452=CARTESIAN_POINT('Ctrl Pts',(0.958850723376994,4.41522081720076,376.103381611147));
#37453=CARTESIAN_POINT('Ctrl Pts',(0.227393887393287,4.57407083759954,376.129757569634));
#37454=CARTESIAN_POINT('Ctrl Pts',(-0.544385108215453,4.54724937289643,
376.15613352812));
#37455=CARTESIAN_POINT('Ctrl Pts',(-1.26304959302181,4.33800360748393,376.182509486607));
#37456=CARTESIAN_POINT('Ctrl Pts',(-1.98171407782812,4.12875784207144,376.208885445093));
#37457=CARTESIAN_POINT('Ctrl Pts',(-2.64726405183205,3.73708777594958,376.23526140358));
#37458=CARTESIAN_POINT('Ctrl Pts',(-3.17912363311765,3.21041157777291,376.261637362067));
#37459=CARTESIAN_POINT('Ctrl Pts',(-3.71098321440328,2.68373537959622,376.288013320553));
#37460=CARTESIAN_POINT('Ctrl Pts',(-4.10915240297055,2.0220530493647,376.31438927904));
#37461=CARTESIAN_POINT('Ctrl Pts',(-4.32542620311525,1.30547222672582,376.340765237526));
#37462=CARTESIAN_POINT('Ctrl Pts',(-4.45293485255022,0.882997322948535,
376.356315724187));
#37463=CARTESIAN_POINT('Ctrl Pts',(-4.51721787315074,0.44144006785591,376.371866210847));
#37464=CARTESIAN_POINT('Ctrl Pts',(-4.51742232703027,-5.89235854892012E-5,
376.387416697508));
#37465=CARTESIAN_POINT('Origin',(0.,0.,387.));
#37466=CARTESIAN_POINT('',(-4.51776278108284,0.000115059314115817,377.387416697508));
#37467=CARTESIAN_POINT('',(-4.51759690135649,-0.00010734614409786,377.112583302492));
#37468=CARTESIAN_POINT('',(-4.51775,5.53264807684796E-16,387.));
#37469=CARTESIAN_POINT('Ctrl Pts',(-4.51759690135649,-0.00010734614409786,
377.112583302492));
#37470=CARTESIAN_POINT('Ctrl Pts',(-4.51713109747156,0.522789201244633,
377.094163788979));
#37471=CARTESIAN_POINT('Ctrl Pts',(-4.42639959069602,1.04584321668838,377.075744275467));
#37472=CARTESIAN_POINT('Ctrl Pts',(-4.24853722021895,1.53736821094173,377.057324761954));
#37473=CARTESIAN_POINT('Ctrl Pts',(-3.99384588448772,2.24121105862155,377.030948803468));
#37474=CARTESIAN_POINT('Ctrl Pts',(-3.56049254147675,2.88040358637871,377.004572844981));
#37475=CARTESIAN_POINT('Ctrl Pts',(-3.00094181327236,3.37756091891157,376.978196886494));
#37476=CARTESIAN_POINT('Ctrl Pts',(-2.44139108506791,3.87471825144449,376.951820928008));
#37477=CARTESIAN_POINT('Ctrl Pts',(-1.75564297167002,4.22984038875309,376.925444969521));
#37478=CARTESIAN_POINT('Ctrl Pts',(-1.02671867551292,4.39993389597404,376.899069011035));
#37479=CARTESIAN_POINT('Ctrl Pts',(-0.297794379355856,4.57002740319499,
376.872693052548));
#37480=CARTESIAN_POINT('Ctrl Pts',(0.474306099560417,4.55509228032832,376.846317094061));
#37481=CARTESIAN_POINT('Ctrl Pts',(1.19610717026038,4.35693667212173,376.819941135575));
#37482=CARTESIAN_POINT('Ctrl Pts',(1.91790824096034,4.15878106391514,376.793565177088));
#37483=CARTESIAN_POINT('Ctrl Pts',(2.58940990344398,3.77740497036863,376.767189218602));
#37484=CARTESIAN_POINT('Ctrl Pts',(3.12931572485767,3.25898030397792,376.740813260115));
#37485=CARTESIAN_POINT('Ctrl Pts',(3.66922154627136,2.74055563758721,376.714437301628));
#37486=CARTESIAN_POINT('Ctrl Pts',(4.07753152661508,2.0850823983523,376.688061343142));
#37487=CARTESIAN_POINT('Ctrl Pts',(4.30481295893208,1.37191651212926,376.661685384655));
#37488=CARTESIAN_POINT('Ctrl Pts',(4.53209439124908,0.658750625906209,376.635309426169));
#37489=CARTESIAN_POINT('Ctrl Pts',(4.57834727553935,-0.112107907304984,
376.608933467682));
#37490=CARTESIAN_POINT('Ctrl Pts',(4.4379719316997,-0.847333854561028,376.582557509196));
#37491=CARTESIAN_POINT('Ctrl Pts',(4.29759658786004,-1.58255980181707,376.556181550709));
#37492=CARTESIAN_POINT('Ctrl Pts',(3.97059301589046,-2.28215316311797,376.529805592222));
#37493=CARTESIAN_POINT('Ctrl Pts',(3.49655043114217,-2.86141653901512,376.503429633736));
#37494=CARTESIAN_POINT('Ctrl Pts',(3.02250784639385,-3.4406799149123,376.477053675249));
#37495=CARTESIAN_POINT('Ctrl Pts',(2.40142624886681,-3.89961330540572,376.450677716762));
#37496=CARTESIAN_POINT('Ctrl Pts',(1.7084978848751,-4.18265519808121,376.424301758276));
#37497=CARTESIAN_POINT('Ctrl Pts',(1.01556952088344,-4.46569709075668,376.397925799789));
#37498=CARTESIAN_POINT('Ctrl Pts',(0.250794390427128,-4.57284748561423,
376.371549841303));
#37499=CARTESIAN_POINT('Ctrl Pts',(-0.493238770703864,-4.4911340483472,
376.345173882816));
#37500=CARTESIAN_POINT('Ctrl Pts',(-1.2372719318349,-4.40942061108017,376.31879792433));
#37501=CARTESIAN_POINT('Ctrl Pts',(-1.96056312364061,-4.13884334168854,
376.292421965843));
#37502=CARTESIAN_POINT('Ctrl Pts',(-2.5755459301882,-3.71216011150867,376.266046007356));
#37503=CARTESIAN_POINT('Ctrl Pts',(-3.19052873673575,-3.28547688132881,
376.23967004887));
#37504=CARTESIAN_POINT('Ctrl Pts',(-3.69720315802519,-2.70268769036073,
376.213294090383));
#37505=CARTESIAN_POINT('Ctrl Pts',(-4.03422783747023,-2.03434885839451,
376.186918131897));
#37506=CARTESIAN_POINT('Ctrl Pts',(-4.350837779367,-1.40649359537751,376.162139855428));
#37507=CARTESIAN_POINT('Ctrl Pts',(-4.51772804111577,-0.703138866533066,
376.13736157896));
#37508=CARTESIAN_POINT('Ctrl Pts',(-4.51809885152616,4.59828434581654E-5,
376.112583302492));
#37509=CARTESIAN_POINT('Ctrl Pts',(-4.51742232703027,-5.89235854892012E-5,
376.387416697508));
#37510=CARTESIAN_POINT('Ctrl Pts',(-4.51756465760558,-0.307408461731671,
376.398242169334));
#37511=CARTESIAN_POINT('Ctrl Pts',(-4.48665292107515,-0.614729763863418,
376.40906764116));
#37512=CARTESIAN_POINT('Ctrl Pts',(-4.42439936040209,-0.915565329693696,
376.419893112986));
#37513=CARTESIAN_POINT('Ctrl Pts',(-4.27272030582208,-1.64854274842831,
376.446269071473));
#37514=CARTESIAN_POINT('Ctrl Pts',(-3.9349837849399,-2.34301827085134,376.472645029959));
#37515=CARTESIAN_POINT('Ctrl Pts',(-3.45207841488762,-2.91491409664169,
376.499020988446));
#37516=CARTESIAN_POINT('Ctrl Pts',(-2.96917304483534,-3.48680992243204,
376.525396946932));
#37517=CARTESIAN_POINT('Ctrl Pts',(-2.34109882561295,-3.93612605158971,
376.551772905419));
#37518=CARTESIAN_POINT('Ctrl Pts',(-1.64389457655484,-4.20846530156397,
376.578148863906));
#37519=CARTESIAN_POINT('Ctrl Pts',(-0.946690327496738,-4.48080455153823,
376.604524822392));
#37520=CARTESIAN_POINT('Ctrl Pts',(-0.180356048602913,-4.57616692232909,
376.630900780879));
#37521=CARTESIAN_POINT('Ctrl Pts',(0.562330763470305,-4.48300721455655,
376.657276739365));
#37522=CARTESIAN_POINT('Ctrl Pts',(1.30501757554357,-4.38984750678402,376.683652697852));
#37523=CARTESIAN_POINT('Ctrl Pts',(2.02405692079622,-4.10816572044807,376.710028656339));
#37524=CARTESIAN_POINT('Ctrl Pts',(2.6323971400614,-3.67206411576684,376.736404614825));
#37525=CARTESIAN_POINT('Ctrl Pts',(3.24073735932655,-3.23596251108564,376.762780573312));
#37526=CARTESIAN_POINT('Ctrl Pts',(3.73837845260424,-2.64544108805917,376.789156531798));
#37527=CARTESIAN_POINT('Ctrl Pts',(4.0650726975356,-1.97199227611499,376.815532490285));
#37528=CARTESIAN_POINT('Ctrl Pts',(4.39176694246694,-1.29854346417084,376.841908448771));
#37529=CARTESIAN_POINT('Ctrl Pts',(4.54751433905197,-0.542167263308996,
376.868284407258));
#37530=CARTESIAN_POINT('Ctrl Pts',(4.51345907728089,0.205564420603285,376.894660365745));
#37531=CARTESIAN_POINT('Ctrl Pts',(4.4794038155098,0.953296104515694,376.921036324231));
#37532=CARTESIAN_POINT('Ctrl Pts',(4.25554589538254,1.69238327147853,376.947412282718));
#37533=CARTESIAN_POINT('Ctrl Pts',(3.86898703740037,2.33334714042606,376.973788241204));
#37534=CARTESIAN_POINT('Ctrl Pts',(3.48242817941824,2.97431100937351,377.000164199691));
#37535=CARTESIAN_POINT('Ctrl Pts',(2.93316838358124,3.51715158030568,377.026540158178));
#37536=CARTESIAN_POINT('Ctrl Pts',(2.28770467380867,3.89614898312949,377.052916116664));
#37537=CARTESIAN_POINT('Ctrl Pts',(1.6422409640361,4.27514638595329,377.079292075151));
#37538=CARTESIAN_POINT('Ctrl Pts',(0.900573340327957,4.49030062066872,377.105668033637));
#37539=CARTESIAN_POINT('Ctrl Pts',(0.152492990912077,4.51556369250058,377.132043992124));
#37540=CARTESIAN_POINT('Ctrl Pts',(-0.595587358503804,4.54082676433243,
377.158419950611));
#37541=CARTESIAN_POINT('Ctrl Pts',(-1.35008043362742,4.3761986732807,377.184795909097));
#37542=CARTESIAN_POINT('Ctrl Pts',(-2.01964231224972,4.04161038496754,377.211171867584));
#37543=CARTESIAN_POINT('Ctrl Pts',(-2.68920419087202,3.70702209665437,377.23754782607));
#37544=CARTESIAN_POINT('Ctrl Pts',(-3.27383487299299,3.20247361107977,377.263923784557));
#37545=CARTESIAN_POINT('Ctrl Pts',(-3.70275510124179,2.58904890520336,377.290299743043));
#37546=CARTESIAN_POINT('Ctrl Pts',(-4.13167532949061,1.97562419932691,377.31667570153));
#37547=CARTESIAN_POINT('Ctrl Pts',(-4.40488510386723,1.25332327314864,377.343051660017));
#37548=CARTESIAN_POINT('Ctrl Pts',(-4.48930784196123,0.509592654393879,
377.369427618503));
#37549=CARTESIAN_POINT('Ctrl Pts',(-4.50850066492699,0.340511546362542,
377.375423978172));
#37550=CARTESIAN_POINT('Ctrl Pts',(-4.51793615737842,0.170322859138234,
377.38142033784));
#37551=CARTESIAN_POINT('Ctrl Pts',(-4.51776278108284,0.000115059314115817,
377.387416697508));
#37552=CARTESIAN_POINT('Origin',(0.,0.,387.));
#37553=CARTESIAN_POINT('',(-4.51797310231548,-9.04168125550817E-5,378.387416697508));
#37554=CARTESIAN_POINT('',(-4.51753028950122,9.61292306860575E-5,378.112583302492));
#37555=CARTESIAN_POINT('',(-4.51775,5.53264807684796E-16,387.));
#37556=CARTESIAN_POINT('Ctrl Pts',(-4.51753028950122,9.61292306860575E-5,
378.112583302492));
#37557=CARTESIAN_POINT('Ctrl Pts',(-4.51772668562278,0.251779003793691,
378.103717915972));
#37558=CARTESIAN_POINT('Ctrl Pts',(-4.49704602585537,0.503429942291254,
378.094852529451));
#37559=CARTESIAN_POINT('Ctrl Pts',(-4.4551993669653,0.751510564258943,378.085987142931));
#37560=CARTESIAN_POINT('Ctrl Pts',(-4.33069878989798,1.48959053081815,378.059611184445));
#37561=CARTESIAN_POINT('Ctrl Pts',(-4.01884552637064,2.19606752935734,378.033235225958));
#37562=CARTESIAN_POINT('Ctrl Pts',(-3.55739459519457,2.78541078149727,378.006859267472));
#37563=CARTESIAN_POINT('Ctrl Pts',(-3.09594366401851,3.3747540336372,377.980483308985));
#37564=CARTESIAN_POINT('Ctrl Pts',(-2.48489506519372,3.84696353937788,377.954107350499));
#37565=CARTESIAN_POINT('Ctrl Pts',(-1.79822638382644,4.14487049256201,377.927731392012));
#37566=CARTESIAN_POINT('Ctrl Pts',(-1.11155770245912,4.44277744574616,377.901355433525));
#37567=CARTESIAN_POINT('Ctrl Pts',(-0.349268938549303,4.56638184637374,
377.874979475039));
#37568=CARTESIAN_POINT('Ctrl Pts',(0.396352188045507,4.50071932813326,377.848603516552));
#37569=CARTESIAN_POINT('Ctrl Pts',(1.14197331464023,4.43505680989279,377.822227558065));
#37570=CARTESIAN_POINT('Ctrl Pts',(1.87092680391995,4.18012737278432,377.795851599579));
#37571=CARTESIAN_POINT('Ctrl Pts',(2.49496072486742,3.76679446067473,377.769475641092));
#37572=CARTESIAN_POINT('Ctrl Pts',(3.11899464581496,3.35346154856509,377.743099682606));
#37573=CARTESIAN_POINT('Ctrl Pts',(3.63810899843023,2.7817251614543,377.716723724119));
#37574=CARTESIAN_POINT('Ctrl Pts',(3.98945636554489,2.120803488071,377.690347765632));
#37575=CARTESIAN_POINT('Ctrl Pts',(4.34080373265956,1.45988181468769,377.663971807146));
#37576=CARTESIAN_POINT('Ctrl Pts',(4.52438411427362,0.709774855031875,377.637595848659));
#37577=CARTESIAN_POINT('Ctrl Pts',(4.517972055111,-0.0387044808375217,377.611219890173));
#37578=CARTESIAN_POINT('Ctrl Pts',(4.51155999594838,-0.787183816706875,
377.584843931686));
#37579=CARTESIAN_POINT('Ctrl Pts',(4.3151554960091,-1.53403552878981,377.558467973199));
#37580=CARTESIAN_POINT('Ctrl Pts',(3.9525365831578,-2.18884080883012,377.532092014713));
#37581=CARTESIAN_POINT('Ctrl Pts',(3.5899176703065,-2.84364608887043,377.505716056226));
#37582=CARTESIAN_POINT('Ctrl Pts',(3.06108434454318,-3.40640493686811,377.47934009774));
#37583=CARTESIAN_POINT('Ctrl Pts',(2.43006066621085,-3.80898604436084,377.452964139253));
#37584=CARTESIAN_POINT('Ctrl Pts',(1.79903698787851,-4.21156715185356,377.426588180766));
#37585=CARTESIAN_POINT('Ctrl Pts',(1.06582295697716,-4.45397051884133,377.40021222228));
#37586=CARTESIAN_POINT('Ctrl Pts',(0.319186313873781,-4.50684919035867,
377.373836263793));
#37587=CARTESIAN_POINT('Ctrl Pts',(-0.427450329229602,-4.55972786187601,
377.347460305307));
#37588=CARTESIAN_POINT('Ctrl Pts',(-1.18750958453502,-4.42308183792293,
377.32108434682));
#37589=CARTESIAN_POINT('Ctrl Pts',(-1.86897365124353,-4.11345438999364,
377.294708388334));
#37590=CARTESIAN_POINT('Ctrl Pts',(-2.55043771795204,-3.80382694206434,
377.268332429847));
#37591=CARTESIAN_POINT('Ctrl Pts',(-3.15330659606364,-3.32121807015883,
377.24195647136));
#37592=CARTESIAN_POINT('Ctrl Pts',(-3.60459299156575,-2.72405559648777,
377.215580512874));
#37593=CARTESIAN_POINT('Ctrl Pts',(-4.05587938706785,-2.1268931228167,377.189204554387));
#37594=CARTESIAN_POINT('Ctrl Pts',(-4.35558329996046,-1.41517704738009,
377.162828595901));
#37595=CARTESIAN_POINT('Ctrl Pts',(-4.46742059218106,-0.675072425860511,
377.136452637414));
#37596=CARTESIAN_POINT('Ctrl Pts',(-4.50115689268563,-0.451816019874252,
377.12849619244));
#37597=CARTESIAN_POINT('Ctrl Pts',(-4.51779810878667,-0.225976373769842,
377.120539747466));
#37598=CARTESIAN_POINT('Ctrl Pts',(-4.51759690135649,-0.00010734614409786,
377.112583302492));
#37599=CARTESIAN_POINT('Ctrl Pts',(-4.51776278108284,0.000115059314115817,
377.387416697508));
#37600=CARTESIAN_POINT('Ctrl Pts',(-4.51717353368206,-0.578363695817441,
377.407796296326));
#37601=CARTESIAN_POINT('Ctrl Pts',(-4.40559318176197,-1.15706321872293,
377.428175895145));
#37602=CARTESIAN_POINT('Ctrl Pts',(-4.18884997964351,-1.69325291121775,
377.448555493963));
#37603=CARTESIAN_POINT('Ctrl Pts',(-3.90833367742039,-2.38720754674346,
377.47493145245));
#37604=CARTESIAN_POINT('Ctrl Pts',(-3.45166537116277,-3.0099565064637,377.501307410936));
#37605=CARTESIAN_POINT('Ctrl Pts',(-2.87413234662247,-3.48610568219112,
377.527683369423));
#37606=CARTESIAN_POINT('Ctrl Pts',(-2.29659932208215,-3.96225485791856,
377.55405932791));
#37607=CARTESIAN_POINT('Ctrl Pts',(-1.59820157925914,-4.29180424965317,
377.580435286396));
#37608=CARTESIAN_POINT('Ctrl Pts',(-0.863491768396101,-4.43485642825323,
377.606811244883));
#37609=CARTESIAN_POINT('Ctrl Pts',(-0.128781957533104,-4.57790860685328,
377.633187203369));
#37610=CARTESIAN_POINT('Ctrl Pts',(0.642239921369918,-4.5344635723188,377.659563161856));
#37611=CARTESIAN_POINT('Ctrl Pts',(1.35622885978989,-4.30978106789426,377.685939120342));
#37612=CARTESIAN_POINT('Ctrl Pts',(2.07021779820986,-4.08509856346973,377.712315078829));
#37613=CARTESIAN_POINT('Ctrl Pts',(2.72717379614679,-3.67917858915515,377.738691037316));
#37614=CARTESIAN_POINT('Ctrl Pts',(3.24756141510707,-3.14116450196653,377.765066995802));
#37615=CARTESIAN_POINT('Ctrl Pts',(3.76794903406735,-2.6031504147779,377.791442954289));
#37616=CARTESIAN_POINT('Ctrl Pts',(4.15176827405098,-1.93304221471522,377.817818912776));
#37617=CARTESIAN_POINT('Ctrl Pts',(4.35255143912362,-1.21196763285564,377.844194871262));
#37618=CARTESIAN_POINT('Ctrl Pts',(4.55333460419626,-0.49089305099606,377.870570829749));
#37619=CARTESIAN_POINT('Ctrl Pts',(4.57108169435792,0.28114791266043,377.896946788235));
#37620=CARTESIAN_POINT('Ctrl Pts',(4.40364412948689,1.01068687244984,377.923322746722));
#37621=CARTESIAN_POINT('Ctrl Pts',(4.23620656461585,1.7402258322393,377.949698705208));
#37622=CARTESIAN_POINT('Ctrl Pts',(3.88358434471212,2.42726278816168,377.976074663695));
#37623=CARTESIAN_POINT('Ctrl Pts',(3.38846824810894,2.98862050198153,378.002450622182));
#37624=CARTESIAN_POINT('Ctrl Pts',(2.89335215150579,3.54997821580136,378.028826580668));
#37625=CARTESIAN_POINT('Ctrl Pts',(2.25574217820322,3.98565668751868,378.055202539155));
#37626=CARTESIAN_POINT('Ctrl Pts',(1.55283160898984,4.2429097995867,378.081578497641));
#37627=CARTESIAN_POINT('Ctrl Pts',(0.849921039776497,4.5001629116547,378.107954456128));
#37628=CARTESIAN_POINT('Ctrl Pts',(0.0817098746523573,4.57899066407343,
378.134330414615));
#37629=CARTESIAN_POINT('Ctrl Pts',(-0.658797161460833,4.46984964773514,
378.160706373101));
#37630=CARTESIAN_POINT('Ctrl Pts',(-1.39930419757415,4.36070863139684,378.187082331588));
#37631=CARTESIAN_POINT('Ctrl Pts',(-2.11210710467651,4.06359884630146,378.213458290074));
#37632=CARTESIAN_POINT('Ctrl Pts',(-2.71090924805577,3.61449036824177,378.239834248561));
#37633=CARTESIAN_POINT('Ctrl Pts',(-3.309711391435,3.16538189018211,378.266210207048));
#37634=CARTESIAN_POINT('Ctrl Pts',(-3.79451277109115,2.56427471915816,378.292586165534));
#37635=CARTESIAN_POINT('Ctrl Pts',(-4.10662012532275,1.8839428652698,378.318962124021));
#37636=CARTESIAN_POINT('Ctrl Pts',(-4.37662833282249,1.29537876422316,378.341780315183));
#37637=CARTESIAN_POINT('Ctrl Pts',(-4.5173887163544,0.647521251956349,378.364598506346));
#37638=CARTESIAN_POINT('Ctrl Pts',(-4.51797310231548,-9.04168125550817E-5,
378.387416697508));
#37639=CARTESIAN_POINT('Origin',(0.,0.,387.));
#37640=CARTESIAN_POINT('',(-4.51737365644452,-1.98811769755447E-6,379.387416697508));
#37641=CARTESIAN_POINT('',(-4.51813007169143,-2.03714566067892E-5,379.112583302492));
#37642=CARTESIAN_POINT('',(-4.51775,5.53264807684796E-16,387.));
#37643=CARTESIAN_POINT('Ctrl Pts',(-4.51813007169143,-2.03714566067892E-5,
379.112583302492));
#37644=CARTESIAN_POINT('Ctrl Pts',(-4.517945231463,0.728944748987095,379.086896084477));
#37645=CARTESIAN_POINT('Ctrl Pts',(-4.33810981632971,1.45799779441603,379.061208866463));
#37646=CARTESIAN_POINT('Ctrl Pts',(-3.99878265125311,2.10316590777759,379.035521648449));
#37647=CARTESIAN_POINT('Ctrl Pts',(-3.65035725094643,2.76563263988363,379.009145689962));
#37648=CARTESIAN_POINT('Ctrl Pts',(-3.13377267064052,3.33965579170571,378.982769731476));
#37649=CARTESIAN_POINT('Ctrl Pts',(-2.51157005653494,3.75574032365363,378.956393772989));
#37650=CARTESIAN_POINT('Ctrl Pts',(-1.88936744242933,4.17182485560157,378.930017814502));
#37651=CARTESIAN_POINT('Ctrl Pts',(-1.16154679452404,4.42997076767533,378.903641856016));
#37652=CARTESIAN_POINT('Ctrl Pts',(-0.416222894566461,4.49892520827358,
378.877265897529));
#37653=CARTESIAN_POINT('Ctrl Pts',(0.329101005391076,4.56787964887184,378.850889939042));
#37654=CARTESIAN_POINT('Ctrl Pts',(1.0919281574009,4.44764261799461,378.824513980556));
#37655=CARTESIAN_POINT('Ctrl Pts',(1.779905660781,4.15277080589822,378.798138022069));
#37656=CARTESIAN_POINT('Ctrl Pts',(2.46788316416111,3.85789899380182,378.771762063583));
#37657=CARTESIAN_POINT('Ctrl Pts',(3.08101101891148,3.38839240048625,378.745386105096));
#37658=CARTESIAN_POINT('Ctrl Pts',(3.54505991145048,2.80109259965241,378.71901014661));
#37659=CARTESIAN_POINT('Ctrl Pts',(4.00910880398948,2.21379279881858,378.692634188123));
#37660=CARTESIAN_POINT('Ctrl Pts',(4.3240787343171,1.50869979046648,378.666258229636));
#37661=CARTESIAN_POINT('Ctrl Pts',(4.45183735932425,0.771176797969019,378.63988227115));
#37662=CARTESIAN_POINT('Ctrl Pts',(4.57959598433139,0.0336538054715552,
378.613506312663));
#37663=CARTESIAN_POINT('Ctrl Pts',(4.52014330401807,-0.736299171171277,
378.587130354177));
#37664=CARTESIAN_POINT('Ctrl Pts',(4.28067705310806,-1.44546653181419,378.56075439569));
#37665=CARTESIAN_POINT('Ctrl Pts',(4.04121080219804,-2.1546338924571,378.534378437203));
#37666=CARTESIAN_POINT('Ctrl Pts',(3.62173098069132,-2.80301563710009,378.508002478717));
#37667=CARTESIAN_POINT('Ctrl Pts',(3.07302259039553,-3.31211438306704,378.48162652023));
#37668=CARTESIAN_POINT('Ctrl Pts',(2.5243142000997,-3.82121312903403,378.455250561744));
#37669=CARTESIAN_POINT('Ctrl Pts',(1.84637724101477,-4.19102887632496,378.428874603257));
#37670=CARTESIAN_POINT('Ctrl Pts',(1.12128724556784,-4.37678928445587,378.40249864477));
#37671=CARTESIAN_POINT('Ctrl Pts',(0.396197250120947,-4.56254969258676,
378.376122686284));
#37672=CARTESIAN_POINT('Ctrl Pts',(-0.37604578168795,-4.56425476155764,
378.349746727797));
#37673=CARTESIAN_POINT('Ctrl Pts',(-1.10194900048777,-4.38169806444086,
378.323370769311));
#37674=CARTESIAN_POINT('Ctrl Pts',(-1.82785221928764,-4.19914136732407,
378.296994810824));
#37675=CARTESIAN_POINT('Ctrl Pts',(-2.50741562507842,-3.83232290411959,
378.270618852338));
#37676=CARTESIAN_POINT('Ctrl Pts',(-3.05836677703682,-3.32565214427459,
378.244242893851));
#37677=CARTESIAN_POINT('Ctrl Pts',(-3.60931792899519,-2.81898138442963,
378.217866935364));
#37678=CARTESIAN_POINT('Ctrl Pts',(-4.0316568271212,-2.17245832794416,378.191490976878));
#37679=CARTESIAN_POINT('Ctrl Pts',(-4.27425233088056,-1.46435533241182,
378.165115018391));
#37680=CARTESIAN_POINT('Ctrl Pts',(-4.435307559621,-0.99425721373283,378.147604446425));
#37681=CARTESIAN_POINT('Ctrl Pts',(-4.51714237540265,-0.497018246743604,
378.130093874458));
#37682=CARTESIAN_POINT('Ctrl Pts',(-4.51753028950122,9.61292306860575E-5,
378.112583302492));
#37683=CARTESIAN_POINT('Ctrl Pts',(-4.51797310231548,-9.04168125550817E-5,
378.387416697508));
#37684=CARTESIAN_POINT('Ctrl Pts',(-4.51806421862098,-0.101064749856769,
378.390974464832));
#37685=CARTESIAN_POINT('Ctrl Pts',(-4.51474759603089,-0.202033106339626,
378.394532232156));
#37686=CARTESIAN_POINT('Ctrl Pts',(-4.50798181202017,-0.302769806622464,
378.398089999481));
#37687=CARTESIAN_POINT('Ctrl Pts',(-4.45782281567894,-1.04959408787382,
378.424465957967));
#37688=CARTESIAN_POINT('Ctrl Pts',(-4.2180914941894,-1.78368611362381,378.450841916454));
#37689=CARTESIAN_POINT('Ctrl Pts',(-3.81781130701489,-2.41617184764166,
378.47721787494));
#37690=CARTESIAN_POINT('Ctrl Pts',(-3.41753111984037,-3.04865758165951,
378.503593833427));
#37691=CARTESIAN_POINT('Ctrl Pts',(-2.85670206698089,-3.57953702394521,
378.529969791913));
#37692=CARTESIAN_POINT('Ctrl Pts',(-2.20322182313489,-3.94453839775569,
378.5563457504));
#37693=CARTESIAN_POINT('Ctrl Pts',(-1.54974157928885,-4.30953977156619,
378.582721708887));
#37694=CARTESIAN_POINT('Ctrl Pts',(-0.803610144456304,-4.50866307690144,
378.609097667373));
#37695=CARTESIAN_POINT('Ctrl Pts',(-0.0551591253652737,-4.51780112933225,
378.63547362586));
#37696=CARTESIAN_POINT('Ctrl Pts',(0.693291893725671,-4.52693918176306,
378.661849584346));
#37697=CARTESIAN_POINT('Ctrl Pts',(1.44406249707508,-4.34609198128947,378.688225542833));
#37698=CARTESIAN_POINT('Ctrl Pts',(2.10625942952888,-3.99715408620027,378.71460150132));
#37699=CARTESIAN_POINT('Ctrl Pts',(2.76845636198275,-3.64821619111103,378.740977459806));
#37700=CARTESIAN_POINT('Ctrl Pts',(3.34207962354098,-3.13118760140616,378.767353418293));
#37701=CARTESIAN_POINT('Ctrl Pts',(3.75768258797375,-2.50866321799992,378.793729376779));
#37702=CARTESIAN_POINT('Ctrl Pts',(4.1732855524065,-1.88613883459371,378.820105335266));
#37703=CARTESIAN_POINT('Ctrl Pts',(4.43086821971381,-1.15811865748618,378.846481293753));
#37704=CARTESIAN_POINT('Ctrl Pts',(4.49924592843132,-0.412741624749648,
378.872857252239));
#37705=CARTESIAN_POINT('Ctrl Pts',(4.56762363714884,0.332635407986881,378.899233210726));
#37706=CARTESIAN_POINT('Ctrl Pts',(4.44679638727653,1.09536929635249,378.925609169213));
#37707=CARTESIAN_POINT('Ctrl Pts',(4.15139232488624,1.78311843077862,378.951985127699));
#37708=CARTESIAN_POINT('Ctrl Pts',(3.85598826249595,2.47086756520474,378.978361086186));
#37709=CARTESIAN_POINT('Ctrl Pts',(3.38600738758769,3.08363194569147,379.004737044672));
#37710=CARTESIAN_POINT('Ctrl Pts',(2.79834869352904,3.54722626325572,379.031113003159));
#37711=CARTESIAN_POINT('Ctrl Pts',(2.2106899994704,4.01082058081996,379.057488961645));
#37712=CARTESIAN_POINT('Ctrl Pts',(1.5053534862614,4.32524483546169,379.083864920132));
#37713=CARTESIAN_POINT('Ctrl Pts',(0.767731857583539,4.4524327471797,379.110240878618));
#37714=CARTESIAN_POINT('Ctrl Pts',(0.030110228905678,4.5796206588977,379.136616837105));
#37715=CARTESIAN_POINT('Ctrl Pts',(-0.739796515241018,4.51957222769198,
379.162992795591));
#37716=CARTESIAN_POINT('Ctrl Pts',(-1.44877837192307,4.27955731382987,379.189368754078));
#37717=CARTESIAN_POINT('Ctrl Pts',(-2.15776022860516,4.03954239996775,379.215744712565));
#37718=CARTESIAN_POINT('Ctrl Pts',(-2.80581719782259,3.61956100344924,379.242120671052));
#37719=CARTESIAN_POINT('Ctrl Pts',(-3.31449121636045,3.0704588500705,379.268496629538));
#37720=CARTESIAN_POINT('Ctrl Pts',(-3.82316523489829,2.52135669669179,379.294872588025));
#37721=CARTESIAN_POINT('Ctrl Pts',(-4.19245630275656,1.84313378645288,379.321248546511));
#37722=CARTESIAN_POINT('Ctrl Pts',(-4.37765560061389,1.11790027091894,379.347624504998));
#37723=CARTESIAN_POINT('Ctrl Pts',(-4.4707894813135,0.753191481541508,379.360888569168));
#37724=CARTESIAN_POINT('Ctrl Pts',(-4.51736785070585,0.376594041376692,
379.374152633338));
#37725=CARTESIAN_POINT('Ctrl Pts',(-4.51737365644452,-1.98811769755447E-6,
379.387416697508));
#37726=CARTESIAN_POINT('Origin',(0.,0.,387.));
#37727=CARTESIAN_POINT('',(-4.51796103056296,9.30366574888874E-5,380.387416697508));
#37728=CARTESIAN_POINT('',(-4.51744861143269,-7.15418913582019E-5,380.112583302492));
#37729=CARTESIAN_POINT('',(-4.51775,5.53264807684796E-16,387.));
#37730=CARTESIAN_POINT('Ctrl Pts',(-4.51744861143269,-7.15418913582019E-5,
380.112583302492));
#37731=CARTESIAN_POINT('Ctrl Pts',(-4.51718913038702,0.45796072853139,380.09645021147));
#37732=CARTESIAN_POINT('Ctrl Pts',(-4.44792028854276,0.916069730534027,
380.080317120448));
#37733=CARTESIAN_POINT('Ctrl Pts',(-4.31082918580142,1.35289366117352,380.064184029426));
#37734=CARTESIAN_POINT('Ctrl Pts',(-4.08669921406521,2.0670562382494,380.037808070939));
#37735=CARTESIAN_POINT('Ctrl Pts',(-3.68128769636301,2.72432612859277,380.011432112453));
#37736=CARTESIAN_POINT('Ctrl Pts',(-3.14367643259018,3.24512989181911,379.985056153966));
#37737=CARTESIAN_POINT('Ctrl Pts',(-2.60606516881736,3.76593365504543,379.958680195479));
#37738=CARTESIAN_POINT('Ctrl Pts',(-1.93625415897387,4.15027129115475,379.932304236993));
#37739=CARTESIAN_POINT('Ctrl Pts',(-1.21533515432327,4.35161234374879,379.905928278506));
#37740=CARTESIAN_POINT('Ctrl Pts',(-0.494416149672638,4.55295339634284,
379.87955232002));
#37741=CARTESIAN_POINT('Ctrl Pts',(0.27761084978516,4.57129786542164,379.853176361533));
#37742=CARTESIAN_POINT('Ctrl Pts',(1.0072791489844,4.40442484822049,379.826800403046));
#37743=CARTESIAN_POINT('Ctrl Pts',(1.73694744818368,4.23755183101932,379.80042444456));
#37744=CARTESIAN_POINT('Ctrl Pts',(2.4242570471244,3.88546132753817,379.774048486073));
#37745=CARTESIAN_POINT('Ctrl Pts',(2.98599769960395,3.39077974300318,379.747672527587));
#37746=CARTESIAN_POINT('Ctrl Pts',(3.5477383520835,2.89609815846819,379.7212965691));
#37747=CARTESIAN_POINT('Ctrl Pts',(3.98391005810188,2.25882549287937,379.694920610614));
#37748=CARTESIAN_POINT('Ctrl Pts',(4.24170698590533,1.55611419032241,379.668544652127));
#37749=CARTESIAN_POINT('Ctrl Pts',(4.49950391370875,0.853402887765529,379.64216869364));
#37750=CARTESIAN_POINT('Ctrl Pts',(4.57892606329728,0.0852529482405344,
379.615792735154));
#37751=CARTESIAN_POINT('Ctrl Pts',(4.47035806391024,-0.655338315706838,
379.589416776667));
#37752=CARTESIAN_POINT('Ctrl Pts',(4.36179006452319,-1.39592957965429,379.56304081818));
#37753=CARTESIAN_POINT('Ctrl Pts',(4.06523191616051,-2.10896216802411,379.536664859694));
#37754=CARTESIAN_POINT('Ctrl Pts',(3.61658690982335,-2.70811163937072,379.510288901207));
#37755=CARTESIAN_POINT('Ctrl Pts',(3.16794190348622,-3.30726111071731,379.483912942721));
#37756=CARTESIAN_POINT('Ctrl Pts',(2.56721003917463,-3.79252746504069,379.457536984234));
#37757=CARTESIAN_POINT('Ctrl Pts',(1.88711988987541,-4.10516114773068,379.431161025748));
#37758=CARTESIAN_POINT('Ctrl Pts',(1.20702974057619,-4.41779483042066,379.404785067261));
#37759=CARTESIAN_POINT('Ctrl Pts',(0.447581306289357,-4.55779584147724,
379.378409108774));
#37760=CARTESIAN_POINT('Ctrl Pts',(-0.299281562218895,-4.50821473247633,
379.352033150288));
#37761=CARTESIAN_POINT('Ctrl Pts',(-1.04614443072715,-4.45863362347542,
379.325657191801));
#37762=CARTESIAN_POINT('Ctrl Pts',(-1.7804217334568,-4.21947039441701,379.299281233315));
#37763=CARTESIAN_POINT('Ctrl Pts',(-2.41321700332044,-3.81967972773712,
379.272905274828));
#37764=CARTESIAN_POINT('Ctrl Pts',(-3.04601227318407,-3.41988906105724,
379.246529316342));
#37765=CARTESIAN_POINT('Ctrl Pts',(-3.57732551018167,-2.85947095675588,
379.220153357855));
#37766=CARTESIAN_POINT('Ctrl Pts',(-3.94283241951303,-2.20627333738088,
379.193777399368));
#37767=CARTESIAN_POINT('Ctrl Pts',(-4.30833932884442,-1.55307571800585,
379.167401440882));
#37768=CARTESIAN_POINT('Ctrl Pts',(-4.50803991050956,-0.807098583557167,
379.141025482395));
#37769=CARTESIAN_POINT('Ctrl Pts',(-4.51775709118839,-0.0586548601377958,
379.114649523908));
#37770=CARTESIAN_POINT('Ctrl Pts',(-4.51801083042644,-0.0391111728918336,
379.113960783436));
#37771=CARTESIAN_POINT('Ctrl Pts',(-4.51813502773401,-0.0195658037794806,
379.113272042964));
#37772=CARTESIAN_POINT('Ctrl Pts',(-4.51813007169143,-2.03714566067892E-5,
379.112583302492));
#37773=CARTESIAN_POINT('Ctrl Pts',(-4.51737365644452,-1.98811769755447E-6,
379.387416697508));
#37774=CARTESIAN_POINT('Ctrl Pts',(-4.51737939557777,-0.372277579931259,
379.400528591825));
#37775=CARTESIAN_POINT('Ctrl Pts',(-4.47187503399554,-0.744551793256104,
379.413640486141));
#37776=CARTESIAN_POINT('Ctrl Pts',(-4.38084409953505,-1.10533911035289,
379.426752380458));
#37777=CARTESIAN_POINT('Ctrl Pts',(-4.19772577274251,-1.83110085526187,
379.453128338944));
#37778=CARTESIAN_POINT('Ctrl Pts',(-3.83038159130104,-2.51038022425081,
379.479504297431));
#37779=CARTESIAN_POINT('Ctrl Pts',(-3.32328467158491,-3.06093916387039,
379.505880255917));
#37780=CARTESIAN_POINT('Ctrl Pts',(-2.81618775186881,-3.61149810348995,
379.532256214404));
#37781=CARTESIAN_POINT('Ctrl Pts',(-2.16933809387807,-4.03333661374015,
379.558632172891));
#37782=CARTESIAN_POINT('Ctrl Pts',(-1.46104759574481,-4.27538413435274,
379.585008131377));
#37783=CARTESIAN_POINT('Ctrl Pts',(-0.752757097611556,-4.51743165496533,
379.611384089864));
#37784=CARTESIAN_POINT('Ctrl Pts',(0.0169742406642152,-4.57968818594031,
379.63776004835));
#37785=CARTESIAN_POINT('Ctrl Pts',(0.75495765194394,-4.45461653984696,379.664136006837));
#37786=CARTESIAN_POINT('Ctrl Pts',(1.49294106322366,-4.32954489375361,379.690511965324));
#37787=CARTESIAN_POINT('Ctrl Pts',(2.19917654750734,-4.01714507059193,379.71688792381));
#37788=CARTESIAN_POINT('Ctrl Pts',(2.78816256572898,-3.55523825929773,379.743263882297));
#37789=CARTESIAN_POINT('Ctrl Pts',(3.37714858395063,-3.09333144800353,379.769639840783));
#37790=CARTESIAN_POINT('Ctrl Pts',(3.84888513611024,-2.48191764857682,379.79601579927));
#37791=CARTESIAN_POINT('Ctrl Pts',(4.14626067493935,-1.79501865972427,379.822391757756));
#37792=CARTESIAN_POINT('Ctrl Pts',(4.44363621376846,-1.10811967087172,379.848767716243));
#37793=CARTESIAN_POINT('Ctrl Pts',(4.56665073926708,-0.34573549259334,379.87514367473));
#37794=CARTESIAN_POINT('Ctrl Pts',(4.50041129930853,0.399834603758797,379.901519633216));
#37795=CARTESIAN_POINT('Ctrl Pts',(4.43417185934997,1.14540470011094,379.927895591703));
#37796=CARTESIAN_POINT('Ctrl Pts',(4.17867845393423,1.87416071453683,379.954271550189));
#37797=CARTESIAN_POINT('Ctrl Pts',(3.76486280466181,2.49787462363122,379.980647508676));
#37798=CARTESIAN_POINT('Ctrl Pts',(3.35104715538937,3.12158853272565,380.007023467163));
#37799=CARTESIAN_POINT('Ctrl Pts',(2.77890926226022,3.64026033648856,380.033399425649));
#37800=CARTESIAN_POINT('Ctrl Pts',(2.11771592297733,3.99109619564288,380.059775384136));
#37801=CARTESIAN_POINT('Ctrl Pts',(1.45652258369447,4.34193205479719,380.086151342622));
#37802=CARTESIAN_POINT('Ctrl Pts',(0.706273798257865,4.52493196934294,380.112527301109));
#37803=CARTESIAN_POINT('Ctrl Pts',(-0.0422003529064303,4.5179407591868,
380.138903259596));
#37804=CARTESIAN_POINT('Ctrl Pts',(-0.790674504070726,4.51094954903066,
380.165279218082));
#37805=CARTESIAN_POINT('Ctrl Pts',(-1.53737402096271,4.31396721417262,380.191655176569));
#37806=CARTESIAN_POINT('Ctrl Pts',(-2.19189852108271,3.95084173899465,380.218031135055));
#37807=CARTESIAN_POINT('Ctrl Pts',(-2.84642302120274,3.58771626381665,380.244407093542));
#37808=CARTESIAN_POINT('Ctrl Pts',(-3.40877250455077,3.05844764831869,380.270783052029));
#37809=CARTESIAN_POINT('Ctrl Pts',(-3.81086522305661,2.42711265189824,380.297159010515));
#37810=CARTESIAN_POINT('Ctrl Pts',(-4.21295794156245,1.7957776554778,380.323534969002));
#37811=CARTESIAN_POINT('Ctrl Pts',(-4.4547938952261,1.06237627813486,380.349910927489));
#37812=CARTESIAN_POINT('Ctrl Pts',(-4.50709482389231,0.315698941635839,
380.376286885975));
#37813=CARTESIAN_POINT('Ctrl Pts',(-4.51445126403015,0.210674283980221,
380.379996823153));
#37814=CARTESIAN_POINT('Ctrl Pts',(-4.51805792159162,0.105386973232761,
380.38370676033));
#37815=CARTESIAN_POINT('Ctrl Pts',(-4.51796103056296,9.30366574888874E-5,
380.387416697508));
#37816=CARTESIAN_POINT('Origin',(0.,0.,387.));
#37817=CARTESIAN_POINT('',(-4.51777632728029,-0.000114640610663838,381.387416697508));
#37818=CARTESIAN_POINT('',(-4.51771140424386,0.000115276608145368,381.112583302492));
#37819=CARTESIAN_POINT('',(-4.51775,5.53264807684796E-16,387.));
#37820=CARTESIAN_POINT('Ctrl Pts',(-4.51771140424386,0.000115276608145367,
381.112583302492));
#37821=CARTESIAN_POINT('Ctrl Pts',(-4.51789787410811,0.186866521003934,
381.106004338462));
#37822=CARTESIAN_POINT('Ctrl Pts',(-4.50653449305084,0.373595224723727,
381.099425374433));
#37823=CARTESIAN_POINT('Ctrl Pts',(-4.48344098370869,0.558861765736475,
381.092846410403));
#37824=CARTESIAN_POINT('Ctrl Pts',(-4.3908559747359,1.30162043908853,381.066470451916));
#37825=CARTESIAN_POINT('Ctrl Pts',(-4.10973064608376,2.02087752596908,381.04009449343));
#37826=CARTESIAN_POINT('Ctrl Pts',(-3.6740998895201,2.62955500597139,381.013718534943));
#37827=CARTESIAN_POINT('Ctrl Pts',(-3.23846913295646,3.23823248597366,380.987342576457));
#37828=CARTESIAN_POINT('Ctrl Pts',(-2.6483329484813,3.73633035909772,380.96096661797));
#37829=CARTESIAN_POINT('Ctrl Pts',(-1.9751371259962,4.06354560219426,380.934590659483));
#37830=CARTESIAN_POINT('Ctrl Pts',(-1.30194130351109,4.3907608452908,380.908214700997));
#37831=CARTESIAN_POINT('Ctrl Pts',(-0.545685843016022,4.54709345835984,
380.88183874251));
#37832=CARTESIAN_POINT('Ctrl Pts',(0.202071967249689,4.51361678121356,380.855462784024));
#37833=CARTESIAN_POINT('Ctrl Pts',(0.949829777515443,4.48014010406728,380.829086825537));
#37834=CARTESIAN_POINT('Ctrl Pts',(1.68908993755185,4.25685413670566,380.802710867051));
#37835=CARTESIAN_POINT('Ctrl Pts',(2.33035272260718,3.87079135524483,380.776334908564));
#37836=CARTESIAN_POINT('Ctrl Pts',(2.97161550766248,3.48472857378402,380.749958950077));
#37837=CARTESIAN_POINT('Ctrl Pts',(3.51488091773671,2.93588897822401,380.723582991591));
#37838=CARTESIAN_POINT('Ctrl Pts',(3.89437764890032,2.29071872025929,380.697207033104));
#37839=CARTESIAN_POINT('Ctrl Pts',(4.27387438006393,1.64554846229457,380.670831074617));
#37840=CARTESIAN_POINT('Ctrl Pts',(4.48960243231693,0.904047541925131,380.644455116131));
#37841=CARTESIAN_POINT('Ctrl Pts',(4.51544434073745,0.155986965169938,380.618079157644));
#37842=CARTESIAN_POINT('Ctrl Pts',(4.54128624915798,-0.592073611585275,
380.591703199158));
#37843=CARTESIAN_POINT('Ctrl Pts',(4.37724201374605,-1.34669384472619,380.565327240671));
#37844=CARTESIAN_POINT('Ctrl Pts',(4.04317191469819,-2.01651441745319,380.538951282185));
#37845=CARTESIAN_POINT('Ctrl Pts',(3.70910181565035,-2.68633499018016,380.512575323698));
#37846=CARTESIAN_POINT('Ctrl Pts',(3.20500585296659,-3.27135590249316,380.486199365211));
#37847=CARTESIAN_POINT('Ctrl Pts',(2.59191321819219,-3.70075065317313,380.459823406725));
#37848=CARTESIAN_POINT('Ctrl Pts',(1.9788205834178,-4.13014540385311,380.433447448238));
#37849=CARTESIAN_POINT('Ctrl Pts',(1.25673127655275,-4.40391399290007,380.407071489751));
#37850=CARTESIAN_POINT('Ctrl Pts',(0.513066205288616,-4.48891218410335,
380.380695531265));
#37851=CARTESIAN_POINT('Ctrl Pts',(-0.230598865975566,-4.57391037530665,
380.354319572778));
#37852=CARTESIAN_POINT('Ctrl Pts',(-0.995839701638859,-4.47013816866624,
380.327943614292));
#37853=CARTESIAN_POINT('Ctrl Pts',(-1.69001118451102,-4.19015891391108,
380.301567655805));
#37854=CARTESIAN_POINT('Ctrl Pts',(-2.38418266738314,-3.91017965915592,
380.275191697319));
#37855=CARTESIAN_POINT('Ctrl Pts',(-3.00728479746414,-3.45399335628602,
380.248815738832));
#37856=CARTESIAN_POINT('Ctrl Pts',(-3.48388070942679,-2.87682893653492,
380.222439780345));
#37857=CARTESIAN_POINT('Ctrl Pts',(-3.96047662138947,-2.2996645167838,380.196063821859));
#37858=CARTESIAN_POINT('Ctrl Pts',(-4.29056631523378,-1.60152198015145,
380.169687863372));
#37859=CARTESIAN_POINT('Ctrl Pts',(-4.43418694927082,-0.866923079931074,
380.143311904886));
#37860=CARTESIAN_POINT('Ctrl Pts',(-4.48996073737275,-0.581648170267025,
380.133069037421));
#37861=CARTESIAN_POINT('Ctrl Pts',(-4.5176133554335,-0.290875321156064,
380.122826169956));
#37862=CARTESIAN_POINT('Ctrl Pts',(-4.51744861143269,-7.15418913582019E-5,
380.112583302492));
#37863=CARTESIAN_POINT('Ctrl Pts',(-4.51796103056296,9.30366574888874E-5,
380.387416697508));
#37864=CARTESIAN_POINT('Ctrl Pts',(-4.5173690706415,-0.643204813367623,
380.410082718817));
#37865=CARTESIAN_POINT('Ctrl Pts',(-4.37853653898567,-1.28674998247137,
380.432748740126));
#37866=CARTESIAN_POINT('Ctrl Pts',(-4.11200700232459,-1.87215597270644,
380.455414761435));
#37867=CARTESIAN_POINT('Ctrl Pts',(-3.80185234842186,-2.55338025489479,
380.481790719921));
#37868=CARTESIAN_POINT('Ctrl Pts',(-3.3187771369476,-3.15587552361643,380.508166678408));
#37869=CARTESIAN_POINT('Ctrl Pts',(-2.72126564826557,-3.60669971648272,
380.534542636895));
#37870=CARTESIAN_POINT('Ctrl Pts',(-2.12375415958355,-4.05752390934902,
380.560918595381));
#37871=CARTESIAN_POINT('Ctrl Pts',(-1.41180639369374,-4.35667702635998,
380.587294553868));
#37872=CARTESIAN_POINT('Ctrl Pts',(-0.671615456256834,-4.46794161244568,
380.613670512354));
#37873=CARTESIAN_POINT('Ctrl Pts',(0.0685754811800957,-4.57920619853139,
380.640046470841));
#37874=CARTESIAN_POINT('Ctrl Pts',(0.837009590164088,-4.50258225369185,
380.666422429328));
#37875=CARTESIAN_POINT('Ctrl Pts',(1.54065515471516,-4.24734637951232,380.692798387814));
#37876=CARTESIAN_POINT('Ctrl Pts',(2.24430071926626,-3.99211050533279,380.719174346301));
#37877=CARTESIAN_POINT('Ctrl Pts',(2.88315773938438,-3.55826270181326,380.745550304787));
#37878=CARTESIAN_POINT('Ctrl Pts',(3.37988195854491,-2.99832745369971,380.771926263274));
#37879=CARTESIAN_POINT('Ctrl Pts',(3.87660617770542,-2.4383922055862,380.79830222176));
#37880=CARTESIAN_POINT('Ctrl Pts',(4.23119759590837,-1.75236951287867,380.824678180247));
#37881=CARTESIAN_POINT('Ctrl Pts',(4.40072703064927,-1.02331382039902,380.851054138734));
#37882=CARTESIAN_POINT('Ctrl Pts',(4.57025646539019,-0.294258127919331,
380.87743009722));
#37883=CARTESIAN_POINT('Ctrl Pts',(4.55472391666906,0.477830564332509,380.903806055707));
#37884=CARTESIAN_POINT('Ctrl Pts',(4.35600985757286,1.19947809235303,380.930182014193));
#37885=CARTESIAN_POINT('Ctrl Pts',(4.15729579847668,1.92112562037352,380.95655797268));
#37886=CARTESIAN_POINT('Ctrl Pts',(3.77540022900545,2.59233198416271,380.982933931167));
#37887=CARTESIAN_POINT('Ctrl Pts',(3.25655795281734,3.131836501679,381.009309889653));
#37888=CARTESIAN_POINT('Ctrl Pts',(2.73771567662922,3.6713410191953,381.03568584814));
#37889=CARTESIAN_POINT('Ctrl Pts',(2.08192669372421,4.07914369043871,381.062061806626));
#37890=CARTESIAN_POINT('Ctrl Pts',(1.36858515603701,4.30587322665008,381.088437765113));
#37891=CARTESIAN_POINT('Ctrl Pts',(0.655243618349795,4.53260276286145,381.1148137236));
#37892=CARTESIAN_POINT('Ctrl Pts',(-0.11565047411956,4.57825916404077,381.141189682086));
#37893=CARTESIAN_POINT('Ctrl Pts',(-0.850767583518968,4.43731496427064,
381.167565640573));
#37894=CARTESIAN_POINT('Ctrl Pts',(-1.58588469291835,4.2963707645005,381.193941599059));
#37895=CARTESIAN_POINT('Ctrl Pts',(-2.28522481924775,3.96882596378091,381.220317557546));
#37896=CARTESIAN_POINT('Ctrl Pts',(-2.8641212210839,3.49433530220608,381.246693516033));
#37897=CARTESIAN_POINT('Ctrl Pts',(-3.44301762292008,3.01984464063123,381.273069474519));
#37898=CARTESIAN_POINT('Ctrl Pts',(-3.90147030026302,2.39840811820112,381.299445433006));
#37899=CARTESIAN_POINT('Ctrl Pts',(-4.18397593959467,1.70526095076376,381.325821391492));
#37900=CARTESIAN_POINT('Ctrl Pts',(-4.40388606866954,1.16569620642928,381.346353160164));
#37901=CARTESIAN_POINT('Ctrl Pts',(-4.51718122901344,0.58267845338523,381.366884928836));
#37902=CARTESIAN_POINT('Ctrl Pts',(-4.51777632728029,-0.000114640610663838,
381.387416697508));
#37903=CARTESIAN_POINT('Origin',(0.,0.,387.));
#37904=CARTESIAN_POINT('',(-4.51741634198117,5.54534861180178E-5,382.387416697508));
#37905=CARTESIAN_POINT('',(-4.51801683772092,-7.91791388051273E-5,382.112583302492));
#37906=CARTESIAN_POINT('',(-4.51775,5.53264807684796E-16,387.));
#37907=CARTESIAN_POINT('Ctrl Pts',(-4.51801683772092,-7.91791388051273E-5,
382.112583302492));
#37908=CARTESIAN_POINT('Ctrl Pts',(-4.51747244268795,0.664048991360067,
382.089182506968));
#37909=CARTESIAN_POINT('Ctrl Pts',(-4.36919765227329,1.32841221793627,382.065781711444));
#37910=CARTESIAN_POINT('Ctrl Pts',(-4.08568376167234,1.92892657382487,382.04238091592));
#37911=CARTESIAN_POINT('Ctrl Pts',(-3.76612408682134,2.60578996102738,382.016004957434));
#37912=CARTESIAN_POINT('Ctrl Pts',(-3.27475081492882,3.20153698377045,381.989628998947));
#37913=CARTESIAN_POINT('Ctrl Pts',(-2.67105284443962,3.64404256695937,381.963253040461));
#37914=CARTESIAN_POINT('Ctrl Pts',(-2.06735487395043,4.08654815014828,381.936877081974));
#37915=CARTESIAN_POINT('Ctrl Pts',(-1.35133220486457,4.37581229378304,381.910501123487));
#37916=CARTESIAN_POINT('Ctrl Pts',(-0.609671277576736,4.47681476732048,
381.884125165001));
#37917=CARTESIAN_POINT('Ctrl Pts',(0.131989649711098,4.57781724085793,381.857749206514));
#37918=CARTESIAN_POINT('Ctrl Pts',(0.899288835200903,4.49055804429805,381.831373248027));
#37919=CARTESIAN_POINT('Ctrl Pts',(1.59933196425767,4.22560135314543,381.804997289541));
#37920=CARTESIAN_POINT('Ctrl Pts',(2.29937509331447,3.9606446619928,381.778621331054));
#37921=CARTESIAN_POINT('Ctrl Pts',(2.93216216593823,3.5179904762474,381.752245372568));
#37922=CARTESIAN_POINT('Ctrl Pts',(3.42108379359719,2.95122943953659,381.725869414081));
#37923=CARTESIAN_POINT('Ctrl Pts',(3.91000542125612,2.38446840282581,381.699493455595));
#37924=CARTESIAN_POINT('Ctrl Pts',(4.25506160395026,1.69360051514964,381.673117497108));
#37925=CARTESIAN_POINT('Ctrl Pts',(4.41447755785592,0.962266812681007,381.646741538621));
#37926=CARTESIAN_POINT('Ctrl Pts',(4.57389351176158,0.23093311021233,381.620365580135));
#37927=CARTESIAN_POINT('Ctrl Pts',(4.54766923687872,-0.540866407048814,
381.593989621648));
#37928=CARTESIAN_POINT('Ctrl Pts',(4.33897961738306,-1.25969258453608,381.567613663161));
#37929=CARTESIAN_POINT('Ctrl Pts',(4.1302899978874,-1.9785187620233,381.541237704675));
#37930=CARTESIAN_POINT('Ctrl Pts',(3.73913503377896,-2.64437159973664,381.514861746188));
#37931=CARTESIAN_POINT('Ctrl Pts',(3.21287053227619,-3.17663854891175,381.488485787702));
#37932=CARTESIAN_POINT('Ctrl Pts',(2.68660603077342,-3.70890549808685,381.462109829215));
#37933=CARTESIAN_POINT('Ctrl Pts',(2.02523199187631,-4.1075865587237,381.435733870728));
#37934=CARTESIAN_POINT('Ctrl Pts',(1.3088187313399,-4.32441476457735,381.409357912242));
#37935=CARTESIAN_POINT('Ctrl Pts',(0.592405470803483,-4.54124297043101,
381.382981953755));
#37936=CARTESIAN_POINT('Ctrl Pts',(-0.179047011372244,-4.57621832150146,
381.356605995269));
#37937=CARTESIAN_POINT('Ctrl Pts',(-0.912141574983824,-4.42510647044643,
381.330230036782));
#37938=CARTESIAN_POINT('Ctrl Pts',(-1.64523613859541,-4.2739946193914,381.303854078296));
#37939=CARTESIAN_POINT('Ctrl Pts',(-2.33997278364284,-3.93679556621089,
381.277478119809));
#37940=CARTESIAN_POINT('Ctrl Pts',(-2.91224209659624,-3.45433285865933,
381.251102161322));
#37941=CARTESIAN_POINT('Ctrl Pts',(-3.48451140954963,-2.97187015110778,
381.224726202836));
#37942=CARTESIAN_POINT('Ctrl Pts',(-3.93431339040899,-2.34414378918517,
381.198350244349));
#37943=CARTESIAN_POINT('Ctrl Pts',(-4.20719203619195,-1.64715047831211,
381.171974285863));
#37944=CARTESIAN_POINT('Ctrl Pts',(-4.4120064713043,-1.1240084389856,381.152177291406));
#37945=CARTESIAN_POINT('Ctrl Pts',(-4.51715029114881,-0.561844529442614,
381.132380296949));
#37946=CARTESIAN_POINT('Ctrl Pts',(-4.51771140424386,0.000115276608145367,
381.112583302492));
#37947=CARTESIAN_POINT('Ctrl Pts',(-4.51777632728029,-0.000114640610663838,
381.387416697508));
#37948=CARTESIAN_POINT('Ctrl Pts',(-4.51794571683875,-0.166001638386794,
381.393260887323));
#37949=CARTESIAN_POINT('Ctrl Pts',(-4.50898407036945,-0.331870434133353,
381.399105077137));
#37950=CARTESIAN_POINT('Ctrl Pts',(-4.49075105445655,-0.496713740704063,
381.404949266952));
#37951=CARTESIAN_POINT('Ctrl Pts',(-4.40846192866641,-1.24068345228999,
381.431325225439));
#37952=CARTESIAN_POINT('Ctrl Pts',(-4.13732507576575,-1.96376506301729,
381.457701183925));
#37953=CARTESIAN_POINT('Ctrl Pts',(-3.71016611657994,-2.57841753032532,
381.484077142412));
#37954=CARTESIAN_POINT('Ctrl Pts',(-3.28300715739413,-3.19306999763336,
381.510453100898));
#37955=CARTESIAN_POINT('Ctrl Pts',(-2.69982609192317,-3.69929332152213,
381.536829059385));
#37956=CARTESIAN_POINT('Ctrl Pts',(-2.03122667735788,-4.03580075802764,
381.563205017872));
#37957=CARTESIAN_POINT('Ctrl Pts',(-1.36262726279259,-4.37230819453315,
381.589580976358));
#37958=CARTESIAN_POINT('Ctrl Pts',(-0.608609499132967,-4.5390997436554,
381.615956934845));
#37959=CARTESIAN_POINT('Ctrl Pts',(0.139540235761641,-4.51598251722816,
381.642332893331));
#37960=CARTESIAN_POINT('Ctrl Pts',(0.887689970656269,-4.49286529080092,
381.668708851818));
#37961=CARTESIAN_POINT('Ctrl Pts',(1.62997167678589,-4.2798392888242,381.695084810305));
#37962=CARTESIAN_POINT('Ctrl Pts',(2.27651982104296,-3.90269484814088,381.721460768791));
#37963=CARTESIAN_POINT('Ctrl Pts',(2.92306796530002,-3.52555040745756,381.747836727278));
#37964=CARTESIAN_POINT('Ctrl Pts',(3.47388254768454,-2.98428752806765,381.774212685764));
#37965=CARTESIAN_POINT('Ctrl Pts',(3.86227831153366,-2.3444350742905,381.800588644251));
#37966=CARTESIAN_POINT('Ctrl Pts',(4.25067407538277,-1.70458262051336,381.826964602737));
#37967=CARTESIAN_POINT('Ctrl Pts',(4.47665102069649,-0.966140592348972,
381.853340561224));
#37968=CARTESIAN_POINT('Ctrl Pts',(4.51285088376856,-0.21850966609316,381.879716519711));
#37969=CARTESIAN_POINT('Ctrl Pts',(4.54905074684063,0.529121260162651,381.906092478197));
#37970=CARTESIAN_POINT('Ctrl Pts',(4.39547352767104,1.28594108450989,381.932468436684));
#37971=CARTESIAN_POINT('Ctrl Pts',(4.07071230023681,1.96032419308837,381.95884439517));
#37972=CARTESIAN_POINT('Ctrl Pts',(3.74595107280257,2.63470730166687,381.985220353657));
#37973=CARTESIAN_POINT('Ctrl Pts',(3.25000583710367,3.2266536944766,382.011596312144));
#37974=CARTESIAN_POINT('Ctrl Pts',(2.64291900376427,3.66449842582154,382.03797227063));
#37975=CARTESIAN_POINT('Ctrl Pts',(2.03583217042486,4.10234315716648,382.064348229117));
#37976=CARTESIAN_POINT('Ctrl Pts',(1.31760373944494,4.38608622704663,382.090724187603));
#37977=CARTESIAN_POINT('Ctrl Pts',(0.575187195343948,4.48137582262626,382.11710014609));
#37978=CARTESIAN_POINT('Ctrl Pts',(-0.167229348757025,4.57666541820589,
382.143476104577));
#37979=CARTESIAN_POINT('Ctrl Pts',(-0.933834005979071,4.48350153948501,
382.169852063063));
#37980=CARTESIAN_POINT('Ctrl Pts',(-1.63181654587318,4.21316322184666,382.19622802155));
#37981=CARTESIAN_POINT('Ctrl Pts',(-2.32979908576728,3.94282490420832,382.222603980037));
#37982=CARTESIAN_POINT('Ctrl Pts',(-2.95915950833345,3.4953121476525,382.248979938523));
#37983=CARTESIAN_POINT('Ctrl Pts',(-3.44370327796121,2.9248038065255,382.27535589701));
#37984=CARTESIAN_POINT('Ctrl Pts',(-3.92824704758899,2.35429546539847,382.301731855496));
#37985=CARTESIAN_POINT('Ctrl Pts',(-4.26797416427836,1.66079153970024,382.328107813983));
#37986=CARTESIAN_POINT('Ctrl Pts',(-4.42175501618481,0.928252201802573,
382.354483772469));
#37987=CARTESIAN_POINT('Ctrl Pts',(-4.48575841876287,0.623370224843185,
382.365461414149));
#37988=CARTESIAN_POINT('Ctrl Pts',(-4.5175519448549,0.311726478256462,382.376439055828));
#37989=CARTESIAN_POINT('Ctrl Pts',(-4.51741634198117,5.54534861180178E-5,
382.387416697508));
#37990=CARTESIAN_POINT('Origin',(0.,0.,387.));
#37991=CARTESIAN_POINT('',(-4.51810647145572,4.12515443024009E-5,383.387416697508));
#37992=CARTESIAN_POINT('',(-4.51737744603353,-1.71510238390164E-5,383.112583302492));
#37993=CARTESIAN_POINT('',(-4.51775,5.53264807684796E-16,387.));
#37994=CARTESIAN_POINT('Ctrl Pts',(-4.51737744603353,-1.71510238390164E-5,
383.112583302492));
#37995=CARTESIAN_POINT('Ctrl Pts',(-4.51732510787532,0.393119355640695,
383.09873663396));
#37996=CARTESIAN_POINT('Ctrl Pts',(-4.46651507043149,0.786269138328428,
383.084889965429));
#37997=CARTESIAN_POINT('Ctrl Pts',(-4.36511527641182,1.16590657912072,383.071043296898));
#37998=CARTESIAN_POINT('Ctrl Pts',(-4.17196291261205,1.8890625754899,383.044667338411));
#37999=CARTESIAN_POINT('Ctrl Pts',(-3.79524613196318,2.56318917681575,383.018291379924));
#38000=CARTESIAN_POINT('Ctrl Pts',(-3.28057275969385,3.10667215778483,382.991915421438));
#38001=CARTESIAN_POINT('Ctrl Pts',(-2.76589938742451,3.65015513875392,382.965539462951));
#38002=CARTESIAN_POINT('Ctrl Pts',(-2.11326942353471,4.06299449936623,382.939163504465));
#38003=CARTESIAN_POINT('Ctrl Pts',(-1.40169456822207,4.29520917593283,382.912787545978));
#38004=CARTESIAN_POINT('Ctrl Pts',(-0.690119712909428,4.52742385249943,
382.886411587491));
#38005=CARTESIAN_POINT('Ctrl Pts',(0.0804000338260355,4.57901384502031,
382.860035629005));
#38006=CARTESIAN_POINT('Ctrl Pts',(0.816580454902776,4.44373332776299,382.833659670518));
#38007=CARTESIAN_POINT('Ctrl Pts',(1.55276087597956,4.30845281050567,382.807283712031));
#38008=CARTESIAN_POINT('Ctrl Pts',(2.2546019713976,3.98630178347012,382.780907753545));
#38009=CARTESIAN_POINT('Ctrl Pts',(2.83713421587333,3.51628198083169,382.754531795058));
#38010=CARTESIAN_POINT('Ctrl Pts',(3.41966646034902,3.04626217819329,382.728155836572));
#38011=CARTESIAN_POINT('Ctrl Pts',(3.88288985388241,2.42837359995203,382.701779878085));
#38012=CARTESIAN_POINT('Ctrl Pts',(4.17072350849794,1.7374219243648,382.675403919598));
#38013=CARTESIAN_POINT('Ctrl Pts',(4.45855716311345,1.04647024877758,382.649027961112));
#38014=CARTESIAN_POINT('Ctrl Pts',(4.57100107881112,0.282455475844346,382.622652002625));
#38015=CARTESIAN_POINT('Ctrl Pts',(4.4944420514052,-0.462125712508384,382.596276044139));
#38016=CARTESIAN_POINT('Ctrl Pts',(4.41788302399928,-1.20670690086118,382.569900085652));
#38017=CARTESIAN_POINT('Ctrl Pts',(4.15232105348975,-1.93185450463351,382.543524127166));
#38018=CARTESIAN_POINT('Ctrl Pts',(3.72990682856509,-2.54977735848138,382.517148168679));
#38019=CARTESIAN_POINT('Ctrl Pts',(3.30749260364046,-3.16770021232922,382.490772210192));
#38020=CARTESIAN_POINT('Ctrl Pts',(2.72822612430073,-3.6783983162526,382.464396251706));
#38021=CARTESIAN_POINT('Ctrl Pts',(2.06223722204694,-4.02004317981846,382.438020293219));
#38022=CARTESIAN_POINT('Ctrl Pts',(1.39624831979316,-4.36168804338432,382.411644334732));
#38023=CARTESIAN_POINT('Ctrl Pts',(0.643536994625335,-4.53427966659265,
382.385268376246));
#38024=CARTESIAN_POINT('Ctrl Pts',(-0.104768541682353,-4.51692296594424,
382.358892417759));
#38025=CARTESIAN_POINT('Ctrl Pts',(-0.853074077990042,-4.49956626529584,
382.332516459273));
#38026=CARTESIAN_POINT('Ctrl Pts',(-1.59697382543758,-4.29226124079071,
382.306140500786));
#38027=CARTESIAN_POINT('Ctrl Pts',(-2.2464063601331,-3.92010560989808,382.2797645423));
#38028=CARTESIAN_POINT('Ctrl Pts',(-2.89583889482865,-3.54794997900543,
382.253388583813));
#38029=CARTESIAN_POINT('Ctrl Pts',(-3.45080421677215,-3.01094374172526,
382.227012625326));
#38030=CARTESIAN_POINT('Ctrl Pts',(-3.84411455331502,-2.37410042512789,
382.20063666684));
#38031=CARTESIAN_POINT('Ctrl Pts',(-4.23742488985787,-1.73725710853056,
382.174260708353));
#38032=CARTESIAN_POINT('Ctrl Pts',(-4.46908024100009,-1.00057671261605,
382.147884749867));
#38033=CARTESIAN_POINT('Ctrl Pts',(-4.51103487766645,-0.253246638827817,
382.12150879138));
#38034=CARTESIAN_POINT('Ctrl Pts',(-4.51576728885779,-0.168949085903131,
382.118533628417));
#38035=CARTESIAN_POINT('Ctrl Pts',(-4.51808605177553,-0.0845160322941951,
382.115558465455));
#38036=CARTESIAN_POINT('Ctrl Pts',(-4.51801683772092,-7.91791388051273E-5,
382.112583302492));
#38037=CARTESIAN_POINT('Ctrl Pts',(-4.51741634198117,5.54534861180178E-5,
382.387416697508));
#38038=CARTESIAN_POINT('Ctrl Pts',(-4.51722613209177,-0.43712489171991,
382.402815014315));
#38039=CARTESIAN_POINT('Ctrl Pts',(-4.45421338524669,-0.874358908440133,
382.418213331122));
#38040=CARTESIAN_POINT('Ctrl Pts',(-4.32915293519383,-1.29306010572185,
382.433611647929));
#38041=CARTESIAN_POINT('Ctrl Pts',(-4.11493541517289,-2.01025832525158,
382.459987606416));
#38042=CARTESIAN_POINT('Ctrl Pts',(-3.71866578800746,-2.67308001421398,
382.486363564902));
#38043=CARTESIAN_POINT('Ctrl Pts',(-3.1883190758562,-3.2012795947618,382.512739523389));
#38044=CARTESIAN_POINT('Ctrl Pts',(-2.65797236370492,-3.72947917530964,
382.539115481875));
#38045=CARTESIAN_POINT('Ctrl Pts',(-1.99354856656775,-4.1230566474429,382.565491440362));
#38046=CARTESIAN_POINT('Ctrl Pts',(-1.27548722410474,-4.33436291909808,
382.591867398849));
#38047=CARTESIAN_POINT('Ctrl Pts',(-0.557425881641732,-4.54566919075325,
382.618243357335));
#38048=CARTESIAN_POINT('Ctrl Pts',(0.214273006147169,-4.57470426193039,
382.644619315822));
#38049=CARTESIAN_POINT('Ctrl Pts',(0.94618246756513,-4.4179529548626,382.670995274309));
#38050=CARTESIAN_POINT('Ctrl Pts',(1.67809192898305,-4.26120164779482,382.697371232795));
#38051=CARTESIAN_POINT('Ctrl Pts',(2.37021196402998,-3.91866396248217,382.723747191282));
#38052=CARTESIAN_POINT('Ctrl Pts',(2.93874994329017,-3.4318097767969,382.750123149768));
#38053=CARTESIAN_POINT('Ctrl Pts',(3.50728792255042,-2.94495559111159,382.776499108255));
#38054=CARTESIAN_POINT('Ctrl Pts',(3.95224384602383,-2.31378490505366,382.802875066742));
#38055=CARTESIAN_POINT('Ctrl Pts',(4.21974840648906,-1.61471141670574,382.829251025228));
#38056=CARTESIAN_POINT('Ctrl Pts',(4.48725296695428,-0.91563792835784,382.855626983715));
#38057=CARTESIAN_POINT('Ctrl Pts',(4.57730616441131,-0.148661637719957,
382.882002942201));
#38058=CARTESIAN_POINT('Ctrl Pts',(4.47900556312629,0.593362232359432,382.908378900688));
#38059=CARTESIAN_POINT('Ctrl Pts',(4.38070496184126,1.33538610243882,382.934754859174));
#38060=CARTESIAN_POINT('Ctrl Pts',(4.09405056181417,2.05245755195971,382.961130817661));
#38061=CARTESIAN_POINT('Ctrl Pts',(3.6537466407651,2.65776316823087,382.987506776148));
#38062=CARTESIAN_POINT('Ctrl Pts',(3.21344271971605,3.26306878450199,383.013882734634));
#38063=CARTESIAN_POINT('Ctrl Pts',(2.61948927764498,3.75660856752342,383.040258693121));
#38064=CARTESIAN_POINT('Ctrl Pts',(1.94379424690704,4.07863132668275,383.066634651607));
#38065=CARTESIAN_POINT('Ctrl Pts',(1.26809921616909,4.4006540858421,383.093010610094));
#38066=CARTESIAN_POINT('Ctrl Pts',(0.510662596764224,4.55115982113938,383.119386568581));
#38067=CARTESIAN_POINT('Ctrl Pts',(-0.236815324157952,4.51192731275126,
383.145762527067));
#38068=CARTESIAN_POINT('Ctrl Pts',(-0.984293245080149,4.47269480436314,
383.172138485554));
#38069=CARTESIAN_POINT('Ctrl Pts',(-1.72181246751965,4.24372405228961,383.19851444404));
#38070=CARTESIAN_POINT('Ctrl Pts',(-2.36008403614551,3.85273577028557,383.224890402527));
#38071=CARTESIAN_POINT('Ctrl Pts',(-2.99835560477138,3.46174748828153,383.251266361013));
#38072=CARTESIAN_POINT('Ctrl Pts',(-3.53737951958361,2.90874167634699,383.2776423195));
#38073=CARTESIAN_POINT('Ctrl Pts',(-3.91189798012409,2.26066887588782,383.304018277987));
#38074=CARTESIAN_POINT('Ctrl Pts',(-4.28641644066456,1.61259607542868,383.330394236473));
#38075=CARTESIAN_POINT('Ctrl Pts',(-4.49642944693329,0.869456286444925,
383.35677019496));
#38076=CARTESIAN_POINT('Ctrl Pts',(-4.51651143527701,0.121218927230134,
383.383146153446));
#38077=CARTESIAN_POINT('Ctrl Pts',(-4.5175952633915,0.0808364375906089,
383.384569668134));
#38078=CARTESIAN_POINT('Ctrl Pts',(-4.51812586459283,0.0404390998600549,
383.385993182821));
#38079=CARTESIAN_POINT('Ctrl Pts',(-4.51810647145572,4.12515443024009E-5,
383.387416697508));
#38080=CARTESIAN_POINT('Origin',(0.,0.,387.));
#38081=CARTESIAN_POINT('',(-4.51758348284472,-0.000105543616906456,384.387416697508));
#38082=CARTESIAN_POINT('',(-4.51791286673421,0.000101789655423226,384.112583302492));
#38083=CARTESIAN_POINT('',(-4.51775,5.53264807684796E-16,387.));
#38084=CARTESIAN_POINT('Ctrl Pts',(-4.51791286673421,0.000101789655423226,
384.112583302492));
#38085=CARTESIAN_POINT('Ctrl Pts',(-4.51803160945122,0.121934720290465,
384.108290760953));
#38086=CARTESIAN_POINT('Ctrl Pts',(-4.51320179205148,0.243758262585871,
384.103998219414));
#38087=CARTESIAN_POINT('Ctrl Pts',(-4.50335615873677,0.365175074681226,
384.099705677874));
#38088=CARTESIAN_POINT('Ctrl Pts',(-4.4428586625063,1.11123303735971,384.073329719388));
#38089=CARTESIAN_POINT('Ctrl Pts',(-4.19298336184317,1.84193444118764,384.046953760901));
#38090=CARTESIAN_POINT('Ctrl Pts',(-3.78398181342604,2.46881574105112,384.020577802415));
#38091=CARTESIAN_POINT('Ctrl Pts',(-3.37498026500888,3.09569704091462,383.994201843928));
#38092=CARTESIAN_POINT('Ctrl Pts',(-2.80685246883769,3.61875823681367,383.967825885442));
#38093=CARTESIAN_POINT('Ctrl Pts',(-2.14837973375322,3.97467408062589,383.941449926955));
#38094=CARTESIAN_POINT('Ctrl Pts',(-1.48990699866878,4.33058992443809,383.915073968468));
#38095=CARTESIAN_POINT('Ctrl Pts',(-0.741089324671071,4.5193604161635,383.888698009982));
#38096=CARTESIAN_POINT('Ctrl Pts',(0.00741646763062709,4.51813175146638,
383.862322051495));
#38097=CARTESIAN_POINT('Ctrl Pts',(0.755922259932325,4.51690308676927,383.835946093009));
#38098=CARTESIAN_POINT('Ctrl Pts',(1.50411617053801,4.32567526564963,383.809570134522));
#38099=CARTESIAN_POINT('Ctrl Pts',(2.16141689576047,3.96759959299347,383.783194176035));
#38100=CARTESIAN_POINT('Ctrl Pts',(2.81871762098293,3.60952392033731,383.756818217549));
#38101=CARTESIAN_POINT('Ctrl Pts',(3.38512516082216,3.08460039614464,383.730442259062));
#38102=CARTESIAN_POINT('Ctrl Pts',(3.79206647204748,2.45637973431923,383.704066300576));
#38103=CARTESIAN_POINT('Ctrl Pts',(4.19900778327279,1.82815907249382,383.677690342089));
#38104=CARTESIAN_POINT('Ctrl Pts',(4.44648286588418,1.09664127303568,383.651314383602));
#38105=CARTESIAN_POINT('Ctrl Pts',(4.50453074947641,0.35038871931369,383.624938425116));
#38106=CARTESIAN_POINT('Ctrl Pts',(4.56257863306864,-0.395863834408303,
383.598562466629));
#38107=CARTESIAN_POINT('Ctrl Pts',(4.4311993176417,-1.15685114239415,383.572186508143));
#38108=CARTESIAN_POINT('Ctrl Pts',(4.12629845211925,-1.84044304764888,383.545810549656));
#38109=CARTESIAN_POINT('Ctrl Pts',(3.8213975865968,-2.52403495290361,383.519434591169));
#38110=CARTESIAN_POINT('Ctrl Pts',(3.34297517097883,-3.13023145542722,383.493058632683));
#38111=CARTESIAN_POINT('Ctrl Pts',(2.74895218738718,-3.58564239698551,383.466682674196));
#38112=CARTESIAN_POINT('Ctrl Pts',(2.15492920379552,-4.04105333854382,383.44030671571));
#38113=CARTESIAN_POINT('Ctrl Pts',(1.44530565223012,-4.34567871913682,383.413930757223));
#38114=CARTESIAN_POINT('Ctrl Pts',(0.705993253592304,-4.46263857526945,
383.387554798737));
#38115=CARTESIAN_POINT('Ctrl Pts',(-0.0333191450455116,-4.57959843140208,
383.36117884025));
#38116=CARTESIAN_POINT('Ctrl Pts',(-0.802320390755788,-4.50889276307437,
383.334802881763));
#38117=CARTESIAN_POINT('Ctrl Pts',(-1.50791010623509,-4.25908166617111,
383.308426923277));
#38118=CARTESIAN_POINT('Ctrl Pts',(-2.21349982171436,-4.00927056926786,
383.28205096479));
#38119=CARTESIAN_POINT('Ctrl Pts',(-2.8556780069626,-3.58035404378911,383.255675006304));
#38120=CARTESIAN_POINT('Ctrl Pts',(-3.35669832323709,-3.02425956134359,
383.229299047817));
#38121=CARTESIAN_POINT('Ctrl Pts',(-3.85771863951158,-2.46816507889806,
383.20292308933));
#38122=CARTESIAN_POINT('Ctrl Pts',(-4.21758108681228,-1.78489263948572,
383.176547130844));
#38123=CARTESIAN_POINT('Ctrl Pts',(-4.39271833698727,-1.05716372407332,
383.150171172357));
#38124=CARTESIAN_POINT('Ctrl Pts',(-4.4759132430793,-0.711472908911519,
383.137641882402));
#38125=CARTESIAN_POINT('Ctrl Pts',(-4.51742480471468,-0.355750464977554,
383.125112592447));
#38126=CARTESIAN_POINT('Ctrl Pts',(-4.51737744603353,-1.71510238390164E-5,
383.112583302492));
#38127=CARTESIAN_POINT('Ctrl Pts',(-4.51810647145572,4.12515443024009E-5,
383.387416697508));
#38128=CARTESIAN_POINT('Ctrl Pts',(-4.51776653385746,-0.70808283654263,
383.412369141307));
#38129=CARTESIAN_POINT('Ctrl Pts',(-4.34843679840707,-1.41636380567975,
383.437321585107));
#38130=CARTESIAN_POINT('Ctrl Pts',(-4.0275273935072,-2.04758215167448,383.462274028906));
#38131=CARTESIAN_POINT('Ctrl Pts',(-3.68831039297495,-2.71481094191849,
383.488649987393));
#38132=CARTESIAN_POINT('Ctrl Pts',(-3.17972542149173,-3.29593359296068,
383.515025945879));
#38133=CARTESIAN_POINT('Ctrl Pts',(-2.56334513970026,-3.72059555287616,
383.541401904366));
#38134=CARTESIAN_POINT('Ctrl Pts',(-1.94696485790879,-4.14525751279165,
383.567777862853));
#38135=CARTESIAN_POINT('Ctrl Pts',(-1.22278926580908,-4.41345878158044,
383.594153821339));
#38136=CARTESIAN_POINT('Ctrl Pts',(-0.478491850582746,-4.49272913964694,
383.620529779826));
#38137=CARTESIAN_POINT('Ctrl Pts',(0.265805564643564,-4.57199949771343,
383.646905738312));
#38138=CARTESIAN_POINT('Ctrl Pts',(1.0302248029965,-4.46233894505765,383.673281696799));
#38139=CARTESIAN_POINT('Ctrl Pts',(1.72222021529061,-4.17702371352512,383.699657655286));
#38140=CARTESIAN_POINT('Ctrl Pts',(2.41421562758474,-3.89170848199258,383.726033613772));
#38141=CARTESIAN_POINT('Ctrl Pts',(3.03378721382,-3.43073857158334,383.752409572259));
#38142=CARTESIAN_POINT('Ctrl Pts',(3.50592553965972,-2.84992204870037,383.778785530746));
#38143=CARTESIAN_POINT('Ctrl Pts',(3.97806386549944,-2.2691055258174,383.805161489232));
#38144=CARTESIAN_POINT('Ctrl Pts',(4.30276893094358,-1.56844239046068,383.831537447719));
#38145=CARTESIAN_POINT('Ctrl Pts',(4.44072979303352,-0.832759556277373,
383.857913406205));
#38146=CARTESIAN_POINT('Ctrl Pts',(4.57869065512346,-0.0970767220940631,
383.884289364692));
#38147=CARTESIAN_POINT('Ctrl Pts',(4.52990731385923,0.673625810915847,383.910665323178));
#38148=CARTESIAN_POINT('Ctrl Pts',(4.30028580320783,1.38604169635549,383.937041281665));
#38149=CARTESIAN_POINT('Ctrl Pts',(4.07066429255644,2.0984575817951,383.963417240152));
#38150=CARTESIAN_POINT('Ctrl Pts',(3.66020461251785,2.75258681966445,383.989793198638));
#38151=CARTESIAN_POINT('Ctrl Pts',(3.11859972691059,3.26923619774099,384.016169157125));
#38152=CARTESIAN_POINT('Ctrl Pts',(2.57699484130331,3.78588557581757,384.042545115611));
#38153=CARTESIAN_POINT('Ctrl Pts',(1.90424475012738,4.16505509410136,384.068921074098));
#38154=CARTESIAN_POINT('Ctrl Pts',(1.18179702927259,4.36083998272228,384.095297032584));
#38155=CARTESIAN_POINT('Ctrl Pts',(0.459349308417798,4.55662487134321,384.121672991071));
#38156=CARTESIAN_POINT('Ctrl Pts',(-0.312796042115809,4.56902513030122,
384.148048949558));
#38157=CARTESIAN_POINT('Ctrl Pts',(-1.04115799889843,4.39653950222634,384.174424908044));
#38158=CARTESIAN_POINT('Ctrl Pts',(-1.76951995568104,4.22405387415146,384.200800866531));
#38159=CARTESIAN_POINT('Ctrl Pts',(-2.45409851871268,3.86668235904368,384.227176825017));
#38160=CARTESIAN_POINT('Ctrl Pts',(-3.0120140790621,3.36769071632751,384.253552783504));
#38161=CARTESIAN_POINT('Ctrl Pts',(-3.56992963941149,2.86869907361137,384.279928741991));
#38162=CARTESIAN_POINT('Ctrl Pts',(-4.00118219707867,2.22808730328684,384.306304700477));
#38163=CARTESIAN_POINT('Ctrl Pts',(-4.25356146494663,1.52341210354517,384.332680658964));
#38164=CARTESIAN_POINT('Ctrl Pts',(-4.42814268873775,1.0359589946372,384.350926005145));
#38165=CARTESIAN_POINT('Ctrl Pts',(-4.51713190568983,0.51785112729682,384.369171351326));
#38166=CARTESIAN_POINT('Ctrl Pts',(-4.51758348284472,-0.000105543616906456,
384.387416697508));
#38167=CARTESIAN_POINT('Origin',(0.,0.,387.));
#38168=CARTESIAN_POINT('',(-4.51754236316255,9.86160820556914E-5,385.387416697508));
#38169=CARTESIAN_POINT('',(-4.51782825948384,-0.000111641905798056,385.112583302492));
#38170=CARTESIAN_POINT('',(-4.51775,5.53264807684796E-16,387.));
#38171=CARTESIAN_POINT('Ctrl Pts',(-4.51782825948384,-0.000111641905798056,
385.112583302492));
#38172=CARTESIAN_POINT('Ctrl Pts',(-4.51721726779753,0.599198793910267,
385.091468929459));
#38173=CARTESIAN_POINT('Ctrl Pts',(-4.39722715972494,1.19874658011254,385.070354556425));
#38174=CARTESIAN_POINT('Ctrl Pts',(-4.16499712691276,1.75110492558535,385.049240183392));
#38175=CARTESIAN_POINT('Ctrl Pts',(-3.87489664914265,2.44110792813221,385.022864224905));
#38176=CARTESIAN_POINT('Ctrl Pts',(-3.40964724164981,3.05747242764947,384.996488266419));
#38177=CARTESIAN_POINT('Ctrl Pts',(-2.82557507506063,3.52557726093145,384.970112307932));
#38178=CARTESIAN_POINT('Ctrl Pts',(-2.24150290847142,3.99368209421345,384.943736349446));
#38179=CARTESIAN_POINT('Ctrl Pts',(-1.53860798278584,4.31352726126017,384.917360390959));
#38180=CARTESIAN_POINT('Ctrl Pts',(-0.801987406950171,4.44639019055842,
384.890984432472));
#38181=CARTESIAN_POINT('Ctrl Pts',(-0.065366831114539,4.57925311985666,
384.864608473986));
#38182=CARTESIAN_POINT('Ctrl Pts',(0.7049793948712,4.52513381140646,384.838232515499));
#38183=CARTESIAN_POINT('Ctrl Pts',(1.41578806149518,4.29058430665667,384.811856557012));
#38184=CARTESIAN_POINT('Ctrl Pts',(2.12659672811916,4.05603480190689,384.785480598526));
#38185=CARTESIAN_POINT('Ctrl Pts',(2.77786783538139,3.64105510085751,384.759104640039));
#38186=CARTESIAN_POINT('Ctrl Pts',(3.29075419525559,3.09588539096791,384.732728681553));
#38187=CARTESIAN_POINT('Ctrl Pts',(3.8036405551298,2.55071568107831,384.706352723066));
#38188=CARTESIAN_POINT('Ctrl Pts',(4.178142167616,1.87535596234848,384.67997676458));
#38189=CARTESIAN_POINT('Ctrl Pts',(4.36891939039539,1.15156974944116,384.653600806093));
#38190=CARTESIAN_POINT('Ctrl Pts',(4.55969661317478,0.427783536533828,384.627224847606));
#38191=CARTESIAN_POINT('Ctrl Pts',(4.56674944624736,-0.344429170550942,
384.60084888912));
#38192=CARTESIAN_POINT('Ctrl Pts',(4.38922402699095,-1.07157919375385,384.574472930633));
#38193=CARTESIAN_POINT('Ctrl Pts',(4.21169860773453,-1.79872921695679,384.548096972147));
#38194=CARTESIAN_POINT('Ctrl Pts',(3.84959493614911,-2.48081655627781,384.52172101366));
#38195=CARTESIAN_POINT('Ctrl Pts',(3.34675167782285,-3.03526320680608,384.495345055174));
#38196=CARTESIAN_POINT('Ctrl Pts',(2.84390841949662,-3.58970985733432,384.468969096687));
#38197=CARTESIAN_POINT('Ctrl Pts',(2.20032557442955,-4.01651581906983,384.4425931382));
#38198=CARTESIAN_POINT('Ctrl Pts',(1.49391953877316,-4.26400913921072,384.416217179714));
#38199=CARTESIAN_POINT('Ctrl Pts',(0.787513503116781,-4.51150245935161,
384.389841221227));
#38200=CARTESIAN_POINT('Ctrl Pts',(0.0182842768710745,-4.57968313789789,
384.363465262741));
#38201=CARTESIAN_POINT('Ctrl Pts',(-0.720640161828923,-4.46029677092904,
384.337089304254));
#38202=CARTESIAN_POINT('Ctrl Pts',(-1.45956460052894,-4.34091040396018,
384.310713345767));
#38203=CARTESIAN_POINT('Ctrl Pts',(-2.16818425168326,-4.03395699147619,
384.284337387281));
#38204=CARTESIAN_POINT('Ctrl Pts',(-2.76070893321464,-3.57659834391139,
384.257961428794));
#38205=CARTESIAN_POINT('Ctrl Pts',(-3.35323361474601,-3.11923969634659,
384.231585470308));
#38206=CARTESIAN_POINT('Ctrl Pts',(-3.82966332665445,-2.51147581370097,
384.205209511821));
#38207=CARTESIAN_POINT('Ctrl Pts',(-4.13231833670975,-1.82688661161363,
384.178833553334));
#38208=CARTESIAN_POINT('Ctrl Pts',(-4.38571791578798,-1.25371052039765,
384.156750136387));
#38209=CARTESIAN_POINT('Ctrl Pts',(-4.51730198273802,-0.626680125117799,
384.134666719439));
#38210=CARTESIAN_POINT('Ctrl Pts',(-4.51791286673421,0.000101789655423226,
384.112583302492));
#38211=CARTESIAN_POINT('Ctrl Pts',(-4.51758348284472,-0.000105543616906456,
384.387416697508));
#38212=CARTESIAN_POINT('Ctrl Pts',(-4.51778471765472,-0.230920834279876,
384.395547309813));
#38213=CARTESIAN_POINT('Ctrl Pts',(-4.50040387332536,-0.461706099887457,
384.403677922118));
#38214=CARTESIAN_POINT('Ctrl Pts',(-4.46518027924831,-0.689735200724739,
384.411808534423));
#38215=CARTESIAN_POINT('Ctrl Pts',(-4.35091384761331,-1.42946867609407,
384.43818449291));
#38216=CARTESIAN_POINT('Ctrl Pts',(-4.04887500627456,-2.14019699767394,
384.464560451397));
#38217=CARTESIAN_POINT('Ctrl Pts',(-3.59563057517656,-2.73587469379764,
384.490936409884));
#38218=CARTESIAN_POINT('Ctrl Pts',(-3.14238614407856,-3.33155238992132,
384.51731236837));
#38219=CARTESIAN_POINT('Ctrl Pts',(-2.53793612322135,-3.81217946058886,
384.543688326857));
#38220=CARTESIAN_POINT('Ctrl Pts',(-1.85545923021652,-4.11956801355568,
384.570064285343));
#38221=CARTESIAN_POINT('Ctrl Pts',(-1.17298233721168,-4.42695656652252,
384.59644024383));
#38222=CARTESIAN_POINT('Ctrl Pts',(-0.412478572059261,-4.56110660178858,
384.622816202316));
#38223=CARTESIAN_POINT('Ctrl Pts',(0.333980449139521,-4.50577702875979,
384.649192160803));
#38224=CARTESIAN_POINT('Ctrl Pts',(1.08043947033828,-4.450447455731,384.67556811929));
#38225=CARTESIAN_POINT('Ctrl Pts',(1.81285374758341,-4.20563827440736,384.701944077776));
#38226=CARTESIAN_POINT('Ctrl Pts',(2.44255236397545,-3.80098770355085,384.728320036263));
#38227=CARTESIAN_POINT('Ctrl Pts',(3.0722509803675,-3.39633713269433,384.754695994749));
#38228=CARTESIAN_POINT('Ctrl Pts',(3.59923393590646,-2.83184517230493,384.781071953236));
#38229=CARTESIAN_POINT('Ctrl Pts',(3.95970118830781,-2.17585295289468,384.807447911723));
#38230=CARTESIAN_POINT('Ctrl Pts',(4.32016844070917,-1.51986073348444,384.833823870209));
#38231=CARTESIAN_POINT('Ctrl Pts',(4.51411998997293,-0.772368255053362,
384.860199828696));
#38232=CARTESIAN_POINT('Ctrl Pts',(4.51807477866807,-0.023871901270034,
384.886575787182));
#38233=CARTESIAN_POINT('Ctrl Pts',(4.52202956736322,0.724624452513337,384.912951745669));
#38234=CARTESIAN_POINT('Ctrl Pts',(4.33598759548973,1.47412468164896,384.939327704155));
#38235=CARTESIAN_POINT('Ctrl Pts',(3.98247233472248,2.13388933088782,384.965703662642));
#38236=CARTESIAN_POINT('Ctrl Pts',(3.62895707395525,2.79365398012665,384.992079621129));
#38237=CARTESIAN_POINT('Ctrl Pts',(3.10796852429429,3.36368304946875,385.018455579615));
#38238=CARTESIAN_POINT('Ctrl Pts',(2.48258100559898,3.77496504936747,385.044831538102));
#38239=CARTESIAN_POINT('Ctrl Pts',(1.8571934869037,4.18624704926618,385.071207496588));
#38240=CARTESIAN_POINT('Ctrl Pts',(1.12740699917409,4.43878197972154,385.097583455075));
#38241=CARTESIAN_POINT('Ctrl Pts',(0.38157432172954,4.50199629168033,385.123959413562));
#38242=CARTESIAN_POINT('Ctrl Pts',(-0.364258355715052,4.56521060363914,
385.150335372048));
#38243=CARTESIAN_POINT('Ctrl Pts',(-1.12613722287458,4.43910429710136,385.176711330535));
#38244=CARTESIAN_POINT('Ctrl Pts',(-1.81182418470336,4.13894463565663,385.203087289021));
#38245=CARTESIAN_POINT('Ctrl Pts',(-2.49751114653216,3.8387849742119,385.229463247508));
#38246=CARTESIAN_POINT('Ctrl Pts',(-3.1070062030302,3.36457195786021,385.255839205995));
#38247=CARTESIAN_POINT('Ctrl Pts',(-3.56651985120111,2.7737169510055,385.282215164481));
#38248=CARTESIAN_POINT('Ctrl Pts',(-4.02603349937199,2.18286194415082,385.308591122968));
#38249=CARTESIAN_POINT('Ctrl Pts',(-4.33556573921576,1.47536494679312,385.334967081454));
#38250=CARTESIAN_POINT('Ctrl Pts',(-4.45764255040047,0.736880225115328,
385.361343039941));
#38251=CARTESIAN_POINT('Ctrl Pts',(-4.49786843733614,0.493539965571841,
385.37003425913));
#38252=CARTESIAN_POINT('Ctrl Pts',(-4.51774064501623,0.246835097138747,
385.378725478319));
#38253=CARTESIAN_POINT('Ctrl Pts',(-4.51754236316255,9.86160820556914E-5,
385.387416697508));
#38254=CARTESIAN_POINT('Origin',(0.,0.,387.));
#38255=CARTESIAN_POINT('',(-4.51812581071634,-2.54303748789628E-5,386.387416697508));
#38256=CARTESIAN_POINT('',(-4.51739693228094,4.16105383547416E-5,386.112583302492));
#38257=CARTESIAN_POINT('',(-4.51775,5.53264807684796E-16,387.));
#38258=CARTESIAN_POINT('Ctrl Pts',(-4.51739693228094,4.16105383547416E-5,
386.112583302492));
#38259=CARTESIAN_POINT('Ctrl Pts',(-4.51750350848484,0.328257645647765,
386.101023056451));
#38260=CARTESIAN_POINT('Ctrl Pts',(-4.48221658085224,0.656451107309221,
386.08946281041));
#38261=CARTESIAN_POINT('Ctrl Pts',(-4.41129467440341,0.976754228647579,
386.077902564369));
#38262=CARTESIAN_POINT('Ctrl Pts',(-4.24947863228365,1.70756063203963,386.051526605882));
#38263=CARTESIAN_POINT('Ctrl Pts',(-3.90215620987833,2.39729198722953,386.025150647396));
#38264=CARTESIAN_POINT('Ctrl Pts',(-3.41137655698045,2.96244485418463,385.998774688909));
#38265=CARTESIAN_POINT('Ctrl Pts',(-2.92059690408257,3.52759772113973,385.972398730423));
#38266=CARTESIAN_POINT('Ctrl Pts',(-2.28636002069214,3.96817209986003,385.946022771936));
#38267=CARTESIAN_POINT('Ctrl Pts',(-1.58545081902196,4.23082914191337,385.91964681345));
#38268=CARTESIAN_POINT('Ctrl Pts',(-0.884541617351764,4.49348618396671,
385.893270854963));
#38269=CARTESIAN_POINT('Ctrl Pts',(-0.116960097401826,4.57822588935307,
385.866894896476));
#38270=CARTESIAN_POINT('Ctrl Pts',(0.624365244915622,4.47478910883432,385.84051893799));
#38271=CARTESIAN_POINT('Ctrl Pts',(1.36569058723307,4.37135232831557,385.814142979503));
#38272=CARTESIAN_POINT('Ctrl Pts',(2.08075975191802,4.07973906189171,385.787767021017));
#38273=CARTESIAN_POINT('Ctrl Pts',(2.68300173612543,3.63525394044883,385.76139106253));
#38274=CARTESIAN_POINT('Ctrl Pts',(3.28524372033282,3.19076881900596,385.735015104043));
#38275=CARTESIAN_POINT('Ctrl Pts',(3.77465852406267,2.5934118425441,385.708639145557));
#38276=CARTESIAN_POINT('Ctrl Pts',(4.09199435398004,1.91550299780405,385.68226318707));
#38277=CARTESIAN_POINT('Ctrl Pts',(4.4093301838974,1.23759415306402,385.655887228584));
#38278=CARTESIAN_POINT('Ctrl Pts',(4.55458704000229,0.479133440045757,385.629511270097));
#38279=CARTESIAN_POINT('Ctrl Pts',(4.51017916650468,-0.268054870554405,
385.60313531161));
#38280=CARTESIAN_POINT('Ctrl Pts',(4.46577129300707,-1.01524318115463,385.576759353124));
#38281=CARTESIAN_POINT('Ctrl Pts',(4.23169868990694,-1.7511590893368,385.550383394637));
#38282=CARTESIAN_POINT('Ctrl Pts',(3.83629973479027,-2.38670774759897,385.524007436151));
#38283=CARTESIAN_POINT('Ctrl Pts',(3.44090077967361,-3.0222564058611,385.497631477664));
#38284=CARTESIAN_POINT('Ctrl Pts',(2.88417547254044,-3.55743781420323,385.471255519177));
#38285=CARTESIAN_POINT('Ctrl Pts',(2.23352466148768,-3.92745937141648,385.444879560691));
#38286=CARTESIAN_POINT('Ctrl Pts',(1.58287385043492,-4.29748092862973,385.418503602204));
#38287=CARTESIAN_POINT('Ctrl Pts',(0.838297535462584,-4.5023426347141,385.392127643717));
#38288=CARTESIAN_POINT('Ctrl Pts',(0.0899390502021953,-4.5172425764895,
385.365751685231));
#38289=CARTESIAN_POINT('Ctrl Pts',(-0.658419435058194,-4.53214251826491,
385.339375726744));
#38290=CARTESIAN_POINT('Ctrl Pts',(-1.41056009060662,-4.35708069573135,
385.312999768258));
#38291=CARTESIAN_POINT('Ctrl Pts',(-2.07542379370768,-4.01325125105728,
385.286623809771));
#38292=CARTESIAN_POINT('Ctrl Pts',(-2.74028749680876,-3.6694218063832,385.260247851285));
#38293=CARTESIAN_POINT('Ctrl Pts',(-3.31787424746246,-3.15682473956861,
385.233871892798));
#38294=CARTESIAN_POINT('Ctrl Pts',(-3.73825757323288,-2.53751844205472,
385.207495934311));
#38295=CARTESIAN_POINT('Ctrl Pts',(-4.15864089900331,-1.91821214454083,
385.181119975825));
#38296=CARTESIAN_POINT('Ctrl Pts',(-4.42182079989046,-1.19219661632765,
385.154744017338));
#38297=CARTESIAN_POINT('Ctrl Pts',(-4.49593497631034,-0.44736809943281,
385.128368058852));
#38298=CARTESIAN_POINT('Ctrl Pts',(-4.51071957921785,-0.298786621658729,
385.123106473398));
#38299=CARTESIAN_POINT('Ctrl Pts',(-4.51798051524647,-0.149456501261902,
385.117844887945));
#38300=CARTESIAN_POINT('Ctrl Pts',(-4.51782825948384,-0.000111641905798056,
385.112583302492));
#38301=CARTESIAN_POINT('Ctrl Pts',(-4.51754236316255,9.86160820556914E-5,
385.387416697508));
#38302=CARTESIAN_POINT('Ctrl Pts',(-4.51713890274882,-0.501956417601758,
385.405101436806));
#38303=CARTESIAN_POINT('Ctrl Pts',(-4.43363680853372,-1.00414233826904,
385.422786176103));
#38304=CARTESIAN_POINT('Ctrl Pts',(-4.26942186585053,-1.47837968895145,
385.440470915401));
#38305=CARTESIAN_POINT('Ctrl Pts',(-4.02450298759024,-2.18568243534247,
385.466846873887));
#38306=CARTESIAN_POINT('Ctrl Pts',(-3.60004384854402,-2.83081548212662,
385.493222832374));
#38307=CARTESIAN_POINT('Ctrl Pts',(-3.04743227963612,-3.33567475547881,
385.519598790861));
#38308=CARTESIAN_POINT('Ctrl Pts',(-2.49482071072822,-3.84053402883101,
385.545974749347));
#38309=CARTESIAN_POINT('Ctrl Pts',(-1.81405671195863,-4.20511952875126,
385.572350707834));
#38310=CARTESIAN_POINT('Ctrl Pts',(-1.0875580758779,-4.38529212309734,385.59872666632));
#38311=CARTESIAN_POINT('Ctrl Pts',(-0.361059439797152,-4.56546471744342,
385.625102624807));
#38312=CARTESIAN_POINT('Ctrl Pts',(0.411173833594756,-4.56122440621533,
385.651478583294));
#38313=CARTESIAN_POINT('Ctrl Pts',(1.13565007634523,-4.37308454953753,385.67785454178));
#38314=CARTESIAN_POINT('Ctrl Pts',(1.86012631909569,-4.18494469285974,385.704230500267));
#38315=CARTESIAN_POINT('Ctrl Pts',(2.53684553120472,-3.81290529073225,385.730606458753));
#38316=CARTESIAN_POINT('Ctrl Pts',(3.08387960874885,-3.30200789400175,385.75698241724));
#38317=CARTESIAN_POINT('Ctrl Pts',(3.63091368629297,-2.79111049727125,385.783358375726));
#38318=CARTESIAN_POINT('Ctrl Pts',(4.04826262927219,-2.14135510593772,385.809734334213));
#38319=CARTESIAN_POINT('Ctrl Pts',(4.28539941412795,-1.43140540543153,385.8361102927));
#38320=CARTESIAN_POINT('Ctrl Pts',(4.52253619898372,-0.721455704925321,
385.862486251186));
#38321=CARTESIAN_POINT('Ctrl Pts',(4.57946082571602,0.048688304753508,385.888862209673));
#38322=CARTESIAN_POINT('Ctrl Pts',(4.44928162248921,0.785787895736858,385.915238168159));
#38323=CARTESIAN_POINT('Ctrl Pts',(4.31910241926241,1.52288748672023,385.941614126646));
#38324=CARTESIAN_POINT('Ctrl Pts',(4.00181938607647,2.22694265900807,385.967990085133));
#38325=CARTESIAN_POINT('Ctrl Pts',(3.53584490557238,2.81271583652609,385.994366043619));
#38326=CARTESIAN_POINT('Ctrl Pts',(3.06987042506831,3.39848901404408,386.020742002106));
#38327=CARTESIAN_POINT('Ctrl Pts',(2.45520449724608,3.86598019679227,386.047117960592));
#38328=CARTESIAN_POINT('Ctrl Pts',(1.76626264498691,4.1585918100038,386.073493919079));
#38329=CARTESIAN_POINT('Ctrl Pts',(1.07732079272774,4.45120342321533,386.099869877566));
#38330=CARTESIAN_POINT('Ctrl Pts',(0.3141030160316,4.56893546689021,386.126245836052));
#38331=CARTESIAN_POINT('Ctrl Pts',(-0.43099049281119,4.49753452109188,386.152621794539));
#38332=CARTESIAN_POINT('Ctrl Pts',(-1.17608400165398,4.42613357529356,386.178997753025));
#38333=CARTESIAN_POINT('Ctrl Pts',(-1.90305324264344,4.16559964002203,386.205373711512));
#38334=CARTESIAN_POINT('Ctrl Pts',(-2.52388651098497,3.74747467676233,386.231749669998));
#38335=CARTESIAN_POINT('Ctrl Pts',(-3.14471977932654,3.3293497135026,386.258125628485));
#38336=CARTESIAN_POINT('Ctrl Pts',(-3.65941707502018,2.75363372225468,386.284501586972));
#38337=CARTESIAN_POINT('Ctrl Pts',(-4.00566573902476,2.09002668894682,386.310877545458));
#38338=CARTESIAN_POINT('Ctrl Pts',(-4.34058663747219,1.44813002069409,386.336390596142));
#38339=CARTESIAN_POINT('Ctrl Pts',(-4.51790043884109,0.723999072118772,
386.361903646825));
#38340=CARTESIAN_POINT('Ctrl Pts',(-4.51812581071634,-2.54303748789628E-5,
386.387416697508));
#38341=CARTESIAN_POINT('Origin',(0.,0.,387.));
#38342=CARTESIAN_POINT('',(-4.51744020728156,-6.7888199640348E-5,387.387416697508));
#38343=CARTESIAN_POINT('',(-4.51807831563064,5.66723631286815E-5,387.112583302492));
#38344=CARTESIAN_POINT('',(-4.51775,5.53264807684796E-16,387.));
#38345=CARTESIAN_POINT('Ctrl Pts',(-4.51807831563064,5.66723631286815E-5,
387.112583302492));
#38346=CARTESIAN_POINT('Ctrl Pts',(-4.51811411951228,0.0569892498064094,
387.110577183443));
#38347=CARTESIAN_POINT('Ctrl Pts',(-4.51706018525489,0.113920500037806,
387.108571064395));
#38348=CARTESIAN_POINT('Ctrl Pts',(-4.51490790649659,0.170810197164546,
387.106564945346));
#38349=CARTESIAN_POINT('Ctrl Pts',(-4.4866102761939,0.918781904413813,387.08018898686));
#38350=CARTESIAN_POINT('Ctrl Pts',(-4.26844906050963,1.65957059993282,387.053813028373));
#38351=CARTESIAN_POINT('Ctrl Pts',(-3.88683629922459,2.30349150435396,387.027437069886));
#38352=CARTESIAN_POINT('Ctrl Pts',(-3.50522353793953,2.94741240877514,387.0010611114));
#38353=CARTESIAN_POINT('Ctrl Pts',(-2.96015923105368,3.49446552209844,386.974685152913));
#38354=CARTESIAN_POINT('Ctrl Pts',(-2.31763246884327,3.87842097598549,386.948309194426));
#38355=CARTESIAN_POINT('Ctrl Pts',(-1.67510570663291,4.26237642987252,386.92193323594));
#38356=CARTESIAN_POINT('Ctrl Pts',(-0.935116489098005,4.48323422432332,
386.895557277453));
#38357=CARTESIAN_POINT('Ctrl Pts',(-0.187252805513337,4.51425585389532,
386.869181318967));
#38358=CARTESIAN_POINT('Ctrl Pts',(0.560610878071331,4.54527748346732,386.84280536048));
#38359=CARTESIAN_POINT('Ctrl Pts',(1.31634902770576,4.38646294816051,386.816429401993));
#38360=CARTESIAN_POINT('Ctrl Pts',(1.98846698422516,4.05703938608529,386.790053443507));
#38361=CARTESIAN_POINT('Ctrl Pts',(2.66058494074455,3.72761582401007,386.76367748502));
#38362=CARTESIAN_POINT('Ctrl Pts',(3.2490827041489,3.22758323516643,386.737301526534));
#38363=CARTESIAN_POINT('Ctrl Pts',(3.68271284262869,2.6174788721857,386.710925568047));
#38364=CARTESIAN_POINT('Ctrl Pts',(4.1163429811085,2.00737450920494,386.684549609561));
#38365=CARTESIAN_POINT('Ctrl Pts',(4.39510549466373,1.28719837208709,386.658173651074));
#38366=CARTESIAN_POINT('Ctrl Pts',(4.48525154955086,0.544139747539571,386.631797692587));
#38367=CARTESIAN_POINT('Ctrl Pts',(4.57539760443799,-0.198918877007948,
386.605421734101));
#38368=CARTESIAN_POINT('Ctrl Pts',(4.47692720065701,-0.96485998898513,386.579045775614));
#38369=CARTESIAN_POINT('Ctrl Pts',(4.20176181661432,-1.66095369111926,386.552669817128));
#38370=CARTESIAN_POINT('Ctrl Pts',(3.92659643257165,-2.35704739325338,386.526293858641));
#38371=CARTESIAN_POINT('Ctrl Pts',(3.47473606826728,-2.98329368554445,386.499917900154));
#38372=CARTESIAN_POINT('Ctrl Pts',(2.90088592819845,-3.46387504959129,386.473541941668));
#38373=CARTESIAN_POINT('Ctrl Pts',(2.32703578812962,-3.94445641363812,386.447165983181));
#38374=CARTESIAN_POINT('Ctrl Pts',(1.63119587229633,-4.27937284944072,386.420790024695));
#38375=CARTESIAN_POINT('Ctrl Pts',(0.897609163487301,-4.4280771580026,386.394414066208));
#38376=CARTESIAN_POINT('Ctrl Pts',(0.164022454678273,-4.57678146656449,
386.368038107722));
#38377=CARTESIAN_POINT('Ctrl Pts',(-0.607311047106494,-4.53927364788568,
386.341662149235));
#38378=CARTESIAN_POINT('Ctrl Pts',(-1.32300860621665,-4.3200946465879,386.315286190748));
#38379=CARTESIAN_POINT('Ctrl Pts',(-2.03870616532682,-4.10091564529013,
386.288910232262));
#38380=CARTESIAN_POINT('Ctrl Pts',(-2.69876778176237,-3.7000654613734,386.262534273775));
#38381=CARTESIAN_POINT('Ctrl Pts',(-3.22328203031241,-3.16607366949443,
386.236158315289));
#38382=CARTESIAN_POINT('Ctrl Pts',(-3.74779627886247,-2.63208187761544,
386.209782356802));
#38383=CARTESIAN_POINT('Ctrl Pts',(-4.136763159527,-1.9649484777742,386.183406398315));
#38384=CARTESIAN_POINT('Ctrl Pts',(-4.34309176894218,-1.24544105205646,
386.157030439829));
#38385=CARTESIAN_POINT('Ctrl Pts',(-4.45898918165419,-0.84128454994014,
386.142214727383));
#38386=CARTESIAN_POINT('Ctrl Pts',(-4.51726034328579,-0.420602931019958,
386.127399014937));
#38387=CARTESIAN_POINT('Ctrl Pts',(-4.51739693228094,4.16105383547416E-5,
386.112583302492));
#38388=CARTESIAN_POINT('Ctrl Pts',(-4.51812581071634,-2.54303748789628E-5,
386.387416697508));
#38389=CARTESIAN_POINT('Ctrl Pts',(-4.51813343329163,-0.024513540432781,
386.388279605311));
#38390=CARTESIAN_POINT('Ctrl Pts',(-4.51793847697299,-0.049001528722538,
386.389142513115));
#38391=CARTESIAN_POINT('Ctrl Pts',(-4.51754018801501,-0.0734862094280138,
386.390005420918));
#38392=CARTESIAN_POINT('Ctrl Pts',(-4.50536594068517,-0.821893999127264,
386.416381379405));
#38393=CARTESIAN_POINT('Ctrl Pts',(-4.30321741370996,-1.56721150315799,
386.442757337891));
#38394=CARTESIAN_POINT('Ctrl Pts',(-3.9355680448604,-2.21920565463873,386.469133296378));
#38395=CARTESIAN_POINT('Ctrl Pts',(-3.56791867601083,-2.87119980611948,
386.495509254864));
#38396=CARTESIAN_POINT('Ctrl Pts',(-3.03476846528691,-3.42987060505022,
386.521885213351));
#38397=CARTESIAN_POINT('Ctrl Pts',(-2.40066410367865,-3.8275816692287,386.548261171838));
#38398=CARTESIAN_POINT('Ctrl Pts',(-1.76655974207041,-4.22529273340718,
386.574637130324));
#38399=CARTESIAN_POINT('Ctrl Pts',(-1.0315012295778,-4.46204406283341,386.601013088811));
#38400=CARTESIAN_POINT('Ctrl Pts',(-0.28447961170951,-4.50917297559413,
386.627389047297));
#38401=CARTESIAN_POINT('Ctrl Pts',(0.4625420061588,-4.55630188835485,386.653765005784));
#38402=CARTESIAN_POINT('Ctrl Pts',(1.22152672940277,-4.4138083844501,386.68014096427));
#38403=CARTESIAN_POINT('Ctrl Pts',(1.90058684718235,-4.09894366997453,386.706516922757));
#38404=CARTESIAN_POINT('Ctrl Pts',(2.57964696496189,-3.78407895549898,386.732892881244));
#38405=CARTESIAN_POINT('Ctrl Pts',(3.17878247727702,-3.29684303045261,386.75926883973));
#38406=CARTESIAN_POINT('Ctrl Pts',(3.62545807607245,-2.69622389870498,386.785644798217));
#38407=CARTESIAN_POINT('Ctrl Pts',(4.07213367486792,-2.0956047669573,386.812020756704));
#38408=CARTESIAN_POINT('Ctrl Pts',(4.3663493601437,-1.38160242850832,386.83839671519));
#38409=CARTESIAN_POINT('Ctrl Pts',(4.47248543497401,-0.64065872916252,386.864772673677));
#38410=CARTESIAN_POINT('Ctrl Pts',(4.57862150980431,0.10028497018324,386.891148632163));
#38411=CARTESIAN_POINT('Ctrl Pts',(4.49667797418915,0.868170030425805,386.91752459065));
#38412=CARTESIAN_POINT('Ctrl Pts',(4.23657545455911,1.57003120705739,386.943900549137));
#38413=CARTESIAN_POINT('Ctrl Pts',(3.97647293492907,2.27189238368897,386.970276507623));
#38414=CARTESIAN_POINT('Ctrl Pts',(3.53821143128416,2.90772967670955,386.99665246611));
#38415=CARTESIAN_POINT('Ctrl Pts',(2.97484978010159,3.40056441773073,387.023028424596));
#38416=CARTESIAN_POINT('Ctrl Pts',(2.41148812891902,3.8933991587519,387.049404383083));
#38417=CARTESIAN_POINT('Ctrl Pts',(1.72302633019879,4.24323134777366,387.07578034157));
#38418=CARTESIAN_POINT('Ctrl Pts',(0.992814123069943,4.40770798605575,387.102156300056));
#38419=CARTESIAN_POINT('Ctrl Pts',(0.262601915941074,4.57218462433785,387.128532258543));
#38420=CARTESIAN_POINT('Ctrl Pts',(-0.509360699596469,4.55130571188027,
387.154908217029));
#38421=CARTESIAN_POINT('Ctrl Pts',(-1.2296148232201,4.34759898792704,387.181284175516));
#38422=CARTESIAN_POINT('Ctrl Pts',(-1.94986894684372,4.14389226397381,387.207660134002));
#38423=CARTESIAN_POINT('Ctrl Pts',(-2.61841457855343,3.75735772852497,387.234036092489));
#38424=CARTESIAN_POINT('Ctrl Pts',(-3.15431316213248,3.23479180914392,387.260412050976));
#38425=CARTESIAN_POINT('Ctrl Pts',(-3.69021174571151,2.71222588976291,387.286788009462));
#38426=CARTESIAN_POINT('Ctrl Pts',(-4.09346328115986,2.05362858644968,387.313163967949));
#38427=CARTESIAN_POINT('Ctrl Pts',(-4.3152474703208,1.33873404498307,387.339539926435));
#38428=CARTESIAN_POINT('Ctrl Pts',(-4.4494392553304,0.906183036834296,387.355498850126));
#38429=CARTESIAN_POINT('Ctrl Pts',(-4.51719722678179,0.453022038514597,
387.371457773817));
#38430=CARTESIAN_POINT('Ctrl Pts',(-4.51744020728156,-6.7888199640348E-5,
387.387416697508));
#38431=CARTESIAN_POINT('Origin',(0.,0.,387.));
#38432=CARTESIAN_POINT('',(-4.51772665650122,0.000115440622527052,388.387416697508));
#38433=CARTESIAN_POINT('',(-4.51762944300479,-0.000110891096316518,388.112583302492));
#38434=CARTESIAN_POINT('',(-4.51775,5.53264807684796E-16,387.));
#38435=CARTESIAN_POINT('Ctrl Pts',(-4.51762944300479,-0.000110891096316518,
388.112583302492));
#38436=CARTESIAN_POINT('Ctrl Pts',(-4.51713192095981,0.534369387836516,
388.093755351949));
#38437=CARTESIAN_POINT('Ctrl Pts',(-4.42224443214638,1.0690216395804,388.074927401406));
#38438=CARTESIAN_POINT('Ctrl Pts',(-4.23657544981682,1.57003120529822,388.056099450863));
#38439=CARTESIAN_POINT('Ctrl Pts',(-3.97647293047822,2.27189238114416,388.029723492377));
#38440=CARTESIAN_POINT('Ctrl Pts',(-3.53821142732417,2.90772967345308,388.00334753389));
#38441=CARTESIAN_POINT('Ctrl Pts',(-2.97484977677246,3.40056441392273,387.976971575404));
#38442=CARTESIAN_POINT('Ctrl Pts',(-2.41148812622074,3.89339915439239,387.950595616917));
#38443=CARTESIAN_POINT('Ctrl Pts',(-1.72302632827134,4.24323134302276,387.924219658431));
#38444=CARTESIAN_POINT('Ctrl Pts',(-0.992814121960003,4.40770798112098,
387.897843699944));
#38445=CARTESIAN_POINT('Ctrl Pts',(-0.262601915648666,4.5721846192192,387.871467741457));
#38446=CARTESIAN_POINT('Ctrl Pts',(0.509360699024613,4.55130570678527,387.845091782971));
#38447=CARTESIAN_POINT('Ctrl Pts',(1.22961482184198,4.34759898306034,387.818715824484));
#38448=CARTESIAN_POINT('Ctrl Pts',(1.94986894465933,4.14389225933542,387.792339865998));
#38449=CARTESIAN_POINT('Ctrl Pts',(2.61841457562078,3.75735772431952,387.765963907511));
#38450=CARTESIAN_POINT('Ctrl Pts',(3.15431315860007,3.2347918055237,387.739587949024));
#38451=CARTESIAN_POINT('Ctrl Pts',(3.69021174157935,2.71222588672787,387.713211990538));
#38452=CARTESIAN_POINT('Ctrl Pts',(4.09346327657648,2.05362858415213,387.686836032051));
#38453=CARTESIAN_POINT('Ctrl Pts',(4.3152474654894,1.3387340434859,387.660460073565));
#38454=CARTESIAN_POINT('Ctrl Pts',(4.53703165440232,0.62383950281966,387.634084115078));
#38455=CARTESIAN_POINT('Ctrl Pts',(4.57734849723102,-0.147352275937061,
387.607708156591));
#38456=CARTESIAN_POINT('Ctrl Pts',(4.4313169703101,-0.881475715061101,387.581332198105));
#38457=CARTESIAN_POINT('Ctrl Pts',(4.28528544338918,-1.61559915418514,387.554956239618));
#38458=CARTESIAN_POINT('Ctrl Pts',(3.95290554671864,-2.3126542536765,387.528580281132));
#38459=CARTESIAN_POINT('Ctrl Pts',(3.47441738908987,-2.88825091257507,387.502204322645));
#38460=CARTESIAN_POINT('Ctrl Pts',(2.99592923146112,-3.46384757147362,387.475828364158));
#38461=CARTESIAN_POINT('Ctrl Pts',(2.37133281287417,-3.91798578977939,387.449452405672));
#38462=CARTESIAN_POINT('Ctrl Pts',(1.67624590710662,-4.19568459092305,387.423076447185));
#38463=CARTESIAN_POINT('Ctrl Pts',(0.981159001339069,-4.47338339206671,
387.396700488698));
#38464=CARTESIAN_POINT('Ctrl Pts',(0.215581608390928,-4.57464277604826,
387.370324530212));
#38465=CARTESIAN_POINT('Ctrl Pts',(-0.527800408696545,-4.48720361207072,
387.343948571725));
#38466=CARTESIAN_POINT('Ctrl Pts',(-1.27118242578404,-4.39976444809319,
387.317572613239));
#38467=CARTESIAN_POINT('Ctrl Pts',(-1.99236906701087,-4.12362673615656,
387.291196654752));
#38468=CARTESIAN_POINT('Ctrl Pts',(-2.60404870735825,-3.69222153415889,
387.264820696266));
#38469=CARTESIAN_POINT('Ctrl Pts',(-3.21572834770564,-3.26081633216121,
387.238444737779));
#38470=CARTESIAN_POINT('Ctrl Pts',(-3.71790098717359,-2.67414364010249,
387.212068779293));
#38471=CARTESIAN_POINT('Ctrl Pts',(-4.049770284447,-2.00322993458336,387.185692820806));
#38472=CARTESIAN_POINT('Ctrl Pts',(-4.35639806038402,-1.38334500078815,
387.161322981368));
#38473=CARTESIAN_POINT('Ctrl Pts',(-4.51764337890668,-0.691546237269266,
387.13695314193));
#38474=CARTESIAN_POINT('Ctrl Pts',(-4.51807831563064,5.66723631286815E-5,
387.112583302492));
#38475=CARTESIAN_POINT('Ctrl Pts',(-4.51744020728156,-6.7888199640348E-5,
387.387416697508));
#38476=CARTESIAN_POINT('Ctrl Pts',(-4.51759881047873,-0.295818004161051,
387.397833732304));
#38477=CARTESIAN_POINT('Ctrl Pts',(-4.48899129636465,-0.591537838638136,
387.408250767099));
#38478=CARTESIAN_POINT('Ctrl Pts',(-4.43131697527066,-0.881475716049439,
387.418667801895));
#38479=CARTESIAN_POINT('Ctrl Pts',(-4.28528544818601,-1.61559915599528,
387.445043760382));
#38480=CARTESIAN_POINT('Ctrl Pts',(-3.95290555114312,-2.31265425626688,
387.471419718868));
#38481=CARTESIAN_POINT('Ctrl Pts',(-3.47441739297849,-2.88825091580966,
387.497795677355));
#38482=CARTESIAN_POINT('Ctrl Pts',(-2.99592923481386,-3.46384757535244,
387.524171635842));
#38483=CARTESIAN_POINT('Ctrl Pts',(-2.37133281552749,-3.91798579416642,
387.550547594328));
#38484=CARTESIAN_POINT('Ctrl Pts',(-1.67624590898167,-4.19568459562072,
387.576923552815));
#38485=CARTESIAN_POINT('Ctrl Pts',(-0.981159002435877,-4.47338339707502,
387.603299511301));
#38486=CARTESIAN_POINT('Ctrl Pts',(-0.215581608630632,-4.57464278116965,
387.629675469788));
#38487=CARTESIAN_POINT('Ctrl Pts',(0.527800409289026,-4.48720361709396,
387.656051428274));
#38488=CARTESIAN_POINT('Ctrl Pts',(1.27118242720868,-4.39976445301828,387.682427386761));
#38489=CARTESIAN_POINT('Ctrl Pts',(1.99236906924277,-4.12362674077227,387.708803345248));
#38490=CARTESIAN_POINT('Ctrl Pts',(2.60404871027476,-3.69222153829144,387.735179303734));
#38491=CARTESIAN_POINT('Ctrl Pts',(3.21572835130679,-3.26081633581058,387.761555262221));
#38492=CARTESIAN_POINT('Ctrl Pts',(3.71790099133673,-2.67414364309488,387.787931220707));
#38493=CARTESIAN_POINT('Ctrl Pts',(4.04977028898144,-2.00322993682453,387.814307179194));
#38494=CARTESIAN_POINT('Ctrl Pts',(4.38163958662613,-1.33231623055421,387.840683137681));
#38495=CARTESIAN_POINT('Ctrl Pts',(4.54320554188561,-0.577161510729227,
387.867059096167));
#38496=CARTESIAN_POINT('Ctrl Pts',(4.51490791155097,0.170810197357385,387.893435054654));
#38497=CARTESIAN_POINT('Ctrl Pts',(4.48661028121633,0.918781905443997,387.919811013141));
#38498=CARTESIAN_POINT('Ctrl Pts',(4.26844906528759,1.65957060179219,387.946186971627));
#38499=CARTESIAN_POINT('Ctrl Pts',(3.88683630357511,2.30349150693406,387.972562930114));
#38500=CARTESIAN_POINT('Ctrl Pts',(3.50522354186264,2.94741241207594,387.9989388886));
#38501=CARTESIAN_POINT('Ctrl Pts',(2.96015923436644,3.49446552601145,388.025314847087));
#38502=CARTESIAN_POINT('Ctrl Pts',(2.31763247143664,3.87842098032811,388.051690805573));
#38503=CARTESIAN_POINT('Ctrl Pts',(1.67510570850681,4.2623764346448,388.07806676406));
#38504=CARTESIAN_POINT('Ctrl Pts',(0.935116490143367,4.48323422934263,388.104442722547));
#38505=CARTESIAN_POINT('Ctrl Pts',(0.187252805721414,4.5142558589491,388.130818681033));
#38506=CARTESIAN_POINT('Ctrl Pts',(-0.560610878700497,4.54527748855557,
388.15719463952));
#38507=CARTESIAN_POINT('Ctrl Pts',(-1.31634902918093,4.38646295307071,388.183570598006));
#38508=CARTESIAN_POINT('Ctrl Pts',(-1.98846698645264,4.05703939062647,388.209946556493));
#38509=CARTESIAN_POINT('Ctrl Pts',(-2.66058494372436,3.72761582818222,388.23632251498));
#38510=CARTESIAN_POINT('Ctrl Pts',(-3.24908270778736,3.22758323877859,388.262698473466));
#38511=CARTESIAN_POINT('Ctrl Pts',(-3.68271284675239,2.6174788751147,388.289074431953));
#38512=CARTESIAN_POINT('Ctrl Pts',(-4.11634298571743,2.00737451145079,388.315450390439));
#38513=CARTESIAN_POINT('Ctrl Pts',(-4.3951054995845,1.28719837352659,388.341826348926));
#38514=CARTESIAN_POINT('Ctrl Pts',(-4.48525155457229,0.544139748147192,
388.368202307413));
#38515=CARTESIAN_POINT('Ctrl Pts',(-4.50714145691119,0.363704999850856,
388.374607104111));
#38516=CARTESIAN_POINT('Ctrl Pts',(-4.51790959247399,0.181920986011914,
388.381011900809));
#38517=CARTESIAN_POINT('Ctrl Pts',(-4.51772665650122,0.000115440622527052,
388.387416697508));
#38518=CARTESIAN_POINT('Origin',(0.,0.,387.));
#38519=CARTESIAN_POINT('',(-4.51800421755028,-8.27334347235434E-5,389.387416697508));
#38520=CARTESIAN_POINT('',(-4.51750342669873,8.9713446903977E-5,389.112583302492));
#38521=CARTESIAN_POINT('',(-4.51775,5.53264807684796E-16,387.));
#38522=CARTESIAN_POINT('Ctrl Pts',(-4.51750342669873,8.9713446903977E-5,
389.112583302492));
#38523=CARTESIAN_POINT('Ctrl Pts',(-4.51769355714261,0.263372352578081,
389.103309478941));
#38524=CARTESIAN_POINT('Ctrl Pts',(-4.49505280568826,0.526622657629559,
389.094035655391));
#38525=CARTESIAN_POINT('Ctrl Pts',(-4.4492816175085,0.7857878948557,389.084761831841));
#38526=CARTESIAN_POINT('Ctrl Pts',(-4.31910241442768,1.52288748501391,389.058385873354));
#38527=CARTESIAN_POINT('Ctrl Pts',(-4.00181938159719,2.22694265651365,389.032009914867));
#38528=CARTESIAN_POINT('Ctrl Pts',(-3.53584490161497,2.81271583337604,389.005633956381));
#38529=CARTESIAN_POINT('Ctrl Pts',(-3.06987042163275,3.39848901023841,388.979257997894));
#38530=CARTESIAN_POINT('Ctrl Pts',(-2.45520449449881,3.86598019246346,388.952882039408));
#38531=CARTESIAN_POINT('Ctrl Pts',(-1.76626264301101,4.15859180534764,388.926506080921));
#38532=CARTESIAN_POINT('Ctrl Pts',(-1.07732079152318,4.45120341823184,388.900130122435));
#38533=CARTESIAN_POINT('Ctrl Pts',(-0.314103015681492,4.56893546177518,
388.873754163948));
#38534=CARTESIAN_POINT('Ctrl Pts',(0.430990492327212,4.49753451605703,388.847378205461));
#38535=CARTESIAN_POINT('Ctrl Pts',(1.1760840003359,4.42613357033888,388.821002246975));
#38536=CARTESIAN_POINT('Ctrl Pts',(1.90305324051159,4.16559963535927,388.794626288488));
#38537=CARTESIAN_POINT('Ctrl Pts',(2.52388650815824,3.74747467256786,388.768250330001));
#38538=CARTESIAN_POINT('Ctrl Pts',(3.14471977580489,3.32934970977646,388.741874371515));
#38539=CARTESIAN_POINT('Ctrl Pts',(3.65941707092249,2.75363371917326,388.715498413028));
#38540=CARTESIAN_POINT('Ctrl Pts',(4.00566573453967,2.09002668660847,388.689122454542));
#38541=CARTESIAN_POINT('Ctrl Pts',(4.35191439815685,1.42641965404367,388.662746496055));
#38542=CARTESIAN_POINT('Ctrl Pts',(4.52971443027359,0.67492157951728,388.636370537568));
#38543=CARTESIAN_POINT('Ctrl Pts',(4.51754018295765,-0.0734862093441271,
388.609994579082));
#38544=CARTESIAN_POINT('Ctrl Pts',(4.50536593564171,-0.821893998205556,
388.583618620595));
#38545=CARTESIAN_POINT('Ctrl Pts',(4.30321740889306,-1.567211501402,388.557242662109));
#38546=CARTESIAN_POINT('Ctrl Pts',(3.93556804045529,-2.21920565215297,388.530866703622));
#38547=CARTESIAN_POINT('Ctrl Pts',(3.56791867201753,-2.87119980290394,388.504490745136));
#38548=CARTESIAN_POINT('Ctrl Pts',(3.03476846189066,-3.42987060120944,388.478114786649));
#38549=CARTESIAN_POINT('Ctrl Pts',(2.40066410099242,-3.8275816649429,388.451738828162));
#38550=CARTESIAN_POINT('Ctrl Pts',(1.7665597400942,-4.22529272867635,388.425362869676));
#38551=CARTESIAN_POINT('Ctrl Pts',(1.03150122842463,-4.46204405783778,388.398986911189));
#38552=CARTESIAN_POINT('Ctrl Pts',(0.284479611392651,-4.509172970546,388.372610952703));
#38553=CARTESIAN_POINT('Ctrl Pts',(-0.462542005639328,-4.55630188325423,
388.346234994216));
#38554=CARTESIAN_POINT('Ctrl Pts',(-1.22152672803371,-4.41380837950926,
388.319859035729));
#38555=CARTESIAN_POINT('Ctrl Pts',(-1.90058684505317,-4.09894366538644,
388.293483077243));
#38556=CARTESIAN_POINT('Ctrl Pts',(-2.57964696207265,-3.78407895126361,
388.267107118756));
#38557=CARTESIAN_POINT('Ctrl Pts',(-3.17878247371721,-3.29684302676292,
388.24073116027));
#38558=CARTESIAN_POINT('Ctrl Pts',(-3.62545807201282,-2.6962238956878,388.214355201783));
#38559=CARTESIAN_POINT('Ctrl Pts',(-4.07213367030842,-2.09560476461269,
388.187979243296));
#38560=CARTESIAN_POINT('Ctrl Pts',(-4.36634935525508,-1.38160242696316,
388.16160328481));
#38561=CARTESIAN_POINT('Ctrl Pts',(-4.47248542996683,-0.640658728446904,
388.135227326323));
#38562=CARTESIAN_POINT('Ctrl Pts',(-4.50285839007941,-0.428622872948985,
388.127679318379));
#38563=CARTESIAN_POINT('Ctrl Pts',(-4.51782889648961,-0.2143807013974,388.120131310436));
#38564=CARTESIAN_POINT('Ctrl Pts',(-4.51762944300479,-0.000110891096316518,
388.112583302492));
#38565=CARTESIAN_POINT('Ctrl Pts',(-4.51772665650122,0.000115440622527052,
388.387416697508));
#38566=CARTESIAN_POINT('Ctrl Pts',(-4.51715623341347,-0.566782797039444,
388.407387859296));
#38567=CARTESIAN_POINT('Ctrl Pts',(-4.41010960182223,-1.13389038388221,
388.427359021084));
#38568=CARTESIAN_POINT('Ctrl Pts',(-4.20176182131765,-1.66095369298009,
388.447330182872));
#38569=CARTESIAN_POINT('Ctrl Pts',(-3.9265964369667,-2.35704739589339,388.473706141359));
#38570=CARTESIAN_POINT('Ctrl Pts',(-3.47473607215626,-2.9832936888854,388.500082099846));
#38571=CARTESIAN_POINT('Ctrl Pts',(-2.90088593144485,-3.46387505347005,
388.526458058332));
#38572=CARTESIAN_POINT('Ctrl Pts',(-2.32703579073342,-3.94445641805472,
388.552834016819));
#38573=CARTESIAN_POINT('Ctrl Pts',(-1.631195874121,-4.27937285423203,388.579209975305));
#38574=CARTESIAN_POINT('Ctrl Pts',(-0.897609164490652,-4.42807716296015,
388.605585933792));
#38575=CARTESIAN_POINT('Ctrl Pts',(-0.164022454860301,-4.57678147168827,
388.631961892278));
#38576=CARTESIAN_POINT('Ctrl Pts',(0.607311047787985,-4.53927365296719,
388.658337850765));
#38577=CARTESIAN_POINT('Ctrl Pts',(1.32300860769931,-4.32009465142378,388.684713809252));
#38578=CARTESIAN_POINT('Ctrl Pts',(2.03870616761062,-4.10091564988038,388.711089767738));
#38579=CARTESIAN_POINT('Ctrl Pts',(2.69876778478497,-3.70006546551466,388.737465726225));
#38580=CARTESIAN_POINT('Ctrl Pts',(3.22328203392201,-3.16607367303769,388.763841684711));
#38581=CARTESIAN_POINT('Ctrl Pts',(3.74779628305905,-2.63208188056073,388.790217643198));
#38582=CARTESIAN_POINT('Ctrl Pts',(4.13676316415879,-1.96494847997252,388.816593601685));
#38583=CARTESIAN_POINT('Ctrl Pts',(4.3430917738047,-1.24544105344924,388.842969560171));
#38584=CARTESIAN_POINT('Ctrl Pts',(4.54942038345061,-0.525933626925946,
388.869345518658));
#38585=CARTESIAN_POINT('Ctrl Pts',(4.57311072164268,0.245947825532416,388.895721477144));
#38586=CARTESIAN_POINT('Ctrl Pts',(4.41129467934152,0.976754229742574,388.922097435631));
#38587=CARTESIAN_POINT('Ctrl Pts',(4.24947863704035,1.70756063395273,388.948473394118));
#38588=CARTESIAN_POINT('Ctrl Pts',(3.90215621424595,2.39729198991468,388.974849352604));
#38589=CARTESIAN_POINT('Ctrl Pts',(3.41137656079843,2.96244485750231,389.001225311091));
#38590=CARTESIAN_POINT('Ctrl Pts',(2.92059690735092,3.52759772508993,389.027601269577));
#38591=CARTESIAN_POINT('Ctrl Pts',(2.2863600232503,3.96817210430322,389.053977228064));
#38592=CARTESIAN_POINT('Ctrl Pts',(1.58545082079536,4.23082914665035,389.08035318655));
#38593=CARTESIAN_POINT('Ctrl Pts',(0.88454161834042,4.49348618899748,389.106729145037));
#38594=CARTESIAN_POINT('Ctrl Pts',(0.116960097531164,4.57822589447844,389.133105103524));
#38595=CARTESIAN_POINT('Ctrl Pts',(-0.624365245616139,4.47478911384364,
389.15948106201));
#38596=CARTESIAN_POINT('Ctrl Pts',(-1.36569058876346,4.37135233320883,389.185857020497));
#38597=CARTESIAN_POINT('Ctrl Pts',(-2.08075975424883,4.07973906645826,389.212232978983));
#38598=CARTESIAN_POINT('Ctrl Pts',(-2.6830017391303,3.63525394451758,389.23860893747));
#38599=CARTESIAN_POINT('Ctrl Pts',(-3.28524372401176,3.19076882257689,389.264984895957));
#38600=CARTESIAN_POINT('Ctrl Pts',(-3.77465852828932,2.59341184544609,389.291360854443));
#38601=CARTESIAN_POINT('Ctrl Pts',(-4.09199435856171,1.91550299994699,389.31773681293));
#38602=CARTESIAN_POINT('Ctrl Pts',(-4.37143979921575,1.3185375205331,389.340963441123));
#38603=CARTESIAN_POINT('Ctrl Pts',(-4.51744597443699,0.659107802205375,
389.364190069315));
#38604=CARTESIAN_POINT('Ctrl Pts',(-4.51800421755028,-8.27334347235434E-5,
389.387416697508));
#38605=CARTESIAN_POINT('Origin',(0.,0.,387.));
#38606=CARTESIAN_POINT('',(-4.51737568732049,-1.26367906908009E-5,390.387416697508));
#38607=CARTESIAN_POINT('',(-4.51813713037119,-8.34916185418341E-6,390.112583302492));
#38608=CARTESIAN_POINT('',(-4.51775,5.53264807684796E-16,387.));
#38609=CARTESIAN_POINT('Ctrl Pts',(-4.5181365124173,-8.33583456870006E-6,
390.112583302492));
#38610=CARTESIAN_POINT('Ctrl Pts',(-4.51805642563476,0.740544543431,390.086487647447));
#38611=CARTESIAN_POINT('Ctrl Pts',(-4.33223070178982,1.48113615227849,390.060391992403));
#38612=CARTESIAN_POINT('Ctrl Pts',(-3.98247233026486,2.13388932849751,390.034296337358));
#38613=CARTESIAN_POINT('Ctrl Pts',(-3.62895706989363,2.79365397699786,390.007920378871));
#38614=CARTESIAN_POINT('Ctrl Pts',(-3.10796852081612,3.36368304570199,389.981544420385));
#38615=CARTESIAN_POINT('Ctrl Pts',(-2.48258100282108,3.7749650451405,389.955168461898));
#38616=CARTESIAN_POINT('Ctrl Pts',(-1.85719348482602,4.18624704457905,389.928792503412));
#38617=CARTESIAN_POINT('Ctrl Pts',(-1.12740699791342,4.43878197475195,389.902416544925));
#38618=CARTESIAN_POINT('Ctrl Pts',(-0.381574321303787,4.50199628664022,
389.876040586438));
#38619=CARTESIAN_POINT('Ctrl Pts',(0.364258355305801,4.56521059852849,389.849664627952));
#38620=CARTESIAN_POINT('Ctrl Pts',(1.12613722161242,4.43910429213214,389.823288669465));
#38621=CARTESIAN_POINT('Ctrl Pts',(1.81182418267365,4.13894463102368,389.796912710979));
#38622=CARTESIAN_POINT('Ctrl Pts',(2.49751114373488,3.83878496991522,389.770536752492));
#38623=CARTESIAN_POINT('Ctrl Pts',(3.10700619955072,3.36457195409465,389.744160794005));
#38624=CARTESIAN_POINT('Ctrl Pts',(3.56651984720739,2.7737169479016,389.717784835519));
#38625=CARTESIAN_POINT('Ctrl Pts',(4.02603349486408,2.18286194170853,389.691408877032));
#38626=CARTESIAN_POINT('Ctrl Pts',(4.33556573436158,1.47536494514296,389.665032918546));
#38627=CARTESIAN_POINT('Ctrl Pts',(4.45764254540988,0.736880224291923,389.638656960059));
#38628=CARTESIAN_POINT('Ctrl Pts',(4.57971935645818,-0.0016044965591186,
389.612281001572));
#38629=CARTESIAN_POINT('Ctrl Pts',(4.51434073905728,-0.77107694169564,389.585905043086));
#38630=CARTESIAN_POINT('Ctrl Pts',(4.26942186107142,-1.47837968729494,389.559529084599));
#38631=CARTESIAN_POINT('Ctrl Pts',(4.02450298308556,-2.18568243289422,389.533153126113));
#38632=CARTESIAN_POINT('Ctrl Pts',(3.60004384451474,-2.83081547895628,389.506777167626));
#38633=CARTESIAN_POINT('Ctrl Pts',(3.04743227622566,-3.33567475174347,389.480401209139));
#38634=CARTESIAN_POINT('Ctrl Pts',(2.49482070793658,-3.84053402453067,389.454025250653));
#38635=CARTESIAN_POINT('Ctrl Pts',(1.81405670992924,-4.205119524043,389.427649292166));
#38636=CARTESIAN_POINT('Ctrl Pts',(1.08755807466189,-4.38529211818763,389.40127333368));
#38637=CARTESIAN_POINT('Ctrl Pts',(0.361059439394515,-4.56546471233226,
389.374897375193));
#38638=CARTESIAN_POINT('Ctrl Pts',(-0.411173833132874,-4.56122440110918,
389.348521416706));
#38639=CARTESIAN_POINT('Ctrl Pts',(-1.13565007507237,-4.37308454464225,
389.32214545822));
#38640=CARTESIAN_POINT('Ctrl Pts',(-1.86012631701186,-4.18494468817533,
389.295769499733));
#38641=CARTESIAN_POINT('Ctrl Pts',(-2.53684552836345,-3.81290528646455,
389.269393541247));
#38642=CARTESIAN_POINT('Ctrl Pts',(-3.08387960529535,-3.30200789030617,
389.24301758276));
#38643=CARTESIAN_POINT('Ctrl Pts',(-3.63091368222724,-2.79111049414779,
389.216641624274));
#38644=CARTESIAN_POINT('Ctrl Pts',(-4.04826262473945,-2.14135510354181,
389.190265665787));
#38645=CARTESIAN_POINT('Ctrl Pts',(-4.28539940932997,-1.43140540383048,
389.1638897073));
#38646=CARTESIAN_POINT('Ctrl Pts',(-4.43915857188131,-0.971075002245244,
389.146787572364));
#38647=CARTESIAN_POINT('Ctrl Pts',(-4.51715280146967,-0.485437663288439,
389.129685437428));
#38648=CARTESIAN_POINT('Ctrl Pts',(-4.51750342669873,8.9713446903977E-5,
389.112583302492));
#38649=CARTESIAN_POINT('Ctrl Pts',(-4.51800421755028,-8.27334347235434E-5,
389.387416697508));
#38650=CARTESIAN_POINT('Ctrl Pts',(-4.51807991049777,-0.089463280026118,
389.390566027802));
#38651=CARTESIAN_POINT('Ctrl Pts',(-4.5154815404334,-0.178839429239229,
389.393715358096));
#38652=CARTESIAN_POINT('Ctrl Pts',(-4.51017917155373,-0.268054870856108,
389.39686468839));
#38653=CARTESIAN_POINT('Ctrl Pts',(-4.46577129800614,-1.01524318229275,
389.423240646876));
#38654=CARTESIAN_POINT('Ctrl Pts',(-4.23169869464373,-1.75115909129866,
389.449616605363));
#38655=CARTESIAN_POINT('Ctrl Pts',(-3.83629973908422,-2.38670775027215,
389.475992563849));
#38656=CARTESIAN_POINT('Ctrl Pts',(-3.4409007835247,-3.02225640924567,389.502368522336));
#38657=CARTESIAN_POINT('Ctrl Pts',(-2.88417547576807,-3.55743781818676,
389.528744480823));
#38658=CARTESIAN_POINT('Ctrl Pts',(-2.23352466398677,-3.92745937581404,
389.555120439309));
#38659=CARTESIAN_POINT('Ctrl Pts',(-1.58287385220546,-4.29748093344132,
389.581496397796));
#38660=CARTESIAN_POINT('Ctrl Pts',(-0.838297536399466,-4.50234263975477,
389.607872356282));
#38661=CARTESIAN_POINT('Ctrl Pts',(-0.0899390503012636,-4.51724258154659,
389.634248314769));
#38662=CARTESIAN_POINT('Ctrl Pts',(0.658419435796918,-4.53214252333841,
389.660624273256));
#38663=CARTESIAN_POINT('Ctrl Pts',(1.4105600921873,-4.3570807006086,389.687000231742));
#38664=CARTESIAN_POINT('Ctrl Pts',(2.07542379603256,-4.01325125554937,389.713376190229));
#38665=CARTESIAN_POINT('Ctrl Pts',(2.74028749987779,-3.66942181049016,389.739752148715));
#38666=CARTESIAN_POINT('Ctrl Pts',(3.31787425117789,-3.15682474310154,389.766128107202));
#38667=CARTESIAN_POINT('Ctrl Pts',(3.7382575774187,-2.53751844489424,389.792504065688));
#38668=CARTESIAN_POINT('Ctrl Pts',(4.15864090365956,-1.91821214668688,389.818880024175));
#38669=CARTESIAN_POINT('Ctrl Pts',(4.4218208048411,-1.19219661766082,389.845255982662));
#38670=CARTESIAN_POINT('Ctrl Pts',(4.4959349813437,-0.447368099932093,389.871631941148));
#38671=CARTESIAN_POINT('Ctrl Pts',(4.5700491578463,0.297460417796599,389.898007899635));
#38672=CARTESIAN_POINT('Ctrl Pts',(4.45509760966997,1.06110192422797,389.924383858122));
#38673=CARTESIAN_POINT('Ctrl Pts',(4.16499713157485,1.7511049275472,389.950759816608));
#38674=CARTESIAN_POINT('Ctrl Pts',(3.87489665347973,2.44110793086643,389.977135775095));
#38675=CARTESIAN_POINT('Ctrl Pts',(3.40964724546582,3.05747243107353,390.003511733581));
#38676=CARTESIAN_POINT('Ctrl Pts',(2.8255750782226,3.52557726487935,390.029887692068));
#38677=CARTESIAN_POINT('Ctrl Pts',(2.24150291097938,3.99368209868516,390.056263650554));
#38678=CARTESIAN_POINT('Ctrl Pts',(1.53860798450686,4.31352726608968,390.082639609041));
#38679=CARTESIAN_POINT('Ctrl Pts',(0.80198740784653,4.44639019553642,390.109015567528));
#38680=CARTESIAN_POINT('Ctrl Pts',(0.0653668311861832,4.57925312498317,
390.135391526014));
#38681=CARTESIAN_POINT('Ctrl Pts',(-0.704979395661959,4.52513381647212,
390.161767484501));
#38682=CARTESIAN_POINT('Ctrl Pts',(-1.41578806308163,4.2905843114595,390.188143442987));
#38683=CARTESIAN_POINT('Ctrl Pts',(-2.1265967305013,4.05603480644688,390.214519401474));
#38684=CARTESIAN_POINT('Ctrl Pts',(-2.7778678384925,3.64105510493269,390.240895359961));
#38685=CARTESIAN_POINT('Ctrl Pts',(-3.2907541989407,3.09588539443257,390.267271318447));
#38686=CARTESIAN_POINT('Ctrl Pts',(-3.8036405593889,2.55071568393247,390.293647276934));
#38687=CARTESIAN_POINT('Ctrl Pts',(-4.17814217229411,1.87535596444644,390.320023235421));
#38688=CARTESIAN_POINT('Ctrl Pts',(-4.36891939528681,1.15156975072878,390.346399193907));
#38689=CARTESIAN_POINT('Ctrl Pts',(-4.46781255254173,0.776380811874881,
390.360071695107));
#38690=CARTESIAN_POINT('Ctrl Pts',(-4.51733762799004,0.388179321285348,
390.373744196308));
#38691=CARTESIAN_POINT('Ctrl Pts',(-4.51737568732049,-1.26367906908009E-5,
390.387416697508));
#38692=CARTESIAN_POINT('Origin',(0.,0.,387.));
#38693=CARTESIAN_POINT('',(-4.51792755410097,9.93894350090341E-5,391.387416697508));
#38694=CARTESIAN_POINT('',(-4.51747010126728,-7.96701847477171E-5,391.112583302492));
#38695=CARTESIAN_POINT('',(-4.51775,5.53264807684796E-16,387.));
#38696=CARTESIAN_POINT('Ctrl Pts',(-4.51747010126728,-7.96701847477171E-5,
391.112583302492));
#38697=CARTESIAN_POINT('Ctrl Pts',(-4.51717195077355,0.469542077919004,
391.09604177444));
#38698=CARTESIAN_POINT('Ctrl Pts',(-4.44429158523714,0.939254240738123,
391.079500246387));
#38699=CARTESIAN_POINT('Ctrl Pts',(-4.30028579839415,1.38604169480228,391.062958718335));
#38700=CARTESIAN_POINT('Ctrl Pts',(-4.07066428800006,2.09845757944446,391.036582759848));
#38701=CARTESIAN_POINT('Ctrl Pts',(-3.66020460842122,2.75258681658163,391.010206801362));
#38702=CARTESIAN_POINT('Ctrl Pts',(-3.11859972342044,3.26923619408001,390.983830842875));
#38703=CARTESIAN_POINT('Ctrl Pts',(-2.57699483841966,3.78588557157838,390.957454884389));
#38704=CARTESIAN_POINT('Ctrl Pts',(-1.90424474799695,4.16505508943795,390.931078925902));
#38705=CARTESIAN_POINT('Ctrl Pts',(-1.181797027951,4.36083997783993,390.904702967415));
#38706=CARTESIAN_POINT('Ctrl Pts',(-0.459349307905077,4.55662486624191,
390.878327008929));
#38707=CARTESIAN_POINT('Ctrl Pts',(0.312796041764081,4.5690251251863,390.851951050442));
#38708=CARTESIAN_POINT('Ctrl Pts',(1.04115799773134,4.39653949730477,390.825575091955));
#38709=CARTESIAN_POINT('Ctrl Pts',(1.76951995369859,4.22405386942324,390.799199133469));
#38710=CARTESIAN_POINT('Ctrl Pts',(2.45409851596394,3.86668235471579,390.772823174982));
#38711=CARTESIAN_POINT('Ctrl Pts',(3.01201407568894,3.36769071255846,390.746447216496));
#38712=CARTESIAN_POINT('Ctrl Pts',(3.56992963541394,2.86869907040112,390.720071258009));
#38713=CARTESIAN_POINT('Ctrl Pts',(4.00118219259857,2.22808730079389,390.693695299523));
#38714=CARTESIAN_POINT('Ctrl Pts',(4.25356146018424,1.52341210184117,390.667319341036));
#38715=CARTESIAN_POINT('Ctrl Pts',(4.5059407277699,0.818736902888453,390.640943382549));
#38716=CARTESIAN_POINT('Ctrl Pts',(4.5794467057566,0.0499982745902433,390.614567424063));
#38717=CARTESIAN_POINT('Ctrl Pts',(4.46518027424979,-0.68973519995098,390.588191465576));
#38718=CARTESIAN_POINT('Ctrl Pts',(4.35091384274297,-1.42946867449225,390.56181550709));
#38719=CARTESIAN_POINT('Ctrl Pts',(4.04887500174263,-2.14019699527652,390.535439548603));
#38720=CARTESIAN_POINT('Ctrl Pts',(3.59563057115222,-2.73587469073354,390.509063590117));
#38721=CARTESIAN_POINT('Ctrl Pts',(3.14238614056185,-3.33155238619052,390.48268763163));
#38722=CARTESIAN_POINT('Ctrl Pts',(2.53793612038144,-3.81217945632025,390.456311673143));
#38723=CARTESIAN_POINT('Ctrl Pts',(1.85545922814075,-4.11956800894318,390.429935714657));
#38724=CARTESIAN_POINT('Ctrl Pts',(1.17298233590006,-4.42695656156612,390.40355975617));
#38725=CARTESIAN_POINT('Ctrl Pts',(0.412478571599103,-4.56110659668227,
390.377183797684));
#38726=CARTESIAN_POINT('Ctrl Pts',(-0.333980448764015,-4.50577702371569,
390.350807839197));
#38727=CARTESIAN_POINT('Ctrl Pts',(-1.08043946912713,-4.45044745074911,
390.32443188071));
#38728=CARTESIAN_POINT('Ctrl Pts',(-1.81285374555241,-4.2056382696998,390.298055922224));
#38729=CARTESIAN_POINT('Ctrl Pts',(-2.44255236123965,-3.80098769929651,
390.271679963737));
#38730=CARTESIAN_POINT('Ctrl Pts',(-3.07225097692695,-3.39633712889319,
390.245304005251));
#38731=CARTESIAN_POINT('Ctrl Pts',(-3.59923393187618,-2.83184516913586,
390.218928046764));
#38732=CARTESIAN_POINT('Ctrl Pts',(-3.95970118387424,-2.17585295046006,
390.192552088277));
#38733=CARTESIAN_POINT('Ctrl Pts',(-4.32016843587225,-1.51986073178434,
390.166176129791));
#38734=CARTESIAN_POINT('Ctrl Pts',(-4.51411998491911,-0.772368254190162,
390.139800171304));
#38735=CARTESIAN_POINT('Ctrl Pts',(-4.51807477361008,-0.0238719012447998,
390.113424212818));
#38736=CARTESIAN_POINT('Ctrl Pts',(-4.51811680206878,-0.0159174565147239,
390.113143909376));
#38737=CARTESIAN_POINT('Ctrl Pts',(-4.51813737266016,-0.00796289840890401,
390.112863605934));
#38738=CARTESIAN_POINT('Ctrl Pts',(-4.5181365124173,-8.33583456870006E-6,
390.112583302492));
#38739=CARTESIAN_POINT('Ctrl Pts',(-4.51737568732049,-1.26367906908009E-5,
390.387416697508));
#38740=CARTESIAN_POINT('Ctrl Pts',(-4.51741104918088,-0.360691336761726,
390.400120154794));
#38741=CARTESIAN_POINT('Ctrl Pts',(-4.47472562929359,-0.721361807575693,
390.412823612081));
#38742=CARTESIAN_POINT('Ctrl Pts',(-4.38922403190431,-1.07157919495506,
390.425527069367));
#38743=CARTESIAN_POINT('Ctrl Pts',(-4.2116986124489,-1.79872921897196,390.451903027853));
#38744=CARTESIAN_POINT('Ctrl Pts',(-3.84959494045787,-2.48081655905642,
390.47827898634));
#38745=CARTESIAN_POINT('Ctrl Pts',(-3.3467516815685,-3.03526321020521,390.504654944827));
#38746=CARTESIAN_POINT('Ctrl Pts',(-2.84390842267912,-3.589709861354,390.531030903313));
#38747=CARTESIAN_POINT('Ctrl Pts',(-2.2003255768914,-4.01651582356711,390.5574068618));
#38748=CARTESIAN_POINT('Ctrl Pts',(-1.49391954044408,-4.26400914398482,
390.583782820286));
#38749=CARTESIAN_POINT('Ctrl Pts',(-0.787513503996787,-4.51150246440253,
390.610158778773));
#38750=CARTESIAN_POINT('Ctrl Pts',(-0.018284276889904,-4.57968314302485,
390.636534737259));
#38751=CARTESIAN_POINT('Ctrl Pts',(0.720640162637278,-4.46029677592208,
390.662910695746));
#38752=CARTESIAN_POINT('Ctrl Pts',(1.45956460216448,-4.34091040881931,390.689286654233));
#38753=CARTESIAN_POINT('Ctrl Pts',(2.16818425411199,-4.03395699599143,390.715662612719));
#38754=CARTESIAN_POINT('Ctrl Pts',(2.76070893630653,-3.57659834791441,390.742038571206));
#38755=CARTESIAN_POINT('Ctrl Pts',(3.35323361850104,-3.11923969983741,390.768414529692));
#38756=CARTESIAN_POINT('Ctrl Pts',(3.8296633309426,-2.51147581651127,390.794790488179));
#38757=CARTESIAN_POINT('Ctrl Pts',(4.13231834133649,-1.82688661365747,390.821166446666));
#38758=CARTESIAN_POINT('Ctrl Pts',(4.43497335173039,-1.14229741080364,390.847542405152));
#38759=CARTESIAN_POINT('Ctrl Pts',(4.5638536600766,-0.380882888422163,390.873918363639));
#38760=CARTESIAN_POINT('Ctrl Pts',(4.50335616377816,0.365175075091525,390.900294322126));
#38761=CARTESIAN_POINT('Ctrl Pts',(4.44285866747971,1.11123303860522,390.926670280612));
#38762=CARTESIAN_POINT('Ctrl Pts',(4.1929833665366,1.84193444325112,390.953046239099));
#38763=CARTESIAN_POINT('Ctrl Pts',(3.78398181766136,2.46881574381626,390.979422197585));
#38764=CARTESIAN_POINT('Ctrl Pts',(3.37498026878612,3.0956970443814,391.005798156072));
#38765=CARTESIAN_POINT('Ctrl Pts',(2.80685247197875,3.61875824086581,391.032174114558));
#38766=CARTESIAN_POINT('Ctrl Pts',(2.14837973615702,3.97467408507625,391.058550073045));
#38767=CARTESIAN_POINT('Ctrl Pts',(1.48990700033531,4.33058992928668,391.084926031532));
#38768=CARTESIAN_POINT('Ctrl Pts',(0.74108932549923,4.51936042122317,391.111301990018));
#38769=CARTESIAN_POINT('Ctrl Pts',(-0.00741646764041988,4.51813175652443,
391.137677948505));
#38770=CARTESIAN_POINT('Ctrl Pts',(-0.75592226078007,4.51690309182569,391.164053906991));
#38771=CARTESIAN_POINT('Ctrl Pts',(-1.5041161722233,4.32567527049173,391.190429865478));
#38772=CARTESIAN_POINT('Ctrl Pts',(-2.16141689818149,3.96759959743449,391.216805823964));
#38773=CARTESIAN_POINT('Ctrl Pts',(-2.81871762413969,3.60952392437724,391.243181782451));
#38774=CARTESIAN_POINT('Ctrl Pts',(-3.38512516461286,3.0846003995967,391.269557740938));
#38775=CARTESIAN_POINT('Ctrl Pts',(-3.79206647629354,2.45637973706784,391.295933699424));
#38776=CARTESIAN_POINT('Ctrl Pts',(-4.19900778797422,1.82815907453898,391.322309657911));
#38777=CARTESIAN_POINT('Ctrl Pts',(-4.44648287086241,1.0966412742618,391.348685616397));
#38778=CARTESIAN_POINT('Ctrl Pts',(-4.50453075451936,0.350388719704337,
391.375061574884));
#38779=CARTESIAN_POINT('Ctrl Pts',(-4.51359442160846,0.233867939052437,
391.379179949092));
#38780=CARTESIAN_POINT('Ctrl Pts',(-4.51803983860459,0.116987923926286,
391.3832983233));
#38781=CARTESIAN_POINT('Ctrl Pts',(-4.51792755410097,9.93894350090341E-5,
391.387416697508));
#38782=CARTESIAN_POINT('Origin',(0.,0.,387.));
#38783=CARTESIAN_POINT('',(-4.51781275651133,-0.000112770352403077,392.387416697508));
#38784=CARTESIAN_POINT('',(-4.51767617872592,0.000114137193723671,392.112583302492));
#38785=CARTESIAN_POINT('',(-4.51775,5.53264807684796E-16,387.));
#38786=CARTESIAN_POINT('Ctrl Pts',(-4.51767617872592,0.000114137193723671,
392.112583302492));
#38787=CARTESIAN_POINT('Ctrl Pts',(-4.5178695555558,0.198463769522385,392.105595901432));
#38788=CARTESIAN_POINT('Ctrl Pts',(-4.5050469141142,0.396788584023774,392.098608500372));
#38789=CARTESIAN_POINT('Ctrl Pts',(-4.47900555811224,0.593362231693622,
392.091621099312));
#38790=CARTESIAN_POINT('Ctrl Pts',(-4.38070495693752,1.33538610094233,392.065245140825));
#38791=CARTESIAN_POINT('Ctrl Pts',(-4.0940505572316,2.05245754966054,392.038869182339));
#38792=CARTESIAN_POINT('Ctrl Pts',(-3.65374663667568,2.65776316525419,392.012493223852));
#38793=CARTESIAN_POINT('Ctrl Pts',(-3.21344271611974,3.26306878084786,391.986117265366));
#38794=CARTESIAN_POINT('Ctrl Pts',(-2.61948927471379,3.75660856331697,391.959741306879));
#38795=CARTESIAN_POINT('Ctrl Pts',(-1.94379424473237,4.07863132211605,391.933365348393));
#38796=CARTESIAN_POINT('Ctrl Pts',(-1.26809921475095,4.40065408091513,391.906989389906));
#38797=CARTESIAN_POINT('Ctrl Pts',(-0.510662596194056,4.55115981604418,
391.88061343142));
#38798=CARTESIAN_POINT('Ctrl Pts',(0.236815323891349,4.51192730770023,391.854237472933));
#38799=CARTESIAN_POINT('Ctrl Pts',(0.984293243976733,4.47269479935628,391.827861514446));
#38800=CARTESIAN_POINT('Ctrl Pts',(1.72181246559064,4.24372404753933,391.80148555596));
#38801=CARTESIAN_POINT('Ctrl Pts',(2.36008403350207,3.85273576597324,391.775109597473));
#38802=CARTESIAN_POINT('Ctrl Pts',(2.99835560141351,3.46174748440714,391.748733638986));
#38803=CARTESIAN_POINT('Ctrl Pts',(3.53737951562248,2.90874167309189,391.7223576805));
#38804=CARTESIAN_POINT('Ctrl Pts',(3.9118979757439,2.2606688733584,391.695981722013));
#38805=CARTESIAN_POINT('Ctrl Pts',(4.28641643586534,1.6125960736249,391.669605763527));
#38806=CARTESIAN_POINT('Ctrl Pts',(4.49642944189922,0.869456285473188,391.64322980504));
#38807=CARTESIAN_POINT('Ctrl Pts',(4.51651143022073,0.121218927096046,391.616853846553));
#38808=CARTESIAN_POINT('Ctrl Pts',(4.53659341854224,-0.627018431281127,
391.590477888067));
#38809=CARTESIAN_POINT('Ctrl Pts',(4.36674438915135,-1.3803533598837,391.56410192958));
#38810=CARTESIAN_POINT('Ctrl Pts',(4.02752738899906,-2.04758214938088,391.537725971094));
#38811=CARTESIAN_POINT('Ctrl Pts',(3.68831038884679,-2.71481093887802,391.511350012607));
#38812=CARTESIAN_POINT('Ctrl Pts',(3.17972541793314,-3.29593358926979,391.48497405412));
#38813=CARTESIAN_POINT('Ctrl Pts',(2.56334513683187,-3.72059554871007,391.458598095634));
#38814=CARTESIAN_POINT('Ctrl Pts',(1.94696485573061,-4.14525750815035,391.432222137147));
#38815=CARTESIAN_POINT('Ctrl Pts',(1.22278926444172,-4.41345877663913,391.405846178661));
#38816=CARTESIAN_POINT('Ctrl Pts',(0.478491850048684,-4.49272913461715,
391.379470220174));
#38817=CARTESIAN_POINT('Ctrl Pts',(-0.265805564344378,-4.57199949259517,
391.353094261688));
#38818=CARTESIAN_POINT('Ctrl Pts',(-1.03022480184161,-4.46233894006242,
391.326718303201));
#38819=CARTESIAN_POINT('Ctrl Pts',(-1.72222021336115,-4.17702370884953,
391.300342344714));
#38820=CARTESIAN_POINT('Ctrl Pts',(-2.41421562488067,-3.89170847763665,
391.273966386228));
#38821=CARTESIAN_POINT('Ctrl Pts',(-3.03378721042251,-3.43073856774365,
391.247590427741));
#38822=CARTESIAN_POINT('Ctrl Pts',(-3.50592553573386,-2.84992204551108,
391.221214469255));
#38823=CARTESIAN_POINT('Ctrl Pts',(-3.97806386104521,-2.26910552327851,
391.194838510768));
#38824=CARTESIAN_POINT('Ctrl Pts',(-4.30276892612607,-1.56844238870636,
391.168462552281));
#38825=CARTESIAN_POINT('Ctrl Pts',(-4.44072978806182,-0.83275955534669,
391.142086593795));
#38826=CARTESIAN_POINT('Ctrl Pts',(-4.4921693025746,-0.558455906816085,
391.13225216336));
#38827=CARTESIAN_POINT('Ctrl Pts',(-4.51764736060392,-0.279283767746957,
391.122417732926));
#38828=CARTESIAN_POINT('Ctrl Pts',(-4.51747010126728,-7.96701847477171E-5,
391.112583302492));
#38829=CARTESIAN_POINT('Ctrl Pts',(-4.51792755410097,9.93894350090341E-5,
391.387416697508));
#38830=CARTESIAN_POINT('Ctrl Pts',(-4.51732071711229,-0.631619894993005,
391.409674281787));
#38831=CARTESIAN_POINT('Ctrl Pts',(-4.38359173091614,-1.26358801454013,
391.431931866065));
#38832=CARTESIAN_POINT('Ctrl Pts',(-4.12629845673798,-1.84044304971073,
391.454189450344));
#38833=CARTESIAN_POINT('Ctrl Pts',(-3.82139759087395,-2.52403495573063,
391.48056540883));
#38834=CARTESIAN_POINT('Ctrl Pts',(-3.34297517472017,-3.13023145893271,
391.506941367317));
#38835=CARTESIAN_POINT('Ctrl Pts',(-2.74895219046335,-3.58564240100063,
391.533317325804));
#38836=CARTESIAN_POINT('Ctrl Pts',(-2.15492920620652,-4.04105334306855,
391.55969328429));
#38837=CARTESIAN_POINT('Ctrl Pts',(-1.44530565384664,-4.34567872400231,
391.586069242777));
#38838=CARTESIAN_POINT('Ctrl Pts',(-0.705993254381129,-4.46263858026562,
391.612445201263));
#38839=CARTESIAN_POINT('Ctrl Pts',(0.0333191450843864,-4.57959843652893,
391.63882115975));
#38840=CARTESIAN_POINT('Ctrl Pts',(0.802320391655539,-4.5088927681218,391.665197118237));
#38841=CARTESIAN_POINT('Ctrl Pts',(1.50791010792466,-4.25908167093864,391.691573076723));
#38842=CARTESIAN_POINT('Ctrl Pts',(2.21349982419377,-4.00927057375548,391.71794903521));
#38843=CARTESIAN_POINT('Ctrl Pts',(2.85567801016084,-3.58035404779628,391.744324993696));
#38844=CARTESIAN_POINT('Ctrl Pts',(3.35669832699602,-3.02425956472802,391.770700952183));
#38845=CARTESIAN_POINT('Ctrl Pts',(3.85771864383119,-2.46816508165977,391.79707691067));
#38846=CARTESIAN_POINT('Ctrl Pts',(4.21758109153447,-1.78489264148247,391.823452869156));
#38847=CARTESIAN_POINT('Ctrl Pts',(4.39271834190528,-1.05716372525534,391.849828827643));
#38848=CARTESIAN_POINT('Ctrl Pts',(4.56785559227609,-0.329434809028198,
391.876204786129));
#38849=CARTESIAN_POINT('Ctrl Pts',(4.55826764531442,0.442750583248765,391.902580744616));
#38850=CARTESIAN_POINT('Ctrl Pts',(4.36511528129817,1.16590658042746,391.928956703102));
#38851=CARTESIAN_POINT('Ctrl Pts',(4.17196291728192,1.88906257760614,391.955332661589));
#38852=CARTESIAN_POINT('Ctrl Pts',(3.79524613621108,2.56318917968655,391.981708620076));
#38853=CARTESIAN_POINT('Ctrl Pts',(3.28057276336538,3.10667216126389,392.008084578562));
#38854=CARTESIAN_POINT('Ctrl Pts',(2.76589939051967,3.65015514284124,392.034460537049));
#38855=CARTESIAN_POINT('Ctrl Pts',(2.11326942589908,4.0629945039155,392.060836495535));
#38856=CARTESIAN_POINT('Ctrl Pts',(1.40169456978973,4.29520918074182,392.087212454022));
#38857=CARTESIAN_POINT('Ctrl Pts',(0.690119713680387,4.52742385756813,392.113588412509));
#38858=CARTESIAN_POINT('Ctrl Pts',(-0.0804000339177079,4.57901385014649,
392.139964370995));
#38859=CARTESIAN_POINT('Ctrl Pts',(-0.816580455818562,4.44373333273746,
392.166340329482));
#38860=CARTESIAN_POINT('Ctrl Pts',(-1.55276087771942,4.30845281532842,392.192716287968));
#38861=CARTESIAN_POINT('Ctrl Pts',(-2.25460197392303,3.98630178793199,392.219092246455));
#38862=CARTESIAN_POINT('Ctrl Pts',(-2.83713421905071,3.51628198476719,392.245468204942));
#38863=CARTESIAN_POINT('Ctrl Pts',(-3.4196664641784,3.0462621816024,392.271844163428));
#38864=CARTESIAN_POINT('Ctrl Pts',(-3.88288985823016,2.42837360266924,392.298220121915));
#38865=CARTESIAN_POINT('Ctrl Pts',(-4.17072351316767,1.73742192630838,392.324596080401));
#38866=CARTESIAN_POINT('Ctrl Pts',(-4.3992382776818,1.18886668648237,392.345536286104));
#38867=CARTESIAN_POINT('Ctrl Pts',(-4.51720537865769,0.59425998006379,392.366476491806));
#38868=CARTESIAN_POINT('Ctrl Pts',(-4.51781275651133,-0.000112770352403077,
392.387416697508));
#38869=CARTESIAN_POINT('Origin',(0.,0.,387.));
#38870=CARTESIAN_POINT('',(-4.51740214664894,4.58334405226135E-5,393.387416697508));
#38871=CARTESIAN_POINT('',(-4.51804470017939,-7.02313581118758E-5,393.112583302492));
#38872=CARTESIAN_POINT('',(-4.51775,5.53264807684796E-16,387.));
#38873=CARTESIAN_POINT('Ctrl Pts',(-4.51804470017939,-7.02313581118758E-5,
393.112583302492));
#38874=CARTESIAN_POINT('Ctrl Pts',(-4.51753951069973,0.675637543377085,
393.088774069938));
#38875=CARTESIAN_POINT('Ctrl Pts',(-4.36387000533556,1.351567384844,393.064964837384));
#38876=CARTESIAN_POINT('Ctrl Pts',(-4.07071229568028,1.96032419089247,393.04115560483));
#38877=CARTESIAN_POINT('Ctrl Pts',(-3.74595106860983,2.63470729871608,393.014779646343));
#38878=CARTESIAN_POINT('Ctrl Pts',(-3.25000583346633,3.2266536908633,392.988403687856));
#38879=CARTESIAN_POINT('Ctrl Pts',(-2.64291900080672,3.66449842171826,392.96202772937));
#38880=CARTESIAN_POINT('Ctrl Pts',(-2.03583216814709,4.10234315257323,392.935651770883));
#38881=CARTESIAN_POINT('Ctrl Pts',(-1.31760373797134,4.38608622213596,392.909275812397));
#38882=CARTESIAN_POINT('Ctrl Pts',(-0.575187194701503,4.48137581760917,
392.88289985391));
#38883=CARTESIAN_POINT('Ctrl Pts',(0.167229348568301,4.57666541308236,392.856523895423));
#38884=CARTESIAN_POINT('Ctrl Pts',(0.933834004932164,4.48350153446603,392.830147936937));
#38885=CARTESIAN_POINT('Ctrl Pts',(1.63181654404497,4.21316321713056,392.80377197845));
#38886=CARTESIAN_POINT('Ctrl Pts',(2.32979908315777,3.94282489979509,392.777396019963));
#38887=CARTESIAN_POINT('Ctrl Pts',(2.95915950501951,3.49531214374047,392.751020061477));
#38888=CARTESIAN_POINT('Ctrl Pts',(3.44370327410501,2.92480380325231,392.72464410299));
#38889=CARTESIAN_POINT('Ctrl Pts',(3.92824704319053,2.35429546276414,392.698268144504));
#38890=CARTESIAN_POINT('Ctrl Pts',(4.26797415949979,1.66079153784243,392.671892186017));
#38891=CARTESIAN_POINT('Ctrl Pts',(4.42175501123433,0.928252200764915,392.64551622753));
#38892=CARTESIAN_POINT('Ctrl Pts',(4.57553586296886,0.195712863687411,392.619140269044));
#38893=CARTESIAN_POINT('Ctrl Pts',(4.54337045012868,-0.575861885545891,
392.592764310557));
#38894=CARTESIAN_POINT('Ctrl Pts',(4.32915293034778,-1.29306010427281,392.566388352071));
#38895=CARTESIAN_POINT('Ctrl Pts',(4.11493541056688,-2.01025832299973,392.540012393584));
#38896=CARTESIAN_POINT('Ctrl Pts',(3.71866578384527,-2.67308001122027,392.513636435098));
#38897=CARTESIAN_POINT('Ctrl Pts',(3.18831907228789,-3.20127959117695,392.487260476611));
#38898=CARTESIAN_POINT('Ctrl Pts',(2.65797236073051,-3.72947917113363,392.460884518124));
#38899=CARTESIAN_POINT('Ctrl Pts',(1.99354856433737,-4.12305664282645,392.434508559638));
#38900=CARTESIAN_POINT('Ctrl Pts',(1.27548722267832,-4.33436291424531,392.408132601151));
#38901=CARTESIAN_POINT('Ctrl Pts',(0.557425881019256,-4.54566918566418,
392.381756642665));
#38902=CARTESIAN_POINT('Ctrl Pts',(-0.214273005905716,-4.57470425680908,
392.355380684178));
#38903=CARTESIAN_POINT('Ctrl Pts',(-0.946182466504358,-4.41795294991702,
392.329004725691));
#38904=CARTESIAN_POINT('Ctrl Pts',(-1.678091927103,-4.26120164302497,392.302628767205));
#38905=CARTESIAN_POINT('Ctrl Pts',(-2.37021196137532,-3.91866395809597,
392.276252808718));
#38906=CARTESIAN_POINT('Ctrl Pts',(-2.93874993999921,-3.43180977295588,
392.249876850232));
#38907=CARTESIAN_POINT('Ctrl Pts',(-3.50728791862308,-2.9449555878158,392.223500891745));
#38908=CARTESIAN_POINT('Ctrl Pts',(-3.95224384159854,-2.31378490246464,
392.197124933258));
#38909=CARTESIAN_POINT('Ctrl Pts',(-4.21974840176451,-1.61471141489946,
392.170748974772));
#38910=CARTESIAN_POINT('Ctrl Pts',(-4.41638684920909,-1.1008333518145,392.151360417345));
#38911=CARTESIAN_POINT('Ctrl Pts',(-4.51713959899635,-0.550264065511563,
392.131971859919));
#38912=CARTESIAN_POINT('Ctrl Pts',(-4.51767617872592,0.000114137193723671,
392.112583302492));
#38913=CARTESIAN_POINT('Ctrl Pts',(-4.51781275651133,-0.000112770352403077,
392.387416697508));
#38914=CARTESIAN_POINT('Ctrl Pts',(-4.51797042238654,-0.154402722371687,
392.392852450292));
#38915=CARTESIAN_POINT('Ctrl Pts',(-4.51021990758361,-0.308676909473601,
392.398288203077));
#38916=CARTESIAN_POINT('Ctrl Pts',(-4.49444205643657,-0.462125713027313,
392.403723955861));
#38917=CARTESIAN_POINT('Ctrl Pts',(-4.41788302894468,-1.20670690221361,
392.430099914348));
#38918=CARTESIAN_POINT('Ctrl Pts',(-4.15232105813761,-1.93185450679764,
392.456475872834));
#38919=CARTESIAN_POINT('Ctrl Pts',(-3.72990683273987,-2.54977736133712,
392.482851831321));
#38920=CARTESIAN_POINT('Ctrl Pts',(-3.30749260734213,-3.16770021587658,
392.509227789807));
#38921=CARTESIAN_POINT('Ctrl Pts',(-2.72822612735372,-3.67839832037151,
392.535603748294));
#38922=CARTESIAN_POINT('Ctrl Pts',(-2.06223722435424,-4.02004318431961,
392.561979706781));
#38923=CARTESIAN_POINT('Ctrl Pts',(-1.39624832135474,-4.36168804826772,
392.588355665267));
#38924=CARTESIAN_POINT('Ctrl Pts',(-0.643536995344169,-4.53427967166901,
392.614731623754));
#38925=CARTESIAN_POINT('Ctrl Pts',(0.10476854180126,-4.5169229710009,392.64110758224));
#38926=CARTESIAN_POINT('Ctrl Pts',(0.853074078946657,-4.4995662703328,392.667483540727));
#38927=CARTESIAN_POINT('Ctrl Pts',(1.59697382722691,-4.29226124559533,392.693859499214));
#38928=CARTESIAN_POINT('Ctrl Pts',(2.24640636264933,-3.92010561428585,392.7202354577));
#38929=CARTESIAN_POINT('Ctrl Pts',(2.89583889807178,-3.54794998297635,392.746611416187));
#38930=CARTESIAN_POINT('Ctrl Pts',(3.45080422063637,-3.01094374509482,392.772987374673));
#38931=CARTESIAN_POINT('Ctrl Pts',(3.84411455761933,-2.37410042778438,392.79936333316));
#38932=CARTESIAN_POINT('Ctrl Pts',(4.23742489460227,-1.73725711047397,392.825739291647));
#38933=CARTESIAN_POINT('Ctrl Pts',(4.46908024600357,-1.00057671373466,392.852115250133));
#38934=CARTESIAN_POINT('Ctrl Pts',(4.51103488271665,-0.253246639109774,
392.87849120862));
#38935=CARTESIAN_POINT('Ctrl Pts',(4.55298951942973,0.494083435515108,392.904867167106));
#38936=CARTESIAN_POINT('Ctrl Pts',(4.40524344145459,1.25206318802556,392.931243125593));
#38937=CARTESIAN_POINT('Ctrl Pts',(4.0856837662456,1.92892657598571,392.95761908408));
#38938=CARTESIAN_POINT('Ctrl Pts',(3.76612409103661,2.60578996394588,392.983995042566));
#38939=CARTESIAN_POINT('Ctrl Pts',(3.27475081859377,3.20153698735573,393.010371001053));
#38940=CARTESIAN_POINT('Ctrl Pts',(2.67105284742856,3.64404257103983,393.03674695954));
#38941=CARTESIAN_POINT('Ctrl Pts',(2.06735487626337,4.08654815472391,393.063122918026));
#38942=CARTESIAN_POINT('Ctrl Pts',(1.35133220637582,4.37581229868225,393.089498876512));
#38943=CARTESIAN_POINT('Ctrl Pts',(0.60967127825766,4.4768147723325,393.115874834999));
#38944=CARTESIAN_POINT('Ctrl Pts',(-0.131989649860521,4.57781724598275,
393.142250793486));
#38945=CARTESIAN_POINT('Ctrl Pts',(-0.89928883620931,4.49055804932491,393.168626751973));
#38946=CARTESIAN_POINT('Ctrl Pts',(-1.5993319660497,4.2256013578754,393.195002710459));
#38947=CARTESIAN_POINT('Ctrl Pts',(-2.29937509589006,3.9606446664259,393.221378668946));
#38948=CARTESIAN_POINT('Ctrl Pts',(-2.93216216922203,3.51799048018475,393.247754627432));
#38949=CARTESIAN_POINT('Ctrl Pts',(-3.42108379742811,2.95122944283932,393.274130585919));
#38950=CARTESIAN_POINT('Ctrl Pts',(-3.91000542563421,2.38446840549387,393.300506544405));
#38951=CARTESIAN_POINT('Ctrl Pts',(-4.25506160871441,1.69360051704413,393.326882502892));
#38952=CARTESIAN_POINT('Ctrl Pts',(-4.41447756279827,0.962266813756684,
393.353258461379));
#38953=CARTESIAN_POINT('Ctrl Pts',(-4.4832948761755,0.646561770734553,393.364644540088));
#38954=CARTESIAN_POINT('Ctrl Pts',(-4.51751793652066,0.323315880315216,
393.376030618798));
#38955=CARTESIAN_POINT('Ctrl Pts',(-4.51740214664894,4.58334405226135E-5,
393.387416697508));
#38956=CARTESIAN_POINT('Origin',(0.,0.,387.));
#38957=CARTESIAN_POINT('',(-4.51808751818987,5.21912322906659E-5,394.387416697508));
#38958=CARTESIAN_POINT('',(-4.5173836733729,-2.76243915998559E-5,394.112583302492));
#38959=CARTESIAN_POINT('',(-4.51775,5.53264807684796E-16,387.));
#38960=CARTESIAN_POINT('Ctrl Pts',(-4.5173836733729,-2.76243915998559E-5,
394.112583302492));
#38961=CARTESIAN_POINT('Ctrl Pts',(-4.51729674156455,0.40470368583773,394.09832819693));
#38962=CARTESIAN_POINT('Ctrl Pts',(-4.46340651421681,0.809457698610517,
394.084073091368));
#38963=CARTESIAN_POINT('Ctrl Pts',(-4.35600985269673,1.19947809100869,394.069817985807));
#38964=CARTESIAN_POINT('Ctrl Pts',(-4.15729579382325,1.92112561822137,394.04344202732));
#38965=CARTESIAN_POINT('Ctrl Pts',(-3.77540022477979,2.59233198125928,394.017066068833));
#38966=CARTESIAN_POINT('Ctrl Pts',(-3.2565579491727,3.13183649817179,393.990690110347));
#38967=CARTESIAN_POINT('Ctrl Pts',(-2.7377156735656,3.6713410150843,393.96431415186));
#38968=CARTESIAN_POINT('Ctrl Pts',(-2.08192669139488,4.0791436858714,393.937938193374));
#38969=CARTESIAN_POINT('Ctrl Pts',(-1.36858515450633,4.30587322182919,393.911562234887));
#38970=CARTESIAN_POINT('Ctrl Pts',(-0.655243617617784,4.53260275778698,
393.885186276401));
#38971=CARTESIAN_POINT('Ctrl Pts',(0.115650473988585,4.57825915891545,393.858810317914));
#38972=CARTESIAN_POINT('Ctrl Pts',(0.850767582565068,4.43731495930334,393.832434359427));
#38973=CARTESIAN_POINT('Ctrl Pts',(1.58588469114154,4.29637075969123,393.806058400941));
#38974=CARTESIAN_POINT('Ctrl Pts',(2.28522481668813,3.96882595933856,393.779682442454));
#38975=CARTESIAN_POINT('Ctrl Pts',(2.86412121787636,3.49433529829511,393.753306483967));
#38976=CARTESIAN_POINT('Ctrl Pts',(3.44301761906461,3.01984463725166,393.726930525481));
#38977=CARTESIAN_POINT('Ctrl Pts',(3.9014702958945,2.39840811551743,393.700554566994));
#38978=CARTESIAN_POINT('Ctrl Pts',(4.18397593491012,1.70526094885616,393.674178608508));
#38979=CARTESIAN_POINT('Ctrl Pts',(4.46648157392573,1.0121137821949,393.647802650021));
#38980=CARTESIAN_POINT('Ctrl Pts',(4.57304017512708,0.247255970606617,393.621426691535));
#38981=CARTESIAN_POINT('Ctrl Pts',(4.49075104942932,-0.496713740146479,
393.595050733048));
#38982=CARTESIAN_POINT('Ctrl Pts',(4.40846192373155,-1.24068345089957,393.568674774561));
#38983=CARTESIAN_POINT('Ctrl Pts',(4.13732507113467,-1.96376506081748,393.542298816075));
#38984=CARTESIAN_POINT('Ctrl Pts',(3.71016611242726,-2.57841752743756,393.515922857588));
#38985=CARTESIAN_POINT('Ctrl Pts',(3.28300715371985,-3.19306999405764,393.489546899101));
#38986=CARTESIAN_POINT('Ctrl Pts',(2.69982608890194,-3.69929331737988,393.463170940615));
#38987=CARTESIAN_POINT('Ctrl Pts',(2.03122667508525,-4.03580075350889,393.436794982129));
#38988=CARTESIAN_POINT('Ctrl Pts',(1.36262726126856,-4.37230818963791,393.410419023642));
#38989=CARTESIAN_POINT('Ctrl Pts',(0.60860949845307,-4.53909973857368,393.384043065155));
#38990=CARTESIAN_POINT('Ctrl Pts',(-0.139540235604001,-4.51598251217256,
393.357667106668));
#38991=CARTESIAN_POINT('Ctrl Pts',(-0.887689969661061,-4.49286528577144,
393.331291148182));
#38992=CARTESIAN_POINT('Ctrl Pts',(-1.62997167495974,-4.27983928403344,
393.304915189695));
#38993=CARTESIAN_POINT('Ctrl Pts',(-2.2765198184931,-3.90269484377256,393.278539231209));
#38994=CARTESIAN_POINT('Ctrl Pts',(-2.92306796202647,-3.52555040351167,
393.252163272722));
#38995=CARTESIAN_POINT('Ctrl Pts',(-3.47388254379453,-2.9842875247279,393.225787314236));
#38996=CARTESIAN_POINT('Ctrl Pts',(-3.86227830720905,-2.3444350716672,393.199411355749));
#38997=CARTESIAN_POINT('Ctrl Pts',(-4.25067407062357,-1.7045826186065,393.173035397262));
#38998=CARTESIAN_POINT('Ctrl Pts',(-4.47665101568456,-0.966140591268864,
393.146659438776));
#38999=CARTESIAN_POINT('Ctrl Pts',(-4.51285087871635,-0.218509665850027,
393.120283480289));
#39000=CARTESIAN_POINT('Ctrl Pts',(-4.51637359912257,-0.145755392857762,
393.117716754357));
#39001=CARTESIAN_POINT('Ctrl Pts',(-4.51809916152901,-0.0729141025000744,
393.115150028424));
#39002=CARTESIAN_POINT('Ctrl Pts',(-4.51804470017939,-7.02313581118758E-5,
393.112583302492));
#39003=CARTESIAN_POINT('Ctrl Pts',(-4.51740214664894,4.58334405226135E-5,
393.387416697508));
#39004=CARTESIAN_POINT('Ctrl Pts',(-4.51724970819312,-0.425542225591553,
393.402406577285));
#39005=CARTESIAN_POINT('Ctrl Pts',(-4.4575812765459,-0.851172152520294,
393.417396457061));
#39006=CARTESIAN_POINT('Ctrl Pts',(-4.33897962224013,-1.25969258594773,
393.432386336838));
#39007=CARTESIAN_POINT('Ctrl Pts',(-4.13029000251061,-1.97851876423963,
393.458762295325));
#39008=CARTESIAN_POINT('Ctrl Pts',(-3.73913503796403,-2.64437160269829,
393.485138253812));
#39009=CARTESIAN_POINT('Ctrl Pts',(-3.21287053587191,-3.1766385524691,393.511514212298));
#39010=CARTESIAN_POINT('Ctrl Pts',(-2.68660603377979,-3.7089055022399,393.537890170785));
#39011=CARTESIAN_POINT('Ctrl Pts',(-2.02523199414213,-4.10758656332286,
393.564266129271));
#39012=CARTESIAN_POINT('Ctrl Pts',(-1.3088187328036,-4.324414769419,393.590642087758));
#39013=CARTESIAN_POINT('Ctrl Pts',(-0.592405471465078,-4.54124297551514,
393.617018046244));
#39014=CARTESIAN_POINT('Ctrl Pts',(0.179047011574318,-4.57621832662447,
393.643394004731));
#39015=CARTESIAN_POINT('Ctrl Pts',(0.912141576006553,-4.42510647540001,
393.669769963218));
#39016=CARTESIAN_POINT('Ctrl Pts',(1.6452361404388,-4.27399462417554,393.696145921704));
#39017=CARTESIAN_POINT('Ctrl Pts',(2.33997278626389,-3.93679557061728,393.722521880191));
#39018=CARTESIAN_POINT('Ctrl Pts',(2.91224209985778,-3.45433286252538,393.748897838677));
#39019=CARTESIAN_POINT('Ctrl Pts',(3.48451141345166,-2.97187015443348,393.775273797164));
#39020=CARTESIAN_POINT('Ctrl Pts',(3.93431339481433,-2.34414379180799,393.801649755651));
#39021=CARTESIAN_POINT('Ctrl Pts',(4.20719204090252,-1.64715048015453,393.828025714137));
#39022=CARTESIAN_POINT('Ctrl Pts',(4.48007068699071,-0.950157168501087,
393.854401672624));
#39023=CARTESIAN_POINT('Ctrl Pts',(4.5760259978044,-0.183896907819673,393.88077763111));
#39024=CARTESIAN_POINT('Ctrl Pts',(4.48344098872769,0.558861766363823,393.907153589597));
#39025=CARTESIAN_POINT('Ctrl Pts',(4.39085597965098,1.30162044054734,393.933529548083));
#39026=CARTESIAN_POINT('Ctrl Pts',(4.10973065068387,2.02087752823294,393.95990550657));
#39027=CARTESIAN_POINT('Ctrl Pts',(3.67409989363231,2.62955500891649,393.986281465057));
#39028=CARTESIAN_POINT('Ctrl Pts',(3.23846913658077,3.23823248960003,394.012657423543));
#39029=CARTESIAN_POINT('Ctrl Pts',(2.64833295144478,3.73633036328149,394.03903338203));
#39030=CARTESIAN_POINT('Ctrl Pts',(1.97513712820591,4.06354560674411,394.065409340517));
#39031=CARTESIAN_POINT('Ctrl Pts',(1.30194130496704,4.39076085020672,394.091785299003));
#39032=CARTESIAN_POINT('Ctrl Pts',(0.54568584362529,4.54709346345051,394.11816125749));
#39033=CARTESIAN_POINT('Ctrl Pts',(-0.202071967477526,4.51361678626648,
394.144537215976));
#39034=CARTESIAN_POINT('Ctrl Pts',(-0.949829778580352,4.48014010908246,
394.170913174463));
#39035=CARTESIAN_POINT('Ctrl Pts',(-1.68908993944425,4.25685414147062,394.19728913295));
#39036=CARTESIAN_POINT('Ctrl Pts',(-2.33035272521732,3.8707913595774,394.223665091436));
#39037=CARTESIAN_POINT('Ctrl Pts',(-2.97161551099039,3.48472857768417,394.250041049923));
#39038=CARTESIAN_POINT('Ctrl Pts',(-3.51488092167263,2.93588898150954,394.276417008409));
#39039=CARTESIAN_POINT('Ctrl Pts',(-3.89437765326087,2.29071872282242,394.302792966896));
#39040=CARTESIAN_POINT('Ctrl Pts',(-4.27387438484911,1.64554846413529,394.329168925382));
#39041=CARTESIAN_POINT('Ctrl Pts',(-4.48960243734335,0.904047542935649,
394.355544883869));
#39042=CARTESIAN_POINT('Ctrl Pts',(-4.51544434579255,0.15598696534298,394.381920842355));
#39043=CARTESIAN_POINT('Ctrl Pts',(-4.51723920487186,0.104030147904069,
394.383752794073));
#39044=CARTESIAN_POINT('Ctrl Pts',(-4.51811804423603,0.0520416863733224,
394.38558474579));
#39045=CARTESIAN_POINT('Ctrl Pts',(-4.51808751818987,5.21912322906659E-5,
394.387416697508));
#39046=CARTESIAN_POINT('Origin',(0.,0.,387.));
#39047=CARTESIAN_POINT('',(-4.51761539860092,-0.000109498206778275,395.387416697508));
#39048=CARTESIAN_POINT('',(-4.51787769339044,0.000106674156513836,395.112583302492));
#39049=CARTESIAN_POINT('',(-4.51775,5.53264807684796E-16,387.));
#39050=CARTESIAN_POINT('Ctrl Pts',(-4.51787769339044,0.000106674156513836,
395.112583302492));
#39051=CARTESIAN_POINT('Ctrl Pts',(-4.51801115526906,0.13353505519604,395.107882323922));
#39052=CARTESIAN_POINT('Ctrl Pts',(-4.51221712826522,0.266951885784635,
395.103181345353));
#39053=CARTESIAN_POINT('Ctrl Pts',(-4.50041129427044,0.39983460330973,395.098480366784));
#39054=CARTESIAN_POINT('Ctrl Pts',(-4.43417185438628,1.14540469882723,395.072104408297));
#39055=CARTESIAN_POINT('Ctrl Pts',(-4.17867844925679,1.87416071243738,395.04572844981));
#39056=CARTESIAN_POINT('Ctrl Pts',(-3.76486280044783,2.49787462083366,395.019352491324));
#39057=CARTESIAN_POINT('Ctrl Pts',(-3.35104715163886,3.12158852922995,394.992976532837));
#39058=CARTESIAN_POINT('Ctrl Pts',(-2.77890925915041,3.64026033241238,394.966600574351));
#39059=CARTESIAN_POINT('Ctrl Pts',(-2.11771592060786,3.99109619117415,394.940224615864));
#39060=CARTESIAN_POINT('Ctrl Pts',(-1.45652258206532,4.34193204993591,394.913848657377));
#39061=CARTESIAN_POINT('Ctrl Pts',(-0.706273797468684,4.52493196427704,
394.887472698891));
#39062=CARTESIAN_POINT('Ctrl Pts',(0.0422003528576968,4.51794075412897,
394.861096740404));
#39063=CARTESIAN_POINT('Ctrl Pts',(0.790674503184078,4.51094954398091,394.834720781918));
#39064=CARTESIAN_POINT('Ctrl Pts',(1.5373740192402,4.31396720934364,394.808344823431));
#39065=CARTESIAN_POINT('Ctrl Pts',(2.19189851862757,3.9508417345724,394.781968864945));
#39066=CARTESIAN_POINT('Ctrl Pts',(2.84642301801496,3.58771625980115,394.755592906458));
#39067=CARTESIAN_POINT('Ctrl Pts',(3.4087725007336,3.05844764489591,394.729216947971));
#39068=CARTESIAN_POINT('Ctrl Pts',(3.81086521878951,2.4271126491824,394.702840989485));
#39069=CARTESIAN_POINT('Ctrl Pts',(4.2129579368454,1.79577765346891,394.676465030998));
#39070=CARTESIAN_POINT('Ctrl Pts',(4.45479389023857,1.06237627694715,394.650089072511));
#39071=CARTESIAN_POINT('Ctrl Pts',(4.50709481884649,0.315698941284091,394.623713114025));
#39072=CARTESIAN_POINT('Ctrl Pts',(4.55939574745442,-0.430978394378985,
394.597337155538));
#39073=CARTESIAN_POINT('Ctrl Pts',(4.4221616512771,-1.19093168918336,394.570961197052));
#39074=CARTESIAN_POINT('Ctrl Pts',(4.11200699772181,-1.8721559706092,394.544585238565));
#39075=CARTESIAN_POINT('Ctrl Pts',(3.80185234416652,-2.55338025203503,394.518209280079));
#39076=CARTESIAN_POINT('Ctrl Pts',(3.31877713323327,-3.15587552008233,394.491833321592));
#39077=CARTESIAN_POINT('Ctrl Pts',(2.72126564522031,-3.60669971244412,394.465457363105));
#39078=CARTESIAN_POINT('Ctrl Pts',(2.12375415720733,-4.05752390480593,394.439081404619));
#39079=CARTESIAN_POINT('Ctrl Pts',(1.41180639211463,-4.35667702148223,394.412705446132));
#39080=CARTESIAN_POINT('Ctrl Pts',(0.67161545550637,-4.46794160744361,394.386329487646));
#39081=CARTESIAN_POINT('Ctrl Pts',(-0.0685754811018632,-4.57920619340499,
394.359953529159));
#39082=CARTESIAN_POINT('Ctrl Pts',(-0.837009589225651,-4.50258224865146,
394.333577570673));
#39083=CARTESIAN_POINT('Ctrl Pts',(-1.54065515298906,-4.2473463747579,394.307201612186));
#39084=CARTESIAN_POINT('Ctrl Pts',(-2.24430071675247,-3.99211050086433,
394.280825653699));
#39085=CARTESIAN_POINT('Ctrl Pts',(-2.88315773615551,-3.55826269783073,
394.254449695213));
#39086=CARTESIAN_POINT('Ctrl Pts',(-3.37988195476012,-2.99832745034422,
394.228073736726));
#39087=CARTESIAN_POINT('Ctrl Pts',(-3.87660617336475,-2.43839220285771,
394.20169777824));
#39088=CARTESIAN_POINT('Ctrl Pts',(-4.23119759117096,-1.75236951091828,
394.175321819753));
#39089=CARTESIAN_POINT('Ctrl Pts',(-4.40072702572232,-1.02331381925484,
394.148945861266));
#39090=CARTESIAN_POINT('Ctrl Pts',(-4.47863287106505,-0.688282323920289,
394.136825008341));
#39091=CARTESIAN_POINT('Ctrl Pts',(-4.51745758988365,-0.34416318088334,
394.124704155417));
#39092=CARTESIAN_POINT('Ctrl Pts',(-4.5173836733729,-2.76243915998559E-5,
394.112583302492));
#39093=CARTESIAN_POINT('Ctrl Pts',(-4.51808751818987,5.21912322906659E-5,
394.387416697508));
#39094=CARTESIAN_POINT('Ctrl Pts',(-4.51767853826069,-0.696489376170657,
394.411960704277));
#39095=CARTESIAN_POINT('Ctrl Pts',(-4.35403905930357,-1.39321647594668,
394.436504711046));
#39096=CARTESIAN_POINT('Ctrl Pts',(-4.0431719192238,-2.01651441971212,394.461048717815));
#39097=CARTESIAN_POINT('Ctrl Pts',(-3.70910181980172,-2.68633499318885,
394.487424676302));
#39098=CARTESIAN_POINT('Ctrl Pts',(-3.20500585655341,-3.27135590615661,
394.513800634789));
#39099=CARTESIAN_POINT('Ctrl Pts',(-2.59191322109249,-3.70075065731708,
394.540176593275));
#39100=CARTESIAN_POINT('Ctrl Pts',(-1.97882058563158,-4.13014540847754,
394.566552551762));
#39101=CARTESIAN_POINT('Ctrl Pts',(-1.25673127795806,-4.40391399783071,
394.592928510249));
#39102=CARTESIAN_POINT('Ctrl Pts',(-0.513066205861354,-4.48891218912888,
394.619304468735));
#39103=CARTESIAN_POINT('Ctrl Pts',(0.230598866235364,-4.57391038042705,
394.645680427222));
#39104=CARTESIAN_POINT('Ctrl Pts',(0.995839702755266,-4.47013817367021,
394.672056385708));
#39105=CARTESIAN_POINT('Ctrl Pts',(1.69001118640443,-4.19015891860138,394.698432344195));
#39106=CARTESIAN_POINT('Ctrl Pts',(2.3841826700536,-3.91017966353254,394.724808302681));
#39107=CARTESIAN_POINT('Ctrl Pts',(3.00728480083202,-3.45399336015171,394.751184261168));
#39108=CARTESIAN_POINT('Ctrl Pts',(3.48388071332803,-2.87682893975429,394.777560219655));
#39109=CARTESIAN_POINT('Ctrl Pts',(3.96047662582402,-2.29966451935688,394.803936178141));
#39110=CARTESIAN_POINT('Ctrl Pts',(4.29056632003761,-1.6015219819429,394.830312136628));
#39111=CARTESIAN_POINT('Ctrl Pts',(4.43418695423518,-0.866923080900132,
394.856688095114));
#39112=CARTESIAN_POINT('Ctrl Pts',(4.57780758843275,-0.132324179857343,
394.883064053601));
#39113=CARTESIAN_POINT('Ctrl Pts',(4.5349591626143,0.638731084814249,394.909440012088));
#39114=CARTESIAN_POINT('Ctrl Pts',(4.31082919062693,1.35289366268957,394.935815970574));
#39115=CARTESIAN_POINT('Ctrl Pts',(4.08669921863955,2.06705624056489,394.962191929061));
#39116=CARTESIAN_POINT('Ctrl Pts',(3.68128770048325,2.72432613164396,394.988567887547));
#39117=CARTESIAN_POINT('Ctrl Pts',(3.14367643610836,3.24512989545316,395.014943846034));
#39118=CARTESIAN_POINT('Ctrl Pts',(2.60606517173349,3.76593365926234,395.04131980452));
#39119=CARTESIAN_POINT('Ctrl Pts',(1.93625416114004,4.15027129580166,395.067695763007));
#39120=CARTESIAN_POINT('Ctrl Pts',(1.21533515568228,4.35161234862086,395.094071721494));
#39121=CARTESIAN_POINT('Ctrl Pts',(0.494416150224501,4.55295340144005,395.12044767998));
#39122=CARTESIAN_POINT('Ctrl Pts',(-0.277610850097608,4.57129787053912,
395.146823638467));
#39123=CARTESIAN_POINT('Ctrl Pts',(-1.00727915011366,4.40442485315088,395.173199596953));
#39124=CARTESIAN_POINT('Ctrl Pts',(-1.73694745012971,4.23755183576263,395.19957555544));
#39125=CARTESIAN_POINT('Ctrl Pts',(-2.42425704983972,3.88546133188709,395.225951513927));
#39126=CARTESIAN_POINT('Ctrl Pts',(-2.98599770294795,3.39077974679813,395.252327472413));
#39127=CARTESIAN_POINT('Ctrl Pts',(-3.54773835605617,2.89609816170917,395.2787034309));
#39128=CARTESIAN_POINT('Ctrl Pts',(-3.9839100625626,2.25882549540681,395.305079389386));
#39129=CARTESIAN_POINT('Ctrl Pts',(-4.24170699065442,1.55611419206311,395.331455347873));
#39130=CARTESIAN_POINT('Ctrl Pts',(-4.42402787244154,1.05913796579184,395.350109131085));
#39131=CARTESIAN_POINT('Ctrl Pts',(-4.5171311009058,0.529431318295306,395.368762914296));
#39132=CARTESIAN_POINT('Ctrl Pts',(-4.51761539860092,-0.000109498206778275,
395.387416697508));
#39133=CARTESIAN_POINT('Origin',(0.,0.,387.));
#39134=CARTESIAN_POINT('',(-4.51751463264715,9.2546932777271E-5,396.387416697508));
#39135=CARTESIAN_POINT('',(-4.51786437784292,-0.000108222965875699,396.112583302492));
#39136=CARTESIAN_POINT('',(-4.51775,5.53264807684796E-16,387.));
#39137=CARTESIAN_POINT('Ctrl Pts',(-4.51786437784292,-0.000108222965875699,
396.112583302492));
#39138=CARTESIAN_POINT('Ctrl Pts',(-4.5172490555957,0.610781207776803,396.091060492428));
#39139=CARTESIAN_POINT('Ctrl Pts',(-4.39244234778488,1.22191440722307,396.069537682365));
#39140=CARTESIAN_POINT('Ctrl Pts',(-4.15139232023937,1.78311842878099,396.048014872301));
#39141=CARTESIAN_POINT('Ctrl Pts',(-3.85598825818002,2.47086756243728,396.021638913814));
#39142=CARTESIAN_POINT('Ctrl Pts',(-3.38600738379809,3.0836319422382,395.995262955328));
#39143=CARTESIAN_POINT('Ctrl Pts',(-2.79834869039748,3.54722625928365,395.968886996841));
#39144=CARTESIAN_POINT('Ctrl Pts',(-2.21068999699688,4.0108205763291,395.942511038355));
#39145=CARTESIAN_POINT('Ctrl Pts',(-1.50535348457759,4.32524483061908,395.916135079868));
#39146=CARTESIAN_POINT('Ctrl Pts',(-0.767731856725531,4.45243274219494,
395.889759121381));
#39147=CARTESIAN_POINT('Ctrl Pts',(-0.0301102288734742,4.5796206537708,
395.863383162895));
#39148=CARTESIAN_POINT('Ctrl Pts',(0.739796514411352,4.51957222263255,395.837007204408));
#39149=CARTESIAN_POINT('Ctrl Pts',(1.44877837029978,4.27955730903937,395.810631245922));
#39150=CARTESIAN_POINT('Ctrl Pts',(2.15776022618821,4.03954239544619,395.784255287435));
#39151=CARTESIAN_POINT('Ctrl Pts',(2.80581719468025,3.61956099939807,395.757879328948));
#39152=CARTESIAN_POINT('Ctrl Pts',(3.31449121264882,3.07045884663426,395.731503370462));
#39153=CARTESIAN_POINT('Ctrl Pts',(3.82316523061738,2.52135669387044,395.705127411975));
#39154=CARTESIAN_POINT('Ctrl Pts',(4.19245629806247,1.84313378439093,395.678751453489));
#39155=CARTESIAN_POINT('Ctrl Pts',(4.37765559571272,1.11790026966896,395.652375495002));
#39156=CARTESIAN_POINT('Ctrl Pts',(4.56285489336297,0.392666754946975,395.625999536516));
#39157=CARTESIAN_POINT('Ctrl Pts',(4.56396242121836,-0.379577365017472,
395.599623578029));
#39158=CARTESIAN_POINT('Ctrl Pts',(4.38084409463107,-1.10533910911399,395.573247619542));
#39159=CARTESIAN_POINT('Ctrl Pts',(4.19772576804378,-1.8311008532105,395.546871661056));
#39160=CARTESIAN_POINT('Ctrl Pts',(3.8303815870138,-2.51038022143909,395.520495702569));
#39161=CARTESIAN_POINT('Ctrl Pts',(3.32328466786559,-3.06093916044248,395.494119744083));
#39162=CARTESIAN_POINT('Ctrl Pts',(2.81618774871737,-3.61149809944587,395.467743785596));
#39163=CARTESIAN_POINT('Ctrl Pts',(2.16933809145092,-4.03333660922406,395.441367827109));
#39164=CARTESIAN_POINT('Ctrl Pts',(1.46104759411067,-4.27538412956593,395.414991868623));
#39165=CARTESIAN_POINT('Ctrl Pts',(0.75275709677042,-4.5174316499078,395.388615910136));
#39166=CARTESIAN_POINT('Ctrl Pts',(-0.0169742406436262,-4.57968818081335,
395.36223995165));
#39167=CARTESIAN_POINT('Ctrl Pts',(-0.754957651097232,-4.45461653486027,
395.335863993163));
#39168=CARTESIAN_POINT('Ctrl Pts',(-1.49294106155083,-4.3295448889072,395.309488034676));
#39169=CARTESIAN_POINT('Ctrl Pts',(-2.19917654504398,-4.01714506609549,
395.28311207619));
#39170=CARTESIAN_POINT('Ctrl Pts',(-2.78816256260641,-3.5552382553186,395.256736117703));
#39171=CARTESIAN_POINT('Ctrl Pts',(-3.37714858016886,-3.0933314445417,395.230360159217));
#39172=CARTESIAN_POINT('Ctrl Pts',(-3.84888513180058,-2.4819176457996,395.20398420073));
#39173=CARTESIAN_POINT('Ctrl Pts',(-4.14626067029702,-1.79501865771611,
395.177608242243));
#39174=CARTESIAN_POINT('Ctrl Pts',(-4.39063506253172,-1.23054545461321,
395.155933262326));
#39175=CARTESIAN_POINT('Ctrl Pts',(-4.51726233565243,-0.615096615266284,
395.134258282409));
#39176=CARTESIAN_POINT('Ctrl Pts',(-4.51787769339044,0.000106674156513836,
395.112583302492));
#39177=CARTESIAN_POINT('Ctrl Pts',(-4.51761539860092,-0.000109498206778275,
395.387416697508));
#39178=CARTESIAN_POINT('Ctrl Pts',(-4.51781588509979,-0.219325458522322,
395.395138872783));
#39179=CARTESIAN_POINT('Ctrl Pts',(-4.5021438757463,-0.438512999682626,
395.402861048058));
#39180=CARTESIAN_POINT('Ctrl Pts',(-4.47035806891458,-0.655338316442091,
395.410583223333));
#39181=CARTESIAN_POINT('Ctrl Pts',(-4.36179006940572,-1.39592958121857,
395.436959181819));
#39182=CARTESIAN_POINT('Ctrl Pts',(-4.06523192071081,-2.10896217038649,
395.463335140306));
#39183=CARTESIAN_POINT('Ctrl Pts',(-3.61658691387121,-2.70811164240368,
395.489711098793));
#39184=CARTESIAN_POINT('Ctrl Pts',(-3.16794190703161,-3.30726111442086,
395.516087057279));
#39185=CARTESIAN_POINT('Ctrl Pts',(-2.56721004204732,-3.79252746928731,
395.542463015766));
#39186=CARTESIAN_POINT('Ctrl Pts',(-1.88711989198663,-4.10516115232706,
395.568838974252));
#39187=CARTESIAN_POINT('Ctrl Pts',(-1.20702974192593,-4.4177948353668,395.595214932739));
#39188=CARTESIAN_POINT('Ctrl Pts',(-0.447581306788832,-4.55779584657986,
395.621590891225));
#39189=CARTESIAN_POINT('Ctrl Pts',(0.299281562555524,-4.50821473752317,
395.647966849712));
#39190=CARTESIAN_POINT('Ctrl Pts',(1.04614443189988,-4.45863362846649,395.674342808199));
#39191=CARTESIAN_POINT('Ctrl Pts',(1.78042173545149,-4.21947039914007,395.700718766685));
#39192=CARTESIAN_POINT('Ctrl Pts',(2.4132170060234,-3.81967973201239,395.727094725172));
#39193=CARTESIAN_POINT('Ctrl Pts',(3.04601227659532,-3.41988906488471,395.753470683659));
#39194=CARTESIAN_POINT('Ctrl Pts',(3.57732551418753,-2.85947095995576,395.779846642145));
#39195=CARTESIAN_POINT('Ctrl Pts',(3.94283242392784,-2.20627333984937,395.806222600631));
#39196=CARTESIAN_POINT('Ctrl Pts',(4.30833933366816,-1.55307571974297,395.832598559118));
#39197=CARTESIAN_POINT('Ctrl Pts',(4.50803991555659,-0.807098584459129,
395.858974517605));
#39198=CARTESIAN_POINT('Ctrl Pts',(4.51775709624605,-0.0586548602019053,
395.885350476092));
#39199=CARTESIAN_POINT('Ctrl Pts',(4.5274742769355,0.689788864055318,395.911726434578));
#39200=CARTESIAN_POINT('Ctrl Pts',(4.34720805642599,1.44069917728592,395.938102393065));
#39201=CARTESIAN_POINT('Ctrl Pts',(3.99878265572902,2.10316591013349,395.964478351551));
#39202=CARTESIAN_POINT('Ctrl Pts',(3.65035725503204,2.76563264298105,395.990854310038));
#39203=CARTESIAN_POINT('Ctrl Pts',(3.13377267414759,3.33965579544558,396.017230268524));
#39204=CARTESIAN_POINT('Ctrl Pts',(2.5115700593453,3.75574032785908,396.043606227011));
#39205=CARTESIAN_POINT('Ctrl Pts',(1.88936744454301,4.17182486027259,396.069982185498));
#39206=CARTESIAN_POINT('Ctrl Pts',(1.16154679582287,4.42997077263507,396.096358143984));
#39207=CARTESIAN_POINT('Ctrl Pts',(0.416222895030907,4.49892521331027,396.122734102471));
#39208=CARTESIAN_POINT('Ctrl Pts',(-0.329101005761055,4.56787965398547,
396.149110060957));
#39209=CARTESIAN_POINT('Ctrl Pts',(-1.09192815862484,4.44764262297338,396.175486019444));
#39210=CARTESIAN_POINT('Ctrl Pts',(-1.77990566277504,4.15277081054664,396.201861977931));
#39211=CARTESIAN_POINT('Ctrl Pts',(-2.46788316692524,3.85789899811989,396.228237936417));
#39212=CARTESIAN_POINT('Ctrl Pts',(-3.08101102236186,3.38839240427848,396.254613894904));
#39213=CARTESIAN_POINT('Ctrl Pts',(-3.54505991542016,2.80109260278699,396.28098985339));
#39214=CARTESIAN_POINT('Ctrl Pts',(-4.00910880847846,2.2137928012955,396.307365811877));
#39215=CARTESIAN_POINT('Ctrl Pts',(-4.32407873915844,1.50869979215393,396.333741770364));
#39216=CARTESIAN_POINT('Ctrl Pts',(-4.45183736430835,0.771176798830757,
396.36011772885));
#39217=CARTESIAN_POINT('Ctrl Pts',(-4.4959138504198,0.516732749092945,396.369217385069));
#39218=CARTESIAN_POINT('Ctrl Pts',(-4.51770775311255,0.258428762447222,
396.378317041289));
#39219=CARTESIAN_POINT('Ctrl Pts',(-4.51751463264715,9.2546932777271E-5,
396.387416697508));
#39220=CARTESIAN_POINT('Origin',(0.,0.,387.));
#39221=CARTESIAN_POINT('',(-4.51813440218219,-1.34914224690988E-5,397.387416697508));
#39222=CARTESIAN_POINT('',(-4.51738673749921,3.14726202902737E-5,397.112583302492));
#39223=CARTESIAN_POINT('',(-4.51775,5.53264807684796E-16,387.));
#39224=CARTESIAN_POINT('Ctrl Pts',(-4.51738673749921,3.14726202902737E-5,
397.112583302492));
#39225=CARTESIAN_POINT('Ctrl Pts',(-4.51746996308395,0.339845959287686,
397.100614619421));
#39226=CARTESIAN_POINT('Ctrl Pts',(-4.47962267703118,0.67964219695818,397.088645936349));
#39227=CARTESIAN_POINT('Ctrl Pts',(-4.40364412455734,1.01068687131693,397.076677253278));
#39228=CARTESIAN_POINT('Ctrl Pts',(-4.236206559874,1.7402258302897,397.050301294792));
#39229=CARTESIAN_POINT('Ctrl Pts',(-3.88358434036526,2.42726278544303,397.023925336305));
#39230=CARTESIAN_POINT('Ctrl Pts',(-3.38846824431658,2.9886204986346,396.997549377818));
#39231=CARTESIAN_POINT('Ctrl Pts',(-2.89335214826789,3.54997821182617,396.971173419332));
#39232=CARTESIAN_POINT('Ctrl Pts',(-2.25574217567927,3.98565668305597,396.944797460845));
#39233=CARTESIAN_POINT('Ctrl Pts',(-1.55283160725287,4.24290979483623,396.918421502359));
#39234=CARTESIAN_POINT('Ctrl Pts',(-0.849921038826476,4.5001629066165,396.892045543872));
#39235=CARTESIAN_POINT('Ctrl Pts',(-0.0817098745623172,4.57899065894722,
396.865669585385));
#39236=CARTESIAN_POINT('Ctrl Pts',(0.658797160721962,4.46984964273134,396.839293626899));
#39237=CARTESIAN_POINT('Ctrl Pts',(1.39930419600623,4.36070862651545,396.812917668412));
#39238=CARTESIAN_POINT('Ctrl Pts',(2.11210710231061,4.06359884175296,396.786541709925));
#39239=CARTESIAN_POINT('Ctrl Pts',(2.71090924501961,3.61449036419631,396.760165751439));
#39240=CARTESIAN_POINT('Ctrl Pts',(3.30971138772862,3.16538188663966,396.733789792952));
#39241=CARTESIAN_POINT('Ctrl Pts',(3.79451276684224,2.56427471628884,396.707413834466));
#39242=CARTESIAN_POINT('Ctrl Pts',(4.10662012072468,1.88394286316225,396.681037875979));
#39243=CARTESIAN_POINT('Ctrl Pts',(4.41872747460713,1.20361101003566,396.654661917493));
#39244=CARTESIAN_POINT('Ctrl Pts',(4.5581408032584,0.444054474133294,396.628285959006));
#39245=CARTESIAN_POINT('Ctrl Pts',(4.50798180697358,-0.302769806282027,
396.601910000519));
#39246=CARTESIAN_POINT('Ctrl Pts',(4.45782281068875,-1.04959408669733,396.575534042033));
#39247=CARTESIAN_POINT('Ctrl Pts',(4.21809148946783,-1.78368611162558,396.549158083546));
#39248=CARTESIAN_POINT('Ctrl Pts',(3.81781130274164,-2.41617184493549,396.52278212506));
#39249=CARTESIAN_POINT('Ctrl Pts',(3.41753111601545,-3.0486575782454,396.496406166573));
#39250=CARTESIAN_POINT('Ctrl Pts',(2.85670206378398,-3.57953701993697,396.470030208087));
#39251=CARTESIAN_POINT('Ctrl Pts',(2.20322182066968,-3.94453839333905,396.4436542496));
#39252=CARTESIAN_POINT('Ctrl Pts',(1.54974157755536,-4.30953976674113,396.417278291113));
#39253=CARTESIAN_POINT('Ctrl Pts',(0.803610143558188,-4.50866307185371,
396.390902332627));
#39254=CARTESIAN_POINT('Ctrl Pts',(0.0551591253050773,-4.51780112427455,
396.36452637414));
#39255=CARTESIAN_POINT('Ctrl Pts',(-0.693291892948023,-4.52693917669538,
396.338150415653));
#39256=CARTESIAN_POINT('Ctrl Pts',(-1.44406249545706,-4.34609197642448,
396.311774457167));
#39257=CARTESIAN_POINT('Ctrl Pts',(-2.10625942716968,-3.9971540817261,396.28539849868));
#39258=CARTESIAN_POINT('Ctrl Pts',(-2.7684563588823,-3.64821618702772,396.259022540194));
#39259=CARTESIAN_POINT('Ctrl Pts',(-3.3420796197985,-3.13118759790186,396.232646581707));
#39260=CARTESIAN_POINT('Ctrl Pts',(-3.7576825837662,-2.5086632151927,396.206270623221));
#39261=CARTESIAN_POINT('Ctrl Pts',(-4.17328554773389,-1.88613883248355,
396.179894664734));
#39262=CARTESIAN_POINT('Ctrl Pts',(-4.43086821475307,-1.15811865619109,
396.153518706247));
#39263=CARTESIAN_POINT('Ctrl Pts',(-4.49924592339428,-0.412741624289035,
396.127142747761));
#39264=CARTESIAN_POINT('Ctrl Pts',(-4.51182734935556,-0.275593039955457,
396.122289599338));
#39265=CARTESIAN_POINT('Ctrl Pts',(-4.51800312599824,-0.137856828684076,
396.117436450915));
#39266=CARTESIAN_POINT('Ctrl Pts',(-4.51786437784292,-0.000108222965875699,
396.112583302492));
#39267=CARTESIAN_POINT('Ctrl Pts',(-4.51751463264715,9.2546932777271E-5,
396.387416697508));
#39268=CARTESIAN_POINT('Ctrl Pts',(-4.51714798060515,-0.490375932126388,
396.404692999775));
#39269=CARTESIAN_POINT('Ctrl Pts',(-4.43752790145426,-0.98096058190497,
396.421969302042));
#39270=CARTESIAN_POINT('Ctrl Pts',(-4.28067705789975,-1.44546653343395,
396.43924560431));
#39271=CARTESIAN_POINT('Ctrl Pts',(-4.04121080672139,-2.1546338948707,396.465621562796));
#39272=CARTESIAN_POINT('Ctrl Pts',(-3.62173098474482,-2.80301564023941,
396.491997521283));
#39273=CARTESIAN_POINT('Ctrl Pts',(-3.07302259383454,-3.3121143867761,396.51837347977));
#39274=CARTESIAN_POINT('Ctrl Pts',(-2.52431420292427,-3.8212131333128,396.544749438256));
#39275=CARTESIAN_POINT('Ctrl Pts',(-1.84637724308029,-4.19102888101748,
396.571125396743));
#39276=CARTESIAN_POINT('Ctrl Pts',(-1.12128724682158,-4.37678928935608,
396.597501355229));
#39277=CARTESIAN_POINT('Ctrl Pts',(-0.396197250562878,-4.56254969769468,
396.623877313716));
#39278=CARTESIAN_POINT('Ctrl Pts',(0.376045782110559,-4.5642547666672,396.650253272203));
#39279=CARTESIAN_POINT('Ctrl Pts',(1.10194900172297,-4.38169806934578,396.676629230689));
#39280=CARTESIAN_POINT('Ctrl Pts',(1.82785222133539,-4.19914137202436,396.703005189176));
#39281=CARTESIAN_POINT('Ctrl Pts',(2.50741562788679,-3.83232290840901,396.729381147662));
#39282=CARTESIAN_POINT('Ctrl Pts',(3.05836678046179,-3.32565214799663,396.755757106149));
#39283=CARTESIAN_POINT('Ctrl Pts',(3.60931793303678,-2.81898138758426,396.782133064635));
#39284=CARTESIAN_POINT('Ctrl Pts',(4.03165683163537,-2.17245833037488,396.808509023122));
#39285=CARTESIAN_POINT('Ctrl Pts',(4.27425233566608,-1.46435533404973,396.834884981609));
#39286=CARTESIAN_POINT('Ctrl Pts',(4.51684783969678,-0.756252337724576,
396.861260940095));
#39287=CARTESIAN_POINT('Ctrl Pts',(4.57969994915959,0.0134305977163408,
396.887636898582));
#39288=CARTESIAN_POINT('Ctrl Pts',(4.45519937195264,0.751510565101793,396.914012857069));
#39289=CARTESIAN_POINT('Ctrl Pts',(4.33069879474569,1.48959053248724,396.940388815555));
#39290=CARTESIAN_POINT('Ctrl Pts',(4.01884553086897,2.19606753181724,396.966764774042));
#39291=CARTESIAN_POINT('Ctrl Pts',(3.5573945991761,2.78541078461679,396.993140732528));
#39292=CARTESIAN_POINT('Ctrl Pts',(3.09594366748323,3.37475403741634,397.019516691015));
#39293=CARTESIAN_POINT('Ctrl Pts',(2.4848950679742,3.84696354368545,397.045892649502));
#39294=CARTESIAN_POINT('Ctrl Pts',(1.79822638583807,4.14487049720285,397.072268607988));
#39295=CARTESIAN_POINT('Ctrl Pts',(1.11155770370195,4.44277745072024,397.098644566475));
#39296=CARTESIAN_POINT('Ctrl Pts',(0.349268938938723,4.56638185148592,397.125020524961));
#39297=CARTESIAN_POINT('Ctrl Pts',(-0.396352188490757,4.50071933317169,
397.151396483448));
#39298=CARTESIAN_POINT('Ctrl Pts',(-1.14197331592023,4.43505681485745,397.177772441934));
#39299=CARTESIAN_POINT('Ctrl Pts',(-1.87092680601596,4.18012737746331,397.204148400421));
#39300=CARTESIAN_POINT('Ctrl Pts',(-2.49496072766192,3.76679446489074,397.230524358908));
#39301=CARTESIAN_POINT('Ctrl Pts',(-3.1189946493079,3.35346155231816,397.256900317394));
#39302=CARTESIAN_POINT('Ctrl Pts',(-3.63810900250409,2.78172516456714,397.283276275881));
#39303=CARTESIAN_POINT('Ctrl Pts',(-3.98945637001185,2.12080349044383,397.309652234368));
#39304=CARTESIAN_POINT('Ctrl Pts',(-4.33474984909618,1.47126982272609,397.335573722081));
#39305=CARTESIAN_POINT('Ctrl Pts',(-4.51800794997827,0.735597803364803,
397.361495209794));
#39306=CARTESIAN_POINT('Ctrl Pts',(-4.51813440218219,-1.34914224690988E-5,
397.387416697508));
#39307=CARTESIAN_POINT('Origin',(0.,0.,387.));
#39308=CARTESIAN_POINT('',(-4.51746064445937,-7.62825515632226E-5,398.387416697508));
#39309=CARTESIAN_POINT('',(-4.51805439081064,6.66898104614677E-5,398.112583302492));
#39310=CARTESIAN_POINT('',(-4.51775,5.53264807684796E-16,387.));
#39311=CARTESIAN_POINT('Ctrl Pts',(-4.51805439081064,6.66898104614677E-5,
398.112583302492));
#39312=CARTESIAN_POINT('Ctrl Pts',(-4.51810357212516,0.0685915430668216,
398.110168746413));
#39313=CARTESIAN_POINT('Ctrl Pts',(-4.51657662108523,0.137114203419027,
398.107754190334));
#39314=CARTESIAN_POINT('Ctrl Pts',(-4.51345907222813,0.205564420371811,
398.105339634255));
#39315=CARTESIAN_POINT('Ctrl Pts',(-4.47940381049539,0.953296103447074,
398.078963675769));
#39316=CARTESIAN_POINT('Ctrl Pts',(-4.255545890619,1.6923832695825,398.052587717282));
#39317=CARTESIAN_POINT('Ctrl Pts',(-3.86898703306984,2.33334713781254,398.026211758796));
#39318=CARTESIAN_POINT('Ctrl Pts',(-3.48242817552068,2.97431100604258,397.999835800309));
#39319=CARTESIAN_POINT('Ctrl Pts',(-2.93316838029875,3.51715157636723,397.973459841822));
#39320=CARTESIAN_POINT('Ctrl Pts',(-2.28770467124889,3.89614897876697,397.947083883336));
#39321=CARTESIAN_POINT('Ctrl Pts',(-1.64224096219904,4.27514638116671,397.920707924849));
#39322=CARTESIAN_POINT('Ctrl Pts',(-0.900573339321256,4.49030061564153,
397.894331966363));
#39323=CARTESIAN_POINT('Ctrl Pts',(-0.15249299074285,4.51556368744535,397.867956007876));
#39324=CARTESIAN_POINT('Ctrl Pts',(0.595587357835559,4.54082675924917,397.841580049389));
#39325=CARTESIAN_POINT('Ctrl Pts',(1.35008043211458,4.37619866838198,397.815204090903));
#39326=CARTESIAN_POINT('Ctrl Pts',(2.01964230998743,4.0416103804436,397.788828132416));
#39327=CARTESIAN_POINT('Ctrl Pts',(2.68920418786027,3.70702209250522,397.76245217393));
#39328=CARTESIAN_POINT('Ctrl Pts',(3.27383486932692,3.20247360749564,397.736076215443));
#39329=CARTESIAN_POINT('Ctrl Pts',(3.70275509709574,2.58904890230608,397.709700256956));
#39330=CARTESIAN_POINT('Ctrl Pts',(4.13167532486456,1.97562419711653,397.68332429847));
#39331=CARTESIAN_POINT('Ctrl Pts',(4.40488509893554,1.25332327174699,397.656948339983));
#39332=CARTESIAN_POINT('Ctrl Pts',(4.48930783693528,0.509592653824902,397.630572381497));
#39333=CARTESIAN_POINT('Ctrl Pts',(4.57373057493501,-0.234137964097188,
397.60419642301));
#39334=CARTESIAN_POINT('Ctrl Pts',(4.4693662768635,-0.999298274571833,397.577820464523));
#39335=CARTESIAN_POINT('Ctrl Pts',(4.18884997495465,-1.69325290932077,397.551444506037));
#39336=CARTESIAN_POINT('Ctrl Pts',(3.9083336730458,-2.3872075440697,397.52506854755));
#39337=CARTESIAN_POINT('Ctrl Pts',(3.4516653672996,-3.00995650309293,397.498692589064));
#39338=CARTESIAN_POINT('Ctrl Pts',(2.87413234340601,-3.48610567828749,397.472316630577));
#39339=CARTESIAN_POINT('Ctrl Pts',(2.29659931951241,-3.96225485348206,397.44594067209));
#39340=CARTESIAN_POINT('Ctrl Pts',(1.5982015774714,-4.29180424484795,397.419564713604));
#39341=CARTESIAN_POINT('Ctrl Pts',(0.863491767430947,-4.43485642328811,
397.393188755117));
#39342=CARTESIAN_POINT('Ctrl Pts',(0.128781957390508,-4.57790860172826,
397.366812796631));
#39343=CARTESIAN_POINT('Ctrl Pts',(-0.642239920649369,-4.53446356724268,
397.340436838144));
#39344=CARTESIAN_POINT('Ctrl Pts',(-1.35622885827011,-4.30978106306993,
397.314060879658));
#39345=CARTESIAN_POINT('Ctrl Pts',(-2.07021779589086,-4.08509855889717,
397.287684921171));
#39346=CARTESIAN_POINT('Ctrl Pts',(-2.72717379309247,-3.67917858503723,
397.261308962684));
#39347=CARTESIAN_POINT('Ctrl Pts',(-3.24756141147036,-3.14116449845108,
397.234933004198));
#39348=CARTESIAN_POINT('Ctrl Pts',(-3.76794902984825,-2.60315041186493,
397.208557045711));
#39349=CARTESIAN_POINT('Ctrl Pts',(-4.15176826940243,-1.93304221255256,
397.182181087224));
#39350=CARTESIAN_POINT('Ctrl Pts',(-4.35255143425054,-1.21196763150028,
397.155805128738));
#39351=CARTESIAN_POINT('Ctrl Pts',(-4.46222473223498,-0.818096823374597,
397.141397853322));
#39352=CARTESIAN_POINT('Ctrl Pts',(-4.51728655488816,-0.409019453899831,
397.126990577907));
#39353=CARTESIAN_POINT('Ctrl Pts',(-4.51738673749921,3.14726202902737E-5,
397.112583302492));
#39354=CARTESIAN_POINT('Ctrl Pts',(-4.51813440218219,-1.34914224690988E-5,
397.387416697508));
#39355=CARTESIAN_POINT('Ctrl Pts',(-4.51813661921663,-0.0129106614282636,
397.387871168281));
#39356=CARTESIAN_POINT('Ctrl Pts',(-4.51808254311073,-0.0258078127678308,
397.388325639054));
#39357=CARTESIAN_POINT('Ctrl Pts',(-4.51797206016886,-0.0387044808823415,
397.388780109827));
#39358=CARTESIAN_POINT('Ctrl Pts',(-4.51156000099881,-0.787183817589628,
397.415156068314));
#39359=CARTESIAN_POINT('Ctrl Pts',(-4.31515550083941,-1.5340355305086,397.4415320268));
#39360=CARTESIAN_POINT('Ctrl Pts',(-3.95253658758193,-2.18884081128186,
397.467907985287));
#39361=CARTESIAN_POINT('Ctrl Pts',(-3.58991767432445,-2.84364609205511,
397.494283943774));
#39362=CARTESIAN_POINT('Ctrl Pts',(-3.06108434796891,-3.40640494068263,
397.52065990226));
#39363=CARTESIAN_POINT('Ctrl Pts',(-2.43006066892999,-3.80898604862584,
397.547035860747));
#39364=CARTESIAN_POINT('Ctrl Pts',(-1.79903698989108,-4.21156715656904,
397.573411819233));
#39365=CARTESIAN_POINT('Ctrl Pts',(-1.0658229581688,-4.45397052382792,397.59978777772));
#39366=CARTESIAN_POINT('Ctrl Pts',(-0.319186314229528,-4.5068491954042,
397.626163736207));
#39367=CARTESIAN_POINT('Ctrl Pts',(0.427450329709741,-4.55972786698048,
397.652539694693));
#39368=CARTESIAN_POINT('Ctrl Pts',(1.18750958586602,-4.42308184287416,397.67891565318));
#39369=CARTESIAN_POINT('Ctrl Pts',(1.86897365333732,-4.11345439459799,397.705291611666));
#39370=CARTESIAN_POINT('Ctrl Pts',(2.55043772080863,-3.80382694632181,397.731667570153));
#39371=CARTESIAN_POINT('Ctrl Pts',(3.15330659959498,-3.32121807387579,397.75804352864));
#39372=CARTESIAN_POINT('Ctrl Pts',(3.60459299560209,-2.72405559953603,397.784419487126));
#39373=CARTESIAN_POINT('Ctrl Pts',(4.0558793916092,-2.12689312519627,397.810795445613));
#39374=CARTESIAN_POINT('Ctrl Pts',(4.35558330483707,-1.41517704896277,397.837171404099));
#39375=CARTESIAN_POINT('Ctrl Pts',(4.46742059718259,-0.675072426614591,
397.863547362586));
#39376=CARTESIAN_POINT('Ctrl Pts',(4.57925788952811,0.065032195733587,397.889923321072));
#39377=CARTESIAN_POINT('Ctrl Pts',(4.50322856099129,0.833525364196443,397.916299279559));
#39378=CARTESIAN_POINT('Ctrl Pts',(4.24853722497469,1.53736821266419,397.942675238046));
#39379=CARTESIAN_POINT('Ctrl Pts',(3.9938458889581,2.24121106113193,397.969051196532));
#39380=CARTESIAN_POINT('Ctrl Pts',(3.56049254546173,2.88040358960456,397.995427155019));
#39381=CARTESIAN_POINT('Ctrl Pts',(3.00094181663071,3.37756092269383,398.021803113505));
#39382=CARTESIAN_POINT('Ctrl Pts',(2.44139108779969,3.87471825578309,398.048179071992));
#39383=CARTESIAN_POINT('Ctrl Pts',(1.75564297363402,4.22984039348899,398.074555030479));
#39384=CARTESIAN_POINT('Ctrl Pts',(1.02671867666087,4.39993390090012,398.100930988965));
#39385=CARTESIAN_POINT('Ctrl Pts',(0.297794379687701,4.57002740831124,398.127306947452));
#39386=CARTESIAN_POINT('Ctrl Pts',(-0.474306100092957,4.55509228542758,
398.153682905938));
#39387=CARTESIAN_POINT('Ctrl Pts',(-1.19610717160092,4.35693667699891,398.180058864425));
#39388=CARTESIAN_POINT('Ctrl Pts',(-1.91790824310887,4.15878106857024,398.206434822912));
#39389=CARTESIAN_POINT('Ctrl Pts',(-2.58940990634414,3.77740497459655,398.232810781398));
#39390=CARTESIAN_POINT('Ctrl Pts',(-3.12931572836207,3.25898030762527,398.259186739885));
#39391=CARTESIAN_POINT('Ctrl Pts',(-3.66922155038001,2.74055564065398,398.285562698372));
#39392=CARTESIAN_POINT('Ctrl Pts',(-4.07753153118063,2.08508240068509,398.311938656858));
#39393=CARTESIAN_POINT('Ctrl Pts',(-4.30481296375181,1.37191651366358,398.338314615345));
#39394=CARTESIAN_POINT('Ctrl Pts',(-4.44585038591782,0.929367920299095,
398.354681976066));
#39395=CARTESIAN_POINT('Ctrl Pts',(-4.51717896496231,0.464603561951737,
398.371049336787));
#39396=CARTESIAN_POINT('Ctrl Pts',(-4.51746064445937,-7.62825515632226E-5,
398.387416697508));
#39397=CARTESIAN_POINT('Origin',(0.,0.,387.));
#39398=CARTESIAN_POINT('',(-4.51769110620511,0.00011483889287206,399.387416697508));
#39399=CARTESIAN_POINT('',(-4.51766328535307,-0.00011344722995056,399.112583302492));
#39400=CARTESIAN_POINT('',(-4.51775,5.53264807684796E-16,387.));
#39401=CARTESIAN_POINT('',(3.43378788736219,2.93584158412962,400.));
#39402=CARTESIAN_POINT('Ctrl Pts',(-4.51769110620511,0.00011483889287206,
399.387416697508));
#39403=CARTESIAN_POINT('Ctrl Pts',(-4.51714363756808,-0.555201766580607,
399.406979422266));
#39404=CARTESIAN_POINT('Ctrl Pts',(-4.41453063358526,-1.11071503909854,
399.426542147024));
#39405=CARTESIAN_POINT('Ctrl Pts',(-4.21442463507641,-1.62855553809715,
399.446104871782));
#39406=CARTESIAN_POINT('Ctrl Pts',(-3.94462645640127,-2.32674761887018,
399.472480830268));
#39407=CARTESIAN_POINT('Ctrl Pts',(-3.49760073249453,-2.95645628495937,
399.498856788754));
#39408=CARTESIAN_POINT('Ctrl Pts',(-2.92746753734289,-3.44144015063649,
399.525232747241));
#39409=CARTESIAN_POINT('Ctrl Pts',(-2.35733434219124,-3.92642401631361,
399.551608705728));
#39410=CARTESIAN_POINT('Ctrl Pts',(-1.66409367579469,-4.26668308157866,
399.577984664215));
#39411=CARTESIAN_POINT('Ctrl Pts',(-0.931673462414912,-4.42103326728196,
399.604360622701));
#39412=CARTESIAN_POINT('Ctrl Pts',(-0.199253249035141,-4.57538345298525,
399.630736581188));
#39413=CARTESIAN_POINT('Ctrl Pts',(0.572346511327848,-4.5438247591268,399.657112539674));
#39414=CARTESIAN_POINT('Ctrl Pts',(1.28970997251907,-4.33015694611576,399.683488498161));
#39415=CARTESIAN_POINT('Ctrl Pts',(2.00707343371029,-4.11648913310473,399.709864456647));
#39416=CARTESIAN_POINT('Ctrl Pts',(2.67020059572975,-3.72071220094113,399.736240415134));
#39417=CARTESIAN_POINT('Ctrl Pts',(3.19881015567137,-3.19078644074148,399.762616373621));
#39418=CARTESIAN_POINT('Ctrl Pts',(3.72741971561299,-2.66086068054184,399.788992332107));
#39419=CARTESIAN_POINT('Ctrl Pts',(4.12151167347679,-1.99678609230616,399.815368290594));
#39420=CARTESIAN_POINT('Ctrl Pts',(4.33336809368492,-1.27886829832022,399.84174424908));
#39421=CARTESIAN_POINT('Ctrl Pts',(4.54522451389304,-0.560950504334284,
399.868120207567));
#39422=CARTESIAN_POINT('Ctrl Pts',(4.57484539644551,0.210810495401909,399.894496166054));
#39423=CARTESIAN_POINT('Ctrl Pts',(4.41862185200597,0.942742363213577,399.92087212454));
#39424=CARTESIAN_POINT('Ctrl Pts',(4.26239830756643,1.67467423102524,399.947248083027));
#39425=CARTESIAN_POINT('Ctrl Pts',(3.92033033613488,2.36677696691239,399.973624041513));
#39426=CARTESIAN_POINT('Ctrl Pts',(3.43378788736214,2.93584158412968,400.));
#39427=CARTESIAN_POINT('',(-3.43408816619742,2.93604416807593,400.));
#39428=CARTESIAN_POINT('Origin',(0.,0.,400.));
#39429=CARTESIAN_POINT('Ctrl Pts',(-3.43408816619742,2.93604416807593,400.));
#39430=CARTESIAN_POINT('Ctrl Pts',(-2.97450238708434,3.47304931101404,399.975093589943));
#39431=CARTESIAN_POINT('Ctrl Pts',(-2.38685943846713,3.90077490879642,399.950187179887));
#39432=CARTESIAN_POINT('Ctrl Pts',(-1.73419289785415,4.17206489997238,399.92528076983));
#39433=CARTESIAN_POINT('Ctrl Pts',(-1.04301719081029,4.45936176567177,399.898904811344));
#39434=CARTESIAN_POINT('Ctrl Pts',(-0.278918372417421,4.57121813647734,
399.872528852857));
#39435=CARTESIAN_POINT('Ctrl Pts',(0.465602633104777,4.49408395991645,399.84615289437));
#39436=CARTESIAN_POINT('Ctrl Pts',(1.21012363862699,4.41694978335555,399.819776935884));
#39437=CARTESIAN_POINT('Ctrl Pts',(1.93506683127852,4.15082505942817,399.793400977397));
#39438=CARTESIAN_POINT('Ctrl Pts',(2.55266298782158,3.72793237180886,399.767025018911));
#39439=CARTESIAN_POINT('Ctrl Pts',(3.17025914436463,3.30503968418955,399.740649060424));
#39440=CARTESIAN_POINT('Ctrl Pts',(3.68050826479921,2.72537903287831,399.714273101937));
#39441=CARTESIAN_POINT('Ctrl Pts',(4.02163754117277,2.05912619043133,399.687897143451));
#39442=CARTESIAN_POINT('Ctrl Pts',(4.36276681754633,1.39287334798434,399.661521184964));
#39443=CARTESIAN_POINT('Ctrl Pts',(4.53477624985888,0.640028314401621,399.635145226478));
#39444=CARTESIAN_POINT('Ctrl Pts',(4.51684061200005,-0.108263669819661,
399.608769267991));
#39445=CARTESIAN_POINT('Ctrl Pts',(4.49890497414122,-0.856555654040941,
399.582393309504));
#39446=CARTESIAN_POINT('Ctrl Pts',(4.29102426611101,-1.60029458890078,399.556017351018));
#39447=CARTESIAN_POINT('Ctrl Pts',(3.91836619751067,-2.24943891706491,399.529641392531));
#39448=CARTESIAN_POINT('Ctrl Pts',(3.54570812891033,-2.89858324522903,399.503265434045));
#39449=CARTESIAN_POINT('Ctrl Pts',(3.00827269973986,-3.45313296669745,399.476889475558));
#39450=CARTESIAN_POINT('Ctrl Pts',(2.37112525795217,-3.84595043629749,399.450513517072));
#39451=CARTESIAN_POINT('Ctrl Pts',(1.73397781616448,-4.23876790589754,399.424137558585));
#39452=CARTESIAN_POINT('Ctrl Pts',(0.99711836175957,-4.4698531236292,399.397761600098));
#39453=CARTESIAN_POINT('Ctrl Pts',(0.249756040315393,-4.51122947332523,
399.371385641612));
#39454=CARTESIAN_POINT('Ctrl Pts',(-0.497606281128785,-4.55260582302126,
399.345009683125));
#39455=CARTESIAN_POINT('Ctrl Pts',(-1.25547146961223,-4.40427330468165,
399.318633724638));
#39456=CARTESIAN_POINT('Ctrl Pts',(-1.93208738383067,-4.08418999214993,
399.292257766152));
#39457=CARTESIAN_POINT('Ctrl Pts',(-2.60870329804912,-3.7641066796182,399.265881807665));
#39458=CARTESIAN_POINT('Ctrl Pts',(-3.20406993800257,-3.27227257289437,
399.239505849179));
#39459=CARTESIAN_POINT('Ctrl Pts',(-3.64610826548277,-2.6682323819666,399.213129890692));
#39460=CARTESIAN_POINT('Ctrl Pts',(-4.08814659296297,-2.06419219103883,
399.186753932205));
#39461=CARTESIAN_POINT('Ctrl Pts',(-4.37685660796992,-1.34794591590712,
399.160377973719));
#39462=CARTESIAN_POINT('Ctrl Pts',(-4.47728517341772,-0.606207058821207,
399.134002015232));
#39463=CARTESIAN_POINT('Ctrl Pts',(-4.50446965905899,-0.405429628414596,
399.126862444319));
#39464=CARTESIAN_POINT('Ctrl Pts',(-4.51785871427772,-0.20278434994614,
399.119722873405));
#39465=CARTESIAN_POINT('Ctrl Pts',(-4.51766328535307,-0.00011344722995056,
399.112583302492));
#39466=CARTESIAN_POINT('Origin',(0.,0.,402.208336844637));
#39467=CARTESIAN_POINT('',(-5.07399177313997,5.16404304284901E-5,375.791663155363));
#39468=CARTESIAN_POINT('',(-5.07400718786956,-4.16755268873004E-5,375.708336844637));
#39469=CARTESIAN_POINT('',(-5.0736,-1.59740085886799E-13,402.208336844637));
#39470=CARTESIAN_POINT('',(1.3130361863572,-4.90075024188303,375.));
#39471=CARTESIAN_POINT('Ctrl Pts',(-5.07400718786956,-4.16755268873182E-5,
375.708336844637));
#39472=CARTESIAN_POINT('Ctrl Pts',(-5.07365763063996,0.800054575924722,
375.683232230984));
#39473=CARTESIAN_POINT('Ctrl Pts',(-4.67875473787853,2.4410987772414,375.631751658845));
#39474=CARTESIAN_POINT('Ctrl Pts',(-2.98728944096456,4.36266186682328,375.553895128218));
#39475=CARTESIAN_POINT('Ctrl Pts',(-0.544875549618088,5.2592655277028,375.474767252759));
#39476=CARTESIAN_POINT('Ctrl Pts',(2.02945798133318,4.88240903418803,375.395639377299));
#39477=CARTESIAN_POINT('Ctrl Pts',(4.1124194375256,3.3233956145555,375.316511501839));
#39478=CARTESIAN_POINT('Ctrl Pts',(5.19956989745793,0.959601216722932,375.237383626379));
#39479=CARTESIAN_POINT('Ctrl Pts',(5.02785240284651,-1.63637626402564,375.15825575092));
#39480=CARTESIAN_POINT('Ctrl Pts',(3.63845954881624,-3.83644847785649,375.07912787546));
#39481=CARTESIAN_POINT('Ctrl Pts',(2.1252131908655,-4.68314727417153,375.026375958487));
#39482=CARTESIAN_POINT('Ctrl Pts',(1.3130361863572,-4.90075024188303,375.));
#39483=CARTESIAN_POINT('',(-1.31318542874413,-4.90112866933894,375.));
#39484=CARTESIAN_POINT('Origin',(0.,0.,375.));
#39485=CARTESIAN_POINT('Ctrl Pts',(-5.07399177313997,5.16404304287937E-5,
375.791663155363));
#39486=CARTESIAN_POINT('Ctrl Pts',(-5.07401862443284,0.0509709830336597,
375.790065473344));
#39487=CARTESIAN_POINT('Ctrl Pts',(-5.06087568855098,0.942498320863251,
375.762091832839));
#39488=CARTESIAN_POINT('Ctrl Pts',(-4.56924148341307,2.66059337382158,375.707742233848));
#39489=CARTESIAN_POINT('Ctrl Pts',(-2.74710339271414,4.51775908713646,375.628614358388));
#39490=CARTESIAN_POINT('Ctrl Pts',(-0.25980027835232,5.28102544478076,375.549486482929));
#39491=CARTESIAN_POINT('Ctrl Pts',(2.29040909674433,4.76557955369675,375.470358607468));
#39492=CARTESIAN_POINT('Ctrl Pts',(4.28603436317887,3.09622956904483,375.391230732009));
#39493=CARTESIAN_POINT('Ctrl Pts',(5.24386820297344,0.677177255244125,375.312102856549));
#39494=CARTESIAN_POINT('Ctrl Pts',(4.93198748823577,-1.90583737857549,375.232974981089));
#39495=CARTESIAN_POINT('Ctrl Pts',(3.42590832840442,-4.02739560248487,375.153847105629));
#39496=CARTESIAN_POINT('Ctrl Pts',(1.13368018117025,-5.15247588128094,375.0761887786));
#39497=CARTESIAN_POINT('Ctrl Pts',(-0.546344062323364,-5.10618409554666,
375.024906410057));
#39498=CARTESIAN_POINT('Ctrl Pts',(-1.31318542874413,-4.90112866933894,
375.));
#39499=CARTESIAN_POINT('Origin',(0.,0.,402.208336844637));
#39500=CARTESIAN_POINT('',(-5.07342806457247,-0.000120553681964564,376.791663155363));
#39501=CARTESIAN_POINT('',(-5.0732320111606,-6.61733612274322E-5,376.708336844637));
#39502=CARTESIAN_POINT('',(-5.0736,-1.59740085886799E-13,402.208336844637));
#39503=CARTESIAN_POINT('Ctrl Pts',(-5.0732320111606,-6.61733612272383E-5,
376.708336844637));
#39504=CARTESIAN_POINT('Ctrl Pts',(-5.07300240190748,0.495753489740335,
376.692786357976));
#39505=CARTESIAN_POINT('Ctrl Pts',(-4.87836138639172,1.83273410665417,376.650859912829));
#39506=CARTESIAN_POINT('Ctrl Pts',(-3.72041242686768,3.75702756739127,376.582557509196));
#39507=CARTESIAN_POINT('Ctrl Pts',(-1.47810086816716,5.0766073897426,376.503429633736));
#39508=CARTESIAN_POINT('Ctrl Pts',(1.12210802704861,5.16697187426544,376.424301758276));
#39509=CARTESIAN_POINT('Ctrl Pts',(3.45061728097363,4.00624077340234,376.345173882816));
#39510=CARTESIAN_POINT('Ctrl Pts',(4.94361743453053,1.87546566308182,376.266046007357));
#39511=CARTESIAN_POINT('Ctrl Pts',(5.23960352937691,-0.709422013391795,
376.186918131896));
#39512=CARTESIAN_POINT('Ctrl Pts',(4.2669075188957,-3.12253502690154,376.107790256437));
#39513=CARTESIAN_POINT('Ctrl Pts',(2.26105138176727,-4.77957859502704,376.028662380977));
#39514=CARTESIAN_POINT('Ctrl Pts',(-0.292280359441297,-5.27932727476591,
375.949534505517));
#39515=CARTESIAN_POINT('Ctrl Pts',(-2.77484145645776,-4.50077558721857,
375.870406630058));
#39516=CARTESIAN_POINT('Ctrl Pts',(-4.58552092957851,-2.63243616845826,
375.791278754598));
#39517=CARTESIAN_POINT('Ctrl Pts',(-5.06368921675185,-0.921683996926001,
375.737255492791));
#39518=CARTESIAN_POINT('Ctrl Pts',(-5.07402489010486,-0.0405600539318397,
375.709608189471));
#39519=CARTESIAN_POINT('Ctrl Pts',(-5.07400718786956,-4.16755268873182E-5,
375.708336844637));
#39520=CARTESIAN_POINT('Ctrl Pts',(-5.07342806457247,-0.000120553681964737,
376.791663155363));
#39521=CARTESIAN_POINT('Ctrl Pts',(-5.07290494961689,0.587111569129446,
376.77324364185));
#39522=CARTESIAN_POINT('Ctrl Pts',(-4.82510106239333,2.01566514286781,376.728448169851));
#39523=CARTESIAN_POINT('Ctrl Pts',(-3.51189274247934,3.95263634434836,376.657276739365));
#39524=CARTESIAN_POINT('Ctrl Pts',(-1.20153141562281,5.1490821475793,376.578148863906));
#39525=CARTESIAN_POINT('Ctrl Pts',(1.39976059245402,5.09876406487689,376.499020988446));
#39526=CARTESIAN_POINT('Ctrl Pts',(3.66212404867255,3.81386577598244,376.419893112986));
#39527=CARTESIAN_POINT('Ctrl Pts',(5.03776558457334,1.60550385251465,376.340765237526));
#39528=CARTESIAN_POINT('Ctrl Pts',(5.19359667332446,-0.99160390296118,376.261637362067));
#39529=CARTESIAN_POINT('Ctrl Pts',(4.09188543028651,-3.34861140308599,376.182509486607));
#39530=CARTESIAN_POINT('Ctrl Pts',(1.99939275591558,-4.89480881330613,376.103381611147));
#39531=CARTESIAN_POINT('Ctrl Pts',(-0.577219342064538,-5.2558103583336,
376.024253735687));
#39532=CARTESIAN_POINT('Ctrl Pts',(-3.01406745721832,-4.34420557675964,
375.945125860227));
#39533=CARTESIAN_POINT('Ctrl Pts',(-4.68664255775979,-2.42036918652462,
375.867595666786));
#39534=CARTESIAN_POINT('Ctrl Pts',(-5.0735753393625,-0.789650899948463,
375.816441431831));
#39535=CARTESIAN_POINT('Ctrl Pts',(-5.07399177313997,5.16404304287937E-5,
375.791663155363));
#39536=CARTESIAN_POINT('Origin',(0.,0.,402.208336844637));
#39537=CARTESIAN_POINT('',(-5.07335325700037,0.000107956674043064,377.791663155363));
#39538=CARTESIAN_POINT('',(-5.07361435362778,0.000129215856731547,377.708336844637));
#39539=CARTESIAN_POINT('',(-5.0736,-1.59740085886799E-13,402.208336844637));
#39540=CARTESIAN_POINT('Ctrl Pts',(-5.07361435362778,0.000129215856731774,
377.708336844637));
#39541=CARTESIAN_POINT('Ctrl Pts',(-5.07380906160703,0.191278857423315,
377.702340484969));
#39542=CARTESIAN_POINT('Ctrl Pts',(-5.01660264728387,1.22311525648581,377.669968166814));
#39543=CARTESIAN_POINT('Ctrl Pts',(-4.33319923422642,3.02986949626759,377.611219890172));
#39544=CARTESIAN_POINT('Ctrl Pts',(-2.36351373006459,4.72974921277116,377.532092014713));
#39545=CARTESIAN_POINT('Ctrl Pts',(0.178456984968689,5.28439948077629,377.452964139253));
#39546=CARTESIAN_POINT('Ctrl Pts',(2.67721733402229,4.55952104001336,377.373836263793));
#39547=CARTESIAN_POINT('Ctrl Pts',(4.52773440567874,2.73063104786141,377.294708388334));
#39548=CARTESIAN_POINT('Ctrl Pts',(5.28193652635228,0.240564543316707,377.215580512874));
#39549=CARTESIAN_POINT('Ctrl Pts',(4.75720630136386,-2.3077506308472,377.136452637414));
#39550=CARTESIAN_POINT('Ctrl Pts',(3.08059835436342,-4.29728269340077,377.057324761954));
#39551=CARTESIAN_POINT('Ctrl Pts',(0.658075181053442,-5.24629982216222,
376.978196886494));
#39552=CARTESIAN_POINT('Ctrl Pts',(-1.923789860657,-4.92501343550216,376.899069011035));
#39553=CARTESIAN_POINT('Ctrl Pts',(-4.03984145181191,-3.4112176436405,376.819941135575));
#39554=CARTESIAN_POINT('Ctrl Pts',(-4.95409465736432,-1.5312714924381,376.756363746775));
#39555=CARTESIAN_POINT('Ctrl Pts',(-5.07339185365009,-0.345231048960516,
376.719162316463));
#39556=CARTESIAN_POINT('Ctrl Pts',(-5.0732320111606,-6.61733612272383E-5,
376.708336844637));
#39557=CARTESIAN_POINT('Ctrl Pts',(-5.07335325700037,0.00010795667404348,
377.791663155363));
#39558=CARTESIAN_POINT('Ctrl Pts',(-5.07357381709386,0.28275711441475,377.782797768842));
#39559=CARTESIAN_POINT('Ctrl Pts',(-4.98125011308217,1.40619065190393,377.747556423836));
#39560=CARTESIAN_POINT('Ctrl Pts',(-4.16308913613231,3.25966463764834,377.685939120343));
#39561=CARTESIAN_POINT('Ctrl Pts',(-2.1043987453421,4.85059075019948,377.606811244883));
#39562=CARTESIAN_POINT('Ctrl Pts',(0.463836508427624,5.26702766261653,377.527683369423));
#39563=CARTESIAN_POINT('Ctrl Pts',(2.91976153075723,4.40814216068722,377.448555493963));
#39564=CARTESIAN_POINT('Ctrl Pts',(4.66871526619766,2.48189896419878,377.369427618503));
#39565=CARTESIAN_POINT('Ctrl Pts',(5.28721789969248,-0.0452944421492617,
377.290299743044));
#39566=CARTESIAN_POINT('Ctrl Pts',(4.62550939154664,-2.56152055897115,377.211171867584));
#39567=CARTESIAN_POINT('Ctrl Pts',(2.84381135938942,-4.45751743210561,377.132043992124));
#39568=CARTESIAN_POINT('Ctrl Pts',(0.373532100567371,-5.27420121678766,
377.052916116664));
#39569=CARTESIAN_POINT('Ctrl Pts',(-2.18719169184094,-4.81382563128935,
376.973788241204));
#39570=CARTESIAN_POINT('Ctrl Pts',(-4.21832369780876,-3.18786290260816,
376.894660365745));
#39571=CARTESIAN_POINT('Ctrl Pts',(-4.99301148124094,-1.34818805955531,
376.833952003797));
#39572=CARTESIAN_POINT('Ctrl Pts',(-5.07365402794313,-0.253779808523861,
376.799619600337));
#39573=CARTESIAN_POINT('Ctrl Pts',(-5.07342806457247,-0.000120553681964737,
376.791663155363));
#39574=CARTESIAN_POINT('Origin',(0.,0.,402.208336844637));
#39575=CARTESIAN_POINT('',(-5.07402683453791,-2.287789782323E-5,378.791663155363));
#39576=CARTESIAN_POINT('',(-5.07385055213498,-0.000101541417780425,378.708336844637));
#39577=CARTESIAN_POINT('',(-5.0736,-1.59740085886799E-13,402.208336844637));
#39578=CARTESIAN_POINT('Ctrl Pts',(-5.07385055213498,-0.000101541417780338,
378.708336844637));
#39579=CARTESIAN_POINT('Ctrl Pts',(-5.07319426513103,0.727190265934581,
378.685518653475));
#39580=CARTESIAN_POINT('Ctrl Pts',(-4.73238867060224,2.2957670138656,378.636324503826));
#39581=CARTESIAN_POINT('Ctrl Pts',(-3.17247821056078,4.22990623671853,378.56075439569));
#39582=CARTESIAN_POINT('Ctrl Pts',(-0.770966287939471,5.23090200164121,
378.48162652023));
#39583=CARTESIAN_POINT('Ctrl Pts',(1.81722219130848,4.96532257515351,378.40249864477));
#39584=CARTESIAN_POINT('Ctrl Pts',(3.96540079385267,3.49747356130477,378.323370769311));
#39585=CARTESIAN_POINT('Ctrl Pts',(5.15342409853101,1.18276998126983,378.244242893851));
#39586=CARTESIAN_POINT('Ctrl Pts',(5.09363218664291,-1.41832151330666,378.165115018391));
#39587=CARTESIAN_POINT('Ctrl Pts',(3.80050266687247,-3.67599024033094,378.085987142931));
#39588=CARTESIAN_POINT('Ctrl Pts',(1.58714516515185,-5.04357958127442,378.006859267472));
#39589=CARTESIAN_POINT('Ctrl Pts',(-1.01051292004705,-5.18995071328536,
377.927731392012));
#39590=CARTESIAN_POINT('Ctrl Pts',(-3.36349224912901,-4.07966232156074,
377.848603516552));
#39591=CARTESIAN_POINT('Ctrl Pts',(-4.78546484347183,-2.14054821676427,
377.77547200076));
#39592=CARTESIAN_POINT('Ctrl Pts',(-5.07295260704762,-0.649523777787379,
377.728716443455));
#39593=CARTESIAN_POINT('Ctrl Pts',(-5.07361435362778,0.000129215856731774,
377.708336844637));
#39594=CARTESIAN_POINT('Ctrl Pts',(-5.07402683453791,-2.28778978229567E-5,
378.791663155363));
#39595=CARTESIAN_POINT('Ctrl Pts',(-5.07381925213896,0.818631858438491,
378.765975937348));
#39596=CARTESIAN_POINT('Ctrl Pts',(-4.66448051806342,2.47809170659261,378.713912760847));
#39597=CARTESIAN_POINT('Ctrl Pts',(-2.9391988257698,4.39520590733944,378.63547362586));
#39598=CARTESIAN_POINT('Ctrl Pts',(-0.487090471470337,5.2649280695866,378.5563457504));
#39599=CARTESIAN_POINT('Ctrl Pts',(2.08295867142411,4.85983619872698,378.47721787494));
#39600=CARTESIAN_POINT('Ctrl Pts',(4.1486543056634,3.27801649742928,378.398089999481));
#39601=CARTESIAN_POINT('Ctrl Pts',(5.20982287752563,0.902480077413658,378.318962124021));
#39602=CARTESIAN_POINT('Ctrl Pts',(5.00952021436078,-1.69157675771122,378.239834248561));
#39603=CARTESIAN_POINT('Ctrl Pts',(3.59624624674644,-3.8760466506584,378.160706373101));
#39604=CARTESIAN_POINT('Ctrl Pts',(1.31220156369858,-5.12199685294173,378.081578497641));
#39605=CARTESIAN_POINT('Ctrl Pts',(-1.28957072085835,-5.12774141910675,
378.002450622182));
#39606=CARTESIAN_POINT('Ctrl Pts',(-3.57909508295452,-3.89188939879962,
377.923322746722));
#39607=CARTESIAN_POINT('Ctrl Pts',(-4.84258096039032,-1.9577252596909,377.853060257782));
#39608=CARTESIAN_POINT('Ctrl Pts',(-5.07291761514975,-0.558169836019873,
377.809173727329));
#39609=CARTESIAN_POINT('Ctrl Pts',(-5.07335325700037,0.00010795667404348,
377.791663155363));
#39610=CARTESIAN_POINT('Origin',(0.,0.,402.208336844637));
#39611=CARTESIAN_POINT('',(-5.07326152951467,-8.03441847486985E-5,379.791663155363));
#39612=CARTESIAN_POINT('',(-5.07317735229637,-2.23272941127382E-6,379.708336844637));
#39613=CARTESIAN_POINT('',(-5.0736,-1.59740085886799E-13,402.208336844637));
#39614=CARTESIAN_POINT('Ctrl Pts',(-5.07317735229636,-2.23272941118208E-6,
379.708336844637));
#39615=CARTESIAN_POINT('Ctrl Pts',(-5.07317083223754,0.422929008539474,
379.695072780467));
#39616=CARTESIAN_POINT('Ctrl Pts',(-4.91684325738401,1.68687545589345,379.65543275781));
#39617=CARTESIAN_POINT('Ctrl Pts',(-3.87882817196482,3.59324599495851,379.589416776668));
#39618=CARTESIAN_POINT('Ctrl Pts',(-1.69545248338881,5.00820982432685,379.510288901207));
#39619=CARTESIAN_POINT('Ctrl Pts',(0.898448589337301,5.21051963821565,379.431161025747));
#39620=CARTESIAN_POINT('Ctrl Pts',(3.27480540417913,4.15118950816177,379.352033150288));
#39621=CARTESIAN_POINT('Ctrl Pts',(4.85822301267979,2.08671845896413,379.272905274828));
#39622=CARTESIAN_POINT('Ctrl Pts',(5.26530339668872,-0.483016468385486,
379.193777399368));
#39623=CARTESIAN_POINT('Ctrl Pts',(4.39747886842774,-2.93579705866137,379.114649523908));
#39624=CARTESIAN_POINT('Ctrl Pts',(2.4648785829925,-4.67772362790043,379.035521648449));
#39625=CARTESIAN_POINT('Ctrl Pts',(-0.0645507124447473,-5.28701787148826,
378.956393772989));
#39626=CARTESIAN_POINT('Ctrl Pts',(-2.57835013545374,-4.61614940691036,
378.877265897529));
#39627=CARTESIAN_POINT('Ctrl Pts',(-4.46784531508162,-2.82755778162292,
378.798138022069));
#39628=CARTESIAN_POINT('Ctrl Pts',(-5.04261473172305,-1.0675305862618,378.741828337772));
#39629=CARTESIAN_POINT('Ctrl Pts',(-5.07395287910916,-0.113499444385656,
378.711894611961));
#39630=CARTESIAN_POINT('Ctrl Pts',(-5.07385055213498,-0.000101541417780338,
378.708336844637));
#39631=CARTESIAN_POINT('Ctrl Pts',(-5.07326152951467,-8.03441847485598E-5,
379.791663155363));
#39632=CARTESIAN_POINT('Ctrl Pts',(-5.07297012272296,0.514306801455685,
379.775530064341));
#39633=CARTESIAN_POINT('Ctrl Pts',(-4.86799754311315,1.86989152588461,379.733021014832));
#39634=CARTESIAN_POINT('Ctrl Pts',(-3.67892986111526,3.7976571438602,379.664136006837));
#39635=CARTESIAN_POINT('Ctrl Pts',(-1.42226240084736,5.09253319757995,379.585008131377));
#39636=CARTESIAN_POINT('Ctrl Pts',(1.17878204679748,5.15433774518764,379.505880255918));
#39637=CARTESIAN_POINT('Ctrl Pts',(3.49440419135096,3.9681058520139,379.426752380457));
#39638=CARTESIAN_POINT('Ctrl Pts',(4.96391496617568,1.82106367650753,379.347624504998));
#39639=CARTESIAN_POINT('Ctrl Pts',(5.2314969825461,-0.766918526917405,379.268496629538));
#39640=CARTESIAN_POINT('Ctrl Pts',(4.23235974285854,-3.16920427116154,379.189368754078));
#39641=CARTESIAN_POINT('Ctrl Pts',(2.20842757301423,-4.80412035237133,379.110240878619));
#39642=CARTESIAN_POINT('Ctrl Pts',(-0.350238295746339,-5.27579926091873,
379.031113003158));
#39643=CARTESIAN_POINT('Ctrl Pts',(-2.82409983509395,-4.47003185970082,
378.951985127699));
#39644=CARTESIAN_POINT('Ctrl Pts',(-4.61415296279982,-2.58192121126957,
378.872857252239));
#39645=CARTESIAN_POINT('Ctrl Pts',(-5.06855147600533,-0.884525550463806,
378.819416594794));
#39646=CARTESIAN_POINT('Ctrl Pts',(-5.07403240035665,-0.0219731198176094,
378.792351895835));
#39647=CARTESIAN_POINT('Ctrl Pts',(-5.07402683453791,-2.28778978229567E-5,
378.791663155363));
#39648=CARTESIAN_POINT('Origin',(0.,0.,402.208336844637));
#39649=CARTESIAN_POINT('',(-5.07355665554129,0.000129459885802874,380.791663155363));
#39650=CARTESIAN_POINT('',(-5.07383699511133,0.000104483598321417,380.708336844637));
#39651=CARTESIAN_POINT('',(-5.0736,-1.59740085886799E-13,402.208336844637));
#39652=CARTESIAN_POINT('Ctrl Pts',(-5.07383699511133,0.000104483598321794,
380.708336844637));
#39653=CARTESIAN_POINT('Ctrl Pts',(-5.07394580731281,0.118353460768718,
380.704626907459));
#39654=CARTESIAN_POINT('Ctrl Pts',(-5.04109883614377,1.0772383012794,380.674541011795));
#39655=CARTESIAN_POINT('Ctrl Pts',(-4.45971656638884,2.84036140577044,380.618079157644));
#39656=CARTESIAN_POINT('Ctrl Pts',(-2.56509888808806,4.6235259772432,380.538951282184));
#39657=CARTESIAN_POINT('Ctrl Pts',(-0.0493855337170155,5.28718127521391,
380.459823406725));
#39658=CARTESIAN_POINT('Ctrl Pts',(2.47828569939099,4.67063429954727,380.380695531265));
#39659=CARTESIAN_POINT('Ctrl Pts',(4.40588161411396,2.92317156019379,380.301567655805));
#39660=CARTESIAN_POINT('Ctrl Pts',(5.26666718771851,0.467911852513223,380.222439780345));
#39661=CARTESIAN_POINT('Ctrl Pts',(4.8522176299277,-2.10064486282949,380.143311904886));
#39662=CARTESIAN_POINT('Ctrl Pts',(3.26288495036134,-4.1605656548862,380.064184029426));
#39663=CARTESIAN_POINT('Ctrl Pts',(0.883499402425967,-5.21307525111868,
379.985056153966));
#39664=CARTESIAN_POINT('Ctrl Pts',(-1.70981070849824,-5.0033261046046,379.905928278506));
#39665=CARTESIAN_POINT('Ctrl Pts',(-3.88911883186622,-3.58210545343612,
379.826800403046));
#39666=CARTESIAN_POINT('Ctrl Pts',(-4.91928148884334,-1.67716650260946,
379.760936591757));
#39667=CARTESIAN_POINT('Ctrl Pts',(-5.07318379755486,-0.418081463015616,
379.721448738954));
#39668=CARTESIAN_POINT('Ctrl Pts',(-5.07317735229636,-2.23272941118208E-6,
379.708336844637));
#39669=CARTESIAN_POINT('Ctrl Pts',(-5.07355665554129,0.000129459885803325,
380.791663155363));
#39670=CARTESIAN_POINT('Ctrl Pts',(-5.07376606808144,0.209858000324401,
380.785084191333));
#39671=CARTESIAN_POINT('Ctrl Pts',(-5.00984200321542,1.26028988400143,380.752129268817));
#39672=CARTESIAN_POINT('Ctrl Pts',(-4.29966508516876,3.07727230850615,380.692798387814));
#39673=CARTESIAN_POINT('Ctrl Pts',(-2.31143093395199,4.75541919738815,380.613670512354));
#39674=CARTESIAN_POINT('Ctrl Pts',(0.236477452546483,5.28212108151216,380.534542636895));
#39675=CARTESIAN_POINT('Ctrl Pts',(2.7271267899117,4.52984593303835,380.455414761435));
#39676=CARTESIAN_POINT('Ctrl Pts',(4.55744811217567,2.68074456264382,380.376286885975));
#39677=CARTESIAN_POINT('Ctrl Pts',(5.28425980776137,0.182545855597361,380.297159010515));
#39678=CARTESIAN_POINT('Ctrl Pts',(4.73157661405697,-2.35985326887651,380.218031135055));
#39679=CARTESIAN_POINT('Ctrl Pts',(3.03322149728047,-4.33085350176541,380.138903259596));
#39680=CARTESIAN_POINT('Ctrl Pts',(0.600422665576261,-5.25321019263273,
380.059775384136));
#39681=CARTESIAN_POINT('Ctrl Pts',(-1.97775844481349,-4.90359013777528,
379.980647508676));
#39682=CARTESIAN_POINT('Ctrl Pts',(-4.07705851709219,-3.36664796994342,
379.901519633216));
#39683=CARTESIAN_POINT('Ctrl Pts',(-4.96242349460837,-1.49409344074893,
379.838524848778));
#39684=CARTESIAN_POINT('Ctrl Pts',(-5.07344654310827,-0.326663721856642,
379.801906022827));
#39685=CARTESIAN_POINT('Ctrl Pts',(-5.07326152951467,-8.03441847485598E-5,
379.791663155363));
#39686=CARTESIAN_POINT('Origin',(0.,0.,402.208336844637));
#39687=CARTESIAN_POINT('',(-5.07389966860957,-8.89210953775033E-5,381.791663155363));
#39688=CARTESIAN_POINT('',(-5.0736295665075,-0.000128745637012367,381.708336844637));
#39689=CARTESIAN_POINT('',(-5.0736,-1.59740085886799E-13,402.208336844637));
#39690=CARTESIAN_POINT('Ctrl Pts',(-5.0736295665075,-0.000128745637012449,
381.708336844637));
#39691=CARTESIAN_POINT('Ctrl Pts',(-5.07296124918876,0.654369409793758,
381.687805075965));
#39692=CARTESIAN_POINT('Ctrl Pts',(-4.78227571732073,2.15023935796871,381.640897348807));
#39693=CARTESIAN_POINT('Ctrl Pts',(-3.35177659407457,4.08929314568265,381.567613663161));
#39694=CARTESIAN_POINT('Ctrl Pts',(-0.995622270609436,5.1928278483096,381.488485787702));
#39695=CARTESIAN_POINT('Ctrl Pts',(1.60160528794473,5.03900637720777,381.409357912242));
#39696=CARTESIAN_POINT('Ctrl Pts',(3.81103098679937,3.66507402184023,381.330230036782));
#39697=CARTESIAN_POINT('Ctrl Pts',(5.09767944760569,1.40370545962173,381.251102161322));
#39698=CARTESIAN_POINT('Ctrl Pts',(5.15001032416474,-1.1975468378773,381.171974285863));
#39699=CARTESIAN_POINT('Ctrl Pts',(3.95535257236717,-3.50883325283227,381.092846410403));
#39700=CARTESIAN_POINT('Ctrl Pts',(1.8029725310162,-4.97051454281288,381.013718534943));
#39701=CARTESIAN_POINT('Ctrl Pts',(-0.785967070782117,-5.22866909753901,
380.934590659483));
#39702=CARTESIAN_POINT('Ctrl Pts',(-3.18459792796892,-4.22078912113472,
380.855462784024));
#39703=CARTESIAN_POINT('Ctrl Pts',(-4.73582433047741,-2.28608714092918,
380.780044845741));
#39704=CARTESIAN_POINT('Ctrl Pts',(-5.07317220227002,-0.722342746081139,
380.731002865946));
#39705=CARTESIAN_POINT('Ctrl Pts',(-5.07383699511133,0.000104483598321794,
380.708336844637));
#39706=CARTESIAN_POINT('Ctrl Pts',(-5.07389966860957,-8.89210953773471E-5,
381.791663155363));
#39707=CARTESIAN_POINT('Ctrl Pts',(-5.07328829289394,0.745751527323211,
381.768262359839));
#39708=CARTESIAN_POINT('Ctrl Pts',(-4.71908116243226,2.33281964194823,381.718485605828));
#39709=CARTESIAN_POINT('Ctrl Pts',(-3.12583571520092,4.26449009693918,381.642332893332));
#39710=CARTESIAN_POINT('Ctrl Pts',(-0.713476057932961,5.23905302703404,
381.563205017871));
#39711=CARTESIAN_POINT('Ctrl Pts',(1.87163986094335,4.94506713162178,381.484077142412));
#39712=CARTESIAN_POINT('Ctrl Pts',(4.00356957706116,3.45371616479241,381.404949266952));
#39713=CARTESIAN_POINT('Ctrl Pts',(5.16610206459392,1.12610575148009,381.325821391492));
#39714=CARTESIAN_POINT('Ctrl Pts',(5.07774957870228,-1.47417228345499,381.246693516033));
#39715=CARTESIAN_POINT('Ctrl Pts',(3.75990519207135,-3.71750422352859,381.167565640573));
#39716=CARTESIAN_POINT('Ctrl Pts',(1.53166282114666,-5.06070486272762,381.088437765113));
#39717=CARTESIAN_POINT('Ctrl Pts',(-1.0674460141586,-5.17854069330105,381.009309889653));
#39718=CARTESIAN_POINT('Ctrl Pts',(-3.40809069944175,-4.04247974511891,
380.930182014193));
#39719=CARTESIAN_POINT('Ctrl Pts',(-4.79752508832052,-2.10343849769112,
380.857633102763));
#39720=CARTESIAN_POINT('Ctrl Pts',(-5.07292650482488,-0.630972144226672,
380.81146014982));
#39721=CARTESIAN_POINT('Ctrl Pts',(-5.07355665554129,0.000129459885803325,
380.791663155363));
#39722=CARTESIAN_POINT('Origin',(0.,0.,402.208336844637));
#39723=CARTESIAN_POINT('',(-5.0731816081447,-1.92612327425123E-5,382.791663155363));
#39724=CARTESIAN_POINT('',(-5.07322528972955,6.22763117692481E-5,382.708336844637));
#39725=CARTESIAN_POINT('',(-5.0736,-1.59740085886799E-13,402.208336844637));
#39726=CARTESIAN_POINT('Ctrl Pts',(-5.07322528972955,6.22763117691383E-5,
382.708336844637));
#39727=CARTESIAN_POINT('Ctrl Pts',(-5.07337757676184,0.350080340895845,
382.697359202958));
#39728=CARTESIAN_POINT('Ctrl Pts',(-4.95188321010373,1.54098189440445,382.660005602791));
#39729=CARTESIAN_POINT('Ctrl Pts',(-4.03004033454984,3.42279121037416,382.596276044139));
#39730=CARTESIAN_POINT('Ctrl Pts',(-1.90965538190854,4.93051124025298,382.517148168679));
#39731=CARTESIAN_POINT('Ctrl Pts',(0.673120594328623,5.24439066369047,382.438020293219));
#39732=CARTESIAN_POINT('Ctrl Pts',(3.09291170766135,4.28842884242289,382.35889241776));
#39733=CARTESIAN_POINT('Ctrl Pts',(4.76380612269667,2.29409589888282,382.2797645423));
#39734=CARTESIAN_POINT('Ctrl Pts',(5.28122477966896,-0.255713891925586,
382.20063666684));
#39735=CARTESIAN_POINT('Ctrl Pts',(4.51988342850276,-2.74360685242242,382.12150879138));
#39736=CARTESIAN_POINT('Ctrl Pts',(2.66412810880644,-4.56718142707082,382.04238091592));
#39737=CARTESIAN_POINT('Ctrl Pts',(0.16329884807764,-5.28488961607806,381.96325304046));
#39738=CARTESIAN_POINT('Ctrl Pts',(-2.37707049000228,-4.72295041827389,
381.884125165001));
#39739=CARTESIAN_POINT('Ctrl Pts',(-4.3418720751543,-3.0174279860352,381.804997289541));
#39740=CARTESIAN_POINT('Ctrl Pts',(-5.01833358746616,-1.21340586700331,
381.746401182753));
#39741=CARTESIAN_POINT('Ctrl Pts',(-5.07381979723383,-0.186425967023143,
381.714181034452));
#39742=CARTESIAN_POINT('Ctrl Pts',(-5.0736295665075,-0.000128745637012449,
381.708336844637));
#39743=CARTESIAN_POINT('Ctrl Pts',(-5.0731816081447,-1.92612327423736E-5,
382.791663155363));
#39744=CARTESIAN_POINT('Ctrl Pts',(-5.07312283046122,0.441487546406695,
382.777816486831));
#39745=CARTESIAN_POINT('Ctrl Pts',(-4.90736705066614,1.72404611325897,382.737593859813));
#39746=CARTESIAN_POINT('Ctrl Pts',(-3.83913463932894,3.63562510806912,382.670995274309));
#39747=CARTESIAN_POINT('Ctrl Pts',(-1.64035202533435,5.0265266276326,382.591867398849));
#39748=CARTESIAN_POINT('Ctrl Pts',(0.955614320991023,5.2003390249901,382.512739523389));
#39749=CARTESIAN_POINT('Ctrl Pts',(3.32019468624774,4.11497654315675,382.433611647929));
#39750=CARTESIAN_POINT('Ctrl Pts',(4.8808455917412,2.03324150432223,382.354483772469));
#39751=CARTESIAN_POINT('Ctrl Pts',(5.25968159463003,-0.540808864968189,
382.27535589701));
#39752=CARTESIAN_POINT('Ctrl Pts',(4.36497391033337,-2.98391143759783,382.19622802155));
#39753=CARTESIAN_POINT('Ctrl Pts',(2.41336099931917,-4.70450989926509,382.11710014609));
#39754=CARTESIAN_POINT('Ctrl Pts',(-0.122606802820077,-5.28599018890692,
382.03797227063));
#39755=CARTESIAN_POINT('Ctrl Pts',(-2.6288874239146,-4.58755660648474,381.958844395171));
#39756=CARTESIAN_POINT('Ctrl Pts',(-4.49862704479611,-2.77832313044165,
381.879716519711));
#39757=CARTESIAN_POINT('Ctrl Pts',(-5.04828738596174,-1.03036438158544,
381.823989439775));
#39758=CARTESIAN_POINT('Ctrl Pts',(-5.07397739854758,-0.0949146237502798,
381.794638318325));
#39759=CARTESIAN_POINT('Ctrl Pts',(-5.07389966860957,-8.89210953773471E-5,
381.791663155363));
#39760=CARTESIAN_POINT('Origin',(0.,0.,402.208336844637));
#39761=CARTESIAN_POINT('',(-5.07378290535392,0.000114313540020838,383.791663155363));
#39762=CARTESIAN_POINT('',(-5.07400033060213,4.63270069165547E-5,383.708336844637));
#39763=CARTESIAN_POINT('',(-5.0736,-1.59740085886799E-13,402.208336844637));
#39764=CARTESIAN_POINT('Ctrl Pts',(-5.07400033060213,4.63270069167923E-5,
383.708336844637));
#39765=CARTESIAN_POINT('Ctrl Pts',(-5.0740221098109,0.0454146017487004,
383.70691332995));
#39766=CARTESIAN_POINT('Ctrl Pts',(-5.06238522132993,0.931389441082911,
383.679113856776));
#39767=CARTESIAN_POINT('Ctrl Pts',(-4.57795151673967,2.64557832586642,383.624938425116));
#39768=CARTESIAN_POINT('Ctrl Pts',(-2.76192026167378,4.50871614055144,383.545810549656));
#39769=CARTESIAN_POINT('Ctrl Pts',(-0.277136335846315,5.28014395819535,
383.466682674197));
#39770=CARTESIAN_POINT('Ctrl Pts',(2.27475150580887,4.77307347049397,383.387554798736));
#39771=CARTESIAN_POINT('Ctrl Pts',(4.27584642055071,3.11028329188466,383.308426923277));
#39772=CARTESIAN_POINT('Ctrl Pts',(5.24161683545466,0.6943901771998,383.229299047817));
#39773=CARTESIAN_POINT('Ctrl Pts',(4.93821764164047,-1.8896378731662,383.150171172357));
#39774=CARTESIAN_POINT('Ctrl Pts',(3.43911186553428,-4.01612180396144,383.071043296897));
#39775=CARTESIAN_POINT('Ctrl Pts',(1.1072828290795,-5.17016919494313,382.991915421438));
#39776=CARTESIAN_POINT('Ctrl Pts',(-1.49265617402097,-5.07234682509687,
382.912787545978));
#39777=CARTESIAN_POINT('Ctrl Pts',(-3.73117351815568,-3.74634074068643,
382.833659670518));
#39778=CARTESIAN_POINT('Ctrl Pts',(-4.88103073617416,-1.82302830121342,
382.765509436738));
#39779=CARTESIAN_POINT('Ctrl Pts',(-5.07301167700312,-0.490907387666408,
382.723735161444));
#39780=CARTESIAN_POINT('Ctrl Pts',(-5.07322528972955,6.22763117691383E-5,
382.708336844637));
#39781=CARTESIAN_POINT('Ctrl Pts',(-5.07378290535392,0.000114313540020942,
383.791663155363));
#39782=CARTESIAN_POINT('Ctrl Pts',(-5.07391625780791,0.136937191492554,
383.787370613824));
#39783=CARTESIAN_POINT('Ctrl Pts',(-5.03516348602304,1.11440684342152,383.756702113798));
#39784=CARTESIAN_POINT('Ctrl Pts',(-4.42825589269063,2.88916500985471,383.699657655286));
#39785=CARTESIAN_POINT('Ctrl Pts',(-2.51417043865664,4.65141609735177,383.620529779826));
#39786=CARTESIAN_POINT('Ctrl Pts',(0.00867922154690349,5.28740478651213,
383.541401904366));
#39787=CARTESIAN_POINT('Ctrl Pts',(2.52942735381344,4.6431370825228,383.462274028906));
#39788=CARTESIAN_POINT('Ctrl Pts',(4.43771707378134,2.87461160478899,383.383146153446));
#39789=CARTESIAN_POINT('Ctrl Pts',(5.27148802998996,0.410047137522666,383.304018277987));
#39790=CARTESIAN_POINT('Ctrl Pts',(4.82885656869832,-2.15380336712922,383.224890402527));
#39791=CARTESIAN_POINT('Ctrl Pts',(3.2169984748157,-4.19614650820864,383.145762527067));
#39792=CARTESIAN_POINT('Ctrl Pts',(0.82619815304806,-5.22246314656389,383.066634651607));
#39793=CARTESIAN_POINT('Ctrl Pts',(-1.76465219517988,-4.98424792073636,
382.987506776148));
#39794=CARTESIAN_POINT('Ctrl Pts',(-3.92822160960685,-3.5391806525149,382.908378900688));
#39795=CARTESIAN_POINT('Ctrl Pts',(-4.9284760402056,-1.63999308805888,382.84309769376));
#39796=CARTESIAN_POINT('Ctrl Pts',(-5.07323479369165,-0.399520902907398,
382.804192445318));
#39797=CARTESIAN_POINT('Ctrl Pts',(-5.0731816081447,-1.92612327423736E-5,
382.791663155363));
#39798=CARTESIAN_POINT('Origin',(0.,0.,402.208336844637));
#39799=CARTESIAN_POINT('',(-5.07368788828891,-0.000125377980982264,384.791663155363));
#39800=CARTESIAN_POINT('',(-5.07341299508847,-0.000118529377325131,384.708336844637));
#39801=CARTESIAN_POINT('',(-5.0736,-1.59740085886799E-13,402.208336844637));
#39802=CARTESIAN_POINT('Ctrl Pts',(-5.07341299508847,-0.000118529377325025,
384.708336844637));
#39803=CARTESIAN_POINT('Ctrl Pts',(-5.07290585727583,0.581565929821983,
384.690091498456));
#39804=CARTESIAN_POINT('Ctrl Pts',(-4.82849439364024,2.00456420438781,384.645470193788));
#39805=CARTESIAN_POINT('Ctrl Pts',(-3.52485021126398,3.94108560628483,384.574472930633));
#39806=CARTESIAN_POINT('Ctrl Pts',(-1.21842922909547,5.14510981239459,384.495345055173));
#39807=CARTESIAN_POINT('Ctrl Pts',(1.38301395642869,5.10333196688562,384.416217179714));
#39808=CARTESIAN_POINT('Ctrl Pts',(3.64958350715001,3.82586787438508,384.337089304254));
#39809=CARTESIAN_POINT('Ctrl Pts',(5.03246761935876,1.62203404033908,384.257961428794));
#39810=CARTESIAN_POINT('Ctrl Pts',(5.19682409785237,-0.974548133184912,
384.178833553334));
#39811=CARTESIAN_POINT('Ctrl Pts',(4.10285677781212,-3.33515982055948,384.099705677875));
#39812=CARTESIAN_POINT('Ctrl Pts',(2.0154514986864,-4.88821849187982,384.020577802414));
#39813=CARTESIAN_POINT('Ctrl Pts',(-0.559961559389509,-5.25767703647906,
383.941449926955));
#39814=CARTESIAN_POINT('Ctrl Pts',(-2.99978931706339,-4.3540772640303,383.862322051495));
#39815=CARTESIAN_POINT('Ctrl Pts',(-4.68244282170845,-2.43143282852321,
383.784617690723));
#39816=CARTESIAN_POINT('Ctrl Pts',(-5.0736185681322,-0.795203160750922,
383.733289288436));
#39817=CARTESIAN_POINT('Ctrl Pts',(-5.07400033060213,4.63270069167923E-5,
383.708336844637));
#39818=CARTESIAN_POINT('Ctrl Pts',(-5.07368788828891,-0.000125377980982003,
384.791663155363));
#39819=CARTESIAN_POINT('Ctrl Pts',(-5.07300172207351,0.67292236196844,384.770548782329));
#39820=CARTESIAN_POINT('Ctrl Pts',(-4.76991529656479,2.18733716132669,384.72305845081));
#39821=CARTESIAN_POINT('Ctrl Pts',(-3.30666744538294,4.12585447040522,384.649192160803));
#39822=CARTESIAN_POINT('Ctrl Pts',(-0.93853660926441,5.20344825460853,384.570064285343));
#39823=CARTESIAN_POINT('Ctrl Pts',(1.65684512644118,5.02111431181428,384.490936409884));
#39824=CARTESIAN_POINT('Ctrl Pts',(3.85104960199139,3.62300174831864,384.411808534424));
#39825=CARTESIAN_POINT('Ctrl Pts',(5.11278700298303,1.34764007340457,384.332680658964));
#39826=CARTESIAN_POINT('Ctrl Pts',(5.13654877856401,-1.25403004379905,384.253552783504));
#39827=CARTESIAN_POINT('Ctrl Pts',(3.91658141328989,-3.55205781743347,384.174424908044));
#39828=CARTESIAN_POINT('Ctrl Pts',(1.74827954439566,-4.99001436270134,384.095297032584));
#39829=CARTESIAN_POINT('Ctrl Pts',(-0.843338895500463,-5.21972261836337,
384.016169157125));
#39830=CARTESIAN_POINT('Ctrl Pts',(-3.23075696562154,-4.18556258278454,
383.937041281665));
#39831=CARTESIAN_POINT('Ctrl Pts',(-4.74882528908407,-2.24901858620394,
383.862205947744));
#39832=CARTESIAN_POINT('Ctrl Pts',(-5.07309686007849,-0.703784911249602,
383.81374657231));
#39833=CARTESIAN_POINT('Ctrl Pts',(-5.07378290535392,0.000114313540020942,
383.791663155363));
#39834=CARTESIAN_POINT('Origin',(0.,0.,402.208336844637));
#39835=CARTESIAN_POINT('',(-5.07320349191978,4.67301704154544E-5,385.791663155363));
#39836=CARTESIAN_POINT('',(-5.07336681616767,0.000110749500208817,385.708336844637));
#39837=CARTESIAN_POINT('',(-5.0736,-1.59740085886799E-13,402.208336844637));
#39838=CARTESIAN_POINT('Ctrl Pts',(-5.07336681616767,0.000110749500209159,
385.708336844637));
#39839=CARTESIAN_POINT('Ctrl Pts',(-5.07358949400792,0.277204924762013,
385.699645625448));
#39840=CARTESIAN_POINT('Ctrl Pts',(-4.98354435800546,1.39507636552693,385.664578447772));
#39841=CARTESIAN_POINT('Ctrl Pts',(-4.1737680903862,3.24597977436508,385.60313531161));
#39842=CARTESIAN_POINT('Ctrl Pts',(-2.12031175571847,4.84365593601313,385.524007436151));
#39843=CARTESIAN_POINT('Ctrl Pts',(0.446542510511727,5.26852204647746,385.44487956069));
#39844=CARTESIAN_POINT('Ctrl Pts',(2.90527399685678,4.41770390260608,385.365751685231));
#39845=CARTESIAN_POINT('Ctrl Pts',(4.66054210967394,2.4972128487314,385.286623809771));
#39846=CARTESIAN_POINT('Ctrl Pts',(5.2873381133244,-0.0279364153108744,
385.207495934311));
#39847=CARTESIAN_POINT('Ctrl Pts',(4.63389386761938,-2.54632134491165,385.128368058852));
#39848=CARTESIAN_POINT('Ctrl Pts',(2.85842993763932,-4.44815726560116,385.049240183392));
#39849=CARTESIAN_POINT('Ctrl Pts',(0.390845137441743,-5.27294650517633,
384.970112307932));
#39850=CARTESIAN_POINT('Ctrl Pts',(-2.1713762578616,-4.82098018194518,384.890984432472));
#39851=CARTESIAN_POINT('Ctrl Pts',(-4.20783530881936,-3.2016943610792,384.811856557012));
#39852=CARTESIAN_POINT('Ctrl Pts',(-4.99079834853979,-1.35930215545066,
384.750974027734));
#39853=CARTESIAN_POINT('Ctrl Pts',(-5.07363898920769,-0.259332620176451,
384.716467456942));
#39854=CARTESIAN_POINT('Ctrl Pts',(-5.07341299508847,-0.000118529377325025,
384.708336844637));
#39855=CARTESIAN_POINT('Ctrl Pts',(-5.07320349191978,4.6730170415385E-5,
385.791663155363));
#39856=CARTESIAN_POINT('Ctrl Pts',(-5.07332318093048,0.368645452041058,
385.780102909322));
#39857=CARTESIAN_POINT('Ctrl Pts',(-4.94327787593756,1.57815905047111,385.742166704794));
#39858=CARTESIAN_POINT('Ctrl Pts',(-3.99220955212729,3.46684115546438,385.67785454178));
#39859=CARTESIAN_POINT('Ctrl Pts',(-1.85539526299902,4.95118502212943,385.59872666632));
#39860=CARTESIAN_POINT('Ctrl Pts',(0.73067187193628,5.23668247279509,385.51959879086));
#39861=CARTESIAN_POINT('Ctrl Pts',(3.13981906729605,4.25420508790564,385.440470915401));
#39862=CARTESIAN_POINT('Ctrl Pts',(4.78871173391359,2.24164328892807,385.361343039941));
#39863=CARTESIAN_POINT('Ctrl Pts',(5.27809816640793,-0.313694837508304,
385.282215164481));
#39864=CARTESIAN_POINT('Ctrl Pts',(4.48948164772799,-2.79307702006795,385.203087289022));
#39865=CARTESIAN_POINT('Ctrl Pts',(2.61381244185943,-4.59616244535579,385.123959413562));
#39866=CARTESIAN_POINT('Ctrl Pts',(0.105252389857621,-5.28636421747,385.044831538102));
#39867=CARTESIAN_POINT('Ctrl Pts',(-2.42879276314368,-4.69656155277656,
384.965703662642));
#39868=CARTESIAN_POINT('Ctrl Pts',(-4.3747464822184,-2.96956527485689,384.886575787182));
#39869=CARTESIAN_POINT('Ctrl Pts',(-5.02482764874857,-1.17623295765146,
384.828562284756));
#39870=CARTESIAN_POINT('Ctrl Pts',(-5.0738588771301,-0.167845167351579,
384.796924740816));
#39871=CARTESIAN_POINT('Ctrl Pts',(-5.07368788828891,-0.000125377980982003,
384.791663155363));
#39872=CARTESIAN_POINT('Origin',(0.,0.,402.208336844637));
#39873=CARTESIAN_POINT('',(-5.07396871057133,6.36451556410011E-5,386.791663155363));
#39874=CARTESIAN_POINT('',(-5.07402204930561,-2.85592496231871E-5,386.708336844637));
#39875=CARTESIAN_POINT('',(-5.0736,-1.59740085886799E-13,402.208336844637));
#39876=CARTESIAN_POINT('Ctrl Pts',(-5.07402204930561,-2.85592496232024E-5,
386.708336844637));
#39877=CARTESIAN_POINT('Ctrl Pts',(-5.07376894837123,0.813077680770696,
386.682823793954));
#39878=CARTESIAN_POINT('Ctrl Pts',(-4.66877404608003,2.46703434122352,386.630934784784));
#39879=CARTESIAN_POINT('Ctrl Pts',(-2.95361232316089,4.38553292227813,386.552669817127));
#39880=CARTESIAN_POINT('Ctrl Pts',(-0.504372453036948,5.26330059910421,
386.473541941668));
#39881=CARTESIAN_POINT('Ctrl Pts',(2.06699274767947,4.86664830750627,386.394414066208));
#39882=CARTESIAN_POINT('Ctrl Pts',(4.1378703204085,3.29161874757629,386.315286190749));
#39883=CARTESIAN_POINT('Ctrl Pts',(5.20683199193,0.919578912180737,386.236158315288));
#39884=CARTESIAN_POINT('Ctrl Pts',(5.01504662121074,-1.67512153439562,386.157030439829));
#39885=CARTESIAN_POINT('Ctrl Pts',(3.60895181930755,-3.86421939514695,386.077902564369));
#39886=CARTESIAN_POINT('Ctrl Pts',(1.32900986066236,-5.11766133679979,385.998774688909));
#39887=CARTESIAN_POINT('Ctrl Pts',(-1.2727295467071,-5.13194741485647,385.91964681345));
#39888=CARTESIAN_POINT('Ctrl Pts',(-3.5662988394905,-3.90361849510962,385.84051893799));
#39889=CARTESIAN_POINT('Ctrl Pts',(-4.83927537814081,-1.96882864770619,
385.770082281719));
#39890=CARTESIAN_POINT('Ctrl Pts',(-5.07291371523136,-0.563715584161085,
385.726021583935));
#39891=CARTESIAN_POINT('Ctrl Pts',(-5.07336681616767,0.000110749500209159,
385.708336844637));
#39892=CARTESIAN_POINT('Ctrl Pts',(-5.07396871057133,6.36451556408537E-5,
386.791663155363));
#39893=CARTESIAN_POINT('Ctrl Pts',(-5.07400891965194,0.0640010310039327,
386.789657036314));
#39894=CARTESIAN_POINT('Ctrl Pts',(-5.05726353871135,0.968550309919132,
386.761274958779));
#39895=CARTESIAN_POINT('Ctrl Pts',(-4.54862274572651,2.695692085973,386.706516922757));
#39896=CARTESIAN_POINT('Ctrl Pts',(-2.71224074091265,4.53877459989496,386.627389047297));
#39897=CARTESIAN_POINT('Ctrl Pts',(-0.219135128106394,5.28286896496098,
386.548261171838));
#39898=CARTESIAN_POINT('Ctrl Pts',(2.32703038082081,4.74780520999492,386.469133296378));
#39899=CARTESIAN_POINT('Ctrl Pts',(4.30974451002784,3.06314004962277,386.390005420918));
#39900=CARTESIAN_POINT('Ctrl Pts',(5.24892628554031,0.636786898642001,386.310877545458));
#39901=CARTESIAN_POINT('Ctrl Pts',(4.91716859158436,-1.94375352019086,386.231749669999));
#39902=CARTESIAN_POINT('Ctrl Pts',(3.39480098979053,-4.05364662310803,386.152621794539));
#39903=CARTESIAN_POINT('Ctrl Pts',(1.05043926306477,-5.18201718059,386.073493919079));
#39904=CARTESIAN_POINT('Ctrl Pts',(-1.54826871412865,-5.0556491862241,385.994366043619));
#39905=CARTESIAN_POINT('Ctrl Pts',(-3.772089388456,-3.70514053050835,385.91523816816));
#39906=CARTESIAN_POINT('Ctrl Pts',(-4.89110742269369,-1.78586579845603,
385.84767053874));
#39907=CARTESIAN_POINT('Ctrl Pts',(-5.07305009743672,-0.472352615975399,
385.806478867808));
#39908=CARTESIAN_POINT('Ctrl Pts',(-5.07320349191978,4.6730170415385E-5,
385.791663155363));
#39909=CARTESIAN_POINT('Origin',(0.,0.,402.208336844637));
#39910=CARTESIAN_POINT('',(-5.07346461004462,-0.000124534794222197,387.791663155363));
#39911=CARTESIAN_POINT('',(-5.07325209134275,-7.62409538748165E-5,387.708336844637));
#39912=CARTESIAN_POINT('',(-5.0736,-1.59740085886799E-13,402.208336844637));
#39913=CARTESIAN_POINT('Ctrl Pts',(-5.07325209134275,-7.62409538748038E-5,
387.708336844637));
#39914=CARTESIAN_POINT('Ctrl Pts',(-5.0729792152731,0.508760470280088,387.692377920946));
#39915=CARTESIAN_POINT('Ctrl Pts',(-4.87111972002504,1.85878392032608,387.650043038769));
#39916=CARTESIAN_POINT('Ctrl Pts',(-3.69137763771595,3.78555886279474,387.581332198105));
#39917=CARTESIAN_POINT('Ctrl Pts',(-1.43897337649567,5.08783651365194,387.502204322645));
#39918=CARTESIAN_POINT('Ctrl Pts',(1.16185415459233,5.15817988164137,387.423076447186));
#39919=CARTESIAN_POINT('Ctrl Pts',(3.48135818778607,3.97955649994419,387.343948571725));
#39920=CARTESIAN_POINT('Ctrl Pts',(4.95790972221771,1.83735025355874,387.264820696266));
#39921=CARTESIAN_POINT('Ctrl Pts',(5.23398656730458,-0.749739542233496,
387.185692820806));
#39922=CARTESIAN_POINT('Ctrl Pts',(4.24274134513742,-3.15529248187465,387.106564945346));
#39923=CARTESIAN_POINT('Ctrl Pts',(2.22418746193322,-4.79684426494046,387.027437069886));
#39924=CARTESIAN_POINT('Ctrl Pts',(-0.332916112977428,-5.27692065788687,
386.948309194427));
#39925=CARTESIAN_POINT('Ctrl Pts',(-2.80940963451955,-4.47927921359921,
386.869181318967));
#39926=CARTESIAN_POINT('Ctrl Pts',(-4.6056517301173,-2.59705543044056,386.790053443507));
#39927=CARTESIAN_POINT('Ctrl Pts',(-5.06711936969965,-0.895633636916161,
386.73643861873));
#39928=CARTESIAN_POINT('Ctrl Pts',(-5.07403060973901,-0.0275296106999626,
386.70919975244));
#39929=CARTESIAN_POINT('Ctrl Pts',(-5.07402204930561,-2.85592496232024E-5,
386.708336844637));
#39930=CARTESIAN_POINT('Ctrl Pts',(-5.07346461004462,-0.000124534794222232,
387.791663155363));
#39931=CARTESIAN_POINT('Ctrl Pts',(-5.07290587442459,0.600116546096426,
387.77283520482));
#39932=CARTESIAN_POINT('Ctrl Pts',(-4.81706146775411,2.04169530250574,387.727631295791));
#39933=CARTESIAN_POINT('Ctrl Pts',(-3.48135818389009,3.97955649548785,387.656051428275));
#39934=CARTESIAN_POINT('Ctrl Pts',(-1.16185415329344,5.15817987586638,387.576923552815));
#39935=CARTESIAN_POINT('Ctrl Pts',(1.43897337488296,5.0878365079566,387.497795677355));
#39936=CARTESIAN_POINT('Ctrl Pts',(3.69137763358211,3.7855588585581,387.418667801895));
#39937=CARTESIAN_POINT('Ctrl Pts',(5.04997670698908,1.56667161976776,387.339539926436));
#39938=CARTESIAN_POINT('Ctrl Pts',(5.1858086147589,-1.03155887685117,387.260412050976));
#39939=CARTESIAN_POINT('Ctrl Pts',(4.06598393848355,-3.38001469187811,387.181284175516));
#39940=CARTESIAN_POINT('Ctrl Pts',(1.96164944276588,-4.91005663602919,387.102156300056));
#39941=CARTESIAN_POINT('Ctrl Pts',(-0.617665566383616,-5.25121071310437,
387.023028424596));
#39942=CARTESIAN_POINT('Ctrl Pts',(-3.04742321760052,-4.32087218488899,
386.943900549136));
#39943=CARTESIAN_POINT('Ctrl Pts',(-4.69640454618417,-2.39441853297418,
386.866778792725));
#39944=CARTESIAN_POINT('Ctrl Pts',(-5.07348026057684,-0.776631949401611,
386.816032994801));
#39945=CARTESIAN_POINT('Ctrl Pts',(-5.07396871057133,6.36451556408537E-5,
386.791663155363));
#39946=CARTESIAN_POINT('Origin',(0.,0.,402.208336844637));
#39947=CARTESIAN_POINT('',(-5.07332308908166,0.000100751512192854,388.791663155363));
#39948=CARTESIAN_POINT('',(-5.07357378438926,0.00012964408007953,388.708336844637));
#39949=CARTESIAN_POINT('',(-5.0736,-1.59740085886799E-13,402.208336844637));
#39950=CARTESIAN_POINT('Ctrl Pts',(-5.07357378438926,0.000129644080079632,
388.708336844637));
#39951=CARTESIAN_POINT('Ctrl Pts',(-5.07377922823885,0.204303981988881,
388.701932047939));
#39952=CARTESIAN_POINT('Ctrl Pts',(-5.01188528533374,1.24917654214382,388.669151292754));
#39953=CARTESIAN_POINT('Ctrl Pts',(-4.30974451485365,3.06314005305047,388.609994579082));
#39954=CARTESIAN_POINT('Ctrl Pts',(-2.32703038342756,4.74780521530929,388.530866703622));
#39955=CARTESIAN_POINT('Ctrl Pts',(0.2191351283499,5.28286897087523,388.451738828163));
#39956=CARTESIAN_POINT('Ctrl Pts',(2.71224074394742,4.53877460497707,388.372610952702));
#39957=CARTESIAN_POINT('Ctrl Pts',(4.54862275081774,2.69569208899244,388.293483077243));
#39958=CARTESIAN_POINT('Ctrl Pts',(5.28363204425109,0.199892943537846,388.214355201783));
#39959=CARTESIAN_POINT('Ctrl Pts',(4.73929845080001,-2.34430692575821,388.135227326323));
#39960=CARTESIAN_POINT('Ctrl Pts',(3.04742322101362,-4.32087218972514,388.056099450863));
#39961=CARTESIAN_POINT('Ctrl Pts',(0.617665567076949,-5.25121071898288,
387.976971575404));
#39962=CARTESIAN_POINT('Ctrl Pts',(-1.96164944496022,-4.9100566415267,387.897843699944));
#39963=CARTESIAN_POINT('Ctrl Pts',(-4.06598394303424,-3.38001469566346,
387.818715824484));
#39964=CARTESIAN_POINT('Ctrl Pts',(-4.95995652391698,-1.50520772763894,
387.755546872715));
#39965=CARTESIAN_POINT('Ctrl Pts',(-5.07343020858722,-0.332214537305361,
387.718753879433));
#39966=CARTESIAN_POINT('Ctrl Pts',(-5.07325209134275,-7.62409538748038E-5,
387.708336844637));
#39967=CARTESIAN_POINT('Ctrl Pts',(-5.07332308908166,0.000100751512193097,
388.791663155363));
#39968=CARTESIAN_POINT('Ctrl Pts',(-5.07353661258784,0.295776873009828,
388.782389331812));
#39969=CARTESIAN_POINT('Ctrl Pts',(-4.97579423080698,1.43225469143156,388.746739549775));
#39970=CARTESIAN_POINT('Ctrl Pts',(-4.13787031577727,3.29161874388992,388.684713809251));
#39971=CARTESIAN_POINT('Ctrl Pts',(-2.0669927453671,4.86664830205737,388.605585933792));
#39972=CARTESIAN_POINT('Ctrl Pts',(0.504372452470541,5.2633005932121,388.526458058332));
#39973=CARTESIAN_POINT('Ctrl Pts',(2.95361231985281,4.38553291736953,388.447330182872));
#39974=CARTESIAN_POINT('Ctrl Pts',(4.68768449948338,2.44588199605403,388.368202307412));
#39975=CARTESIAN_POINT('Ctrl Pts',(5.28671249546426,-0.0859982303311033,
388.289074431953));
#39976=CARTESIAN_POINT('Ctrl Pts',(4.60565172496217,-2.59705542753155,388.209946556493));
#39977=CARTESIAN_POINT('Ctrl Pts',(2.80940963137597,-4.47927920858367,388.130818681033));
#39978=CARTESIAN_POINT('Ctrl Pts',(0.332916112606594,-5.27692065197923,
388.051690805573));
#39979=CARTESIAN_POINT('Ctrl Pts',(-2.22418745944155,-4.79684425957118,
387.972562930114));
#39980=CARTESIAN_POINT('Ctrl Pts',(-4.24274134038657,-3.15529247834378,
387.893435054654));
#39981=CARTESIAN_POINT('Ctrl Pts',(-4.99812636818859,-1.3221248286521,387.833135129737));
#39982=CARTESIAN_POINT('Ctrl Pts',(-5.07368860366989,-0.240757440453781,
387.799211163307));
#39983=CARTESIAN_POINT('Ctrl Pts',(-5.07346461004462,-0.000124534794222232,
387.791663155363));
#39984=CARTESIAN_POINT('Origin',(0.,0.,402.208336844637));
#39985=CARTESIAN_POINT('',(-5.07403406771079,-9.36144982375056E-6,389.791663155363));
#39986=CARTESIAN_POINT('',(-5.07388549569213,-9.2912700738374E-5,389.708336844637));
#39987=CARTESIAN_POINT('',(-5.0736,-1.59740085886799E-13,402.208336844637));
#39988=CARTESIAN_POINT('Ctrl Pts',(-5.07388549569213,-9.2912700738277E-5,
389.708336844637));
#39989=CARTESIAN_POINT('Ctrl Pts',(-5.07325856807114,0.740202389523463,
389.685110216444));
#39990=CARTESIAN_POINT('Ctrl Pts',(-4.72308495981242,2.32174429013103,389.635507629765));
#39991=CARTESIAN_POINT('Ctrl Pts',(-3.13981907081257,4.25420509266713,389.559529084599));
#39992=CARTESIAN_POINT('Ctrl Pts',(-0.730671872756092,5.23668247865729,
389.48040120914));
#39993=CARTESIAN_POINT('Ctrl Pts',(1.85539526507438,4.95118502767294,389.401273333679));
#39994=CARTESIAN_POINT('Ctrl Pts',(3.99220955659535,3.46684115934693,389.32214545822));
#39995=CARTESIAN_POINT('Ctrl Pts',(5.16237725796638,1.14305984722794,389.24301758276));
#39996=CARTESIAN_POINT('Ctrl Pts',(5.08256188536855,-1.45749423645932,389.1638897073));
#39997=CARTESIAN_POINT('Ctrl Pts',(3.77208939268016,-3.70514053465492,389.08476183184));
#39998=CARTESIAN_POINT('Ctrl Pts',(1.54826871586373,-5.05564919188336,389.005633956381));
#39999=CARTESIAN_POINT('Ctrl Pts',(-1.05043926423896,-5.18201718639165,
388.926506080921));
#40000=CARTESIAN_POINT('Ctrl Pts',(-3.39480099358967,-4.05364662764723,
388.847378205461));
#40001=CARTESIAN_POINT('Ctrl Pts',(-4.79394457591898,-2.1145332421108,388.7746551267));
#40002=CARTESIAN_POINT('Ctrl Pts',(-5.07293317820744,-0.636518001009154,
388.728308006425));
#40003=CARTESIAN_POINT('Ctrl Pts',(-5.07357378438926,0.000129644080079632,
388.708336844637));
#40004=CARTESIAN_POINT('Ctrl Pts',(-5.07403406771079,-9.36144982382212E-6,
389.791663155363));
#40005=CARTESIAN_POINT('Ctrl Pts',(-5.07394412729799,0.831658855747162,
389.765567500318));
#40006=CARTESIAN_POINT('Ctrl Pts',(-4.65432422371577,2.50401601420859,389.713095886787));
#40007=CARTESIAN_POINT('Ctrl Pts',(-2.90527399360582,4.41770389765948,389.634248314769));
#40008=CARTESIAN_POINT('Ctrl Pts',(-0.446542510013585,5.2685220405792,389.55512043931));
#40009=CARTESIAN_POINT('Ctrl Pts',(2.12031175334316,4.84365593059135,389.475992563849));
#40010=CARTESIAN_POINT('Ctrl Pts',(4.17376808571255,3.24597977073262,389.39686468839));
#40011=CARTESIAN_POINT('Ctrl Pts',(5.21661647505316,0.862344048232485,389.31773681293));
#40012=CARTESIAN_POINT('Ctrl Pts',(4.99634867366186,-1.73009382303836,389.23860893747));
#40013=CARTESIAN_POINT('Ctrl Pts',(3.56629883549932,-3.90361849073832,389.15948106201));
#40014=CARTESIAN_POINT('Ctrl Pts',(1.27272954528402,-5.13194740911081,389.08035318655));
#40015=CARTESIAN_POINT('Ctrl Pts',(-1.3290098591728,-5.11766133107102,389.001225311091));
#40016=CARTESIAN_POINT('Ctrl Pts',(-3.60895181526604,-3.86421939082217,
388.922097435631));
#40017=CARTESIAN_POINT('Ctrl Pts',(-4.85025165556801,-1.93168481258741,
388.852243383721));
#40018=CARTESIAN_POINT('Ctrl Pts',(-5.07292932400786,-0.545164413360684,
388.808765290299));
#40019=CARTESIAN_POINT('Ctrl Pts',(-5.07332308908166,0.000100751512193097,
388.791663155363));
#40020=CARTESIAN_POINT('Origin',(0.,0.,402.208336844637));
#40021=CARTESIAN_POINT('',(-5.0732856633921,-8.9472558095216E-5,390.791663155363));
#40022=CARTESIAN_POINT('',(-5.07317963304504,-1.41915822972106E-5,390.708336844637));
#40023=CARTESIAN_POINT('',(-5.0736,-1.59740085886799E-13,402.208336844637));
#40024=CARTESIAN_POINT('Ctrl Pts',(-5.07317963304504,-1.41915822972002E-5,
390.708336844637));
#40025=CARTESIAN_POINT('Ctrl Pts',(-5.07313689101218,0.435939705489138,
390.694664343437));
#40026=CARTESIAN_POINT('Ctrl Pts',(-4.9102234101679,1.71293434968472,390.65461588375));
#40027=CARTESIAN_POINT('Ctrl Pts',(-3.85104960630393,3.62300175237324,390.588191465576));
#40028=CARTESIAN_POINT('Ctrl Pts',(-1.65684512829777,5.02111431743484,390.509063590116));
#40029=CARTESIAN_POINT('Ctrl Pts',(0.938536610313288,5.20344826043412,390.429935714657));
#40030=CARTESIAN_POINT('Ctrl Pts',(3.30666744908329,4.12585447502528,390.350807839197));
#40031=CARTESIAN_POINT('Ctrl Pts',(4.874144221702,2.04925422384882,390.271679963737));
#40032=CARTESIAN_POINT('Ctrl Pts',(5.26142871608132,-0.523538569265068,
390.192552088277));
#40033=CARTESIAN_POINT('Ctrl Pts',(4.37474648711696,-2.96956527817979,390.113424212818));
#40034=CARTESIAN_POINT('Ctrl Pts',(2.42879276586438,-4.69656155803349,390.034296337358));
#40035=CARTESIAN_POINT('Ctrl Pts',(-0.105252389973582,-5.28636422338813,
389.955168461898));
#40036=CARTESIAN_POINT('Ctrl Pts',(-2.61381244478399,-4.59616245050211,
389.876040586438));
#40037=CARTESIAN_POINT('Ctrl Pts',(-4.48948165275299,-2.79307702319636,
389.796912710979));
#40038=CARTESIAN_POINT('Ctrl Pts',(-5.04661334373894,-1.04147487532298,
389.741011463711));
#40039=CARTESIAN_POINT('Ctrl Pts',(-5.07397050166598,-0.10047056555588,
389.711486174931));
#40040=CARTESIAN_POINT('Ctrl Pts',(-5.07388549569213,-9.2912700738277E-5,
389.708336844637));
#40041=CARTESIAN_POINT('Ctrl Pts',(-5.0732856633921,-8.94725580950079E-5,
390.791663155363));
#40042=CARTESIAN_POINT('Ctrl Pts',(-5.07295082938292,0.527313084285289,
390.77512162731));
#40043=CARTESIAN_POINT('Ctrl Pts',(-4.86059546998445,1.89593815106623,390.732204140772));
#40044=CARTESIAN_POINT('Ctrl Pts',(-3.64958350306562,3.82586787010077,390.662910695746));
#40045=CARTESIAN_POINT('Ctrl Pts',(-1.38301395488213,5.10333196117197,390.583782820286));
#40046=CARTESIAN_POINT('Ctrl Pts',(1.21842922772966,5.14510980663504,390.504654944826));
#40047=CARTESIAN_POINT('Ctrl Pts',(3.52485020731651,3.94108560187402,390.425527069367));
#40048=CARTESIAN_POINT('Ctrl Pts',(4.97778782502355,1.78279361519087,390.346399193907));
#40049=CARTESIAN_POINT('Ctrl Pts',(5.2254376041702,-0.807171945896316,390.267271318447));
#40050=CARTESIAN_POINT('Ctrl Pts',(4.2078353041098,-3.20169435749343,390.188143442988));
#40051=CARTESIAN_POINT('Ctrl Pts',(2.17137625543244,-4.82098017654731,390.109015567527));
#40052=CARTESIAN_POINT('Ctrl Pts',(-0.390845137002325,-5.27294649927341,
390.029887692068));
#40053=CARTESIAN_POINT('Ctrl Pts',(-2.85842993443779,-4.44815726062243,
389.950759816608));
#40054=CARTESIAN_POINT('Ctrl Pts',(-4.63389386243089,-2.54632134206259,
389.871631941148));
#40055=CARTESIAN_POINT('Ctrl Pts',(-5.07183812704173,-0.858476903537314,
389.818599720733));
#40056=CARTESIAN_POINT('Ctrl Pts',(-5.07403503379527,-0.00894262882346251,
389.791943458805));
#40057=CARTESIAN_POINT('Ctrl Pts',(-5.07403406771079,-9.36144982382212E-6,
389.791663155363));
#40058=CARTESIAN_POINT('Origin',(0.,0.,402.208336844637));
#40059=CARTESIAN_POINT('',(-5.07351709598447,0.000128180283586465,391.791663155363));
#40060=CARTESIAN_POINT('',(-5.07379939980891,0.000111618004047815,391.708336844637));
#40061=CARTESIAN_POINT('',(-5.0736,-1.59740085886799E-13,402.208336844637));
#40062=CARTESIAN_POINT('Ctrl Pts',(-5.07379939980891,0.000111618004048301,
391.708336844637));
#40063=CARTESIAN_POINT('Ctrl Pts',(-5.07392549945089,0.131381756589591,
391.704218470429));
#40064=CARTESIAN_POINT('Ctrl Pts',(-5.03695972030326,1.10329526429473,391.673724137734));
#40065=CARTESIAN_POINT('Ctrl Pts',(-4.43771707875037,2.8746116080056,391.616853846554));
#40066=CARTESIAN_POINT('Ctrl Pts',(-2.52942735664669,4.64313708771996,391.537725971094));
#40067=CARTESIAN_POINT('Ctrl Pts',(-0.00867922155838994,5.28740479243137,
391.458598095634));
#40068=CARTESIAN_POINT('Ctrl Pts',(2.51417044146968,4.65141610255989,391.379470220174));
#40069=CARTESIAN_POINT('Ctrl Pts',(4.42825589764708,2.88916501309064,391.300342344714));
#40070=CARTESIAN_POINT('Ctrl Pts',(5.27011345519119,0.427351070346123,391.221214469255));
#40071=CARTESIAN_POINT('Ctrl Pts',(4.8359014254693,-2.1379387669101,391.142086593795));
#40072=CARTESIAN_POINT('Ctrl Pts',(3.23075696923981,-4.18556258746916,391.062958718335));
#40073=CARTESIAN_POINT('Ctrl Pts',(0.843338896446427,-5.21972262420654,
390.983830842875));
#40074=CARTESIAN_POINT('Ctrl Pts',(-1.7482795463511,-4.99001436828829,390.904702967415));
#40075=CARTESIAN_POINT('Ctrl Pts',(-3.91658141767327,-3.55205782141137,
390.825575091956));
#40076=CARTESIAN_POINT('Ctrl Pts',(-4.92575069087544,-1.65110613686035,
390.760119717696));
#40077=CARTESIAN_POINT('Ctrl Pts',(-5.07321934571947,-0.405069684288436,
390.721040301923));
#40078=CARTESIAN_POINT('Ctrl Pts',(-5.07317963304504,-1.41915822972002E-5,
390.708336844637));
#40079=CARTESIAN_POINT('Ctrl Pts',(-5.07351709598447,0.0001281802835865,
391.791663155363));
#40080=CARTESIAN_POINT('Ctrl Pts',(-5.07373426530186,0.222882138466162,
391.784675754303));
#40081=CARTESIAN_POINT('Ctrl Pts',(-5.00497588579108,1.28635201118677,391.751312394756));
#40082=CARTESIAN_POINT('Ctrl Pts',(-4.27584641576499,3.1102832884012,391.691573076723));
#40083=CARTESIAN_POINT('Ctrl Pts',(-2.27475150326393,4.77307346514974,391.612445201264));
#40084=CARTESIAN_POINT('Ctrl Pts',(0.277136335534271,5.28014395228432,391.533317325804));
#40085=CARTESIAN_POINT('Ctrl Pts',(2.76192025858026,4.50871613550486,391.454189450344));
#40086=CARTESIAN_POINT('Ctrl Pts',(4.57795151161372,2.64557832290629,391.375061574885));
#40087=CARTESIAN_POINT('Ctrl Pts',(5.28550858366077,0.141858088829558,391.295933699424));
#40088=CARTESIAN_POINT('Ctrl Pts',(4.71326839627705,-2.39621070233275,391.216805823965));
#40089=CARTESIAN_POINT('Ctrl Pts',(2.99978931370662,-4.35407725915487,391.137677948505));
#40090=CARTESIAN_POINT('Ctrl Pts',(0.559961558764467,-5.2576770305929,391.058550073045));
#40091=CARTESIAN_POINT('Ctrl Pts',(-2.01545149642842,-4.88821848640817,
390.979422197585));
#40092=CARTESIAN_POINT('Ctrl Pts',(-4.10285677321784,-3.33515981682715,
390.900294322126));
#40093=CARTESIAN_POINT('Ctrl Pts',(-4.96813235745424,-1.46802940120253,
390.837707974718));
#40094=CARTESIAN_POINT('Ctrl Pts',(-5.07348473216978,-0.313645979534272,
390.801497585797));
#40095=CARTESIAN_POINT('Ctrl Pts',(-5.0732856633921,-8.94725580950079E-5,
390.791663155363));
#40096=CARTESIAN_POINT('Origin',(0.,0.,402.208336844637));
#40097=CARTESIAN_POINT('',(-5.07393095917883,-7.88724074329838E-5,392.791663155363));
#40098=CARTESIAN_POINT('',(-5.07367047787857,-0.000126645267990005,392.708336844637));
#40099=CARTESIAN_POINT('',(-5.0736,-1.59740085886799E-13,402.208336844637));
#40100=CARTESIAN_POINT('Ctrl Pts',(-5.07367047787857,-0.000126645267989993,
392.708336844637));
#40101=CARTESIAN_POINT('Ctrl Pts',(-5.07298837013062,0.667375891727513,
392.687396638935));
#40102=CARTESIAN_POINT('Ctrl Pts',(-4.77363543308555,2.17624796267435,392.640080474746));
#40103=CARTESIAN_POINT('Ctrl Pts',(-3.32019468996614,4.11497654776232,392.566388352071));
#40104=CARTESIAN_POINT('Ctrl Pts',(-0.955614322062658,5.20033903081154,
392.487260476611));
#40105=CARTESIAN_POINT('Ctrl Pts',(1.64035202716895,5.02652663326038,392.408132601151));
#40106=CARTESIAN_POINT('Ctrl Pts',(3.83913464362559,3.63562511214056,392.329004725691));
#40107=CARTESIAN_POINT('Ctrl Pts',(5.10833519286426,1.36441794376124,392.249876850232));
#40108=CARTESIAN_POINT('Ctrl Pts',(5.14063804785052,-1.23716014683014,392.170748974772));
#40109=CARTESIAN_POINT('Ctrl Pts',(3.92822161400576,-3.53918065647562,392.091621099312));
#40110=CARTESIAN_POINT('Ctrl Pts',(1.76465219715718,-4.98424792631562,392.012493223852));
#40111=CARTESIAN_POINT('Ctrl Pts',(-0.826198153971171,-5.22246315241074,
391.933365348392));
#40112=CARTESIAN_POINT('Ctrl Pts',(-3.21699847841567,-4.19614651290735,
391.854237472933));
#40113=CARTESIAN_POINT('Ctrl Pts',(-4.74496408021847,-2.26010134957161,
391.779227971681));
#40114=CARTESIAN_POINT('Ctrl Pts',(-5.07311789947229,-0.7093324551461,391.730594428916));
#40115=CARTESIAN_POINT('Ctrl Pts',(-5.07379939980891,0.000111618004048301,
391.708336844637));
#40116=CARTESIAN_POINT('Ctrl Pts',(-5.07393095917883,-7.88724074328884E-5,
392.791663155363));
#40117=CARTESIAN_POINT('Ctrl Pts',(-5.07336361274665,0.758765898971362,
392.767853922809));
#40118=CARTESIAN_POINT('Ctrl Pts',(-4.7096061531202,2.35878746105711,392.717668731768));
#40119=CARTESIAN_POINT('Ctrl Pts',(-3.09291170420029,4.28842883762094,392.64110758224));
#40120=CARTESIAN_POINT('Ctrl Pts',(-0.67312059357683,5.24439065781915,392.561979706781));
#40121=CARTESIAN_POINT('Ctrl Pts',(1.90965537976903,4.9305112347339,392.482851831321));
#40122=CARTESIAN_POINT('Ctrl Pts',(4.03004033003705,3.4227912065437,392.403723955861));
#40123=CARTESIAN_POINT('Ctrl Pts',(5.17461860283211,1.0862996918631,392.324596080401));
#40124=CARTESIAN_POINT('Ctrl Pts',(5.06624976530063,-1.51322107469774,392.245468204942));
#40125=CARTESIAN_POINT('Ctrl Pts',(3.73117351397988,-3.74634073649114,392.166340329482));
#40126=CARTESIAN_POINT('Ctrl Pts',(1.49265617235166,-5.07234681941786,392.087212454022));
#40127=CARTESIAN_POINT('Ctrl Pts',(-1.10728282783815,-5.1701691891555,392.008084578562));
#40128=CARTESIAN_POINT('Ctrl Pts',(-3.43911186168285,-4.01612179946654,
391.928956703103));
#40129=CARTESIAN_POINT('Ctrl Pts',(-4.80583883513493,-2.07741741105628,
391.856816228703));
#40130=CARTESIAN_POINT('Ctrl Pts',(-5.07291449714329,-0.617966855796078,
391.811051712789));
#40131=CARTESIAN_POINT('Ctrl Pts',(-5.07351709598447,0.0001281802835865,
391.791663155363));
#40132=CARTESIAN_POINT('Origin',(0.,0.,402.208336844637));
#40133=CARTESIAN_POINT('',(-5.07318860167667,-3.10232113821807E-5,393.791663155363));
#40134=CARTESIAN_POINT('',(-5.07320934784751,5.14726455261062E-5,393.708336844637));
#40135=CARTESIAN_POINT('',(-5.0736,-1.59740085886799E-13,402.208336844637));
#40136=CARTESIAN_POINT('Ctrl Pts',(-5.07320934784751,5.14726455259906E-5,
393.708336844637));
#40137=CARTESIAN_POINT('Ctrl Pts',(-5.07333938414724,0.363095667172288,
393.696950765927));
#40138=CARTESIAN_POINT('Ctrl Pts',(-4.94587345760415,1.56704518273248,393.659188728731));
#40139=CARTESIAN_POINT('Ctrl Pts',(-4.00356958154437,3.45371616865744,393.595050733048));
#40140=CARTESIAN_POINT('Ctrl Pts',(-1.8716398630404,4.94506713715712,393.515922857588));
#40141=CARTESIAN_POINT('Ctrl Pts',(0.713476058729831,5.23905303289941,393.436794982128));
#40142=CARTESIAN_POINT('Ctrl Pts',(3.12583571869877,4.26449010171441,393.357667106669));
#40143=CARTESIAN_POINT('Ctrl Pts',(4.78132668327137,2.25735241283907,393.278539231209));
#40144=CARTESIAN_POINT('Ctrl Pts',(5.2790995798779,-0.296365304389928,393.199411355749));
#40145=CARTESIAN_POINT('Ctrl Pts',(4.49862704983328,-2.77832313355043,393.120283480289));
#40146=CARTESIAN_POINT('Ctrl Pts',(2.62888742685924,-4.58755661161959,393.041155604829));
#40147=CARTESIAN_POINT('Ctrl Pts',(0.122606802959192,-5.28599019482455,
392.96202772937));
#40148=CARTESIAN_POINT('Ctrl Pts',(-2.41336100201929,-4.70450990453263,
392.88289985391));
#40149=CARTESIAN_POINT('Ctrl Pts',(-4.3649739152189,-2.98391144093985,392.80377197845));
#40150=CARTESIAN_POINT('Ctrl Pts',(-5.02290836650147,-1.18734550240995,
392.745584308693));
#40151=CARTESIAN_POINT('Ctrl Pts',(-5.07384754247588,-0.173399956222615,
392.713772597422));
#40152=CARTESIAN_POINT('Ctrl Pts',(-5.07367047787857,-0.000126645267989993,
392.708336844637));
#40153=CARTESIAN_POINT('Ctrl Pts',(-5.07318860167666,-3.10232113822501E-5,
393.791663155363));
#40154=CARTESIAN_POINT('Ctrl Pts',(-5.07309097404724,0.454497176795154,
393.777408049801));
#40155=CARTESIAN_POINT('Ctrl Pts',(-4.90058989979703,1.75010317897161,393.736776985753));
#40156=CARTESIAN_POINT('Ctrl Pts',(-3.81103098253419,3.66507401773587,393.669769963218));
#40157=CARTESIAN_POINT('Ctrl Pts',(-1.60160528615343,5.03900637156607,393.590642087758));
#40158=CARTESIAN_POINT('Ctrl Pts',(0.995622269493122,5.19282784249655,393.511514212298));
#40159=CARTESIAN_POINT('Ctrl Pts',(3.3517765903209,4.08929314110579,393.432386336838));
#40160=CARTESIAN_POINT('Ctrl Pts',(4.89635442297923,1.99560468778007,393.353258461378));
#40161=CARTESIAN_POINT('Ctrl Pts',(5.2553621496497,-0.581285972088894,393.274130585919));
#40162=CARTESIAN_POINT('Ctrl Pts',(4.34187207029457,-3.01742798265574,393.195002710459));
#40163=CARTESIAN_POINT('Ctrl Pts',(2.37707048734272,-4.72295041298575,393.115874834999));
#40164=CARTESIAN_POINT('Ctrl Pts',(-0.163298847893048,-5.28488961016167,
393.03674695954));
#40165=CARTESIAN_POINT('Ctrl Pts',(-2.66412810582239,-4.56718142195876,
392.957619084079));
#40166=CARTESIAN_POINT('Ctrl Pts',(-4.51988342344183,-2.74360684935247,
392.87849120862));
#40167=CARTESIAN_POINT('Ctrl Pts',(-5.05214048257081,-1.00431002992741,
392.823172565714));
#40168=CARTESIAN_POINT('Ctrl Pts',(-5.07399212128462,-0.0818852283646697,
392.794229881295));
#40169=CARTESIAN_POINT('Ctrl Pts',(-5.07393095917883,-7.88724074328884E-5,
392.791663155363));
#40170=CARTESIAN_POINT('Origin',(0.,0.,402.208336844637));
#40171=CARTESIAN_POINT('',(-5.07374340439062,0.000119799015104727,394.791663155363));
#40172=CARTESIAN_POINT('',(-5.07397904538501,5.86126803115486E-5,394.708336844637));
#40173=CARTESIAN_POINT('',(-5.0736,-1.59740085886799E-13,402.208336844637));
#40174=CARTESIAN_POINT('Ctrl Pts',(-5.07397904538501,5.86126803111056E-5,
394.708336844637));
#40175=CARTESIAN_POINT('Ctrl Pts',(-5.07401332726156,0.0584447346541764,
394.706504892919));
#40176=CARTESIAN_POINT('Ctrl Pts',(-5.05881623778616,0.957440994697868,
394.678296982715));
#40177=CARTESIAN_POINT('Ctrl Pts',(-4.55744811727866,2.68074456564335,394.623713114025));
#40178=CARTESIAN_POINT('Ctrl Pts',(-2.72712679296628,4.52984593810856,394.544585238565));
#40179=CARTESIAN_POINT('Ctrl Pts',(-0.236477452813074,5.28212108742541,
394.465457363106));
#40180=CARTESIAN_POINT('Ctrl Pts',(2.31143093653793,4.75541920271268,394.386329487645));
#40181=CARTESIAN_POINT('Ctrl Pts',(4.29966508998112,3.07727231195273,394.307201612186));
#40182=CARTESIAN_POINT('Ctrl Pts',(5.2468074522505,0.654015540275394,394.228073736726));
#40183=CARTESIAN_POINT('Ctrl Pts',(4.92352338499734,-1.92760012588128,394.148945861266));
#40184=CARTESIAN_POINT('Ctrl Pts',(3.40809070325859,-4.04247974964323,394.069817985806));
#40185=CARTESIAN_POINT('Ctrl Pts',(1.06744601535546,-5.17854069909805,393.990690110347));
#40186=CARTESIAN_POINT('Ctrl Pts',(-1.53166282285958,-5.06070486839363,
393.911562234887));
#40187=CARTESIAN_POINT('Ctrl Pts',(-3.75990519627929,-3.71750422769163,
393.832434359427));
#40188=CARTESIAN_POINT('Ctrl Pts',(-4.88811881465991,-1.79697577151505,
393.764692562677));
#40189=CARTESIAN_POINT('Ctrl Pts',(-5.07303815383513,-0.477899626088436,
393.723326724414));
#40190=CARTESIAN_POINT('Ctrl Pts',(-5.07320934784751,5.14726455259906E-5,
393.708336844637));
#40191=CARTESIAN_POINT('Ctrl Pts',(-5.07374340439062,0.000119799015104727,
394.791663155363));
#40192=CARTESIAN_POINT('Ctrl Pts',(-5.07389328700639,0.149964795759533,
394.786962176793));
#40193=CARTESIAN_POINT('Ctrl Pts',(-5.03087783588661,1.1404650386697,394.755885239737));
#40194=CARTESIAN_POINT('Ctrl Pts',(-4.40588160918252,2.92317155691987,394.698432344195));
#40195=CARTESIAN_POINT('Ctrl Pts',(-2.47828569661807,4.67063429431767,394.619304468735));
#40196=CARTESIAN_POINT('Ctrl Pts',(0.0493855336599835,5.28718126929493,
394.540176593275));
#40197=CARTESIAN_POINT('Ctrl Pts',(2.56509888521489,4.623525972068,394.461048717816));
#40198=CARTESIAN_POINT('Ctrl Pts',(4.45971656139522,2.84036140259214,394.381920842355));
#40199=CARTESIAN_POINT('Ctrl Pts',(5.27448866684743,0.369450955630144,394.302792966896));
#40200=CARTESIAN_POINT('Ctrl Pts',(4.81213180090847,-2.19091584411711,394.223665091436));
#40201=CARTESIAN_POINT('Ctrl Pts',(3.18459792440514,-4.2207891164085,394.144537215977));
#40202=CARTESIAN_POINT('Ctrl Pts',(0.785967069903959,-5.22866909168525,
394.065409340517));
#40203=CARTESIAN_POINT('Ctrl Pts',(-1.8029725289961,-4.97051453724898,393.986281465057));
#40204=CARTESIAN_POINT('Ctrl Pts',(-3.95535256793798,-3.50883324890547,
393.907153589597));
#40205=CARTESIAN_POINT('Ctrl Pts',(-4.9347894212868,-1.61393147469998,393.842280819699));
#40206=CARTESIAN_POINT('Ctrl Pts',(-5.0732716126465,-0.386507955183392,
393.803784008288));
#40207=CARTESIAN_POINT('Ctrl Pts',(-5.07318860167666,-3.10232113822501E-5,
393.791663155363));
#40208=CARTESIAN_POINT('Origin',(0.,0.,402.208336844637));
#40209=CARTESIAN_POINT('',(-5.07372845053928,-0.000121538385184292,395.791663155363));
#40210=CARTESIAN_POINT('',(-5.07344883766069,-0.000122970527678777,395.708336844637));
#40211=CARTESIAN_POINT('',(-5.0736,-1.59740085886799E-13,402.208336844637));
#40212=CARTESIAN_POINT('Ctrl Pts',(-5.07344883766069,-0.000122970527678921,
395.708336844637));
#40213=CARTESIAN_POINT('Ctrl Pts',(-5.07290495347366,0.594570911737787,
395.689683061425));
#40214=CARTESIAN_POINT('Ctrl Pts',(-4.82050381961586,2.03059585572183,395.644653319727));
#40215=CARTESIAN_POINT('Ctrl Pts',(-3.49440419526435,3.96810585645496,395.573247619542));
#40216=CARTESIAN_POINT('Ctrl Pts',(-1.17878204811896,5.1543377509575,395.494119744082));
#40217=CARTESIAN_POINT('Ctrl Pts',(1.42226240243777,5.09253320328156,395.414991868623));
#40218=CARTESIAN_POINT('Ctrl Pts',(3.67892986523249,3.79765714811298,395.335863993163));
#40219=CARTESIAN_POINT('Ctrl Pts',(5.0448061610774,1.58324210563915,395.256736117703));
#40220=CARTESIAN_POINT('Ctrl Pts',(5.18916725226161,-1.01452845991075,395.177608242243));
#40221=CARTESIAN_POINT('Ctrl Pts',(4.07705852165763,-3.36664797371096,395.098480366784));
#40222=CARTESIAN_POINT('Ctrl Pts',(1.97775844702931,-4.90359014326416,395.019352491324));
#40223=CARTESIAN_POINT('Ctrl Pts',(-0.60042266624658,-5.25321019851391,
394.940224615864));
#40224=CARTESIAN_POINT('Ctrl Pts',(-3.03322150067462,-4.33085350661488,
394.861096740404));
#40225=CARTESIAN_POINT('Ctrl Pts',(-4.69225666341608,-2.40548544911562,
394.783800816662));
#40226=CARTESIAN_POINT('Ctrl Pts',(-5.07351974582911,-0.782183276838963,
394.732880851406));
#40227=CARTESIAN_POINT('Ctrl Pts',(-5.07397904538501,5.86126803111056E-5,
394.708336844637));
#40228=CARTESIAN_POINT('Ctrl Pts',(-5.07372845053928,-0.000121538385184274,
395.791663155363));
#40229=CARTESIAN_POINT('Ctrl Pts',(-5.07303742094413,0.685929840247112,
395.770140345299));
#40230=CARTESIAN_POINT('Ctrl Pts',(-4.76110728643783,2.2133386185757,395.722241576749));
#40231=CARTESIAN_POINT('Ctrl Pts',(-3.27480540051438,4.15118950351341,395.647966849712));
#40232=CARTESIAN_POINT('Ctrl Pts',(-0.898448588333209,5.21051963238218,
395.568838974252));
#40233=CARTESIAN_POINT('Ctrl Pts',(1.69545248148909,5.00820981872071,395.489711098793));
#40234=CARTESIAN_POINT('Ctrl Pts',(3.87882816762124,3.59324599093717,395.410583223333));
#40235=CARTESIAN_POINT('Ctrl Pts',(5.12301066540628,1.30823790934658,395.331455347873));
#40236=CARTESIAN_POINT('Ctrl Pts',(5.12674204938754,-1.29353804132683,395.252327472413));
#40237=CARTESIAN_POINT('Ctrl Pts',(3.88911882751359,-3.58210544942458,395.173199596953));
#40238=CARTESIAN_POINT('Ctrl Pts',(1.70981070658587,-5.00332609900278,395.094071721494));
#40239=CARTESIAN_POINT('Ctrl Pts',(-0.883499401435098,-5.21307524528295,
395.014943846034));
#40240=CARTESIAN_POINT('Ctrl Pts',(-3.26288494670713,-4.16056565022955,
394.935815970574));
#40241=CARTESIAN_POINT('Ctrl Pts',(-4.7577955410693,-2.22302453301642,394.861389073684));
#40242=CARTESIAN_POINT('Ctrl Pts',(-5.07305233493801,-0.690776202139344,
394.81333813528));
#40243=CARTESIAN_POINT('Ctrl Pts',(-5.07374340439062,0.000119799015104727,
394.791663155363));
#40244=CARTESIAN_POINT('Origin',(0.,0.,402.208336844637));
#40245=CARTESIAN_POINT('',(-5.07319204280361,3.5344916511082E-5,396.791663155363));
#40246=CARTESIAN_POINT('',(-5.07333567377535,0.000103933621521292,396.708336844637));
#40247=CARTESIAN_POINT('',(-5.0736,-1.59740085886799E-13,402.208336844637));
#40248=CARTESIAN_POINT('Ctrl Pts',(-5.07333567377534,0.000103933621520939,
396.708336844637));
#40249=CARTESIAN_POINT('Ctrl Pts',(-5.07355255518605,0.290225038825201,
396.699237188418));
#40250=CARTESIAN_POINT('Ctrl Pts',(-4.9781337482961,1.42114034886055,396.663761573712));
#40251=CARTESIAN_POINT('Ctrl Pts',(-4.14865431030898,3.27801650109757,396.601910000519));
#40252=CARTESIAN_POINT('Ctrl Pts',(-2.08295867375766,4.85983620416686,396.52278212506));
#40253=CARTESIAN_POINT('Ctrl Pts',(0.487090472013812,5.26492807548086,396.4436542496));
#40254=CARTESIAN_POINT('Ctrl Pts',(2.93919882905869,4.3952059122609,396.36452637414));
#40255=CARTESIAN_POINT('Ctrl Pts',(4.67962948341671,2.46125835008237,396.28539849868));
#40256=CARTESIAN_POINT('Ctrl Pts',(5.2869663411736,-0.0686416434144708,
396.206270623221));
#40257=CARTESIAN_POINT('Ctrl Pts',(4.61415296796628,-2.58192121415839,396.127142747761));
#40258=CARTESIAN_POINT('Ctrl Pts',(2.82409983825713,-4.47003186470401,396.048014872301));
#40259=CARTESIAN_POINT('Ctrl Pts',(0.350238296140284,-5.27579926682488,
395.968886996841));
#40260=CARTESIAN_POINT('Ctrl Pts',(-2.20842757548492,-4.80412035775031,
395.889759121382));
#40261=CARTESIAN_POINT('Ctrl Pts',(-4.23235974759556,-3.16920427471092,
395.810631245921));
#40262=CARTESIAN_POINT('Ctrl Pts',(-4.99595812955649,-1.33323876922698,
395.750157153674));
#40263=CARTESIAN_POINT('Ctrl Pts',(-5.07367399139889,-0.246310585215766,
395.716059019912));
#40264=CARTESIAN_POINT('Ctrl Pts',(-5.07344883766069,-0.000122970527678921,
395.708336844637));
#40265=CARTESIAN_POINT('Ctrl Pts',(-5.07319204280361,3.53449165107697E-5,
396.791663155363));
#40266=CARTESIAN_POINT('Ctrl Pts',(-5.07328550820695,0.381659555984483,
396.779694472291));
#40267=CARTESIAN_POINT('Ctrl Pts',(-4.93711373649749,1.60422160810075,396.741349830733));
#40268=CARTESIAN_POINT('Ctrl Pts',(-3.96540078941456,3.49747355738801,396.676629230689));
#40269=CARTESIAN_POINT('Ctrl Pts',(-1.81722218927578,4.96532256959422,396.597501355229));
#40270=CARTESIAN_POINT('Ctrl Pts',(0.770966287074601,5.23090199578547,396.51837347977));
#40271=CARTESIAN_POINT('Ctrl Pts',(3.17247820700774,4.22990623198423,396.43924560431));
#40272=CARTESIAN_POINT('Ctrl Pts',(4.8058277352491,2.20470961453625,396.36011772885));
#40273=CARTESIAN_POINT('Ctrl Pts',(5.275526676699,-0.354320460537079,396.28098985339));
#40274=CARTESIAN_POINT('Ctrl Pts',(4.46784531008081,-2.82755777845599,396.201861977931));
#40275=CARTESIAN_POINT('Ctrl Pts',(2.57835013256881,-4.61614940174172,396.122734102471));
#40276=CARTESIAN_POINT('Ctrl Pts',(0.0645507123742531,-5.2870178655694,
396.043606227011));
#40277=CARTESIAN_POINT('Ctrl Pts',(-2.46487858023149,-4.67772362266456,
395.964478351551));
#40278=CARTESIAN_POINT('Ctrl Pts',(-4.39747886350376,-2.93579705537622,
395.885350476092));
#40279=CARTESIAN_POINT('Ctrl Pts',(-5.02925481295834,-1.15017365368594,
395.827745410695));
#40280=CARTESIAN_POINT('Ctrl Pts',(-5.0738842698389,-0.154818306903111,
395.796516303786));
#40281=CARTESIAN_POINT('Ctrl Pts',(-5.07372845053928,-0.000121538385184274,
395.791663155363));
#40282=CARTESIAN_POINT('Origin',(0.,0.,402.208336844637));
#40283=CARTESIAN_POINT('',(-5.0739418421154,7.48951186854696E-5,397.791663155363));
#40284=CARTESIAN_POINT('',(-5.07403169783887,-1.51513653288439E-5,397.708336844637));
#40285=CARTESIAN_POINT('',(-5.0736,-1.59740085886799E-13,402.208336844637));
#40286=CARTESIAN_POINT('Ctrl Pts',(-5.07403169783887,-1.51513653288493E-5,
397.708336844637));
#40287=CARTESIAN_POINT('Ctrl Pts',(-5.07388968734652,0.82610348406882,397.682415356923));
#40288=CARTESIAN_POINT('Ctrl Pts',(-4.6586701596041,2.49296234041498,397.630117910723));
#40289=CARTESIAN_POINT('Ctrl Pts',(-2.91976153402742,4.40814216562114,397.551444506037));
#40290=CARTESIAN_POINT('Ctrl Pts',(-0.463836508948714,5.26702766851281,
397.472316630577));
#40291=CARTESIAN_POINT('Ctrl Pts',(2.10439874769627,4.85059075563045,397.393188755117));
#40292=CARTESIAN_POINT('Ctrl Pts',(4.16308914079174,3.25966464129901,397.314060879657));
#40293=CARTESIAN_POINT('Ctrl Pts',(5.21375731827273,0.87946540242969,397.234933004198));
#40294=CARTESIAN_POINT('Ctrl Pts',(5.00200160188481,-1.71368163398425,397.155805128738));
#40295=CARTESIAN_POINT('Ctrl Pts',(3.57909508696266,-3.89188940315535,397.076677253278));
#40296=CARTESIAN_POINT('Ctrl Pts',(1.28957072230382,-5.12774142484681,396.997549377819));
#40297=CARTESIAN_POINT('Ctrl Pts',(-1.31220156516579,-5.12199685867627,
396.918421502358));
#40298=CARTESIAN_POINT('Ctrl Pts',(-3.59624625077107,-3.87604665499891,
396.839293626899));
#40299=CARTESIAN_POINT('Ctrl Pts',(-4.84699459687274,-1.94278943218135,
396.769265407658));
#40300=CARTESIAN_POINT('Ctrl Pts',(-5.07292390999909,-0.550710271536964,
396.725613146904));
#40301=CARTESIAN_POINT('Ctrl Pts',(-5.07333567377534,0.000103933621520939,
396.708336844637));
#40302=CARTESIAN_POINT('Ctrl Pts',(-5.0739418421154,7.48951186850533E-5,
397.791663155363));
#40303=CARTESIAN_POINT('Ctrl Pts',(-5.07399707454689,0.0770308345755981,
397.789248599284));
#40304=CARTESIAN_POINT('Ctrl Pts',(-5.05354999565328,0.994603307815543,
397.760458084718));
#40305=CARTESIAN_POINT('Ctrl Pts',(-4.52773440061085,2.73063104480294,397.705291611666));
#40306=CARTESIAN_POINT('Ctrl Pts',(-2.67721733102668,4.55952103490808,397.626163736206));
#40307=CARTESIAN_POINT('Ctrl Pts',(-0.178456984770649,5.28439947486034,
397.547035860747));
#40308=CARTESIAN_POINT('Ctrl Pts',(2.36351372741711,4.72974920747697,397.467907985287));
#40309=CARTESIAN_POINT('Ctrl Pts',(4.33319922937441,3.02986949287705,397.388780109827));
#40310=CARTESIAN_POINT('Ctrl Pts',(5.25367321071018,0.596357694998765,397.309652234368));
#40311=CARTESIAN_POINT('Ctrl Pts',(4.90205833425909,-1.98155211711401,397.230524358907));
#40312=CARTESIAN_POINT('Ctrl Pts',(3.36349224536493,-4.07966231699243,397.151396483448));
#40313=CARTESIAN_POINT('Ctrl Pts',(1.01051291891753,-5.18995070747486,397.072268607988));
#40314=CARTESIAN_POINT('Ctrl Pts',(-1.58714516337332,-5.04357957562867,
396.993140732529));
#40315=CARTESIAN_POINT('Ctrl Pts',(-3.80050266261658,-3.67599023621695,
396.914012857068));
#40316=CARTESIAN_POINT('Ctrl Pts',(-4.89803666817087,-1.7598107945601,396.84685366468));
#40317=CARTESIAN_POINT('Ctrl Pts',(-5.07307953403386,-0.459343943622233,
396.806070430778));
#40318=CARTESIAN_POINT('Ctrl Pts',(-5.07319204280361,3.53449165107697E-5,
396.791663155363));
#40319=CARTESIAN_POINT('Origin',(0.,0.,402.208336844637));
#40320=CARTESIAN_POINT('',(-5.07350261625086,-0.000127405426567639,398.791663155363));
#40321=CARTESIAN_POINT('',(-5.07327504304777,-8.56681209023223E-5,398.708336844637));
#40322=CARTESIAN_POINT('',(-5.0736,-1.59740085886799E-13,402.208336844637));
#40323=CARTESIAN_POINT('Ctrl Pts',(-5.07327504304777,-8.56681209025073E-5,
398.708336844637));
#40324=CARTESIAN_POINT('Ctrl Pts',(-5.07295870657578,0.521766948573649,
398.691969483916));
#40325=CARTESIAN_POINT('Ctrl Pts',(-4.86376568515234,1.88483153888263,398.649226164708));
#40326=CARTESIAN_POINT('Ctrl Pts',(-3.66212405277363,3.81386578025083,398.580106887014));
#40327=CARTESIAN_POINT('Ctrl Pts',(-1.39976059402284,5.09876407058445,398.500979011554));
#40328=CARTESIAN_POINT('Ctrl Pts',(1.2015314169661,5.14908215334412,398.421851136094));
#40329=CARTESIAN_POINT('Ctrl Pts',(3.51189274640949,3.9526363487746,398.342723260634));
#40330=CARTESIAN_POINT('Ctrl Pts',(4.97190814582059,1.79912594262636,398.263595385175));
#40331=CARTESIAN_POINT('Ctrl Pts',(5.22805937238099,-0.790012637095727,
398.184467509715));
#40332=CARTESIAN_POINT('Ctrl Pts',(4.21832370253235,-3.18786290617544,398.105339634255));
#40333=CARTESIAN_POINT('Ctrl Pts',(2.18719169429123,-4.81382563667766,398.026211758795));
#40334=CARTESIAN_POINT('Ctrl Pts',(-0.37353210098369,-5.27420122269227,
397.947083883336));
#40335=CARTESIAN_POINT('Ctrl Pts',(-2.84381136257153,-4.45751743709679,
397.867956007876));
#40336=CARTESIAN_POINT('Ctrl Pts',(-4.62550939672404,-2.56152056184034,
397.788828132416));
#40337=CARTESIAN_POINT('Ctrl Pts',(-5.07044892396789,-0.869584543074369,
397.73562174467));
#40338=CARTESIAN_POINT('Ctrl Pts',(-5.07403418765037,-0.0144991493159696,
397.70879131541));
#40339=CARTESIAN_POINT('Ctrl Pts',(-5.07403169783887,-1.51513653288493E-5,
397.708336844637));
#40340=CARTESIAN_POINT('Ctrl Pts',(-5.07350261625086,-0.000127405426567848,
398.791663155363));
#40341=CARTESIAN_POINT('Ctrl Pts',(-5.07291128030502,0.613121580961722,
398.77242676779));
#40342=CARTESIAN_POINT('Ctrl Pts',(-4.80890661569317,2.06772180201207,398.72681442173));
#40343=CARTESIAN_POINT('Ctrl Pts',(-3.45061727711166,4.00624076891526,398.654826117184));
#40344=CARTESIAN_POINT('Ctrl Pts',(-1.12210802579434,5.16697186848109,398.575698241724));
#40345=CARTESIAN_POINT('Ctrl Pts',(1.47810086651078,5.07660738405961,398.496570366264));
#40346=CARTESIAN_POINT('Ctrl Pts',(3.72041242270134,3.75702756318667,398.417442490805));
#40347=CARTESIAN_POINT('Ctrl Pts',(5.06188850671742,1.52774652711538,398.338314615344));
#40348=CARTESIAN_POINT('Ctrl Pts',(5.17771318239863,-1.0714527081918,398.259186739885));
#40349=CARTESIAN_POINT('Ctrl Pts',(4.03984144729043,-3.41121763982034,398.180058864425));
#40350=CARTESIAN_POINT('Ctrl Pts',(1.92378985850489,-4.92501342998799,398.100930988965));
#40351=CARTESIAN_POINT('Ctrl Pts',(-0.658075180315041,-5.24629981628919,
398.021803113506));
#40352=CARTESIAN_POINT('Ctrl Pts',(-3.08059835091328,-4.29728268859095,
397.942675238046));
#40353=CARTESIAN_POINT('Ctrl Pts',(-4.70604526230202,-2.36846041862021,
397.865961918665));
#40354=CARTESIAN_POINT('Ctrl Pts',(-5.07339373038246,-0.763615063923845,
397.81562455777));
#40355=CARTESIAN_POINT('Ctrl Pts',(-5.0739418421154,7.48951186850533E-5,
397.791663155363));
#40356=CARTESIAN_POINT('Origin',(0.,0.,402.208336844637));
#40357=CARTESIAN_POINT('',(-5.07330191118131,0.000105688062508047,399.791663155363));
#40358=CARTESIAN_POINT('',(-5.07353386009457,0.000128968315485679,399.708336844637));
#40359=CARTESIAN_POINT('',(-5.0736,-1.59740085886799E-13,402.208336844637));
#40360=CARTESIAN_POINT('',(-1.31303618635556,-4.90075024188347,400.));
#40361=CARTESIAN_POINT('Ctrl Pts',(-1.31303618635555,-4.90075024188347,
400.));
#40362=CARTESIAN_POINT('Ctrl Pts',(-2.12521319086393,-4.68314727417224,
399.973624041513));
#40363=CARTESIAN_POINT('Ctrl Pts',(-3.63845957255092,-3.83644859241818,
399.92087212454));
#40364=CARTESIAN_POINT('Ctrl Pts',(-4.85784323874867,-1.90558193017489,
399.851426509661));
#40365=CARTESIAN_POINT('Ctrl Pts',(-5.07295978880057,-0.532132079631421,
399.808356853268));
#40366=CARTESIAN_POINT('Ctrl Pts',(-5.07330191118131,0.000105688062508012,
399.791663155363));
#40367=CARTESIAN_POINT('',(1.31318543090008,-4.90112867346845,400.));
#40368=CARTESIAN_POINT('Origin',(0.,0.,400.));
#40369=CARTESIAN_POINT('Ctrl Pts',(1.31318543090008,-4.90112867346845,400.));
#40370=CARTESIAN_POINT('Ctrl Pts',(0.546344064728336,-5.10618409880194,
399.975093589943));
#40371=CARTESIAN_POINT('Ctrl Pts',(-1.13368018453605,-5.15247589033718,
399.923811221401));
#40372=CARTESIAN_POINT('Ctrl Pts',(-3.42590833126468,-4.02739560525483,
399.84615289437));
#40373=CARTESIAN_POINT('Ctrl Pts',(-4.8023079180703,-2.08851222235156,399.77383825264));
#40374=CARTESIAN_POINT('Ctrl Pts',(-5.07291903260815,-0.623512076348425,
399.727899569395));
#40375=CARTESIAN_POINT('Ctrl Pts',(-5.07353386009457,0.000128968315485402,
399.708336844637));
#40376=CARTESIAN_POINT('Origin',(0.,0.,20.5));
#40377=CARTESIAN_POINT('',(4.51807726312575,-5.77016670283426E-5,39.6125833024919));
#40378=CARTESIAN_POINT('',(4.51743491291879,0.00013078575649096,39.887416697508));
#40379=CARTESIAN_POINT('',(4.51775,5.53264807684796E-16,20.5));
#40380=CARTESIAN_POINT('',(3.43378788736186,2.93584158413001,40.));
#40381=CARTESIAN_POINT('Ctrl Pts',(4.51743491291879,0.00013078575649096,
39.887416697508));
#40382=CARTESIAN_POINT('Ctrl Pts',(4.51757757737092,0.314458352690014,39.8984871683209));
#40383=CARTESIAN_POINT('Ctrl Pts',(4.48524528727997,0.628740973485904,39.9095576391338));
#40384=CARTESIAN_POINT('Ctrl Pts',(4.42014586550123,0.936043740039879,39.9206281099466));
#40385=CARTESIAN_POINT('Ctrl Pts',(4.26456488388791,1.67046602470259,39.9470854066311));
#40386=CARTESIAN_POINT('Ctrl Pts',(3.92183073605335,2.36502208507763,39.9735427033156));
#40387=CARTESIAN_POINT('Ctrl Pts',(3.43378788736169,2.9358415841302,40.));
#40388=CARTESIAN_POINT('',(4.51775,5.53264807684796E-16,40.));
#40389=CARTESIAN_POINT('Origin',(0.,0.,40.));
#40390=CARTESIAN_POINT('',(4.51775,-5.53264807684796E-16,41.));
#40391=CARTESIAN_POINT('',(4.51775,5.53264807684796E-16,20.5));
#40392=CARTESIAN_POINT('Origin',(0.,0.,41.));
#40393=CARTESIAN_POINT('',(-3.4340910891448,2.93606647242268,40.));
#40394=CARTESIAN_POINT('Origin',(0.,0.,40.));
#40395=CARTESIAN_POINT('Ctrl Pts',(-3.4340910891448,2.93606647242268,40.));
#40396=CARTESIAN_POINT('Ctrl Pts',(-2.96705577784696,3.4818800261268,39.974686898954));
#40397=CARTESIAN_POINT('Ctrl Pts',(-2.36757358452893,3.91460873741648,39.949373797908));
#40398=CARTESIAN_POINT('Ctrl Pts',(-1.70215900486053,4.18523117809469,39.9240606968621));
#40399=CARTESIAN_POINT('Ctrl Pts',(-1.00666654344796,4.46808621784234,39.8976034001776));
#40400=CARTESIAN_POINT('Ctrl Pts',(-0.239146468763622,4.57384880856985,
39.8711461034931));
#40401=CARTESIAN_POINT('Ctrl Pts',(0.506923795872781,4.48961228541996,39.8446888068086));
#40402=CARTESIAN_POINT('Ctrl Pts',(1.25299406050918,4.40537576227008,39.8182315101241));
#40403=CARTESIAN_POINT('Ctrl Pts',(1.97761451509765,4.1311401252428,39.7917742134397));
#40404=CARTESIAN_POINT('Ctrl Pts',(2.59252418705981,3.70032015205324,39.7653169167552));
#40405=CARTESIAN_POINT('Ctrl Pts',(3.2074338590219,3.26950017886373,39.7388596200708));
#40406=CARTESIAN_POINT('Ctrl Pts',(3.71263274835769,2.68209586951196,39.7124023233863));
#40407=CARTESIAN_POINT('Ctrl Pts',(4.0465897798431,2.00964543895381,39.6859450267018));
#40408=CARTESIAN_POINT('Ctrl Pts',(4.35525905337691,1.38811402527266,39.6614911186319));
#40409=CARTESIAN_POINT('Ctrl Pts',(4.51763802149368,0.693928511700309,39.6370372105619));
#40410=CARTESIAN_POINT('Ctrl Pts',(4.51807726312575,-5.77016670283426E-5,
39.6125833024919));
#40411=CARTESIAN_POINT('Origin',(0.,0.,20.5));
#40412=CARTESIAN_POINT('',(4.5173663293175,-1.61899228900975E-5,38.6125833024919));
#40413=CARTESIAN_POINT('',(4.51813342681501,1.37750411066654E-5,38.887416697508));
#40414=CARTESIAN_POINT('',(4.51775,5.53264807684796E-16,20.5));
#40415=CARTESIAN_POINT('Ctrl Pts',(4.51813342681501,1.37750411066654E-5,
38.887416697508));
#40416=CARTESIAN_POINT('Ctrl Pts',(4.51813570137199,0.0130379216071904,
38.8878756447561));
#40417=CARTESIAN_POINT('Ctrl Pts',(4.51808056261842,0.0260620488529043,
38.8883345920043));
#40418=CARTESIAN_POINT('Ctrl Pts',(4.51796789313227,0.039085678406741,38.8887935392524));
#40419=CARTESIAN_POINT('Ctrl Pts',(4.5114727457387,0.789869199672342,38.9152508359369));
#40420=CARTESIAN_POINT('Ctrl Pts',(4.31378754306059,1.53899875733816,38.9417081326213));
#40421=CARTESIAN_POINT('Ctrl Pts',(3.94899006576268,2.19523105353971,38.9681654293058));
#40422=CARTESIAN_POINT('Ctrl Pts',(3.58419258846473,2.85146334974134,38.9946227259902));
#40423=CARTESIAN_POINT('Ctrl Pts',(3.05228283654696,3.41479838447868,39.0210800226747));
#40424=CARTESIAN_POINT('Ctrl Pts',(2.4180469390752,3.81662285121831,39.0475373193592));
#40425=CARTESIAN_POINT('Ctrl Pts',(1.78381104160343,4.21844731795794,39.0739946160436));
#40426=CARTESIAN_POINT('Ctrl Pts',(1.04724899857768,4.45876121669985,39.1004519127281));
#40427=CARTESIAN_POINT('Ctrl Pts',(0.298073044029034,4.50829405706009,39.1269092094126));
#40428=CARTESIAN_POINT('Ctrl Pts',(-0.45110291051953,4.55782689742033,39.1533665060971));
#40429=CARTESIAN_POINT('Ctrl Pts',(-1.21289277659099,4.41657867939895,39.1798238027815));
#40430=CARTESIAN_POINT('Ctrl Pts',(-1.89451099954058,4.10175426806426,39.206281099466));
#40431=CARTESIAN_POINT('Ctrl Pts',(-2.57612922249017,3.78692985672956,39.2327383961504));
#40432=CARTESIAN_POINT('Ctrl Pts',(-3.17757580231788,3.29852925208155,39.2591956928349));
#40433=CARTESIAN_POINT('Ctrl Pts',(-3.62559595151898,2.69603724086566,39.2856529895194));
#40434=CARTESIAN_POINT('Ctrl Pts',(-4.07361610072013,2.0935452296497,39.3121102862039));
#40435=CARTESIAN_POINT('Ctrl Pts',(-4.36820981929462,1.37696181186582,39.3385675828883));
#40436=CARTESIAN_POINT('Ctrl Pts',(-4.4734945205513,0.633569578843569,39.3650248795728));
#40437=CARTESIAN_POINT('Ctrl Pts',(-4.57877922180797,-0.109822654178678,
39.3914821762572));
#40438=CARTESIAN_POINT('Ctrl Pts',(-4.49475490574683,-0.880023702439293,
39.4179394729417));
#40439=CARTESIAN_POINT('Ctrl Pts',(-4.23165828048028,-1.5832305850457,39.4443967696262));
#40440=CARTESIAN_POINT('Ctrl Pts',(-3.96856165521376,-2.28643746765202,
39.4708540663107));
#40441=CARTESIAN_POINT('Ctrl Pts',(-3.52639272074186,-2.92265018460415,
39.4973113629951));
#40442=CARTESIAN_POINT('Ctrl Pts',(-2.95900217961984,-3.41436616507676,
39.5237686596796));
#40443=CARTESIAN_POINT('Ctrl Pts',(-2.39161163849769,-3.90608214554949,
39.5502259563641));
#40444=CARTESIAN_POINT('Ctrl Pts',(-1.69899949072535,-4.25330138954263,
39.5766832530485));
#40445=CARTESIAN_POINT('Ctrl Pts',(-0.965534545329121,-4.41375671437606,
39.603140549733));
#40446=CARTESIAN_POINT('Ctrl Pts',(-0.232069599933061,-4.57421203920946,
39.6295978464175));
#40447=CARTESIAN_POINT('Ctrl Pts',(0.542248143086867,-4.54790344488323,
39.6560551431019));
#40448=CARTESIAN_POINT('Ctrl Pts',(1.26312545635919,-4.33799038903366,39.6825124397864));
#40449=CARTESIAN_POINT('Ctrl Pts',(1.98400276963152,-4.12807733318409,39.7089697364709));
#40450=CARTESIAN_POINT('Ctrl Pts',(2.65143965315624,-3.73455981581118,39.7354270331553));
#40451=CARTESIAN_POINT('Ctrl Pts',(3.18410908512153,-3.20545326780569,39.7618843298398));
#40452=CARTESIAN_POINT('Ctrl Pts',(3.71677851708688,-2.67634671980015,39.7883416265243));
#40453=CARTESIAN_POINT('Ctrl Pts',(4.11468049749276,-2.01165114116199,39.8147989232087));
#40454=CARTESIAN_POINT('Ctrl Pts',(4.32941757999969,-1.29215909736769,39.8412562198932));
#40455=CARTESIAN_POINT('Ctrl Pts',(4.45430267828147,-0.873722590951435,
39.8566430457648));
#40456=CARTESIAN_POINT('Ctrl Pts',(4.51723662387398,-0.436752488749845,
39.8720298716364));
#40457=CARTESIAN_POINT('Ctrl Pts',(4.51743491291879,0.00013078575649096,
39.887416697508));
#40458=CARTESIAN_POINT('Ctrl Pts',(4.51807726312575,-5.77016670283426E-5,
39.6125833024919));
#40459=CARTESIAN_POINT('Ctrl Pts',(4.51811324803589,-0.0569125845144851,
39.6105799138774));
#40460=CARTESIAN_POINT('Ctrl Pts',(4.51706233879025,-0.113766129714702,
39.6085765252629));
#40461=CARTESIAN_POINT('Ctrl Pts',(4.51491593042487,-0.170578278221581,
39.6065731366484));
#40462=CARTESIAN_POINT('Ctrl Pts',(4.48656987588623,-0.920855013074376,
39.580115839964));
#40463=CARTESIAN_POINT('Ctrl Pts',(4.26716259317389,-1.66391193101533,39.5536585432795));
#40464=CARTESIAN_POINT('Ctrl Pts',(3.88341809255801,-2.30924747945226,39.527201246595));
#40465=CARTESIAN_POINT('Ctrl Pts',(3.49967359194214,-2.9545830278892,39.5007439499106));
#40466=CARTESIAN_POINT('Ctrl Pts',(2.95159187342274,-3.50219720682209,39.4742866532261));
#40467=CARTESIAN_POINT('Ctrl Pts',(2.305928447501,-3.88539017854137,39.4478293565416));
#40468=CARTESIAN_POINT('Ctrl Pts',(1.66026502157934,-4.2685831502606,39.4213720598571));
#40469=CARTESIAN_POINT('Ctrl Pts',(0.917019888255395,-4.48735491476624,
39.3949147631727));
#40470=CARTESIAN_POINT('Ctrl Pts',(0.16671960730651,-4.51505986234427,39.3684574664882));
#40471=CARTESIAN_POINT('Ctrl Pts',(-0.58358067364246,-4.54276480992229,
39.3420001698038));
#40472=CARTESIAN_POINT('Ctrl Pts',(-1.34093610221634,-4.37940294057267,
39.3155428731193));
#40473=CARTESIAN_POINT('Ctrl Pts',(-2.0131016916631,-4.0448712583889,39.2890855764348));
#40474=CARTESIAN_POINT('Ctrl Pts',(-2.68526728110987,-3.71033957620513,
39.2626282797503));
#40475=CARTESIAN_POINT('Ctrl Pts',(-3.27224303142949,-3.20463808118724,
39.2361709830659));
#40476=CARTESIAN_POINT('Ctrl Pts',(-3.70253591076623,-2.58936080975925,
39.2097136863814));
#40477=CARTESIAN_POINT('Ctrl Pts',(-4.13282879010292,-1.97408353833133,
39.1832563896969));
#40478=CARTESIAN_POINT('Ctrl Pts',(-4.40643879845674,-1.24923049049336,
39.1567990930125));
#40479=CARTESIAN_POINT('Ctrl Pts',(-4.49004055820742,-0.503087883692005,
39.130341796328));
#40480=CARTESIAN_POINT('Ctrl Pts',(-4.5736423179581,0.243054723109393,39.1038844996435));
#40481=CARTESIAN_POINT('Ctrl Pts',(-4.46723582910558,1.01048688887427,39.0774272029591));
#40482=CARTESIAN_POINT('Ctrl Pts',(-4.18378127438633,1.70573618195759,39.0509699062746));
#40483=CARTESIAN_POINT('Ctrl Pts',(-3.90032671966707,2.40098547504095,39.0245126095901));
#40484=CARTESIAN_POINT('Ctrl Pts',(-3.43982409908106,3.02405189544285,38.9980553129056));
#40485=CARTESIAN_POINT('Ctrl Pts',(-2.85836212737563,3.49904666560209,38.9715980162212));
#40486=CARTESIAN_POINT('Ctrl Pts',(-2.27690015567025,3.97404143576128,38.9451407195367));
#40487=CARTESIAN_POINT('Ctrl Pts',(-1.5744788328455,4.30096455567782,38.9186834228523));
#40488=CARTESIAN_POINT('Ctrl Pts',(-0.836652295869176,4.43999713904635,
38.8922261261678));
#40489=CARTESIAN_POINT('Ctrl Pts',(-0.0988257588928058,4.57902972241489,
38.8657688294833));
#40490=CARTESIAN_POINT('Ctrl Pts',(0.67440599223512,4.53017176923538,38.8393115327988));
#40491=CARTESIAN_POINT('Ctrl Pts',(1.38886418452495,4.29937413054893,38.8128542361144));
#40492=CARTESIAN_POINT('Ctrl Pts',(2.10332237681477,4.06857649186248,38.7863969394299));
#40493=CARTESIAN_POINT('Ctrl Pts',(2.75900701026648,3.6558391676691,38.7599396427455));
#40494=CARTESIAN_POINT('Ctrl Pts',(3.27605642296661,3.11143310386805,38.733482346061));
#40495=CARTESIAN_POINT('Ctrl Pts',(3.79310583566678,2.56702704006697,38.7070250493765));
#40496=CARTESIAN_POINT('Ctrl Pts',(4.17152002761535,1.89095223665823,38.680567752692));
#40497=CARTESIAN_POINT('Ctrl Pts',(4.36520856862573,1.1655538582636,38.6541104560076));
#40498=CARTESIAN_POINT('Ctrl Pts',(4.46654587798484,0.786027431472861,38.6402680715023));
#40499=CARTESIAN_POINT('Ctrl Pts',(4.51731724698707,0.392999398715342,38.6264256869971));
#40500=CARTESIAN_POINT('Ctrl Pts',(4.5173663293175,-1.61899228900975E-5,
38.6125833024919));
#40501=CARTESIAN_POINT('Origin',(0.,0.,20.5));
#40502=CARTESIAN_POINT('',(4.51799626797168,8.54686663623316E-5,37.6125833024919));
#40503=CARTESIAN_POINT('',(4.51744515673179,-7.51896715610657E-5,37.887416697508));
#40504=CARTESIAN_POINT('',(4.51775,5.53264807684796E-16,20.5));
#40505=CARTESIAN_POINT('Ctrl Pts',(4.51744515673179,-7.51896715610657E-5,
37.887416697508));
#40506=CARTESIAN_POINT('Ctrl Pts',(4.51717073079397,0.462828384782965,37.9037214178759));
#40507=CARTESIAN_POINT('Ctrl Pts',(4.44640538068968,0.925813963613659,37.9200261382437));
#40508=CARTESIAN_POINT('Ctrl Pts',(4.30642900683072,1.36683241594085,37.9363308586115));
#40509=CARTESIAN_POINT('Ctrl Pts',(4.07929254766704,2.0824629679108,37.962788155296));
#40510=CARTESIAN_POINT('Ctrl Pts',(3.66991785444932,2.74025229569321,37.9892454519805));
#40511=CARTESIAN_POINT('Ctrl Pts',(3.12816631171535,3.26008238708871,38.0157027486649));
#40512=CARTESIAN_POINT('Ctrl Pts',(2.58641476898142,3.77991247848417,38.0421600453494));
#40513=CARTESIAN_POINT('Ctrl Pts',(1.91228637673127,4.16178333349271,38.0686173420339));
#40514=CARTESIAN_POINT('Ctrl Pts',(1.18788922711554,4.35918350473768,38.0950746387183));
#40515=CARTESIAN_POINT('Ctrl Pts',(0.463492077499819,4.55658367598265,38.1215319354028));
#40516=CARTESIAN_POINT('Ctrl Pts',(-0.311173829481454,4.56951316346404,
38.1479892320873));
#40517=CARTESIAN_POINT('Ctrl Pts',(-1.04175504380602,4.39639716966122,38.1744465287717));
#40518=CARTESIAN_POINT('Ctrl Pts',(-1.77233625813064,4.2232811758584,38.2009038254562));
#40519=CARTESIAN_POINT('Ctrl Pts',(-2.45883277979851,3.86411970077134,38.2273611221407));
#40520=CARTESIAN_POINT('Ctrl Pts',(-3.01763009204679,3.36265821505168,38.2538184188251));
#40521=CARTESIAN_POINT('Ctrl Pts',(-3.57642740429506,2.86119672933201,38.2802757155096));
#40522=CARTESIAN_POINT('Ctrl Pts',(-4.00752550712371,2.21743523297976,38.3067330121941));
#40523=CARTESIAN_POINT('Ctrl Pts',(-4.25841712907836,1.50978316287097,38.3331903088785));
#40524=CARTESIAN_POINT('Ctrl Pts',(-4.50930875103297,0.802131092762298,
38.359647605563));
#40525=CARTESIAN_POINT('Ctrl Pts',(-4.57999389211364,0.0305884488970126,
38.3861049022475));
#40526=CARTESIAN_POINT('Ctrl Pts',(-4.46186317968564,-0.710871726876464,
38.412562198932));
#40527=CARTESIAN_POINT('Ctrl Pts',(-4.34373246725763,-1.45233190264998,
38.4390194956164));
#40528=CARTESIAN_POINT('Ctrl Pts',(-4.03678590132095,-2.16370961033178,
38.4654767923008));
#40529=CARTESIAN_POINT('Ctrl Pts',(-3.57840923518433,-2.75835983566992,
38.4919340889853));
#40530=CARTESIAN_POINT('Ctrl Pts',(-3.12003256904766,-3.35301006100813,
38.5183913856698));
#40531=CARTESIAN_POINT('Ctrl Pts',(-2.51022580271103,-3.83093280400264,
38.5448486823543));
#40532=CARTESIAN_POINT('Ctrl Pts',(-1.82326272299569,-4.13391759737145,
38.5713059790388));
#40533=CARTESIAN_POINT('Ctrl Pts',(-1.13629964328034,-4.43690239074026,
38.5977632757232));
#40534=CARTESIAN_POINT('Ctrl Pts',(-0.372180250186292,-4.56494923448336,
38.6242205724077));
#40535=CARTESIAN_POINT('Ctrl Pts',(0.376026555300945,-4.50246217629699,
38.6506778690921));
#40536=CARTESIAN_POINT('Ctrl Pts',(1.12423336078818,-4.4399751181106,38.6771351657766));
#40537=CARTESIAN_POINT('Ctrl Pts',(1.85652757866858,-4.18695415799474,38.7035924624611));
#40538=CARTESIAN_POINT('Ctrl Pts',(2.48371659230794,-3.77421694705527,38.7300497591456));
#40539=CARTESIAN_POINT('Ctrl Pts',(3.1109056059473,-3.3614797361158,38.7565070558301));
#40540=CARTESIAN_POINT('Ctrl Pts',(3.63298941534561,-2.78902627435273,38.7829643525145));
#40541=CARTESIAN_POINT('Ctrl Pts',(3.98637877399025,-2.12658080103845,38.8094216491989));
#40542=CARTESIAN_POINT('Ctrl Pts',(4.33363798730682,-1.47562658212673,38.8354199986353));
#40543=CARTESIAN_POINT('Ctrl Pts',(4.51800457817832,-0.737775404274226,
38.8614183480717));
#40544=CARTESIAN_POINT('Ctrl Pts',(4.51813342681501,1.37750411066654E-5,
38.887416697508));
#40545=CARTESIAN_POINT('Ctrl Pts',(4.5173663293175,-1.61899228900975E-5,
38.6125833024919));
#40546=CARTESIAN_POINT('Ctrl Pts',(4.51741105927625,-0.358181153038861,
38.5999683903127));
#40547=CARTESIAN_POINT('Ctrl Pts',(4.4753302503181,-0.71633578114697,38.5873534781335));
#40548=CARTESIAN_POINT('Ctrl Pts',(4.39100556896819,-1.06425172631817,38.5747385659542));
#40549=CARTESIAN_POINT('Ctrl Pts',(4.21415113822809,-1.79393697912487,38.5482812692697));
#40550=CARTESIAN_POINT('Ctrl Pts',(3.85147938667571,-2.47858553135783,38.5218239725852));
#40551=CARTESIAN_POINT('Ctrl Pts',(3.34716333215496,-3.0348079465722,38.4953666759008));
#40552=CARTESIAN_POINT('Ctrl Pts',(2.84284727763424,-3.59103036178655,38.4689093792163));
#40553=CARTESIAN_POINT('Ctrl Pts',(2.19688692014516,-4.01882663998234,38.4424520825318));
#40554=CARTESIAN_POINT('Ctrl Pts',(1.48795951638629,-4.26609166819816,38.4159947858474));
#40555=CARTESIAN_POINT('Ctrl Pts',(0.779032112627345,-4.513356696414,38.3895374891629));
#40556=CARTESIAN_POINT('Ctrl Pts',(0.00713766259859555,-4.58009047464984,
38.3630801924784));
#40557=CARTESIAN_POINT('Ctrl Pts',(-0.733707943998393,-4.45816490243132,
38.336622895794));
#40558=CARTESIAN_POINT('Ctrl Pts',(-1.4745535505953,-4.33623933021282,38.3101655991095));
#40559=CARTESIAN_POINT('Ctrl Pts',(-2.18435031376045,-4.02565440754,38.283708302425));
#40560=CARTESIAN_POINT('Ctrl Pts',(-2.77664577327751,-3.56423903433536,
38.2572510057406));
#40561=CARTESIAN_POINT('Ctrl Pts',(-3.36894123279463,-3.10282366113066,
38.2307937090561));
#40562=CARTESIAN_POINT('Ctrl Pts',(-3.84373538866364,-2.49057783739411,
38.2043364123716));
#40563=CARTESIAN_POINT('Ctrl Pts',(-4.14319883817823,-1.80207242682554,
38.1778791156872));
#40564=CARTESIAN_POINT('Ctrl Pts',(-4.44266228769283,-1.11356701625697,
38.1514218190027));
#40565=CARTESIAN_POINT('Ctrl Pts',(-4.56679503085301,-0.348802018856373,
38.1249645223182));
#40566=CARTESIAN_POINT('Ctrl Pts',(-4.50047783691868,0.399075035061113,
38.0985072256338));
#40567=CARTESIAN_POINT('Ctrl Pts',(-4.43416064298434,1.14695208897856,38.0720499289493));
#40568=CARTESIAN_POINT('Ctrl Pts',(-4.17739351195555,1.87794119941278,38.0455926322648));
#40569=CARTESIAN_POINT('Ctrl Pts',(-3.76145039622188,2.50300870173274,38.0191353355804));
#40570=CARTESIAN_POINT('Ctrl Pts',(-3.34550728048821,3.1280762040527,37.9926780388959));
#40571=CARTESIAN_POINT('Ctrl Pts',(-2.77038818004956,3.64722209825836,37.9662207422114));
#40572=CARTESIAN_POINT('Ctrl Pts',(-2.10614196483595,3.99721498898437,37.9397634455269));
#40573=CARTESIAN_POINT('Ctrl Pts',(-1.4418957496223,4.34720787971039,37.9133061488425));
#40574=CARTESIAN_POINT('Ctrl Pts',(-0.688522419633467,4.52804776695686,
37.886848852158));
#40575=CARTESIAN_POINT('Ctrl Pts',(0.0622179873187612,4.51770855260138,
37.8603915554735));
#40576=CARTESIAN_POINT('Ctrl Pts',(0.812958394270905,4.5073693382459,37.8339342587891));
#40577=CARTESIAN_POINT('Ctrl Pts',(1.56106587818642,4.30585102228859,37.8074769621046));
#40578=CARTESIAN_POINT('Ctrl Pts',(2.21542177547896,3.93769831258472,37.7810196654202));
#40579=CARTESIAN_POINT('Ctrl Pts',(2.86977767277154,3.56954560288082,37.7545623687357));
#40580=CARTESIAN_POINT('Ctrl Pts',(3.43038198344099,3.03475849943036,37.7281050720512));
#40581=CARTESIAN_POINT('Ctrl Pts',(3.82895372288588,2.3984734795689,37.7016477753667));
#40582=CARTESIAN_POINT('Ctrl Pts',(4.22752546233078,1.76218845970743,37.6751904786822));
#40583=CARTESIAN_POINT('Ctrl Pts',(4.46406463055111,1.02440552343496,37.6487331819978));
#40584=CARTESIAN_POINT('Ctrl Pts',(4.50976101864303,0.274985815861593,37.6222758853133));
#40585=CARTESIAN_POINT('Ctrl Pts',(4.51534128170496,0.18346963073906,37.6190450243729));
#40586=CARTESIAN_POINT('Ctrl Pts',(4.51807563365308,0.0917799142062647,
37.6158141634324));
#40587=CARTESIAN_POINT('Ctrl Pts',(4.51799626797168,8.54686663623316E-5,
37.6125833024919));
#40588=CARTESIAN_POINT('Origin',(0.,0.,20.5));
#40589=CARTESIAN_POINT('',(4.51763788794132,-0.000113968307276224,36.612583302492));
#40590=CARTESIAN_POINT('',(4.51778606435352,0.000115791782295315,36.887416697508));
#40591=CARTESIAN_POINT('',(4.51775,5.53264807684796E-16,20.5));
#40592=CARTESIAN_POINT('Ctrl Pts',(4.51778606435352,0.000115791782295315,
36.887416697508));
#40593=CARTESIAN_POINT('Ctrl Pts',(4.51795287012522,0.16171502012428,36.8931098943111));
#40594=CARTESIAN_POINT('Ctrl Pts',(4.50945045543959,0.323296786803073,36.8988030911142));
#40595=CARTESIAN_POINT('Ctrl Pts',(4.49214571371295,0.483930295567246,36.9044962879172));
#40596=CARTESIAN_POINT('Ctrl Pts',(4.41172750549954,1.23042274011835,36.9309535846017));
#40597=CARTESIAN_POINT('Ctrl Pts',(4.14121195660595,1.9564363604895,36.9574108812862));
#40598=CARTESIAN_POINT('Ctrl Pts',(3.71354756149943,2.57354350122142,36.9838681779707));
#40599=CARTESIAN_POINT('Ctrl Pts',(3.28588316639293,3.1906506419533,37.0103254746552));
#40600=CARTESIAN_POINT('Ctrl Pts',(2.70106992507351,3.69885130304599,37.0367827713396));
#40601=CARTESIAN_POINT('Ctrl Pts',(2.0303374431028,4.03624720641988,37.0632400680241));
#40602=CARTESIAN_POINT('Ctrl Pts',(1.35960496113208,4.37364310979377,37.0896973647085));
#40603=CARTESIAN_POINT('Ctrl Pts',(0.602953238510051,4.54023425544888,37.116154661393));
#40604=CARTESIAN_POINT('Ctrl Pts',(-0.147458382357975,4.51573002621609,
37.1426119580775));
#40605=CARTESIAN_POINT('Ctrl Pts',(-0.897870003226045,4.49122579698331,
37.169069254762));
#40606=CARTESIAN_POINT('Ctrl Pts',(-1.64204152234013,4.27562619286261,37.1955265514464));
#40607=CARTESIAN_POINT('Ctrl Pts',(-2.28933367227002,3.89519100702498,37.2219838481309));
#40608=CARTESIAN_POINT('Ctrl Pts',(-2.93662582219991,3.51475582118734,37.2484411448154));
#40609=CARTESIAN_POINT('Ctrl Pts',(-3.48703860294563,2.96948505363274,37.2748984414998));
#40610=CARTESIAN_POINT('Ctrl Pts',(-3.87353234697123,2.32579208038141,37.3013557381843));
#40611=CARTESIAN_POINT('Ctrl Pts',(-4.26002609099678,1.68209910713015,37.3278130348688));
#40612=CARTESIAN_POINT('Ctrl Pts',(-4.48260079830228,0.939983928182159,
37.3542703315532));
#40613=CARTESIAN_POINT('Ctrl Pts',(-4.51414711586847,0.18983535101083,37.3807276282377));
#40614=CARTESIAN_POINT('Ctrl Pts',(-4.54569343343466,-0.560313226160541,
37.4071849249222));
#40615=CARTESIAN_POINT('Ctrl Pts',(-4.38621136126154,-1.31849520155516,
37.4336422216066));
#40616=CARTESIAN_POINT('Ctrl Pts',(-4.05512563923565,-1.99236484967302,
37.4600995182911));
#40617=CARTESIAN_POINT('Ctrl Pts',(-3.72403991720973,-2.66623449779091,
37.4865568149756));
#40618=CARTESIAN_POINT('Ctrl Pts',(-3.22135054533102,-3.25579181863192,
37.51301411166));
#40619=CARTESIAN_POINT('Ctrl Pts',(-2.60828453275295,-3.68922938300066,
37.5394714083445));
#40620=CARTESIAN_POINT('Ctrl Pts',(-1.99521852017489,-4.1226669473694,37.565928705029));
#40621=CARTESIAN_POINT('Ctrl Pts',(-1.27177586689746,-4.39998475526589,
37.5923860017135));
#40622=CARTESIAN_POINT('Ctrl Pts',(-0.52607108743212,-4.48740580460162,
37.6188432983979));
#40623=CARTESIAN_POINT('Ctrl Pts',(0.219633692033175,-4.57482685393735,
37.6453005950824));
#40624=CARTESIAN_POINT('Ctrl Pts',(0.987600597686399,-4.47235114471234,
37.6717578917668));
#40625=CARTESIAN_POINT('Ctrl Pts',(1.68429211034969,-4.19246010490277,37.6982151884513));
#40626=CARTESIAN_POINT('Ctrl Pts',(2.38098362301298,-3.9125690650932,37.7246724851358));
#40627=CARTESIAN_POINT('Ctrl Pts',(3.00639974268637,-3.45526269469905,37.7511297818202));
#40628=CARTESIAN_POINT('Ctrl Pts',(3.48436547816537,-2.87624040350849,37.7775870785047));
#40629=CARTESIAN_POINT('Ctrl Pts',(3.96233121364435,-2.29721811231796,37.8040443751892));
#40630=CARTESIAN_POINT('Ctrl Pts',(4.29284656492897,-1.596479900331,37.8305016718736));
#40631=CARTESIAN_POINT('Ctrl Pts',(4.43565512801649,-0.859374906258841,
37.8569589685581));
#40632=CARTESIAN_POINT('Ctrl Pts',(4.49045569410255,-0.576522323285484,
37.8671115448747));
#40633=CARTESIAN_POINT('Ctrl Pts',(4.51761603548433,-0.288314654125513,
37.8772641211914));
#40634=CARTESIAN_POINT('Ctrl Pts',(4.51744515673179,-7.51896715610657E-5,
37.887416697508));
#40635=CARTESIAN_POINT('Ctrl Pts',(4.51799626797168,8.54686663623316E-5,
37.6125833024919));
#40636=CARTESIAN_POINT('Ctrl Pts',(4.51742571357972,-0.659099555590392,
37.5893568667479));
#40637=CARTESIAN_POINT('Ctrl Pts',(4.37144018896989,-1.31852897836833,37.5661304310039));
#40638=CARTESIAN_POINT('Ctrl Pts',(4.09200051244546,-1.91548778391919,37.5429039952599));
#40639=CARTESIAN_POINT('Ctrl Pts',(3.77369001019247,-2.59548519725224,37.5164466985755));
#40640=CARTESIAN_POINT('Ctrl Pts',(3.282215397723,-3.19442354504401,37.489989401891));
#40641=CARTESIAN_POINT('Ctrl Pts',(2.67743773890556,-3.63935279939737,37.4635321052065));
#40642=CARTESIAN_POINT('Ctrl Pts',(2.07266008008816,-4.08428205375071,37.4370748085221));
#40643=CARTESIAN_POINT('Ctrl Pts',(1.3545793749228,-4.37520221466565,37.4106175118376));
#40644=CARTESIAN_POINT('Ctrl Pts',(0.610657058576267,-4.47667952851312,
37.3841602151531));
#40645=CARTESIAN_POINT('Ctrl Pts',(-0.133265257770265,-4.57815684236059,
37.3577029184686));
#40646=CARTESIAN_POINT('Ctrl Pts',(-0.903029185297969,-4.49019130914057,
37.3312456217842));
#40647=CARTESIAN_POINT('Ctrl Pts',(-1.60487832955574,-4.22349703344512,
37.3047883250997));
#40648=CARTESIAN_POINT('Ctrl Pts',(-2.30672747381355,-3.95680275774965,
37.2783310284153));
#40649=CARTESIAN_POINT('Ctrl Pts',(-2.94066183480143,-3.51137973957871,
37.2518737317308));
#40650=CARTESIAN_POINT('Ctrl Pts',(-3.42946890894599,-2.94148000958195,
37.2254164350463));
#40651=CARTESIAN_POINT('Ctrl Pts',(-3.91827598309049,-2.37158027958525,
37.1989591383619));
#40652=CARTESIAN_POINT('Ctrl Pts',(-4.26195577039172,-1.67720383776276,
37.1725018416774));
#40653=CARTESIAN_POINT('Ctrl Pts',(-4.41864845311754,-0.942924966240358,
37.1460445449929));
#40654=CARTESIAN_POINT('Ctrl Pts',(-4.57534113584337,-0.208646094717874,
37.1195872483085));
#40655=CARTESIAN_POINT('Ctrl Pts',(-4.54504671399375,0.565535206504528,
37.093129951624));
#40656=CARTESIAN_POINT('Ctrl Pts',(-4.33145501462218,1.28532451174858,37.0666726549395));
#40657=CARTESIAN_POINT('Ctrl Pts',(-4.11786331525061,2.00511381699263,37.040215358255));
#40658=CARTESIAN_POINT('Ctrl Pts',(-3.72097433835709,2.67051112625834,37.0137580615706));
#40659=CARTESIAN_POINT('Ctrl Pts',(-3.18912872207783,3.20047178369309,36.9873007648861));
#40660=CARTESIAN_POINT('Ctrl Pts',(-2.65728310579862,3.73043244112779,36.9608434682017));
#40661=CARTESIAN_POINT('Ctrl Pts',(-1.99048085013371,4.12495644673157,36.9343861715172));
#40662=CARTESIAN_POINT('Ctrl Pts',(-1.26993773185218,4.33599121325395,36.9079288748327));
#40663=CARTESIAN_POINT('Ctrl Pts',(-0.549394613570651,4.54702597977633,
36.8814715781482));
#40664=CARTESIAN_POINT('Ctrl Pts',(0.224889367327489,4.57457150721731,36.8550142814638));
#40665=CARTESIAN_POINT('Ctrl Pts',(0.958607278893124,4.41527278082006,36.8285569847793));
#40666=CARTESIAN_POINT('Ctrl Pts',(1.69232519045884,4.25597405442279,36.8020996880948));
#40667=CARTESIAN_POINT('Ctrl Pts',(2.38547703269204,3.90983107418726,36.7756423914104));
#40668=CARTESIAN_POINT('Ctrl Pts',(2.95363767834151,3.4190036720189,36.7491850947259));
#40669=CARTESIAN_POINT('Ctrl Pts',(3.52179832399097,2.92817626985055,36.7227277980414));
#40670=CARTESIAN_POINT('Ctrl Pts',(3.9649677730567,2.29266444574938,36.6962705013569));
#40671=CARTESIAN_POINT('Ctrl Pts',(4.22916847711195,1.58987283655014,36.6698132046725));
#40672=CARTESIAN_POINT('Ctrl Pts',(4.41966640325359,1.08313556444126,36.6507365706123));
#40673=CARTESIAN_POINT('Ctrl Pts',(4.51712003309545,0.541420116342586,36.6316599365521));
#40674=CARTESIAN_POINT('Ctrl Pts',(4.51763788794132,-0.000113968307276224,
36.612583302492));
#40675=CARTESIAN_POINT('Origin',(0.,0.,20.5));
#40676=CARTESIAN_POINT('',(4.51755220121239,0.000103541448102373,35.6125833024919));
#40677=CARTESIAN_POINT('',(4.51785557016588,-0.00011040733672244,35.887416697508));
#40678=CARTESIAN_POINT('',(4.51775,5.53264807684796E-16,20.5));
#40679=CARTESIAN_POINT('Ctrl Pts',(4.51785557016588,-0.000110407336722441,
35.887416697508));
#40680=CARTESIAN_POINT('Ctrl Pts',(4.51723269271139,0.611237967146432,35.9089556674308));
#40681=CARTESIAN_POINT('Ctrl Pts',(4.39224914626368,1.22283323831731,35.9304946373536));
#40682=CARTESIAN_POINT('Ctrl Pts',(4.1508481772843,1.78438254119822,35.9520336072764));
#40683=CARTESIAN_POINT('Ctrl Pts',(3.85432438440574,2.47415909794758,35.9784909039609));
#40684=CARTESIAN_POINT('Ctrl Pts',(3.38214618261964,3.08842466341222,36.0049482006454));
#40685=CARTESIAN_POINT('Ctrl Pts',(2.79182435432918,3.55236237154543,36.0314054973298));
#40686=CARTESIAN_POINT('Ctrl Pts',(2.20150252603872,4.01630007967864,36.0578627940143));
#40687=CARTESIAN_POINT('Ctrl Pts',(1.4930370712439,4.32990993048042,36.0843200906988));
#40688=CARTESIAN_POINT('Ctrl Pts',(0.752718298257879,4.45499459120493,36.1107773873832));
#40689=CARTESIAN_POINT('Ctrl Pts',(0.0123995252718205,4.58007925192944,
36.1372346840677));
#40690=CARTESIAN_POINT('Ctrl Pts',(-0.759772565905438,4.51663872257667,
36.1636919807522));
#40691=CARTESIAN_POINT('Ctrl Pts',(-1.46974826915546,4.27239998941016,36.1901492774366));
#40692=CARTESIAN_POINT('Ctrl Pts',(-2.17972397240549,4.02816125624364,36.2166065741211));
#40693=CARTESIAN_POINT('Ctrl Pts',(-2.82750328772828,3.60312431926339,36.2430638708056));
#40694=CARTESIAN_POINT('Ctrl Pts',(-3.33418741143512,3.04905820699195,36.26952116749));
#40695=CARTESIAN_POINT('Ctrl Pts',(-3.84087153514189,2.49499209472058,36.2959784641745));
#40696=CARTESIAN_POINT('Ctrl Pts',(-4.20646046723274,1.81189680715804,36.322435760859));
#40697=CARTESIAN_POINT('Ctrl Pts',(-4.3864258803877,1.08297259432656,36.3488930575434));
#40698=CARTESIAN_POINT('Ctrl Pts',(-4.56639129354267,0.354048381494999,
36.3753503542279));
#40699=CARTESIAN_POINT('Ctrl Pts',(-4.56073318776171,-0.420704756605515,
36.4018076509124));
#40700=CARTESIAN_POINT('Ctrl Pts',(-4.37014071406692,-1.14692274519782,
36.4282649475969));
#40701=CARTESIAN_POINT('Ctrl Pts',(-4.17954824037214,-1.87314073379008,
36.4547222442813));
#40702=CARTESIAN_POINT('Ctrl Pts',(-3.80402139876356,-2.55082357287414,
36.4811795409658));
#40703=CARTESIAN_POINT('Ctrl Pts',(-3.28929894294182,-3.09743024266232,
36.5076368376502));
#40704=CARTESIAN_POINT('Ctrl Pts',(-2.77457648712008,-3.64403691245051,
36.5340941343347));
#40705=CARTESIAN_POINT('Ctrl Pts',(-2.12065841708519,-4.05956741294281,
36.5605514310192));
#40706=CARTESIAN_POINT('Ctrl Pts',(-1.40719123005584,-4.29341058905986,
36.5870087277037));
#40707=CARTESIAN_POINT('Ctrl Pts',(-0.693724043026525,-4.52725376517689,
36.6134660243881));
#40708=CARTESIAN_POINT('Ctrl Pts',(0.0792922609972423,-4.57940961691868,
36.6399233210726));
#40709=CARTESIAN_POINT('Ctrl Pts',(0.817705151706661,-4.4435256192656,36.6663806177571));
#40710=CARTESIAN_POINT('Ctrl Pts',(1.55611804241612,-4.30764162161251,36.6928379144415));
#40711=CARTESIAN_POINT('Ctrl Pts',(2.25992751981123,-3.98371777456452,36.719295211126));
#40712=CARTESIAN_POINT('Ctrl Pts',(2.84341036847319,-3.51120764419544,36.7457525078105));
#40713=CARTESIAN_POINT('Ctrl Pts',(3.42689321713519,-3.03869751382634,36.7722098044949));
#40714=CARTESIAN_POINT('Ctrl Pts',(3.89004943706403,-2.41760110013612,36.7986671011794));
#40715=CARTESIAN_POINT('Ctrl Pts',(4.17646711326182,-1.72356725892547,36.8251243978639));
#40716=CARTESIAN_POINT('Ctrl Pts',(4.40125218133937,-1.17887865480133,36.8458884977453));
#40717=CARTESIAN_POINT('Ctrl Pts',(4.51717769407857,-0.589265294821556,
36.8666525976266));
#40718=CARTESIAN_POINT('Ctrl Pts',(4.51778606435352,0.000115791782295315,
36.887416697508));
#40719=CARTESIAN_POINT('Ctrl Pts',(4.51763788794132,-0.000113968307276224,
36.612583302492));
#40720=CARTESIAN_POINT('Ctrl Pts',(4.51783824361694,-0.209631033306269,
36.6052026398677));
#40721=CARTESIAN_POINT('Ctrl Pts',(4.50352846951492,-0.419120950359322,
36.5978219772434));
#40722=CARTESIAN_POINT('Ctrl Pts',(4.47448319596349,-0.626547502778321,
36.5904413146191));
#40723=CARTESIAN_POINT('Ctrl Pts',(4.37036525171502,-1.37010483861031,36.5639840179346));
#40724=CARTESIAN_POINT('Ctrl Pts',(4.07689740417331,-2.08714811597701,36.5375267212501));
#40725=CARTESIAN_POINT('Ctrl Pts',(3.62982371237891,-2.69034225726936,36.5110694245657));
#40726=CARTESIAN_POINT('Ctrl Pts',(3.18275002058453,-3.29353639856167,36.4846121278812));
#40727=CARTESIAN_POINT('Ctrl Pts',(2.58207048453748,-3.78288140377964,36.4581548311967));
#40728=CARTESIAN_POINT('Ctrl Pts',(1.90094720693747,-4.09877559286112,36.4316975345123));
#40729=CARTESIAN_POINT('Ctrl Pts',(1.21982392933739,-4.41466978194264,36.4052402378278));
#40730=CARTESIAN_POINT('Ctrl Pts',(0.458256910184331,-4.55711315488762,
36.3787829411434));
#40731=CARTESIAN_POINT('Ctrl Pts',(-0.290995830438852,-4.50875626651792,
36.3523256444589));
#40732=CARTESIAN_POINT('Ctrl Pts',(-1.04024857106204,-4.46039937814821,
36.3258683477744));
#40733=CARTESIAN_POINT('Ctrl Pts',(-1.77718703315534,-4.2212422284638,36.2994110510899));
#40734=CARTESIAN_POINT('Ctrl Pts',(-2.41205292762861,-3.82041389361357,
36.2729537544055));
#40735=CARTESIAN_POINT('Ctrl Pts',(-3.04691882210185,-3.41958555876337,
36.246496457721));
#40736=CARTESIAN_POINT('Ctrl Pts',(-3.57971214895505,-2.85708603874736,
36.2200391610366));
#40737=CARTESIAN_POINT('Ctrl Pts',(-3.94553927063653,-2.20142715256771,
36.1935818643521));
#40738=CARTESIAN_POINT('Ctrl Pts',(-4.311366392318,-1.54576826638806,36.1671245676676));
#40739=CARTESIAN_POINT('Ctrl Pts',(-4.51022730882774,-0.796950014044777,
36.1406672709831));
#40740=CARTESIAN_POINT('Ctrl Pts',(-4.51790098062044,-0.0461776299327186,
36.1142099742986));
#40741=CARTESIAN_POINT('Ctrl Pts',(-4.52557465241315,0.70459475417934,36.0877526776142));
#40742=CARTESIAN_POINT('Ctrl Pts',(-4.34206107948882,1.45732127006017,36.0612953809297));
#40743=CARTESIAN_POINT('Ctrl Pts',(-3.98971201192945,2.12032066114143,36.0348380842453));
#40744=CARTESIAN_POINT('Ctrl Pts',(-3.63736294437007,2.78332005222269,36.0083807875608));
#40745=CARTESIAN_POINT('Ctrl Pts',(-3.11617838217574,3.3565923185043,35.9819234908763));
#40746=CARTESIAN_POINT('Ctrl Pts',(-2.48963802821032,3.77031353241165,35.9554661941919));
#40747=CARTESIAN_POINT('Ctrl Pts',(-1.86309767424487,4.18403474631902,35.9290088975074));
#40748=CARTESIAN_POINT('Ctrl Pts',(-1.13120152850826,4.43820490785206,35.9025516008229));
#40749=CARTESIAN_POINT('Ctrl Pts',(-0.383093731539153,4.501866372634,35.8760943041385));
#40750=CARTESIAN_POINT('Ctrl Pts',(0.365014065429868,4.56552783741593,35.849637007454));
#40751=CARTESIAN_POINT('Ctrl Pts',(1.12933351363151,4.43868060544686,35.8231797107695));
#40752=CARTESIAN_POINT('Ctrl Pts',(1.81677135017102,4.13677452919484,35.7967224140851));
#40753=CARTESIAN_POINT('Ctrl Pts',(2.50420918671061,3.83486845294278,35.7702651174006));
#40754=CARTESIAN_POINT('Ctrl Pts',(3.11476541158806,3.35790353240771,35.7438078207161));
#40755=CARTESIAN_POINT('Ctrl Pts',(3.57407495233493,2.76397356703885,35.7173505240316));
#40756=CARTESIAN_POINT('Ctrl Pts',(4.03338449308179,2.17004360166999,35.6908932273472));
#40757=CARTESIAN_POINT('Ctrl Pts',(4.34144734969803,1.45914859146745,35.6644359306627));
#40758=CARTESIAN_POINT('Ctrl Pts',(4.46074180719067,0.717874761903989,35.6379786339782));
#40759=CARTESIAN_POINT('Ctrl Pts',(4.49891051264125,0.480701442593838,35.6295135234828));
#40760=CARTESIAN_POINT('Ctrl Pts',(4.51775492478579,0.240418231912197,35.6210484129874));
#40761=CARTESIAN_POINT('Ctrl Pts',(4.51755220121239,0.000103541448102373,
35.6125833024919));
#40762=CARTESIAN_POINT('Origin',(0.,0.,20.5));
#40763=CARTESIAN_POINT('',(4.51806911322653,-6.09724841136444E-5,34.6125833024919));
#40764=CARTESIAN_POINT('',(4.51740954388543,5.82741782004033E-5,34.887416697508));
#40765=CARTESIAN_POINT('',(4.51775,5.53264807684796E-16,20.5));
#40766=CARTESIAN_POINT('Ctrl Pts',(4.51740954388543,5.82741782004033E-5,
34.887416697508));
#40767=CARTESIAN_POINT('Ctrl Pts',(4.51755065915555,0.31030389790581,34.8983441438661));
#40768=CARTESIAN_POINT('Ctrl Pts',(4.48605373157874,0.620521268509011,34.9092715902241));
#40769=CARTESIAN_POINT('Ctrl Pts',(4.42263045256682,0.924067921868281,34.9201990365822));
#40770=CARTESIAN_POINT('Ctrl Pts',(4.26907138171545,1.65900851112936,34.9466563332667));
#40771=CARTESIAN_POINT('Ctrl Pts',(3.92835669717202,2.35484465771423,34.9731136299511));
#40772=CARTESIAN_POINT('Ctrl Pts',(3.44198507043434,2.92682428907246,34.9995709266356));
#40773=CARTESIAN_POINT('Ctrl Pts',(2.95561344369671,3.49880392043062,35.02602822332));
#40774=CARTESIAN_POINT('Ctrl Pts',(2.32358487476487,3.94692703656216,35.0524855200045));
#40775=CARTESIAN_POINT('Ctrl Pts',(1.62287974384894,4.21661273787411,35.078942816689));
#40776=CARTESIAN_POINT('Ctrl Pts',(0.922174612932932,4.48629843918609,35.1054001133734));
#40777=CARTESIAN_POINT('Ctrl Pts',(0.152792920032838,4.57754672567843,35.1318574100579));
#40778=CARTESIAN_POINT('Ctrl Pts',(-0.591555496154874,4.47924365704371,
35.1583147067424));
#40779=CARTESIAN_POINT('Ctrl Pts',(-1.3359039123425,4.380940588409,35.1847720034269));
#40780=CARTESIAN_POINT('Ctrl Pts',(-2.05521905181772,4.09308616464727,35.2112293001113));
#40781=CARTESIAN_POINT('Ctrl Pts',(-2.66188912668102,3.65074073599519,35.2376865967958));
#40782=CARTESIAN_POINT('Ctrl Pts',(-3.26855920154439,3.20839530734307,35.2641438934803));
#40783=CARTESIAN_POINT('Ctrl Pts',(-3.76258421179579,2.61155887380058,35.2906011901647));
#40784=CARTESIAN_POINT('Ctrl Pts',(-4.08379245793952,1.93292545243568,35.3170584868492));
#40785=CARTESIAN_POINT('Ctrl Pts',(-4.40500070408323,1.25429203107082,35.3435157835337));
#40786=CARTESIAN_POINT('Ctrl Pts',(-4.55339218611928,0.493861621883449,
35.3699730802181));
#40787=CARTESIAN_POINT('Ctrl Pts',(-4.51089298576514,-0.255746192879281,
35.3964303769026));
#40788=CARTESIAN_POINT('Ctrl Pts',(-4.468393785411,-1.00535400764205,35.4228876735871));
#40789=CARTESIAN_POINT('Ctrl Pts',(-4.23500390266671,-1.74413922798016,
35.4493449702715));
#40790=CARTESIAN_POINT('Ctrl Pts',(-3.83914996695061,-2.38211863169333,
35.475802266956));
#40791=CARTESIAN_POINT('Ctrl Pts',(-3.44329603123454,-3.02009803540644,
35.5022595636405));
#40792=CARTESIAN_POINT('Ctrl Pts',(-2.88497804254663,-3.55727162249458,
35.5287168603249));
#40793=CARTESIAN_POINT('Ctrl Pts',(-2.23219851400125,-3.92821224455706,
35.5551741570094));
#40794=CARTESIAN_POINT('Ctrl Pts',(-1.57941898545579,-4.29915286661958,
35.5816314536939));
#40795=CARTESIAN_POINT('Ctrl Pts',(-0.83217791705278,-4.50386052365648,
35.6080887503783));
#40796=CARTESIAN_POINT('Ctrl Pts',(-0.081488443928666,-4.51740204959703,
35.6345460470628));
#40797=CARTESIAN_POINT('Ctrl Pts',(0.669201029195319,-4.53094357553758,
35.6610033437473));
#40798=CARTESIAN_POINT('Ctrl Pts',(1.42333890704038,-4.35331897038184,35.6874606404318));
#40799=CARTESIAN_POINT('Ctrl Pts',(2.08907203071298,-4.00616271445508,35.7139179371162));
#40800=CARTESIAN_POINT('Ctrl Pts',(2.75480515438577,-3.65900645852822,35.7403752338007));
#40801=CARTESIAN_POINT('Ctrl Pts',(3.33213352388603,-3.14231855183025,35.7668325304851));
#40802=CARTESIAN_POINT('Ctrl Pts',(3.75073918275594,-2.51903100956234,35.7932898271696));
#40803=CARTESIAN_POINT('Ctrl Pts',(4.16934484162576,-1.89574346729458,35.8197471238541));
#40804=CARTESIAN_POINT('Ctrl Pts',(4.42922778986531,-1.16585628945694,35.8462044205385));
#40805=CARTESIAN_POINT('Ctrl Pts',(4.49873457199958,-0.4182689265211,35.872661717223));
#40806=CARTESIAN_POINT('Ctrl Pts',(4.51165566030144,-0.279294828839705,
35.8775800439847));
#40807=CARTESIAN_POINT('Ctrl Pts',(4.51799780142692,-0.139709054890449,
35.8824983707463));
#40808=CARTESIAN_POINT('Ctrl Pts',(4.51785557016588,-0.000110407336722441,
35.887416697508));
#40809=CARTESIAN_POINT('Ctrl Pts',(4.51755220121239,0.000103541448102373,
35.6125833024919));
#40810=CARTESIAN_POINT('Ctrl Pts',(4.51712132198412,-0.510673802465055,
35.5945911163029));
#40811=CARTESIAN_POINT('Ctrl Pts',(4.43064412559555,-1.02159335775301,35.5765989301139));
#40812=CARTESIAN_POINT('Ctrl Pts',(4.26078183149926,-1.50309674624197,35.5586067439248));
#40813=CARTESIAN_POINT('Ctrl Pts',(4.01100133994626,-2.21114177590013,35.5321494472404));
#40814=CARTESIAN_POINT('Ctrl Pts',(3.58091429847129,-2.85557918629222,35.5056921505559));
#40815=CARTESIAN_POINT('Ctrl Pts',(3.02290483273525,-3.35791721405148,35.4792348538714));
#40816=CARTESIAN_POINT('Ctrl Pts',(2.46489536699924,-3.86025524181071,35.452777557187));
#40817=CARTESIAN_POINT('Ctrl Pts',(1.77896347700217,-4.22049388693713,35.4263202605025));
#40818=CARTESIAN_POINT('Ctrl Pts',(1.04865490780343,-4.39475648114172,35.399862963818));
#40819=CARTESIAN_POINT('Ctrl Pts',(0.318346338604615,-4.56901907534632,
35.3734056671336));
#40820=CARTESIAN_POINT('Ctrl Pts',(-0.456338909795902,-4.55730561862904,
35.3469483704491));
#40821=CARTESIAN_POINT('Ctrl Pts',(-1.18104503151125,-4.36104279705439,
35.3204910737646));
#40822=CARTESIAN_POINT('Ctrl Pts',(-1.9057511532266,-4.16477997547974,35.2940337770802));
#40823=CARTESIAN_POINT('Ctrl Pts',(-2.5804781482568,-3.78396778904771,35.2675764803957));
#40824=CARTESIAN_POINT('Ctrl Pts',(-3.1230450153486,-3.26498874060901,35.2411191837112));
#40825=CARTESIAN_POINT('Ctrl Pts',(-3.66561188244036,-2.74600969217034,
35.2146618870268));
#40826=CARTESIAN_POINT('Ctrl Pts',(-4.07601862159375,-2.08886378172499,
35.1882045903423));
#40827=CARTESIAN_POINT('Ctrl Pts',(-4.30427814618982,-1.37359065388133,
35.1617472936578));
#40828=CARTESIAN_POINT('Ctrl Pts',(-4.53253767078589,-0.658317526037631,
35.1352899969733));
#40829=CARTESIAN_POINT('Ctrl Pts',(-4.57864998082464,0.115082819204295,
35.1088327002889));
#40830=CARTESIAN_POINT('Ctrl Pts',(-4.43699864797729,0.852411075740494,
35.0823754036044));
#40831=CARTESIAN_POINT('Ctrl Pts',(-4.29534731512995,1.58973933227665,35.0559181069199));
#40832=CARTESIAN_POINT('Ctrl Pts',(-3.9659323393965,2.29099550010699,35.0294608102355));
#40833=CARTESIAN_POINT('Ctrl Pts',(-3.48887610024745,2.87076735409185,35.003003513551));
#40834=CARTESIAN_POINT('Ctrl Pts',(-3.0118198610984,3.45053920807671,34.9765462168666));
#40835=CARTESIAN_POINT('Ctrl Pts',(-2.38712235853373,3.90882674821612,34.9500889201821));
#40836=CARTESIAN_POINT('Ctrl Pts',(-1.69087105699361,4.18981105932221,34.9236316234976));
#40837=CARTESIAN_POINT('Ctrl Pts',(-0.994619755453442,4.47079537042831,
34.8971743268131));
#40838=CARTESIAN_POINT('Ctrl Pts',(-0.22681465493779,4.57447645250109,34.8707170301287));
#40839=CARTESIAN_POINT('Ctrl Pts',(0.519026433064394,4.48822606449116,34.8442597334442));
#40840=CARTESIAN_POINT('Ctrl Pts',(1.26486752106653,4.40197567648124,34.8178024367597));
#40841=CARTESIAN_POINT('Ctrl Pts',(1.98874459655524,4.12579381838863,34.7913451400753));
#40842=CARTESIAN_POINT('Ctrl Pts',(2.60249023287332,3.69331913486993,34.7648878433908));
#40843=CARTESIAN_POINT('Ctrl Pts',(3.2162358691914,3.26084445135124,34.7384305467063));
#40844=CARTESIAN_POINT('Ctrl Pts',(3.71985006633887,2.67207694240644,34.7119732500218));
#40845=CARTESIAN_POINT('Ctrl Pts',(4.05199317246873,1.99872783901765,34.6855159533374));
#40846=CARTESIAN_POINT('Ctrl Pts',(4.35719035466755,1.38000583275685,34.6612050697222));
#40847=CARTESIAN_POINT('Ctrl Pts',(4.51760990627478,0.689869322963186,34.6368941861071));
#40848=CARTESIAN_POINT('Ctrl Pts',(4.51806911322653,-6.09724841136444E-5,
34.6125833024919));
#40849=CARTESIAN_POINT('Origin',(0.,0.,20.5));
#40850=CARTESIAN_POINT('',(4.5173649459528,-1.24327273773317E-5,33.6125833024919));
#40851=CARTESIAN_POINT('',(4.51813527504661,9.51052893547258E-6,33.887416697508));
#40852=CARTESIAN_POINT('',(4.51775,5.53264807684796E-16,20.5));
#40853=CARTESIAN_POINT('Ctrl Pts',(4.51813527504661,9.51052893547258E-6,
33.887416697508));
#40854=CARTESIAN_POINT('Ctrl Pts',(4.51813637042829,0.00897485417732503,
33.8877326203013));
#40855=CARTESIAN_POINT('Ctrl Pts',(4.51811024333632,0.0179401914138076,
33.8880485430946));
#40856=CARTESIAN_POINT('Ctrl Pts',(4.51805685504966,0.0269053663078375,
33.8883644658879));
#40857=CARTESIAN_POINT('Ctrl Pts',(4.51358579512714,0.777703653204736,33.9148217625724));
#40858=CARTESIAN_POINT('Ctrl Pts',(4.31792089423795,1.52736336648647,33.9412790592569));
#40859=CARTESIAN_POINT('Ctrl Pts',(3.95489392076193,2.18457678274711,33.9677363559413));
#40860=CARTESIAN_POINT('Ctrl Pts',(3.59186694728593,2.84179019900772,33.9941936526258));
#40861=CARTESIAN_POINT('Ctrl Pts',(3.06147790122311,3.40655731824726,34.0206509493103));
#40862=CARTESIAN_POINT('Ctrl Pts',(2.42832758138582,3.81009013038776,34.0471082459947));
#40863=CARTESIAN_POINT('Ctrl Pts',(1.79517726154854,4.21362294252827,34.0735655426792));
#40864=CARTESIAN_POINT('Ctrl Pts',(1.05926566793676,4.45592144756974,34.1000228393637));
#40865=CARTESIAN_POINT('Ctrl Pts',(0.310226018196078,4.50747395575744,34.1264801360482));
#40866=CARTESIAN_POINT('Ctrl Pts',(-0.438813631544642,4.55902646394514,
34.1529374327326));
#40867=CARTESIAN_POINT('Ctrl Pts',(-1.20098133741429,4.41983297527906,34.1793947294171));
#40868=CARTESIAN_POINT('Ctrl Pts',(-1.8834459163527,4.10684710262894,34.2058520261016));
#40869=CARTESIAN_POINT('Ctrl Pts',(-2.56591049529112,3.79386122997882,34.232309322786));
#40870=CARTESIAN_POINT('Ctrl Pts',(-3.16867194729824,3.30708297334475,34.2587666194705));
#40871=CARTESIAN_POINT('Ctrl Pts',(-3.61831459461467,2.70580138565192,34.2852239161549));
#40872=CARTESIAN_POINT('Ctrl Pts',(-4.06795724193109,2.10451979795912,34.3116812128394));
#40873=CARTESIAN_POINT('Ctrl Pts',(-4.36448108455674,1.38873487920764,34.3381385095239));
#40874=CARTESIAN_POINT('Ctrl Pts',(-4.47176984663203,0.645628440319887,
34.3645958062084));
#40875=CARTESIAN_POINT('Ctrl Pts',(-4.57905860870732,-0.0974779985678242,
34.3910531028928));
#40876=CARTESIAN_POINT('Ctrl Pts',(-4.49711229023226,-0.86790595759181,
34.4175103995773));
#40877=CARTESIAN_POINT('Ctrl Pts',(-4.23591186210457,-1.57181816399963,
34.4439676962618));
#40878=CARTESIAN_POINT('Ctrl Pts',(-3.97471143397686,-2.27573037040753,
34.4704249929462));
#40879=CARTESIAN_POINT('Ctrl Pts',(-3.53425689619645,-2.91312682419928,
34.4968822896307));
#40880=CARTESIAN_POINT('Ctrl Pts',(-2.96819512400025,-3.40637334272956,
34.5233395863152));
#40881=CARTESIAN_POINT('Ctrl Pts',(-2.40213335180411,-3.89961986125978,
34.5497968829996));
#40882=CARTESIAN_POINT('Ctrl Pts',(-1.71046434519219,-4.24871644452859,
34.5762541796841));
#40883=CARTESIAN_POINT('Ctrl Pts',(-0.977432623678127,-4.41114351504993,
34.6027114763686));
#40884=CARTESIAN_POINT('Ctrl Pts',(-0.244400902164024,-4.57357058557128,
34.629168773053));
#40885=CARTESIAN_POINT('Ctrl Pts',(0.529993534252376,-4.54932814334514,
34.6556260697375));
#40886=CARTESIAN_POINT('Ctrl Pts',(1.25143030026179,-4.34136889100478,34.682083366422));
#40887=CARTESIAN_POINT('Ctrl Pts',(1.97286706627129,-4.13340963866439,34.7085406631064));
#40888=CARTESIAN_POINT('Ctrl Pts',(2.64134616187382,-3.74173357620983,34.7349979597909));
#40889=CARTESIAN_POINT('Ctrl Pts',(3.17544757305189,-3.21404641456781,34.7614552564754));
#40890=CARTESIAN_POINT('Ctrl Pts',(3.70954898422987,-2.68635925292589,34.7879125531598));
#40891=CARTESIAN_POINT('Ctrl Pts',(4.10927271098332,-2.0226609920966,34.8143698498443));
#40892=CARTESIAN_POINT('Ctrl Pts',(4.3259328457804,-1.30378934571338,34.8408271465288));
#40893=CARTESIAN_POINT('Ctrl Pts',(4.45310757210366,-0.881827525298336,
34.8563569968552));
#40894=CARTESIAN_POINT('Ctrl Pts',(4.51720899391685,-0.440856093465167,
34.8718868471816));
#40895=CARTESIAN_POINT('Ctrl Pts',(4.51740954388543,5.82741782004033E-5,
34.887416697508));
#40896=CARTESIAN_POINT('Ctrl Pts',(4.51806911322653,-6.09724841136444E-5,
34.6125833024919));
#40897=CARTESIAN_POINT('Ctrl Pts',(4.51810965670567,-0.0609750645635587,
34.6104368894226));
#40898=CARTESIAN_POINT('Ctrl Pts',(4.51690328345783,-0.121887549168861,
34.6082904763533));
#40899=CARTESIAN_POINT('Ctrl Pts',(4.51443954418555,-0.182749134310292,
34.606144063284));
#40900=CARTESIAN_POINT('Ctrl Pts',(4.48407079466025,-0.932946306416683,
34.5796867665996));
#40901=CARTESIAN_POINT('Ctrl Pts',(4.26266128049739,-1.67540995279661,34.5532294699151));
#40902=CARTESIAN_POINT('Ctrl Pts',(3.87717843548116,-2.3197088230287,34.5267721732306));
#40903=CARTESIAN_POINT('Ctrl Pts',(3.49169559046496,-2.96400769326076,34.5003148765461));
#40904=CARTESIAN_POINT('Ctrl Pts',(2.94213941459544,-3.51014178734499,34.4738575798616));
#40905=CARTESIAN_POINT('Ctrl Pts',(2.2954452418825,-3.8915925770456,34.4474002831772));
#40906=CARTESIAN_POINT('Ctrl Pts',(1.64875106916955,-4.2730433667462,34.4209429864927));
#40907=CARTESIAN_POINT('Ctrl Pts',(0.904918899613214,-4.48981085206318,
34.3944856898083));
#40908=CARTESIAN_POINT('Ctrl Pts',(0.154546668243127,-4.51549299318827,
34.3680283931238));
#40909=CARTESIAN_POINT('Ctrl Pts',(-0.595825563126962,-4.54117513431336,
34.3415710964393));
#40910=CARTESIAN_POINT('Ctrl Pts',(-1.35273785631077,-4.37577193124655,
34.3151137997548));
#40911=CARTESIAN_POINT('Ctrl Pts',(-2.02399913169702,-4.03942931106451,
34.2886565030704));
#40912=CARTESIAN_POINT('Ctrl Pts',(-2.69526040708323,-3.70308669088248,
34.2621992063859));
#40913=CARTESIAN_POINT('Ctrl Pts',(-3.28087066467185,-3.19580465358524,
34.2357419097014));
#40914=CARTESIAN_POINT('Ctrl Pts',(-3.7095032232018,-2.57936958989069,34.209284613017));
#40915=CARTESIAN_POINT('Ctrl Pts',(-4.13813578173176,-1.9629345261961,34.1828273163325));
#40916=CARTESIAN_POINT('Ctrl Pts',(-4.40979064120305,-1.23734643610409,
34.1563700196481));
#40917=CARTESIAN_POINT('Ctrl Pts',(-4.49138054038088,-0.490981145957072,
34.1299127229636));
#40918=CARTESIAN_POINT('Ctrl Pts',(-4.57297043955872,0.255384144190028,
34.1034554262791));
#40919=CARTESIAN_POINT('Ctrl Pts',(-4.46449537844313,1.02252663439224,34.0769981295946));
#40920=CARTESIAN_POINT('Ctrl Pts',(-4.17916749942524,1.71700921836348,34.0505408329102));
#40921=CARTESIAN_POINT('Ctrl Pts',(-3.89383962040737,2.41149180233465,34.0240835362257));
#40922=CARTESIAN_POINT('Ctrl Pts',(-3.43165892348727,3.03331448007484,33.9976262395413));
#40923=CARTESIAN_POINT('Ctrl Pts',(-2.84891850603996,3.50673993762589,33.9711689428568));
#40924=CARTESIAN_POINT('Ctrl Pts',(-2.26617808859268,3.98016539517692,33.9447116461723));
#40925=CARTESIAN_POINT('Ctrl Pts',(-1.56287795061823,4.30519363253881,33.9182543494878));
#40926=CARTESIAN_POINT('Ctrl Pts',(-0.824679270557638,4.44223657011982,
33.8917970528033));
#40927=CARTESIAN_POINT('Ctrl Pts',(-0.0864805904969625,4.57927950770084,
33.8653397561189));
#40928=CARTESIAN_POINT('Ctrl Pts',(0.686616631649836,4.52833714550091,33.8388824594344));
#40929=CARTESIAN_POINT('Ctrl Pts',(1.40045000983613,4.2956142068565,33.81242516275));
#40930=CARTESIAN_POINT('Ctrl Pts',(2.11428338802235,4.0628912682121,33.7859678660655));
#40931=CARTESIAN_POINT('Ctrl Pts',(2.76885292224806,3.64838775312326,33.759510569381));
#40932=CARTESIAN_POINT('Ctrl Pts',(3.28443276767714,3.10258973098379,33.7330532726965));
#40933=CARTESIAN_POINT('Ctrl Pts',(3.80001261310627,2.55679170884426,33.7065959760121));
#40934=CARTESIAN_POINT('Ctrl Pts',(4.17660276973874,1.87969917965409,33.6801386793276));
#40935=CARTESIAN_POINT('Ctrl Pts',(4.36833497328078,1.15378126410918,33.6536813826432));
#40936=CARTESIAN_POINT('Ctrl Pts',(4.46761225473945,0.777907227895749,33.6399820225928));
#40937=CARTESIAN_POINT('Ctrl Pts',(4.51732765695876,0.388942719447438,33.6262826625424));
#40938=CARTESIAN_POINT('Ctrl Pts',(4.5173649459528,-1.24327273773317E-5,
33.6125833024919));
#40939=CARTESIAN_POINT('Origin',(0.,0.,20.5));
#40940=CARTESIAN_POINT('',(4.51800690475437,8.25810157162321E-5,32.6125833024919));
#40941=CARTESIAN_POINT('',(4.5174378855045,-7.22228901865168E-5,32.887416697508));
#40942=CARTESIAN_POINT('',(4.51775,5.53264807684796E-16,20.5));
#40943=CARTESIAN_POINT('Ctrl Pts',(4.5174378855045,-7.22228901865168E-5,
32.887416697508));
#40944=CARTESIAN_POINT('Ctrl Pts',(4.51717714450692,0.458772891828189,32.9035783934211));
#40945=CARTESIAN_POINT('Ctrl Pts',(4.44766773093088,0.917695233524441,32.9197400893341));
#40946=CARTESIAN_POINT('Ctrl Pts',(4.31009826091021,1.35521755651858,32.9359017852471));
#40947=CARTESIAN_POINT('Ctrl Pts',(4.08489192720295,2.07145785505129,32.9623590819316));
#40948=CARTESIAN_POINT('Ctrl Pts',(3.67729208498414,2.73034844367792,32.988816378616));
#40949=CARTESIAN_POINT('Ctrl Pts',(3.13694394393257,3.25163717791855,33.0152736753005));
#40950=CARTESIAN_POINT('Ctrl Pts',(2.596595802881,3.77292591215919,33.0417309719849));
#40951=CARTESIAN_POINT('Ctrl Pts',(1.92349936299679,4.15661279201376,33.0681882686694));
#40952=CARTESIAN_POINT('Ctrl Pts',(1.19963702572075,4.35596518015436,33.0946455653539));
#40953=CARTESIAN_POINT('Ctrl Pts',(0.475774688444753,4.55531756829496,33.1211028620384));
#40954=CARTESIAN_POINT('Ctrl Pts',(-0.298853546223071,4.57033546472152,
33.1475601587228));
#40955=CARTESIAN_POINT('Ctrl Pts',(-1.02989881660521,4.39918970627007,33.1740174554073));
#40956=CARTESIAN_POINT('Ctrl Pts',(-1.76094408698744,4.2280439478186,33.2004747520918));
#40957=CARTESIAN_POINT('Ctrl Pts',(-2.4484063930841,3.87073453448909,33.2269320487762));
#40958=CARTESIAN_POINT('Ctrl Pts',(-3.00855358684862,3.37078135737958,33.2533893454607));
#40959=CARTESIAN_POINT('Ctrl Pts',(-3.56870078061313,2.87082818027007,33.2798466421452));
#40960=CARTESIAN_POINT('Ctrl Pts',(-4.0015328620455,2.22823123938057,33.3063039388296));
#40961=CARTESIAN_POINT('Ctrl Pts',(-4.25433136265604,1.52125813092933,33.3327612355141));
#40962=CARTESIAN_POINT('Ctrl Pts',(-4.50712986326656,0.814285022478126,
33.3592185321986));
#40963=CARTESIAN_POINT('Ctrl Pts',(-4.57989478305528,0.0429357464651833,
33.3856758288831));
#40964=CARTESIAN_POINT('Ctrl Pts',(-4.46376343532313,-0.698840208967454,
33.4121331255675));
#40965=CARTESIAN_POINT('Ctrl Pts',(-4.34763208759097,-1.44061616440009,
33.438590422252));
#40966=CARTESIAN_POINT('Ctrl Pts',(-4.04260447233795,-2.15281879925242,
33.4650477189364));
#40967=CARTESIAN_POINT('Ctrl Pts',(-3.5858326155183,-2.74870262081633,33.4915050156209));
#40968=CARTESIAN_POINT('Ctrl Pts',(-3.12906075869862,-3.34458644238028,
33.5179623123054));
#40969=CARTESIAN_POINT('Ctrl Pts',(-2.52054466031228,-3.82415145065579,
33.5444196089899));
#40970=CARTESIAN_POINT('Ctrl Pts',(-1.83440090767899,-4.12898715838447,
33.5708769056743));
#40971=CARTESIAN_POINT('Ctrl Pts',(-1.14825715504573,-4.43382286611314,
33.5973342023588));
#40972=CARTESIAN_POINT('Ctrl Pts',(-0.384485748165517,-4.56392927329501,
33.6237914990433));
#40973=CARTESIAN_POINT('Ctrl Pts',(0.363886800893304,-4.50345956352814,
33.6502487957277));
#40974=CARTESIAN_POINT('Ctrl Pts',(1.11225934995217,-4.44298985376126,33.6767060924122));
#40975=CARTESIAN_POINT('Ctrl Pts',(1.84523304118964,-4.19194402704563,33.7031633890966));
#40976=CARTESIAN_POINT('Ctrl Pts',(2.47353249021786,-3.78089918723496,33.7296206857811));
#40977=CARTESIAN_POINT('Ctrl Pts',(3.10183193924602,-3.36985434742433,33.7560779824656));
#40978=CARTESIAN_POINT('Ctrl Pts',(3.62545714606495,-2.7988104945187,33.7825352791501));
#40979=CARTESIAN_POINT('Ctrl Pts',(3.98063113999648,-2.1373201378099,33.8089925758346));
#40980=CARTESIAN_POINT('Ctrl Pts',(4.3315640520969,-1.48372854278193,33.8351339497257));
#40981=CARTESIAN_POINT('Ctrl Pts',(4.51804463650222,-0.741837565236255,
33.8612753236169));
#40982=CARTESIAN_POINT('Ctrl Pts',(4.51813527504661,9.51052893547258E-6,
33.887416697508));
#40983=CARTESIAN_POINT('Ctrl Pts',(4.5173649459528,-1.24327273773317E-5,
33.6125833024919));
#40984=CARTESIAN_POINT('Ctrl Pts',(4.51739967243793,-0.362238490490815,
33.5998253658579));
#40985=CARTESIAN_POINT('Ctrl Pts',(4.47434946667155,-0.724456433726874,
33.5870674292238));
#40986=CARTESIAN_POINT('Ctrl Pts',(4.38812044853862,-1.07608576485082,33.5743094925897));
#40987=CARTESIAN_POINT('Ctrl Pts',(4.20929946980279,-1.80529157636637,33.5478521959053));
#40988=CARTESIAN_POINT('Ctrl Pts',(3.84478326187951,-2.48895989749788,33.5213948992208));
#40989=CARTESIAN_POINT('Ctrl Pts',(3.33896949547234,-3.04382068336861,33.4949376025364));
#40990=CARTESIAN_POINT('Ctrl Pts',(2.83315572906515,-3.59868146923937,33.4684803058519));
#40991=CARTESIAN_POINT('Ctrl Pts',(2.18604440417407,-4.02473471984934,33.4420230091674));
#40992=CARTESIAN_POINT('Ctrl Pts',(1.47645296399252,-4.27008762080067,33.4155657124829));
#40993=CARTESIAN_POINT('Ctrl Pts',(0.766861523811012,-4.51544052175197,
33.3891084157985));
#40994=CARTESIAN_POINT('Ctrl Pts',(-0.00521003166095199,-4.58009307304465,
33.362651119114));
#40995=CARTESIAN_POINT('Ctrl Pts',(-0.745724241442587,-4.45617066548424,
33.3361938224295));
#40996=CARTESIAN_POINT('Ctrl Pts',(-1.48623845122422,-4.33224825792383,
33.3097365257451));
#40997=CARTESIAN_POINT('Ctrl Pts',(-2.19519531531565,-4.01975089151028,
33.2832792290606));
#40998=CARTESIAN_POINT('Ctrl Pts',(-2.78624467229499,-3.55674039962226,
33.2568219323761));
#40999=CARTESIAN_POINT('Ctrl Pts',(-3.37729402927434,-3.09372990773425,
33.2303646356917));
#41000=CARTESIAN_POINT('Ctrl Pts',(-3.85043587914167,-2.48020629037183,
33.2039073390072));
#41001=CARTESIAN_POINT('Ctrl Pts',(-4.14804206822415,-1.7908960451238,33.1774500423227));
#41002=CARTESIAN_POINT('Ctrl Pts',(-4.44564825730663,-1.10158579987578,
33.1509927456383));
#41003=CARTESIAN_POINT('Ctrl Pts',(-4.56771878560417,-0.33648892674225,
33.1245354489538));
#41004=CARTESIAN_POINT('Ctrl Pts',(-4.49938559786941,0.411206621885727,
33.0980781522693));
#41005=CARTESIAN_POINT('Ctrl Pts',(-4.43105241013465,1.15890217051366,33.0716208555848));
#41006=CARTESIAN_POINT('Ctrl Pts',(-4.17231550636761,1.88919639463604,33.0451635589004));
#41007=CARTESIAN_POINT('Ctrl Pts',(-3.75468875509488,2.51314026599421,33.0187062622159));
#41008=CARTESIAN_POINT('Ctrl Pts',(-3.33706200382211,3.13708413735244,32.9922489655315));
#41009=CARTESIAN_POINT('Ctrl Pts',(-2.76054540504362,3.65467765594643,32.965791668847));
#41010=CARTESIAN_POINT('Ctrl Pts',(-2.09535804244172,4.00287850404833,32.9393343721625));
#41011=CARTESIAN_POINT('Ctrl Pts',(-1.43017067983982,4.35107935215023,32.912877075478));
#41012=CARTESIAN_POINT('Ctrl Pts',(-0.676312553414512,4.52988752976003,
32.8864197787936));
#41013=CARTESIAN_POINT('Ctrl Pts',(0.0743972513539278,4.51752439873747,
32.8599624821091));
#41014=CARTESIAN_POINT('Ctrl Pts',(0.825107056122282,4.50516126771491,32.8335051854247));
#41015=CARTESIAN_POINT('Ctrl Pts',(1.57266853923377,4.30162682806002,32.8070478887402));
#41016=CARTESIAN_POINT('Ctrl Pts',(2.22602953939506,3.93171134926485,32.7805905920557));
#41017=CARTESIAN_POINT('Ctrl Pts',(2.87939053955642,3.56179587046963,32.7541332953712));
#41018=CARTESIAN_POINT('Ctrl Pts',(3.43855105676757,3.02549935253409,32.7276759986868));
#41019=CARTESIAN_POINT('Ctrl Pts',(3.83540595887257,2.38814211780667,32.7012187020023));
#41020=CARTESIAN_POINT('Ctrl Pts',(4.23226086097758,1.75078488307926,32.6747614053179));
#41021=CARTESIAN_POINT('Ctrl Pts',(4.46681014797645,1.01236693155997,32.6483041086334));
#41022=CARTESIAN_POINT('Ctrl Pts',(4.51048597629574,0.262826752513661,32.6218468119489));
#41023=CARTESIAN_POINT('Ctrl Pts',(4.51558339111607,0.175347765528612,32.6187589754633));
#41024=CARTESIAN_POINT('Ctrl Pts',(4.51808086670496,0.0877172796610649,
32.6156711389776));
#41025=CARTESIAN_POINT('Ctrl Pts',(4.51800690475437,8.25810157162321E-5,
32.6125833024919));
#41026=CARTESIAN_POINT('Origin',(0.,0.,20.5));
#41027=CARTESIAN_POINT('',(4.51762600826661,-0.000112987348963034,31.612583302492));
#41028=CARTESIAN_POINT('',(4.51779894817057,0.000115094980599771,31.887416697508));
#41029=CARTESIAN_POINT('',(4.51775,5.53264807684796E-16,20.5));
#41030=CARTESIAN_POINT('Ctrl Pts',(4.51779894817057,0.000115094980599771,
31.887416697508));
#41031=CARTESIAN_POINT('Ctrl Pts',(4.51796156278444,0.157653334629133,31.8929668698563));
#41032=CARTESIAN_POINT('Ctrl Pts',(4.50988180917274,0.315174976505045,31.8985170422046));
#41033=CARTESIAN_POINT('Ctrl Pts',(4.49343403803756,0.471817962781026,31.9040672145528));
#41034=CARTESIAN_POINT('Ctrl Pts',(4.41502862404034,1.21852449753214,31.9305245112373));
#41035=CARTESIAN_POINT('Ctrl Pts',(4.14647135042176,1.94526477434642,31.9569818079218));
#41036=CARTESIAN_POINT('Ctrl Pts',(3.72047219588784,2.56352263181406,31.9834391046062));
#41037=CARTESIAN_POINT('Ctrl Pts',(3.29447304135392,3.1817804892817,32.0098964012907));
#41038=CARTESIAN_POINT('Ctrl Pts',(2.71103200590467,3.69155592740269,32.0363536979752));
#41039=CARTESIAN_POINT('Ctrl Pts',(2.04121156194539,4.0307588619983,32.0628109946597));
#41040=CARTESIAN_POINT('Ctrl Pts',(1.37139111798607,4.36996179659393,32.0892682913441));
#41041=CARTESIAN_POINT('Ctrl Pts',(0.615191265516699,4.53859222766416,32.1157255880286));
#41042=CARTESIAN_POINT('Ctrl Pts',(-0.135283690341923,4.51611115533319,
32.1421828847131));
#41043=CARTESIAN_POINT('Ctrl Pts',(-0.885758646200546,4.49363008300222,
32.1686401813975));
#41044=CARTESIAN_POINT('Ctrl Pts',(-1.63050870544842,4.28003750727005,32.195097478082));
#41045=CARTESIAN_POINT('Ctrl Pts',(-2.27882413510731,3.9013487674713,32.2215547747665));
#41046=CARTESIAN_POINT('Ctrl Pts',(-2.92713956476612,3.52266002767259,32.2480120714509));
#41047=CARTESIAN_POINT('Ctrl Pts',(-3.47902036483595,2.97887512380733,32.2744693681354));
#41048=CARTESIAN_POINT('Ctrl Pts',(-3.86724806465204,2.33622645534256,32.3009266648198));
#41049=CARTESIAN_POINT('Ctrl Pts',(-4.25547576446814,1.69357778687776,32.3273839615043));
#41050=CARTESIAN_POINT('Ctrl Pts',(-4.48005036403047,0.952065353813438,
32.3538412581888));
#41051=CARTESIAN_POINT('Ctrl Pts',(-4.51361892565606,0.202004549841869,
32.3802985548733));
#41052=CARTESIAN_POINT('Ctrl Pts',(-4.54718748728165,-0.548056254129699,
32.4067558515577));
#41053=CARTESIAN_POINT('Ctrl Pts',(-4.38975001097049,-1.30666542900852,
32.4332131482422));
#41054=CARTESIAN_POINT('Ctrl Pts',(-4.06048220709632,-1.98142521687081,
32.4596704449267));
#41055=CARTESIAN_POINT('Ctrl Pts',(-3.73121440322213,-2.65618500473315,
32.4861277416111));
#41056=CARTESIAN_POINT('Ctrl Pts',(-3.23011627178491,-3.24709540557894,
32.5125850382956));
#41057=CARTESIAN_POINT('Ctrl Pts',(-2.61822101061276,-3.68218418656418,
32.5390423349801));
#41058=CARTESIAN_POINT('Ctrl Pts',(-2.00632574944065,-4.11727296754938,
32.5654996316645));
#41059=CARTESIAN_POINT('Ctrl Pts',(-1.28363335853361,-4.39654012867405,
32.591956928349));
#41060=CARTESIAN_POINT('Ctrl Pts',(-0.538166971277905,-4.48597123878686,
32.6184142250335));
#41061=CARTESIAN_POINT('Ctrl Pts',(0.207299415977802,-4.57540234889968,
32.6448715217179));
#41062=CARTESIAN_POINT('Ctrl Pts',(0.975539799582185,-4.47499740800066,
32.6713288184024));
#41063=CARTESIAN_POINT('Ctrl Pts',(1.67298335104786,-4.19698562677001,32.6977861150869));
#41064=CARTESIAN_POINT('Ctrl Pts',(2.37042690251357,-3.91897384553935,32.7242434117713));
#41065=CARTESIAN_POINT('Ctrl Pts',(2.99707362184056,-3.46335522397704,32.7507007084558));
#41066=CARTESIAN_POINT('Ctrl Pts',(3.47659863214429,-2.88562360594202,32.7771580051403));
#41067=CARTESIAN_POINT('Ctrl Pts',(3.95612364244802,-2.30789198790701,32.8036153018248));
#41068=CARTESIAN_POINT('Ctrl Pts',(4.28852694372849,-1.60804737339928,32.8300725985092));
#41069=CARTESIAN_POINT('Ctrl Pts',(4.43332218177084,-0.871330061926005,
32.8565298951937));
#41070=CARTESIAN_POINT('Ctrl Pts',(4.48966784634383,-0.584643655117203,
32.8668254959651));
#41071=CARTESIAN_POINT('Ctrl Pts',(4.51760398720758,-0.292373608988289,
32.8771210967366));
#41072=CARTESIAN_POINT('Ctrl Pts',(4.5174378855045,-7.22228901865168E-5,
32.887416697508));
#41073=CARTESIAN_POINT('Ctrl Pts',(4.51800690475437,8.25810157162321E-5,
32.6125833024919));
#41074=CARTESIAN_POINT('Ctrl Pts',(4.51744714361788,-0.663157072879468,
32.5892138422931));
#41075=CARTESIAN_POINT('Ctrl Pts',(4.36960026846028,-1.32663802677704,32.5658443820943));
#41076=CARTESIAN_POINT('Ctrl Pts',(4.08682159368458,-1.92651262793442,32.5424749218955));
#41077=CARTESIAN_POINT('Ctrl Pts',(3.76667901311444,-2.60564942276291,32.516017625211));
#41078=CARTESIAN_POINT('Ctrl Pts',(3.27359148233441,-3.20326060584664,32.4895603285266));
#41079=CARTESIAN_POINT('Ctrl Pts',(2.66761651687815,-3.64655779648099,32.4631030318421));
#41080=CARTESIAN_POINT('Ctrl Pts',(2.06164155142182,-4.08985498711538,32.4366457351576));
#41081=CARTESIAN_POINT('Ctrl Pts',(1.34277915128922,-4.37883818530036,32.4101884384731));
#41082=CARTESIAN_POINT('Ctrl Pts',(0.598585961229044,-4.47830955732371,
32.3837311417887));
#41083=CARTESIAN_POINT('Ctrl Pts',(-0.14560722883109,-4.57778092934705,
32.3572738451042));
#41084=CARTESIAN_POINT('Ctrl Pts',(-0.915131208818801,-4.4877404752088,
32.3308165484198));
#41085=CARTESIAN_POINT('Ctrl Pts',(-1.6162588096278,-4.2191550225724,32.3043592517353));
#41086=CARTESIAN_POINT('Ctrl Pts',(-2.31738641043684,-3.95056956993598,
32.2779019550508));
#41087=CARTESIAN_POINT('Ctrl Pts',(-2.95011763206717,-3.5034391188014,32.2514446583663));
#41088=CARTESIAN_POINT('Ctrl Pts',(-3.4373865119876,-2.93222366326361,32.2249873616819));
#41089=CARTESIAN_POINT('Ctrl Pts',(-3.924655391908,-2.36100820772586,32.1985300649974));
#41090=CARTESIAN_POINT('Ctrl Pts',(-4.26646193011853,-1.66570774778492,
32.172072768313));
#41091=CARTESIAN_POINT('Ctrl Pts',(-4.42117446855311,-0.931009109950869,
32.1456154716285));
#41092=CARTESIAN_POINT('Ctrl Pts',(-4.57588700698769,-0.196310472116814,
32.119158174944));
#41093=CARTESIAN_POINT('Ctrl Pts',(-4.54350554564632,0.577786343610359,
32.0927008782595));
#41094=CARTESIAN_POINT('Ctrl Pts',(-4.3279741106828,1.2969972017922,32.0662435815751));
#41095=CARTESIAN_POINT('Ctrl Pts',(-4.11244267571929,2.01620805997403,32.0397862848906));
#41096=CARTESIAN_POINT('Ctrl Pts',(-3.71376126713363,2.68053296061054,32.0133289882062));
#41097=CARTESIAN_POINT('Ctrl Pts',(-3.18048883925839,3.2090578660333,31.9868716915217));
#41098=CARTESIAN_POINT('Ctrl Pts',(-2.64721641138316,3.73758277145606,31.9604143948372));
#41099=CARTESIAN_POINT('Ctrl Pts',(-1.97935296421834,4.13030768166508,31.9339570981527));
#41100=CARTESIAN_POINT('Ctrl Pts',(-1.25824352648329,4.33939913723781,31.9074998014683));
#41101=CARTESIAN_POINT('Ctrl Pts',(-0.537134088748201,4.54849059281056,
31.8810425047838));
#41102=CARTESIAN_POINT('Ctrl Pts',(0.237221339557133,4.57394859374701,31.8545852080993));
#41103=CARTESIAN_POINT('Ctrl Pts',(0.970507124268449,4.41267238370826,31.8281279114149));
#41104=CARTESIAN_POINT('Ctrl Pts',(1.70379290897972,4.25139617366952,31.8016706147304));
#41105=CARTESIAN_POINT('Ctrl Pts',(2.39600905009698,3.90338575265561,31.7752133180459));
#41106=CARTESIAN_POINT('Ctrl Pts',(2.96284438772936,3.41102840479202,31.7487560213615));
#41107=CARTESIAN_POINT('Ctrl Pts',(3.52967972536174,2.91867105692843,31.722298724677));
#41108=CARTESIAN_POINT('Ctrl Pts',(3.97113425950925,2.28196678221515,31.6958414279925));
#41109=CARTESIAN_POINT('Ctrl Pts',(4.23343931648423,1.57846545665177,31.669384131308));
#41110=CARTESIAN_POINT('Ctrl Pts',(4.42115243039411,1.07501948430126,31.6504505217027));
#41111=CARTESIAN_POINT('Ctrl Pts',(4.5171186342718,0.537365078236716,31.6315169120973));
#41112=CARTESIAN_POINT('Ctrl Pts',(4.51762600826661,-0.000112987348963034,
31.612583302492));
#41113=CARTESIAN_POINT('Origin',(0.,0.,20.5));
#41114=CARTESIAN_POINT('',(4.5175628644093,0.000105298910395568,30.612583302492));
#41115=CARTESIAN_POINT('',(4.51784283093286,-0.000111697445491984,30.8874166975081));
#41116=CARTESIAN_POINT('',(4.51775,5.53264807684796E-16,20.5));
#41117=CARTESIAN_POINT('Ctrl Pts',(4.51784283093286,-0.000111697445491984,
30.8874166975081));
#41118=CARTESIAN_POINT('Ctrl Pts',(4.51722105684837,0.607182099716009,30.908812642976));
#41119=CARTESIAN_POINT('Ctrl Pts',(4.39393696701912,1.21472067967305,30.930208588444));
#41120=CARTESIAN_POINT('Ctrl Pts',(4.15564368858641,1.77318560159654,30.951604533912));
#41121=CARTESIAN_POINT('Ctrl Pts',(3.86098057239723,2.46375906325124,30.9780618305965));
#41122=CARTESIAN_POINT('Ctrl Pts',(3.3904601122214,3.07929536251675,31.0045191272809));
#41123=CARTESIAN_POINT('Ctrl Pts',(2.80139117936865,3.54482285937575,31.0309764239654));
#41124=CARTESIAN_POINT('Ctrl Pts',(2.21232224651588,4.01035035623478,31.0574337206499));
#41125=CARTESIAN_POINT('Ctrl Pts',(1.50470484098616,4.32586905068731,31.0838910173343));
#41126=CARTESIAN_POINT('Ctrl Pts',(0.764725979630773,4.45294911494339,31.1103483140188));
#41127=CARTESIAN_POINT('Ctrl Pts',(0.0247471182753856,4.58002917919947,
31.1368056107033));
#41128=CARTESIAN_POINT('Ctrl Pts',(-0.747593198905696,4.51867061325911,
31.1632629073878));
#41129=CARTESIAN_POINT('Ctrl Pts',(-1.45822477605293,4.27634682254641,31.1897202040722));
#41130=CARTESIAN_POINT('Ctrl Pts',(-2.16885635320013,4.03402303183372,31.2161775007567));
#41131=CARTESIAN_POINT('Ctrl Pts',(-2.81777919031341,3.61073401634878,31.2426347974411));
#41132=CARTESIAN_POINT('Ctrl Pts',(-3.32595520401574,3.05803590971036,31.2690920941256));
#41133=CARTESIAN_POINT('Ctrl Pts',(-3.83413121771806,2.50533780307193,31.2955493908101));
#41134=CARTESIAN_POINT('Ctrl Pts',(-4.20156040800938,1.82323060527995,31.3220066874946));
#41135=CARTESIAN_POINT('Ctrl Pts',(-4.38349030615745,1.09479421811638,31.348463984179));
#41136=CARTESIAN_POINT('Ctrl Pts',(-4.56542020430551,0.366357830952816,
31.3749212808635));
#41137=CARTESIAN_POINT('Ctrl Pts',(-4.56185081031042,-0.408407745582352,
31.4013785775479));
#41138=CARTESIAN_POINT('Ctrl Pts',(-4.3732168724104,-1.13513692172461,31.4278358742324));
#41139=CARTESIAN_POINT('Ctrl Pts',(-4.18458293451036,-1.86186609786691,
31.4542931709169));
#41140=CARTESIAN_POINT('Ctrl Pts',(-3.81088445270536,-2.54055887361621,
31.4807504676013));
#41141=CARTESIAN_POINT('Ctrl Pts',(-3.29763748849549,-3.08855122001668,
31.5072077642858));
#41142=CARTESIAN_POINT('Ctrl Pts',(-2.78439052428562,-3.63654356641715,
31.5336650609703));
#41143=CARTESIAN_POINT('Ctrl Pts',(-2.13159507767086,-4.05383548346882,
31.5601223576548));
#41144=CARTESIAN_POINT('Ctrl Pts',(-1.4187609115798,-4.28960127750478,31.5865796543392));
#41145=CARTESIAN_POINT('Ctrl Pts',(-0.705926745488817,-4.52536707154071,
31.6130369510237));
#41146=CARTESIAN_POINT('Ctrl Pts',(0.0669461400784679,-4.57960674256098,
31.6394942477081));
#41147=CARTESIAN_POINT('Ctrl Pts',(0.805722683022508,-4.44571395866405,
31.6659515443926));
#41148=CARTESIAN_POINT('Ctrl Pts',(1.54449922596663,-4.31182117476711,31.6924088410771));
#41149=CARTESIAN_POINT('Ctrl Pts',(2.24917942628753,-3.98979593595292,31.7188661377616));
#41150=CARTESIAN_POINT('Ctrl Pts',(2.83393401547767,-3.51886055991368,31.745323434446));
#41151=CARTESIAN_POINT('Ctrl Pts',(3.41868860466777,-3.04792518387447,31.7717807311305));
#41152=CARTESIAN_POINT('Ctrl Pts',(3.88351758272714,-2.42807967061021,31.798238027815));
#41153=CARTESIAN_POINT('Ctrl Pts',(4.1718052945689,-1.73482051763412,31.8246953244994));
#41154=CARTESIAN_POINT('Ctrl Pts',(4.39961643899369,-1.18699223867807,31.8456024488356));
#41155=CARTESIAN_POINT('Ctrl Pts',(4.51718638990429,-0.593320812476893,
31.8665095731718));
#41156=CARTESIAN_POINT('Ctrl Pts',(4.51779894817057,0.000115094980599771,
31.887416697508));
#41157=CARTESIAN_POINT('Ctrl Pts',(4.51762600826661,-0.000112987348963034,
31.612583302492));
#41158=CARTESIAN_POINT('Ctrl Pts',(4.51782762450612,-0.213691742886314,
31.6050596154129));
#41159=CARTESIAN_POINT('Ctrl Pts',(4.50295585827573,-0.42724265346175,31.5975359283338));
#41160=CARTESIAN_POINT('Ctrl Pts',(4.47277779830256,-0.638608182854815,
31.5900122412547));
#41161=CARTESIAN_POINT('Ctrl Pts',(4.36665564334343,-1.38188212038452,31.5635549445702));
#41162=CARTESIAN_POINT('Ctrl Pts',(4.07125575362272,-2.09813161903045,31.5370976478857));
#41163=CARTESIAN_POINT('Ctrl Pts',(3.62255750878013,-2.70011828255321,31.5106403512012));
#41164=CARTESIAN_POINT('Ctrl Pts',(3.17385926393751,-3.302104946076,31.4841830545168));
#41165=CARTESIAN_POINT('Ctrl Pts',(2.57186266397298,-3.78982877447561,31.4577257578323));
#41166=CARTESIAN_POINT('Ctrl Pts',(1.88989022851381,-4.10388554523215,31.4312684611479));
#41167=CARTESIAN_POINT('Ctrl Pts',(1.20791779305463,-4.4179423159887,31.4048111644634));
#41168=CARTESIAN_POINT('Ctrl Pts',(0.44596952210079,-4.55833202910217,31.3783538677789));
#41169=CARTESIAN_POINT('Ctrl Pts',(-0.303150128217454,-4.50795537288904,
31.3518965710945));
#41170=CARTESIAN_POINT('Ctrl Pts',(-1.05226977853561,-4.45757871667591,
31.32543927441));
#41171=CARTESIAN_POINT('Ctrl Pts',(-1.7885608082182,-4.2164356911362,31.2989819777255));
#41172=CARTESIAN_POINT('Ctrl Pts',(-2.42234378472615,-3.81389724990016,
31.272524681041));
#41173=CARTESIAN_POINT('Ctrl Pts',(-3.05612676123416,-3.41135880866406,
31.2460673843566));
#41174=CARTESIAN_POINT('Ctrl Pts',(-3.58740168456753,-2.84742495173157,
31.2196100876721));
#41175=CARTESIAN_POINT('Ctrl Pts',(-3.95145985704278,-2.19078219875388,
31.1931527909876));
#41176=CARTESIAN_POINT('Ctrl Pts',(-4.31551802951802,-1.53413944577618,
31.1666954943032));
#41177=CARTESIAN_POINT('Ctrl Pts',(-4.51235945113515,-0.784787796753247,
31.1402381976187));
#41178=CARTESIAN_POINT('Ctrl Pts',(-4.51800905459174,-0.0339974532052471,
31.1137809009342));
#41179=CARTESIAN_POINT('Ctrl Pts',(-4.52365865804833,0.716792890342667,
31.0873236042498));
#41180=CARTESIAN_POINT('Ctrl Pts',(-4.33811644334446,1.46902192841556,31.0608663075653));
#41181=CARTESIAN_POINT('Ctrl Pts',(-3.98398124688566,2.13106899669175,31.0344090108808));
#41182=CARTESIAN_POINT('Ctrl Pts',(-3.62984605042683,2.79311606496798,31.0079517141964));
#41183=CARTESIAN_POINT('Ctrl Pts',(-3.10711787221305,3.36498116344739,30.9814944175119));
#41184=CARTESIAN_POINT('Ctrl Pts',(-2.47946442583117,3.77701175603613,30.9550371208274));
#41185=CARTESIAN_POINT('Ctrl Pts',(-1.85181097944929,4.18904234862487,30.928579824143));
#41186=CARTESIAN_POINT('Ctrl Pts',(-1.11923226489916,4.44123843532298,30.9021225274585));
#41187=CARTESIAN_POINT('Ctrl Pts',(-0.370955558845505,4.50288281188385,
30.875665230774));
#41188=CARTESIAN_POINT('Ctrl Pts',(0.377321147208236,4.56452718844472,30.8492079340895));
#41189=CARTESIAN_POINT('Ctrl Pts',(1.14129584476551,4.43561985486838,30.8227506374051));
#41190=CARTESIAN_POINT('Ctrl Pts',(1.82791726117872,4.13186158171862,30.7962933407206));
#41191=CARTESIAN_POINT('Ctrl Pts',(2.51453867759182,3.82810330856891,30.7698360440361));
#41192=CARTESIAN_POINT('Ctrl Pts',(3.12380681286076,3.34949409584584,30.7433787473517));
#41193=CARTESIAN_POINT('Ctrl Pts',(3.58151348240585,2.75432801596732,30.7169214506672));
#41194=CARTESIAN_POINT('Ctrl Pts',(4.039220151951,2.15916193608874,30.6904641539828));
#41195=CARTESIAN_POINT('Ctrl Pts',(4.34536535577227,1.44743898905468,30.6640068572983));
#41196=CARTESIAN_POINT('Ctrl Pts',(4.4626609468647,0.705846242127884,30.6375495606138));
#41197=CARTESIAN_POINT('Ctrl Pts',(4.49955602397321,0.47257983095123,30.6292274745732));
#41198=CARTESIAN_POINT('Ctrl Pts',(4.5177662531821,0.236358091141789,30.6209053885326));
#41199=CARTESIAN_POINT('Ctrl Pts',(4.5175628644093,0.000105298910395568,
30.612583302492));
#41200=CARTESIAN_POINT('Origin',(0.,0.,20.5));
#41201=CARTESIAN_POINT('',(4.51806064718817,-6.4525231641549E-5,29.612583302492));
#41202=CARTESIAN_POINT('',(4.51741540695923,6.15435095971417E-5,29.887416697508));
#41203=CARTESIAN_POINT('',(4.51775,5.53264807684796E-16,20.5));
#41204=CARTESIAN_POINT('Ctrl Pts',(4.51741540695923,6.15435095971417E-5,
29.887416697508));
#41205=CARTESIAN_POINT('Ctrl Pts',(4.51756272899121,0.306245363704865,29.8982011194113));
#41206=CARTESIAN_POINT('Ctrl Pts',(4.48689091473443,0.612400072796405,29.9089855413145));
#41207=CARTESIAN_POINT('Ctrl Pts',(4.42510561599225,0.912141398858333,29.9197699632178));
#41208=CARTESIAN_POINT('Ctrl Pts',(4.27352846199847,1.64749330398352,29.9462272599022));
#41209=CARTESIAN_POINT('Ctrl Pts',(3.93469095105298,2.34424546963053,29.9726845565867));
#41210=CARTESIAN_POINT('Ctrl Pts',(3.44986311698689,2.91753425314097,29.9991418532711));
#41211=CARTESIAN_POINT('Ctrl Pts',(2.96503528292081,3.49082303665141,30.0255991499556));
#41212=CARTESIAN_POINT('Ctrl Pts',(2.33421712573414,3.94064843802526,30.0520564466401));
#41213=CARTESIAN_POINT('Ctrl Pts',(1.63424159882604,4.21222222121102,30.0785137433246));
#41214=CARTESIAN_POINT('Ctrl Pts',(0.934266071917943,4.48379600439678,30.104971040009));
#41215=CARTESIAN_POINT('Ctrl Pts',(0.165133175288441,4.57711816939443,30.1314283366935));
#41216=CARTESIAN_POINT('Ctrl Pts',(-0.579477555476409,4.48082217978983,
30.157885633378));
#41217=CARTESIAN_POINT('Ctrl Pts',(-1.32408828624126,4.38452619018523,30.1843429300624));
#41218=CARTESIAN_POINT('Ctrl Pts',(-2.04417685114143,4.09861204597837,30.2108002267469));
#41219=CARTESIAN_POINT('Ctrl Pts',(-2.65203725991661,3.65790377350353,30.2372575234314));
#41220=CARTESIAN_POINT('Ctrl Pts',(-3.2598976686918,3.21719550102869,30.2637148201158));
#41221=CARTESIAN_POINT('Ctrl Pts',(-3.75552992134198,2.62169310028588,30.2901721168003));
#41222=CARTESIAN_POINT('Ctrl Pts',(-4.07856655802606,1.94392810462446,30.3166294134847));
#41223=CARTESIAN_POINT('Ctrl Pts',(-4.40160319471017,1.26616310896299,30.3430867101692));
#41224=CARTESIAN_POINT('Ctrl Pts',(-4.55204421542814,0.506135518382923,
30.3695440068537));
#41225=CARTESIAN_POINT('Ctrl Pts',(-4.51156607035432,-0.243584147729374,
30.3960013035382));
#41226=CARTESIAN_POINT('Ctrl Pts',(-4.47108792528051,-0.993303813841587,
30.4224586002227));
#41227=CARTESIAN_POINT('Ctrl Pts',(-4.2396906144149,-1.73271555548614,30.4489158969071));
#41228=CARTESIAN_POINT('Ctrl Pts',(-3.84555807412635,-2.37175984086058,
30.4753731935916));
#41229=CARTESIAN_POINT('Ctrl Pts',(-3.45142553383776,-3.01080412623509,
30.501830490276));
#41230=CARTESIAN_POINT('Ctrl Pts',(-2.89455776412619,-3.54948095533957,
30.5282877869605));
#41231=CARTESIAN_POINT('Ctrl Pts',(-2.24278064303953,-3.92218008655959,
30.554745083645));
#41232=CARTESIAN_POINT('Ctrl Pts',(-1.59100352195292,-4.29487921777957,
30.5812023803295));
#41233=CARTESIAN_POINT('Ctrl Pts',(-0.844317049491253,-4.5016006511151,
30.6076596770139));
#41234=CARTESIAN_POINT('Ctrl Pts',(-0.0936668116191134,-4.51716594477096,
30.6341169736984));
#41235=CARTESIAN_POINT('Ctrl Pts',(0.656983426253069,-4.53273123842682,
30.6605742703828));
#41236=CARTESIAN_POINT('Ctrl Pts',(1.4115974295357,-4.35714039240299,30.6870315670673));
#41237=CARTESIAN_POINT('Ctrl Pts',(2.07826404778386,-4.01178017741331,30.7134888637518));
#41238=CARTESIAN_POINT('Ctrl Pts',(2.74493066603195,-3.66641996242367,30.7399461604362));
#41239=CARTESIAN_POINT('Ctrl Pts',(3.32364989924556,-3.15129037846822,30.7664034571207));
#41240=CARTESIAN_POINT('Ctrl Pts',(3.74393438530595,-2.52913363876272,30.7928607538052));
#41241=CARTESIAN_POINT('Ctrl Pts',(4.16421887136636,-1.90697689905718,30.8193180504897));
#41242=CARTESIAN_POINT('Ctrl Pts',(4.42606861027353,-1.17779300360159,30.8457753471741));
#41243=CARTESIAN_POINT('Ctrl Pts',(4.49759059362584,-0.430395743851834,
30.8722326438586));
#41244=CARTESIAN_POINT('Ctrl Pts',(4.51127293924728,-0.287416660427361,
30.8772939950751));
#41245=CARTESIAN_POINT('Ctrl Pts',(4.51798991567019,-0.143771027837287,
30.8823553462916));
#41246=CARTESIAN_POINT('Ctrl Pts',(4.51784283093286,-0.000111697445491984,
30.8874166975081));
#41247=CARTESIAN_POINT('Ctrl Pts',(4.5175628644093,0.000105298910395568,
30.612583302492));
#41248=CARTESIAN_POINT('Ctrl Pts',(4.51711964642055,-0.514728858223211,
30.5944480918481));
#41249=CARTESIAN_POINT('Ctrl Pts',(4.42923445822943,-1.02971047605454,30.5763128812042));
#41250=CARTESIAN_POINT('Ctrl Pts',(4.25671408259971,-1.51457811392965,30.5581776705604));
#41251=CARTESIAN_POINT('Ctrl Pts',(4.00502564887872,-2.22194717624094,30.5317203738759));
#41252=CARTESIAN_POINT('Ctrl Pts',(3.57320280307314,-2.86522275404404,30.5052630771915));
#41253=CARTESIAN_POINT('Ctrl Pts',(3.01384108989026,-3.36605459389572,30.478805780507));
#41254=CARTESIAN_POINT('Ctrl Pts',(2.45447937670739,-3.86688643374739,30.4523484838226));
#41255=CARTESIAN_POINT('Ctrl Pts',(1.7675787961471,-4.22527453564767,30.425891187138));
#41256=CARTESIAN_POINT('Ctrl Pts',(1.03680307870754,-4.3975676254243,30.3994338904536));
#41257=CARTESIAN_POINT('Ctrl Pts',(0.306027361267937,-4.56986071520095,
30.3729765937691));
#41258=CARTESIAN_POINT('Ctrl Pts',(-0.468623493050924,-4.55605879285401,
30.3465192970847));
#41259=CARTESIAN_POINT('Ctrl Pts',(-1.19279786752355,-4.35784291725031,
30.3200620004002));
#41260=CARTESIAN_POINT('Ctrl Pts',(-1.91697224199613,-4.15962704164662,
30.2936047037158));
#41261=CARTESIAN_POINT('Ctrl Pts',(-2.59067013662245,-3.77699721278612,
30.2671474070313));
#41262=CARTESIAN_POINT('Ctrl Pts',(-3.1318358934393,-3.25655732035575,30.2406901103468));
#41263=CARTESIAN_POINT('Ctrl Pts',(-3.67300165025612,-2.73611742792542,
30.2142328136623));
#41264=CARTESIAN_POINT('Ctrl Pts',(-4.08163526926355,-2.0778674719253,30.1877755169779));
#41265=CARTESIAN_POINT('Ctrl Pts',(-4.30796562791422,-1.3619815684902,30.1613182202934));
#41266=CARTESIAN_POINT('Ctrl Pts',(-4.5342959865649,-0.64609566505506,30.1348609236089));
#41267=CARTESIAN_POINT('Ctrl Pts',(-4.5783230848587,0.127426185815075,30.1084036269244));
#41268=CARTESIAN_POINT('Ctrl Pts',(-4.4346844709496,0.864369878764792,30.08194633024));
#41269=CARTESIAN_POINT('Ctrl Pts',(-4.29104585704049,1.60131357171455,30.0554890335555));
#41270=CARTESIAN_POINT('Ctrl Pts',(-3.95974153092847,2.30167910674398,30.029031736871));
#41271=CARTESIAN_POINT('Ctrl Pts',(-3.48112399286914,2.88016273680294,30.0025744401866));
#41272=CARTESIAN_POINT('Ctrl Pts',(-3.00250645480984,3.45864636686186,29.9761171435021));
#41273=CARTESIAN_POINT('Ctrl Pts',(-2.37657570480325,3.91524809195029,29.9496598468177));
#41274=CARTESIAN_POINT('Ctrl Pts',(-1.67956941546306,4.19435432728787,29.9232025501332));
#41275=CARTESIAN_POINT('Ctrl Pts',(-0.982563126122875,4.47346056262544,
29.8967452534487));
#41276=CARTESIAN_POINT('Ctrl Pts',(-0.214481297449103,4.57507130821215,
29.8702879567642));
#41277=CARTESIAN_POINT('Ctrl Pts',(0.53112455388596,4.48681048769132,29.8438306600798));
#41278=CARTESIAN_POINT('Ctrl Pts',(1.27673040522102,4.39854966717049,29.8173733633953));
#41279=CARTESIAN_POINT('Ctrl Pts',(1.99986027921735,4.12041728054213,29.7909160667108));
#41280=CARTESIAN_POINT('Ctrl Pts',(2.61243775753263,3.68628954467976,29.7644587700264));
#41281=CARTESIAN_POINT('Ctrl Pts',(3.22501523584791,3.25216180881739,29.7380014733419));
#41282=CARTESIAN_POINT('Ctrl Pts',(3.72704031848211,2.66203872372102,29.7115441766574));
#41283=CARTESIAN_POINT('Ctrl Pts',(4.05736690597726,1.98779662804773,29.685086879973));
#41284=CARTESIAN_POINT('Ctrl Pts',(4.35910923962182,1.37189893439675,29.6609190208126));
#41285=CARTESIAN_POINT('Ctrl Pts',(4.51758267646005,0.685810539097339,29.6367511616523));
#41286=CARTESIAN_POINT('Ctrl Pts',(4.51806064718817,-6.4525231641549E-5,
29.612583302492));
#41287=CARTESIAN_POINT('Origin',(0.,0.,20.5));
#41288=CARTESIAN_POINT('',(4.51736349586412,-8.67285085925565E-6,28.612583302492));
#41289=CARTESIAN_POINT('',(4.51813672578305,5.21363961469835E-6,28.8874166975081));
#41290=CARTESIAN_POINT('',(4.51775,5.53264807684796E-16,20.5));
#41291=CARTESIAN_POINT('Ctrl Pts',(4.51813645424719,5.20997890686523E-6,
28.8874166975081));
#41292=CARTESIAN_POINT('Ctrl Pts',(4.51813678764949,0.00491176269805106,
28.8875895958466));
#41293=CARTESIAN_POINT('Ctrl Pts',(4.51812896220818,0.00981831434884656,
28.887762494185));
#41294=CARTESIAN_POINT('Ctrl Pts',(4.51811297150728,0.0147248393885022,
28.8879353925235));
#41295=CARTESIAN_POINT('Ctrl Pts',(4.51566603811481,0.7655324515643,28.914392689208));
#41296=CARTESIAN_POINT('Ctrl Pts',(4.32202288903541,1.51571694218793,28.9408499858924));
#41297=CARTESIAN_POINT('Ctrl Pts',(3.96076904551605,2.17390667055403,28.9673072825769));
#41298=CARTESIAN_POINT('Ctrl Pts',(3.59951520199672,2.83209639892005,28.9937645792614));
#41299=CARTESIAN_POINT('Ctrl Pts',(3.07065066403746,3.39829136502856,29.0202218759458));
#41300=CARTESIAN_POINT('Ctrl Pts',(2.43859054705081,3.8035296486332,29.0466791726303));
#41301=CARTESIAN_POINT('Ctrl Pts',(1.80653043006408,4.20876793223789,29.0731364693148));
#41302=CARTESIAN_POINT('Ctrl Pts',(1.07127473404993,4.45304953333867,29.0995937659992));
#41303=CARTESIAN_POINT('Ctrl Pts',(0.32237678905244,4.50662122327555,29.1260510626837));
#41304=CARTESIAN_POINT('Ctrl Pts',(-0.426521155945046,4.56019291321243,
29.1525083593682));
#41305=CARTESIAN_POINT('Ctrl Pts',(-1.18906134992587,4.42305469198539,29.1789656560527));
#41306=CARTESIAN_POINT('Ctrl Pts',(-1.87236724119019,4.11190984316476,29.2054229527371));
#41307=CARTESIAN_POINT('Ctrl Pts',(-2.55567313245444,3.80076499434415,29.2318802494216));
#41308=CARTESIAN_POINT('Ctrl Pts',(-3.15974472100221,3.31561351792999,29.258337546106));
#41309=CARTESIAN_POINT('Ctrl Pts',(-3.61100675589329,2.7155463268172,29.2847948427905));
#41310=CARTESIAN_POINT('Ctrl Pts',(-4.06226879078437,2.11547913570442,29.311252139475));
#41311=CARTESIAN_POINT('Ctrl Pts',(-4.36072127201875,1.40049622989302,29.3377094361595));
#41312=CARTESIAN_POINT('Ctrl Pts',(-4.47001301768878,0.657681736016911,
29.3641667328439));
#41313=CARTESIAN_POINT('Ctrl Pts',(-4.57930476335883,-0.0851327578592831,
29.3906240295284));
#41314=CARTESIAN_POINT('Ctrl Pts',(-4.49943577346447,-0.855778839800193,
29.4170813262128));
#41315=CARTESIAN_POINT('Ctrl Pts',(-4.24013400258134,-1.56039266992349,
29.4435386228973));
#41316=CARTESIAN_POINT('Ctrl Pts',(-3.98083223169821,-2.26500650004679,
29.4699959195818));
#41317=CARTESIAN_POINT('Ctrl Pts',(-3.54209767982631,-2.90358807835248,
29.4964532162663));
#41318=CARTESIAN_POINT('Ctrl Pts',(-2.97736772982241,-3.39835887534109,
29.5229105129507));
#41319=CARTESIAN_POINT('Ctrl Pts',(-2.41263777981851,-3.8931296723297,29.5493678096352));
#41320=CARTESIAN_POINT('Ctrl Pts',(-1.72191243168261,-4.24408968800123,
29.5758251063197));
#41321=CARTESIAN_POINT('Ctrl Pts',(-0.989321268370363,-4.40849238086531,
29.6022824030041));
#41322=CARTESIAN_POINT('Ctrl Pts',(-0.256730105058199,-4.57289507372936,
29.6287396996886));
#41323=CARTESIAN_POINT('Ctrl Pts',(0.517726873430306,-4.55074044378599,
29.655196996373));
#41324=CARTESIAN_POINT('Ctrl Pts',(1.23972166423099,-4.34472690044308,29.6816542930575));
#41325=CARTESIAN_POINT('Ctrl Pts',(1.96171645503171,-4.13871335710016,29.708111589742));
#41326=CARTESIAN_POINT('Ctrl Pts',(2.63124905814461,-3.74884090035768,29.7345688864265));
#41327=CARTESIAN_POINT('Ctrl Pts',(3.16677114350317,-3.22259556396285,29.761026183111));
#41328=CARTESIAN_POINT('Ctrl Pts',(3.70229322886173,-2.69635022756802,29.7874834797954));
#41329=CARTESIAN_POINT('Ctrl Pts',(4.10380479646594,-2.03373201152084,29.8139407764799));
#41330=CARTESIAN_POINT('Ctrl Pts',(4.32240218174702,-1.31544708119558,29.8403980731643));
#41331=CARTESIAN_POINT('Ctrl Pts',(4.45189573839702,-0.889946702056473,
29.8560709479456));
#41332=CARTESIAN_POINT('Ctrl Pts',(4.51720130556553,-0.444911837263118,
29.8717438227268));
#41333=CARTESIAN_POINT('Ctrl Pts',(4.51741540695923,6.15435095971417E-5,
29.887416697508));
#41334=CARTESIAN_POINT('Ctrl Pts',(4.51806064718817,-6.4525231641549E-5,
29.612583302492));
#41335=CARTESIAN_POINT('Ctrl Pts',(4.51810592567614,-0.065037930559881,
29.6102938649678));
#41336=CARTESIAN_POINT('Ctrl Pts',(4.51673336863491,-0.130009421477303,
29.6080044274437));
#41337=CARTESIAN_POINT('Ctrl Pts',(4.51393045695516,-0.194919147263631,
29.6057149899196));
#41338=CARTESIAN_POINT('Ctrl Pts',(4.48153932808183,-0.945031720651385,
29.5792576932351));
#41339=CARTESIAN_POINT('Ctrl Pts',(4.25812897797913,-1.68689576117669,29.5528003965506));
#41340=CARTESIAN_POINT('Ctrl Pts',(3.87091054003435,-2.33015304974767,29.5263430998662));
#41341=CARTESIAN_POINT('Ctrl Pts',(3.48369210208957,-2.97341033831866,29.4998858031817));
#41342=CARTESIAN_POINT('Ctrl Pts',(2.9326655763027,-3.51806087493531,29.4734285064972));
#41343=CARTESIAN_POINT('Ctrl Pts',(2.28494538367634,-3.89776682701949,29.4469712098128));
#41344=CARTESIAN_POINT('Ctrl Pts',(1.63722519105001,-4.27747277910364,29.4205139131283));
#41345=CARTESIAN_POINT('Ctrl Pts',(0.892811331584192,-4.49223414665534,
29.3940566164438));
#41346=CARTESIAN_POINT('Ctrl Pts',(0.142372589495739,-4.5158932327899,29.3675993197594));
#41347=CARTESIAN_POINT('Ctrl Pts',(-0.608066152592799,-4.53955231892447,
29.3411420230749));
#41348=CARTESIAN_POINT('Ctrl Pts',(-1.36452977730397,-4.37210912364185,
29.3146847263904));
#41349=CARTESIAN_POINT('Ctrl Pts',(-2.03488185234987,-4.03395804281286,
29.288227429706));
#41350=CARTESIAN_POINT('Ctrl Pts',(-2.70523392739576,-3.69580696198387,
29.2617701330215));
#41351=CARTESIAN_POINT('Ctrl Pts',(-3.28947445277638,-3.18694799560851,
29.235312836337));
#41352=CARTESIAN_POINT('Ctrl Pts',(-3.71644357909758,-2.56935960262119,
29.2088555396525));
#41353=CARTESIAN_POINT('Ctrl Pts',(-4.14341270541876,-1.95177120963391,
29.1823982429681));
#41354=CARTESIAN_POINT('Ctrl Pts',(-4.41311043268056,-1.22545339003468,
29.1559409462836));
#41355=CARTESIAN_POINT('Ctrl Pts',(-4.49268787618537,-0.478870850412086,
29.1294836495992));
#41356=CARTESIAN_POINT('Ctrl Pts',(-4.57226531969018,0.267711689210511,
29.1030263529147));
#41357=CARTESIAN_POINT('Ctrl Pts',(-4.46172247943801,1.03455894885648,29.0765690562302));
#41358=CARTESIAN_POINT('Ctrl Pts',(-4.17452335103036,1.72826978099475,29.0501117595457));
#41359=CARTESIAN_POINT('Ctrl Pts',(-3.88732422262269,2.42198061313306,29.0236544628612));
#41360=CARTESIAN_POINT('Ctrl Pts',(-3.42346880605953,3.04255501776367,28.9971971661768));
#41361=CARTESIAN_POINT('Ctrl Pts',(-2.83945417771499,3.51440771921163,28.9707398694923));
#41362=CARTESIAN_POINT('Ctrl Pts',(-2.25543954937045,3.98626042065959,28.9442825728079));
#41363=CARTESIAN_POINT('Ctrl Pts',(-1.55126570924453,4.3093914189249,28.9178252761234));
#41364=CARTESIAN_POINT('Ctrl Pts',(-0.812700251733401,4.44444371603802,
28.8913679794389));
#41365=CARTESIAN_POINT('Ctrl Pts',(-0.0741347942223568,4.57949601315112,
28.8649106827545));
#41366=CARTESIAN_POINT('Ctrl Pts',(0.698822280673891,4.52646960911207,28.83845338607));
#41367=CARTESIAN_POINT('Ctrl Pts',(1.41202565668872,4.29182306124684,28.8119960893855));
#41368=CARTESIAN_POINT('Ctrl Pts',(2.12522903270359,4.05717651338159,28.785538792701));
#41369=CARTESIAN_POINT('Ctrl Pts',(2.77867870983704,3.64090982169015,28.7590814960166));
#41370=CARTESIAN_POINT('Ctrl Pts',(3.29278524060738,3.09372380852518,28.7326241993321));
#41371=CARTESIAN_POINT('Ctrl Pts',(3.80689177137772,2.54653779536021,28.7061669026477));
#41372=CARTESIAN_POINT('Ctrl Pts',(4.18165515578495,1.86843246072172,28.6797096059632));
#41373=CARTESIAN_POINT('Ctrl Pts',(4.37142962837061,1.14200028388831,28.6532523092787));
#41374=CARTESIAN_POINT('Ctrl Pts',(4.46866731930057,0.769786958618117,28.6396959736831));
#41375=CARTESIAN_POINT('Ctrl Pts',(4.517338221792,0.384885956569512,28.6261396380875));
#41376=CARTESIAN_POINT('Ctrl Pts',(4.51736392670147,-8.66318320566495E-6,
28.612583302492));
#41377=CARTESIAN_POINT('Origin',(0.,0.,20.5));
#41378=CARTESIAN_POINT('',(4.51801726226543,7.95831363512023E-5,27.612583302492));
#41379=CARTESIAN_POINT('',(4.51743092439869,-6.91819792334251E-5,27.8874166975081));
#41380=CARTESIAN_POINT('',(4.51775,5.53264807684796E-16,20.5));
#41381=CARTESIAN_POINT('Ctrl Pts',(4.51743092439869,-6.91819792334251E-5,
27.8874166975081));
#41382=CARTESIAN_POINT('Ctrl Pts',(4.51718386244179,0.454717345983238,27.9034353689663));
#41383=CARTESIAN_POINT('Ctrl Pts',(4.44891863177309,0.909576397762494,27.9194540404245));
#41384=CARTESIAN_POINT('Ctrl Pts',(4.31373618863887,1.34359284719174,27.9354727118827));
#41385=CARTESIAN_POINT('Ctrl Pts',(4.09046161721975,2.06043768656892,27.9619300085671));
#41386=CARTESIAN_POINT('Ctrl Pts',(3.68463958850139,2.72042474717273,27.9883873052516));
#41387=CARTESIAN_POINT('Ctrl Pts',(3.14569877644576,3.24316833544992,28.0148446019361));
#41388=CARTESIAN_POINT('Ctrl Pts',(2.60675796439011,3.76591192372714,28.0413018986205));
#41389=CARTESIAN_POINT('Ctrl Pts',(1.93469836899718,4.15141203967772,28.067759195305));
#41390=CARTESIAN_POINT('Ctrl Pts',(1.21137610519651,4.3527151958239,28.0942164919895));
#41391=CARTESIAN_POINT('Ctrl Pts',(0.48805384139591,4.55401835197006,28.1206737886739));
#41392=CARTESIAN_POINT('Ctrl Pts',(-0.286531090812426,4.57112454831186,
28.1471310853584));
#41393=CARTESIAN_POINT('Ctrl Pts',(-1.01803510394287,4.40195026906682,28.1735883820429));
#41394=CARTESIAN_POINT('Ctrl Pts',(-1.7495391170734,4.23277598982176,28.2000456787273));
#41395=CARTESIAN_POINT('Ctrl Pts',(-2.43796221112602,3.87732123498983,28.2265029754118));
#41396=CARTESIAN_POINT('Ctrl Pts',(-2.99945521514446,3.37888000031668,28.2529602720963));
#41397=CARTESIAN_POINT('Ctrl Pts',(-3.56094821916288,2.88043876564355,28.2794175687807));
#41398=CARTESIAN_POINT('Ctrl Pts',(-3.99551113314713,2.23901105112923,28.3058748654652));
#41399=CARTESIAN_POINT('Ctrl Pts',(-4.25021467511827,1.53272204251347,28.3323321621497));
#41400=CARTESIAN_POINT('Ctrl Pts',(-4.50491821708942,0.826433033897707,
28.3587894588341));
#41401=CARTESIAN_POINT('Ctrl Pts',(-4.57976238704747,0.0552827311804979,
28.3852467555186));
#41402=CARTESIAN_POINT('Ctrl Pts',(-4.4656312479239,-0.686803612223317,
28.4117040522031));
#41403=CARTESIAN_POINT('Ctrl Pts',(-4.35150010880033,-1.42888995562718,
28.4381613488875));
#41404=CARTESIAN_POINT('Ctrl Pts',(-4.04839366059513,-2.14191233971764,
28.464618645572));
#41405=CARTESIAN_POINT('Ctrl Pts',(-3.59322993324233,-2.73902542723662,
28.4910759422565));
#41406=CARTESIAN_POINT('Ctrl Pts',(-3.13806620588952,-3.3361385147556,28.517533238941));
#41407=CARTESIAN_POINT('Ctrl Pts',(-2.5308451993891,-3.8173423057031,28.5439905356254));
#41408=CARTESIAN_POINT('Ctrl Pts',(-1.84552576030239,-4.12402671090497,
28.5704478323099));
#41409=CARTESIAN_POINT('Ctrl Pts',(-1.16020632121576,-4.4307111161068,28.5969051289944));
#41410=CARTESIAN_POINT('Ctrl Pts',(-0.396788449542842,-4.56287613556305,
28.6233624256788));
#41411=CARTESIAN_POINT('Ctrl Pts',(0.351744402845005,-4.50442421617509,
28.6498197223633));
#41412=CARTESIAN_POINT('Ctrl Pts',(1.10027725523294,-4.44597229678712,28.6762770190477));
#41413=CARTESIAN_POINT('Ctrl Pts',(1.8339250883358,-4.19690343855492,28.7027343157322));
#41414=CARTESIAN_POINT('Ctrl Pts',(2.46333040803262,-3.78755395275886,28.7291916124167));
#41415=CARTESIAN_POINT('Ctrl Pts',(3.09273572772936,-3.37820446696285,28.7556489091012));
#41416=CARTESIAN_POINT('Ctrl Pts',(3.61789853402009,-2.80857435360303,28.7821062057856));
#41417=CARTESIAN_POINT('Ctrl Pts',(3.97485457831268,-2.14804393005918,28.8085635024701));
#41418=CARTESIAN_POINT('Ctrl Pts',(4.32947791614233,-1.49183007045257,28.8348479008161));
#41419=CARTESIAN_POINT('Ctrl Pts',(4.51808576967277,-0.745900085055985,
28.8611322991621));
#41420=CARTESIAN_POINT('Ctrl Pts',(4.51813645424719,5.20997890686523E-6,
28.8874166975081));
#41421=CARTESIAN_POINT('Ctrl Pts',(4.51736392670147,-8.66318320566495E-6,
28.612583302492));
#41422=CARTESIAN_POINT('Ctrl Pts',(4.5173883889195,-0.366295738162854,28.5996823414031));
#41423=CARTESIAN_POINT('Ctrl Pts',(4.47335741760473,-0.732577033027994,
28.5867813803142));
#41424=CARTESIAN_POINT('Ctrl Pts',(4.38520343465814,-1.08791198212899,28.5738804192253));
#41425=CARTESIAN_POINT('Ctrl Pts',(4.20441720759592,-1.81663305228457,28.5474231225409));
#41426=CARTESIAN_POINT('Ctrl Pts',(3.8380591927074,-2.49931617356742,28.5209658258564));
#41427=CARTESIAN_POINT('Ctrl Pts',(3.33075139074614,-3.05281129735201,28.4945085291719));
#41428=CARTESIAN_POINT('Ctrl Pts',(2.82344358878484,-3.60630642113663,28.4680512324875));
#41429=CARTESIAN_POINT('Ctrl Pts',(2.17518599975079,-4.03061354742298,28.441593935803));
#41430=CARTESIAN_POINT('Ctrl Pts',(1.46493568054142,-4.27405253782332,28.4151366391185));
#41431=CARTESIAN_POINT('Ctrl Pts',(0.754685361332094,-4.51749152822365,
28.388679342434));
#41432=CARTESIAN_POINT('Ctrl Pts',(-0.0175576880525484,-4.580062382738,
28.3622220457496));
#41433=CARTESIAN_POINT('Ctrl Pts',(-0.757735118862955,-4.45414404053564,
28.3357647490651));
#41434=CARTESIAN_POINT('Ctrl Pts',(-1.49791254967336,-4.32822569833327,
28.3093074523807));
#41435=CARTESIAN_POINT('Ctrl Pts',(-2.20602436190953,-4.01381815941419,
28.2828501556962));
#41436=CARTESIAN_POINT('Ctrl Pts',(-2.79582332053056,-3.54921591405409,
28.2563928590117));
#41437=CARTESIAN_POINT('Ctrl Pts',(-3.38562227915162,-3.08461366869397,
28.2299355623272));
#41438=CARTESIAN_POINT('Ctrl Pts',(-3.85710838415752,-2.46981671689283,
28.2034782656428));
#41439=CARTESIAN_POINT('Ctrl Pts',(-4.15285514976694,-1.77970664696505,
28.1770209689583));
#41440=CARTESIAN_POINT('Ctrl Pts',(-4.44860191537634,-1.08959657703732,
28.1505636722738));
#41441=CARTESIAN_POINT('Ctrl Pts',(-4.56860934158928,-0.32417338898296,
28.1241063755894));
#41442=CARTESIAN_POINT('Ctrl Pts',(-4.49826065670898,0.423335220010742,
28.0976490789049));
#41443=CARTESIAN_POINT('Ctrl Pts',(-4.42791197182868,1.17084382900444,28.0711917822204));
#41444=CARTESIAN_POINT('Ctrl Pts',(-4.16720717585513,1.90043785893749,28.0447344855359));
#41445=CARTESIAN_POINT('Ctrl Pts',(-3.7478998244078,2.52325356442854,28.0182771888515));
#41446=CARTESIAN_POINT('Ctrl Pts',(-3.32859247296047,3.14606926991958,27.991819892167));
#41447=CARTESIAN_POINT('Ctrl Pts',(-2.75068256603934,3.66210665096863,27.9653625954826));
#41448=CARTESIAN_POINT('Ctrl Pts',(-2.08455889071647,4.00851292567859,27.9389052987981));
#41449=CARTESIAN_POINT('Ctrl Pts',(-1.41843521539359,4.35491920038855,27.9124480021136));
#41450=CARTESIAN_POINT('Ctrl Pts',(-0.664097771668966,4.53169436875941,
27.8859907054291));
#41451=CARTESIAN_POINT('Ctrl Pts',(0.0865759746605513,4.51730741092622,
27.8595334087447));
#41452=CARTESIAN_POINT('Ctrl Pts',(0.837249720990026,4.50292045309303,27.8330761120602));
#41453=CARTESIAN_POINT('Ctrl Pts',(1.58425976992439,4.2973713690558,27.8066188153758));
#41454=CARTESIAN_POINT('Ctrl Pts',(2.23662112424281,3.92569580976267,27.7801615186913));
#41455=CARTESIAN_POINT('Ctrl Pts',(2.88898247856131,3.5540202504695,27.7537042220068));
#41456=CARTESIAN_POINT('Ctrl Pts',(3.44669513826383,3.0162182159204,27.7272469253223));
#41457=CARTESIAN_POINT('Ctrl Pts',(3.84183031863663,2.37779339872113,27.7007896286379));
#41458=CARTESIAN_POINT('Ctrl Pts',(4.23696549900942,1.73936858152187,27.6743323319534));
#41459=CARTESIAN_POINT('Ctrl Pts',(4.46952320005248,1.00032098167245,27.647875035269));
#41460=CARTESIAN_POINT('Ctrl Pts',(4.51117815115764,0.250665778907488,27.6214177385845));
#41461=CARTESIAN_POINT('Ctrl Pts',(4.51581452813225,0.167225898922454,27.6184729265537));
#41462=CARTESIAN_POINT('Ctrl Pts',(4.51808587645197,0.0836546049852204,
27.6155281145228));
#41463=CARTESIAN_POINT('Ctrl Pts',(4.51801726226543,7.95831363512023E-5,
27.612583302492));
#41464=CARTESIAN_POINT('Origin',(0.,0.,20.5));
#41465=CARTESIAN_POINT('',(4.51761428595877,-0.000111883206665997,26.612583302492));
#41466=CARTESIAN_POINT('',(4.51781182322151,0.000114263439177032,26.8874166975081));
#41467=CARTESIAN_POINT('',(4.51775,5.53264807684796E-16,20.5));
#41468=CARTESIAN_POINT('Ctrl Pts',(4.51781182322151,0.000114263439177032,
26.8874166975081));
#41469=CARTESIAN_POINT('Ctrl Pts',(4.51797007849026,0.153591581624792,26.8928238454015));
#41470=CARTESIAN_POINT('Ctrl Pts',(4.51030214935632,0.307053160819986,26.898230993295));
#41471=CARTESIAN_POINT('Ctrl Pts',(4.49468970350708,0.459702200761322,26.9036381411884));
#41472=CARTESIAN_POINT('Ctrl Pts',(4.41829765358665,1.20661739855353,26.9300954378729));
#41473=CARTESIAN_POINT('Ctrl Pts',(4.1517006071518,1.93407904976938,26.9565527345573));
#41474=CARTESIAN_POINT('Ctrl Pts',(3.727369789407,2.55348313039531,26.9830100312418));
#41475=CARTESIAN_POINT('Ctrl Pts',(3.30303897166215,3.17288721102131,27.0094673279263));
#41476=CARTESIAN_POINT('Ctrl Pts',(2.72097438260733,3.68423372105737,27.0359246246107));
#41477=CARTESIAN_POINT('Ctrl Pts',(2.05207084500035,4.02524122150424,27.0623819212952));
#41478=CARTESIAN_POINT('Ctrl Pts',(1.38316730739341,4.36624872195109,27.0888392179797));
#41479=CARTESIAN_POINT('Ctrl Pts',(0.627424821234327,4.53691721280878,27.1152965146642));
#41480=CARTESIAN_POINT('Ctrl Pts',(-0.123108015066531,4.51645946077497,
27.1417538113486));
#41481=CARTESIAN_POINT('Ctrl Pts',(-0.873640851367389,4.49600170874117,
27.1682111080331));
#41482=CARTESIAN_POINT('Ctrl Pts',(-1.61896403781002,4.28441771381588,27.1946684047176));
#41483=CARTESIAN_POINT('Ctrl Pts',(-2.26829803515817,3.9074781724144,27.221125701402));
#41484=CARTESIAN_POINT('Ctrl Pts',(-2.91763203250632,3.53053863101291,27.2475829980865));
#41485=CARTESIAN_POINT('Ctrl Pts',(-3.47097684075998,2.98824354313522,27.274040294771));
#41486=CARTESIAN_POINT('Ctrl Pts',(-3.86093567467783,2.34664385030993,27.3004975914554));
#41487=CARTESIAN_POINT('Ctrl Pts',(-4.25089450859569,1.70504415748464,27.3269548881399));
#41488=CARTESIAN_POINT('Ctrl Pts',(-4.47746736817774,0.96413985971173,27.3534121848244));
#41489=CARTESIAN_POINT('Ctrl Pts',(-4.51305792988216,0.214172280478033,
27.3798694815088));
#41490=CARTESIAN_POINT('Ctrl Pts',(-4.54864849158657,-0.535795298755707,
27.4063267781933));
#41491=CARTESIAN_POINT('Ctrl Pts',(-4.39325675541333,-1.29482615945024,
27.4327840748778));
#41492=CARTESIAN_POINT('Ctrl Pts',(-4.06580926285144,-1.97047118281612,
27.4592413715622));
#41493=CARTESIAN_POINT('Ctrl Pts',(-3.73836177028958,-2.64611620618197,
27.4856986682467));
#41494=CARTESIAN_POINT('Ctrl Pts',(-3.23885852133909,-3.23837539221917,
27.5121559649312));
#41495=CARTESIAN_POINT('Ctrl Pts',(-2.62813845890629,-3.67511222754014,
27.5386132616156));
#41496=CARTESIAN_POINT('Ctrl Pts',(-2.0174183964735,-4.11184906286111,27.5650705583001));
#41497=CARTESIAN_POINT('Ctrl Pts',(-1.29548152055841,-4.39306354746584,
27.5915278549846));
#41498=CARTESIAN_POINT('Ctrl Pts',(-0.550258943657392,-4.48450406835833,
27.617985151669));
#41499=CARTESIAN_POINT('Ctrl Pts',(0.194963633243671,-4.57594458925083,
27.6444424483535));
#41500=CARTESIAN_POINT('Ctrl Pts',(0.963471911130666,-4.47761114643107,
27.670899745038));
#41501=CARTESIAN_POINT('Ctrl Pts',(1.66166243228906,-4.20148064440581,27.6973570417224));
#41502=CARTESIAN_POINT('Ctrl Pts',(2.35985295344741,-3.92535014238055,27.7238143384069));
#41503=CARTESIAN_POINT('Ctrl Pts',(2.98772571787716,-3.47142258114982,27.7502716350914));
#41504=CARTESIAN_POINT('Ctrl Pts',(3.46880651775718,-2.89498583529569,27.7767289317758));
#41505=CARTESIAN_POINT('Ctrl Pts',(3.94988731763719,-2.31854908944157,27.8031862284603));
#41506=CARTESIAN_POINT('Ctrl Pts',(4.28417615296746,-1.61960315896406,27.8296435251448));
#41507=CARTESIAN_POINT('Ctrl Pts',(4.43095701357266,-0.883278884650025,
27.8561008218292));
#41508=CARTESIAN_POINT('Ctrl Pts',(4.48886884079068,-0.592764958142916,
27.8665394470555));
#41509=CARTESIAN_POINT('Ctrl Pts',(4.517591923217,-0.296432468768919,27.8769780722818));
#41510=CARTESIAN_POINT('Ctrl Pts',(4.51743092439869,-6.91819792334251E-5,
27.8874166975081));
#41511=CARTESIAN_POINT('Ctrl Pts',(4.51801726226543,7.95831363512023E-5,
27.612583302492));
#41512=CARTESIAN_POINT('Ctrl Pts',(4.5174694208443,-0.667214763012837,27.5890708178383));
#41513=CARTESIAN_POINT('Ctrl Pts',(4.36774838447631,-1.33474676446109,27.5655583331847));
#41514=CARTESIAN_POINT('Ctrl Pts',(4.08161297138008,-1.93752346980862,27.5420458485311));
#41515=CARTESIAN_POINT('Ctrl Pts',(3.7596406393301,-2.61579471007933,27.5155885518466));
#41516=CARTESIAN_POINT('Ctrl Pts',(3.26494377406285,-3.21207438494031,27.4891312551621));
#41517=CARTESIAN_POINT('Ctrl Pts',(2.65777590627143,-3.65373628991481,27.4626739584777));
#41518=CARTESIAN_POINT('Ctrl Pts',(2.05060803847998,-4.09539819488933,27.4362166617932));
#41519=CARTESIAN_POINT('Ctrl Pts',(1.33096916816432,-4.38244232997737,27.4097593651087));
#41520=CARTESIAN_POINT('Ctrl Pts',(0.586510513282131,-4.47990703720589,
27.3833020684243));
#41521=CARTESIAN_POINT('Ctrl Pts',(-0.15794814160006,-4.57737174443442,
27.3568447717398));
#41522=CARTESIAN_POINT('Ctrl Pts',(-0.927226581048814,-4.48525702380344,
27.3303874750553));
#41523=CARTESIAN_POINT('Ctrl Pts',(-1.62762754252371,-4.21478234633956,
27.3039301783709));
#41524=CARTESIAN_POINT('Ctrl Pts',(-2.32802850399852,-3.94430766887572,
27.2774728816864));
#41525=CARTESIAN_POINT('Ctrl Pts',(-2.95955198749952,-3.49547303457901,
27.2510155850019));
#41526=CARTESIAN_POINT('Ctrl Pts',(-3.44527913166303,-2.92294600516749,
27.2245582883174));
#41527=CARTESIAN_POINT('Ctrl Pts',(-3.93100627582659,-2.35041897575591,
27.198100991633));
#41528=CARTESIAN_POINT('Ctrl Pts',(-4.27093708065265,-1.65419955122946,
27.1716436949485));
#41529=CARTESIAN_POINT('Ctrl Pts',(-4.42366835032541,-0.919086486967716,
27.1451863982641));
#41530=CARTESIAN_POINT('Ctrl Pts',(-4.57639961999816,-0.183973422706017,
27.1187291015796));
#41531=CARTESIAN_POINT('Ctrl Pts',(-4.54193135451766,0.590033281290875,
27.0922718048951));
#41532=CARTESIAN_POINT('Ctrl Pts',(-4.32446175047231,1.30866046509374,27.0658145082107));
#41533=CARTESIAN_POINT('Ctrl Pts',(-4.10699214642695,2.02728764889665,27.0393572115262));
#41534=CARTESIAN_POINT('Ctrl Pts',(-3.7065212038167,2.69053531250543,27.0128999148417));
#41535=CARTESIAN_POINT('Ctrl Pts',(-3.17182584023783,3.21762062452939,26.9864426181572));
#41536=CARTESIAN_POINT('Ctrl Pts',(-2.63713047665899,3.74470593655333,26.9599853214728));
#41537=CARTESIAN_POINT('Ctrl Pts',(-1.96821069211152,4.13562889699249,26.9335280247883));
#41538=CARTESIAN_POINT('Ctrl Pts',(-1.2465401760389,4.34277552191203,26.9070707281038));
#41539=CARTESIAN_POINT('Ctrl Pts',(-0.524869659966319,4.54992214683155,
26.8806134314194));
#41540=CARTESIAN_POINT('Ctrl Pts',(0.249551587631431,4.57329243623147,26.8541561347349));
#41541=CARTESIAN_POINT('Ctrl Pts',(0.982399915873105,4.41003991472752,26.8276988380504));
#41542=CARTESIAN_POINT('Ctrl Pts',(1.71524824411482,4.24678739322355,26.801241541366));
#41543=CARTESIAN_POINT('Ctrl Pts',(2.40652365300059,3.89691206081561,26.7747842446815));
#41544=CARTESIAN_POINT('Ctrl Pts',(2.97202956278397,3.40302834577314,26.748326947997));
#41545=CARTESIAN_POINT('Ctrl Pts',(3.53753547256739,2.90914463073064,26.7218696513126));
#41546=CARTESIAN_POINT('Ctrl Pts',(3.97727188324847,2.27125253305366,26.6954123546281));
#41547=CARTESIAN_POINT('Ctrl Pts',(4.23767938667642,1.56704660426395,26.6689550579436));
#41548=CARTESIAN_POINT('Ctrl Pts',(4.42262682954492,1.06690323639616,26.6501644727931));
#41549=CARTESIAN_POINT('Ctrl Pts',(4.5171177314681,0.533310047910147,26.6313738876425));
#41550=CARTESIAN_POINT('Ctrl Pts',(4.51761428595877,-0.000111883206665997,
26.612583302492));
#41551=CARTESIAN_POINT('Origin',(0.,0.,20.5));
#41552=CARTESIAN_POINT('',(4.51757373878986,0.000106944042679857,25.612583302492));
#41553=CARTESIAN_POINT('',(4.51783003468408,-0.000112853895665516,25.8874166975081));
#41554=CARTESIAN_POINT('',(4.51775,5.53264807684796E-16,20.5));
#41555=CARTESIAN_POINT('Ctrl Pts',(4.51783003468408,-0.000112853895665516,
25.8874166975081));
#41556=CARTESIAN_POINT('Ctrl Pts',(4.51721010591009,0.603126320584693,25.9086696185212));
#41557=CARTESIAN_POINT('Ctrl Pts',(4.39561298077165,1.20660788106352,25.9299225395344));
#41558=CARTESIAN_POINT('Ctrl Pts',(4.16040899613699,1.76197577425452,25.9511754605476));
#41559=CARTESIAN_POINT('Ctrl Pts',(3.86760869828648,2.45334112163804,25.977632757232));
#41560=CARTESIAN_POINT('Ctrl Pts',(3.39874939952398,3.0701436809076,26.0040900539165));
#41561=CARTESIAN_POINT('Ctrl Pts',(2.81093764353751,3.53725758297881,26.030547350601));
#41562=CARTESIAN_POINT('Ctrl Pts',(2.22312588755105,4.00437148505003,26.0570046472854));
#41563=CARTESIAN_POINT('Ctrl Pts',(1.51636167434063,4.32179672992291,26.0834619439699));
#41564=CARTESIAN_POINT('Ctrl Pts',(0.776728102877261,4.45087127407636,26.1099192406544));
#41565=CARTESIAN_POINT('Ctrl Pts',(0.0370945314138876,4.57994581822981,
26.1363765373388));
#41566=CARTESIAN_POINT('Ctrl Pts',(-0.735408398302442,4.52066966166383,
26.1628338340233));
#41567=CARTESIAN_POINT('Ctrl Pts',(-1.4466906843854,4.28026257464538,26.1892911307078));
#41568=CARTESIAN_POINT('Ctrl Pts',(-2.15797297046839,4.03985548762692,26.2157484273923));
#41569=CARTESIAN_POINT('Ctrl Pts',(-2.80803461291801,3.61831747015598,26.2422057240767));
#41570=CARTESIAN_POINT('Ctrl Pts',(-3.31769882312739,3.06699138623123,26.2686630207612));
#41571=CARTESIAN_POINT('Ctrl Pts',(-3.82736303333674,2.51566530230651,26.2951203174456));
#41572=CARTESIAN_POINT('Ctrl Pts',(-4.19662981130587,1.834551151928,26.3215776141301));
#41573=CARTESIAN_POINT('Ctrl Pts',(-4.38052287215722,1.1066078848015,26.3480349108146));
#41574=CARTESIAN_POINT('Ctrl Pts',(-4.56441593300857,0.378664617674993,
26.3744922074991));
#41575=CARTESIAN_POINT('Ctrl Pts',(-4.56293527674215,-0.396107766199503,
26.4009495041835));
#41576=CARTESIAN_POINT('Ctrl Pts',(-4.3762612456525,-1.12334284793087,26.427406800868));
#41577=CARTESIAN_POINT('Ctrl Pts',(-4.18958721456285,-1.85057792966224,
26.4538640975524));
#41578=CARTESIAN_POINT('Ctrl Pts',(-3.81771980864998,-2.53027570925048,
26.4803213942369));
#41579=CARTESIAN_POINT('Ctrl Pts',(-3.30595206639681,-3.0796497493845,26.5067786909214));
#41580=CARTESIAN_POINT('Ctrl Pts',(-2.79418432414364,-3.62902378951853,
26.5332359876059));
#41581=CARTESIAN_POINT('Ctrl Pts',(-2.14251624555017,-4.04807409019834,
26.5596932842903));
#41582=CARTESIAN_POINT('Ctrl Pts',(-1.43032028136767,-4.28576078857718,
26.5861505809748));
#41583=CARTESIAN_POINT('Ctrl Pts',(-0.718124317185119,-4.52344748695604,
26.6126078776593));
#41584=CARTESIAN_POINT('Ctrl Pts',(0.0545995325864684,-4.57977058303392,
26.6390651743437));
#41585=CARTESIAN_POINT('Ctrl Pts',(0.793734358242524,-4.44786998604306,
26.6655224710282));
#41586=CARTESIAN_POINT('Ctrl Pts',(1.53286918389854,-4.31596938905221,26.6919797677127));
#41587=CARTESIAN_POINT('Ctrl Pts',(2.23841498543902,-3.99584509899264,26.7184370643971));
#41588=CARTESIAN_POINT('Ctrl Pts',(2.82443706508592,-3.52648790010206,26.7448943610816));
#41589=CARTESIAN_POINT('Ctrl Pts',(3.41045914473281,-3.05713070121148,26.7713516577661));
#41590=CARTESIAN_POINT('Ctrl Pts',(3.87695750248613,-2.43854059348989,26.7978089544505));
#41591=CARTESIAN_POINT('Ctrl Pts',(4.1671131546598,-1.74606116744478,26.824266251135));
#41592=CARTESIAN_POINT('Ctrl Pts',(4.39796892664792,-1.19510559829445,26.845316399926));
#41593=CARTESIAN_POINT('Ctrl Pts',(4.51719573188836,-0.59737640031138,26.8663665487171));
#41594=CARTESIAN_POINT('Ctrl Pts',(4.51781182322151,0.000114263439177032,
26.8874166975081));
#41595=CARTESIAN_POINT('Ctrl Pts',(4.51761428595877,-0.000111883206665997,
26.612583302492));
#41596=CARTESIAN_POINT('Ctrl Pts',(4.51781688422861,-0.217752368533235,
26.604916590958));
#41597=CARTESIAN_POINT('Ctrl Pts',(4.50237218377303,-0.435364344536763,
26.5972498794241));
#41598=CARTESIAN_POINT('Ctrl Pts',(4.47103989191871,-0.65066422144523,26.5895831678902));
#41599=CARTESIAN_POINT('Ctrl Pts',(4.36291429755835,-1.39364935846232,26.5631258712058));
#41600=CARTESIAN_POINT('Ctrl Pts',(4.06558451266292,-2.10909987259421,26.5366685745213));
#41601=CARTESIAN_POINT('Ctrl Pts',(3.61526497596852,-2.70987468303106,26.5102112778368));
#41602=CARTESIAN_POINT('Ctrl Pts',(3.16494543927413,-3.31064949346792,26.4837539811524));
#41603=CARTESIAN_POINT('Ctrl Pts',(2.56163615078078,-3.79674860020972,26.4572966844679));
#41604=CARTESIAN_POINT('Ctrl Pts',(1.87881951412572,-4.10896567003641,26.4308393877834));
#41605=CARTESIAN_POINT('Ctrl Pts',(1.19600287747066,-4.4211827398631,26.4043820910989));
#41606=CARTESIAN_POINT('Ctrl Pts',(0.433678892653904,-4.55951777277466,
26.3779247944145));
#41607=CARTESIAN_POINT('Ctrl Pts',(-0.315302222661645,-4.50712171486216,
26.35146749773));
#41608=CARTESIAN_POINT('Ctrl Pts',(-1.06428333797715,-4.45472565694967,
26.3250102010456));
#41609=CARTESIAN_POINT('Ctrl Pts',(-1.79992158379143,-4.21159850821314,
26.2985529043611));
#41610=CARTESIAN_POINT('Ctrl Pts',(-2.43261703591816,-3.80735288629228,
26.2720956076766));
#41611=CARTESIAN_POINT('Ctrl Pts',(-3.06531248804499,-3.40310726437134,
26.2456383109922));
#41612=CARTESIAN_POINT('Ctrl Pts',(-3.59506514648422,-2.83774316926603,
26.2191810143077));
#41613=CARTESIAN_POINT('Ctrl Pts',(-3.95735172373175,-2.18012132205405,
26.1927237176232));
#41614=CARTESIAN_POINT('Ctrl Pts',(-4.31963830097924,-1.52249947484215,
26.1662664209387));
#41615=CARTESIAN_POINT('Ctrl Pts',(-4.51445879703509,-0.772619875523507,
26.1398091242543));
#41616=CARTESIAN_POINT('Ctrl Pts',(-4.51808429109356,-0.0218170293801812,
26.1133518275698));
#41617=CARTESIAN_POINT('Ctrl Pts',(-4.52170978515203,0.728985816763102,
26.0868945308853));
#41618=CARTESIAN_POINT('Ctrl Pts',(-4.33414027721319,1.48071190973118,26.0604372342009));
#41619=CARTESIAN_POINT('Ctrl Pts',(-3.97822152575495,2.1418018433593,26.0339799375164));
#41620=CARTESIAN_POINT('Ctrl Pts',(-3.62230277429665,2.80289177698754,26.0075226408319));
#41621=CARTESIAN_POINT('Ctrl Pts',(-3.09803477931891,3.37334555127578,25.9810653441475));
#41622=CARTESIAN_POINT('Ctrl Pts',(-2.46927280238623,3.78368252785471,25.954608047463));
#41623=CARTESIAN_POINT('Ctrl Pts',(-1.84051082545367,4.19401950443358,25.9281507507785));
#41624=CARTESIAN_POINT('Ctrl Pts',(-1.10725486656624,4.44423968330318,25.9016934540941));
#41625=CARTESIAN_POINT('Ctrl Pts',(-0.358814689999135,4.50386652360371,
25.8752361574096));
#41626=CARTESIAN_POINT('Ctrl Pts',(0.389625486568016,4.56349336390425,25.8487788607251));
#41627=CARTESIAN_POINT('Ctrl Pts',(1.15324988081482,4.43252686563568,25.8223215640406));
#41628=CARTESIAN_POINT('Ctrl Pts',(1.83904988664902,4.1269186033424,25.7958642673562));
#41629=CARTESIAN_POINT('Ctrl Pts',(2.52484989248321,3.82131034104913,25.7694069706717));
#41630=CARTESIAN_POINT('Ctrl Pts',(3.13282550990476,3.34106031473115,25.7429496739873));
#41631=CARTESIAN_POINT('Ctrl Pts',(3.58892598157735,2.74466244608629,25.7164923773028));
#41632=CARTESIAN_POINT('Ctrl Pts',(4.04502645324994,2.14826457744144,25.6900350806183));
#41633=CARTESIAN_POINT('Ctrl Pts',(4.34925177917356,1.43571886646971,25.6635777839338));
#41634=CARTESIAN_POINT('Ctrl Pts',(4.46454765134638,0.693812592170858,25.6371204872494));
#41635=CARTESIAN_POINT('Ctrl Pts',(4.50019044774909,0.464458203445785,25.6289414256636));
#41636=CARTESIAN_POINT('Ctrl Pts',(4.51777748758952,0.232297861633777,25.6207623640778));
#41637=CARTESIAN_POINT('Ctrl Pts',(4.51757373878986,0.000106944042679857,
25.612583302492));
#41638=CARTESIAN_POINT('Origin',(0.,0.,20.5));
#41639=CARTESIAN_POINT('',(4.51805179992706,-6.79869438786201E-5,24.612583302492));
#41640=CARTESIAN_POINT('',(4.51742159705025,6.47500723078405E-5,24.8874166975081));
#41641=CARTESIAN_POINT('',(4.51775,5.53264807684796E-16,20.5));
#41642=CARTESIAN_POINT('Ctrl Pts',(4.51742159705025,6.47500723078405E-5,
24.8874166975081));
#41643=CARTESIAN_POINT('Ctrl Pts',(4.51757480489056,0.3021867342129,24.8980580949565));
#41644=CARTESIAN_POINT('Ctrl Pts',(4.4877169204789,0.604278844221435,24.9086994924049));
#41645=CARTESIAN_POINT('Ctrl Pts',(4.42754861718235,0.90020824628754,24.9193408898533));
#41646=CARTESIAN_POINT('Ctrl Pts',(4.27795448172836,1.63596612264488,24.9457981865378));
#41647=CARTESIAN_POINT('Ctrl Pts',(3.94099660709531,2.33362924326996,24.9722554832222));
#41648=CARTESIAN_POINT('Ctrl Pts',(3.4577160894917,2.90822301219621,24.9987127799067));
#41649=CARTESIAN_POINT('Ctrl Pts',(2.97443557188809,3.48281678112246,25.0251700765912));
#41650=CARTESIAN_POINT('Ctrl Pts',(2.34483241131392,3.93434119834988,25.0516273732757));
#41651=CARTESIAN_POINT('Ctrl Pts',(1.64559157592564,4.20780108957635,25.0780846699601));
#41652=CARTESIAN_POINT('Ctrl Pts',(0.946350740537367,4.48126098080282,25.1045419666446));
#41653=CARTESIAN_POINT('Ctrl Pts',(0.177472230334982,4.57665634602833,25.1309992633291));
#41654=CARTESIAN_POINT('Ctrl Pts',(-0.567395403080719,4.48236813534545,
25.1574565600135));
#41655=CARTESIAN_POINT('Ctrl Pts',(-1.31226303649646,4.38807992466257,25.183913856698));
#41656=CARTESIAN_POINT('Ctrl Pts',(-2.03311979312552,4.10410813807126,25.2103711533825));
#41657=CARTESIAN_POINT('Ctrl Pts',(-2.64216611780515,3.66504022489793,25.2368284500669));
#41658=CARTESIAN_POINT('Ctrl Pts',(-3.25121244248478,3.22597231172459,25.2632857467514));
#41659=CARTESIAN_POINT('Ctrl Pts',(-3.74844833521498,2.63180827196922,25.2897430434359));
#41660=CARTESIAN_POINT('Ctrl Pts',(-4.07331101456769,1.95491662809413,25.3162003401203));
#41661=CARTESIAN_POINT('Ctrl Pts',(-4.39817369392037,1.27802498421911,25.3426576368048));
#41662=CARTESIAN_POINT('Ctrl Pts',(-4.55066315989561,0.518405736224393,
25.3691149334893));
#41663=CARTESIAN_POINT('Ctrl Pts',(-4.51220636430247,-0.231420332178628,
25.3955722301737));
#41664=CARTESIAN_POINT('Ctrl Pts',(-4.47374956870933,-0.981246400581734,
25.4220295268582));
#41665=CARTESIAN_POINT('Ctrl Pts',(-4.24434651154778,-1.72127928939314,
25.4484868235427));
#41666=CARTESIAN_POINT('Ctrl Pts',(-3.85193823129256,-2.36138381177311,
25.4749441202271));
#41667=CARTESIAN_POINT('Ctrl Pts',(-3.45952995103737,-3.00148833415305,
25.5014014169116));
#41668=CARTESIAN_POINT('Ctrl Pts',(-2.90411644768853,-3.54166449010157,
25.5278587135961));
#41669=CARTESIAN_POINT('Ctrl Pts',(-2.25334647126047,-3.91611942165396,
25.5543160102806));
#41670=CARTESIAN_POINT('Ctrl Pts',(-1.60257649483241,-4.29057435320635,
25.580773306965));
#41671=CARTESIAN_POINT('Ctrl Pts',(-0.856450045325122,-4.49930806036262,
25.6072306036495));
#41672=CARTESIAN_POINT('Ctrl Pts',(-0.105844498527155,-4.51689700860324,
25.6336879003339));
#41673=CARTESIAN_POINT('Ctrl Pts',(0.644761048270813,-4.53448595684386,
25.6601451970184));
#41674=CARTESIAN_POINT('Ctrl Pts',(1.39984569235946,-4.36093014616883,25.6866024937029));
#41675=CARTESIAN_POINT('Ctrl Pts',(2.06744095976455,-4.01736848223874,25.7130597903874));
#41676=CARTESIAN_POINT('Ctrl Pts',(2.73503622716964,-3.67380681830865,25.7395170870718));
#41677=CARTESIAN_POINT('Ctrl Pts',(3.31514211789117,-3.16023930112349,25.7659743837563));
#41678=CARTESIAN_POINT('Ctrl Pts',(3.73710237646057,-2.53921788589521,25.7924316804407));
#41679=CARTESIAN_POINT('Ctrl Pts',(4.15906263502999,-1.9181964706669,25.8188889771252));
#41680=CARTESIAN_POINT('Ctrl Pts',(4.42287726144725,-1.18972115739545,25.8453462738097));
#41681=CARTESIAN_POINT('Ctrl Pts',(4.49641392618663,-0.442519433010954,
25.8718035704942));
#41682=CARTESIAN_POINT('Ctrl Pts',(4.51087921466574,-0.295538487742104,
25.8770079461655));
#41683=CARTESIAN_POINT('Ctrl Pts',(4.51798184168639,-0.147832938193592,
25.8822123218368));
#41684=CARTESIAN_POINT('Ctrl Pts',(4.51783003468408,-0.000112853895665516,
25.8874166975081));
#41685=CARTESIAN_POINT('Ctrl Pts',(4.51757373878986,0.000106944042679857,
25.612583302492));
#41686=CARTESIAN_POINT('Ctrl Pts',(4.51711840923619,-0.518783901194552,
25.5943050673933));
#41687=CARTESIAN_POINT('Ctrl Pts',(4.42781321686835,-1.03782744645157,25.5760268322946));
#41688=CARTESIAN_POINT('Ctrl Pts',(4.25261539535607,-1.52604847346927,25.557748597196));
#41689=CARTESIAN_POINT('Ctrl Pts',(3.99902084877091,-2.2327364271846,25.5312913005115));
#41690=CARTESIAN_POINT('Ctrl Pts',(3.56546533717857,-2.87484549698929,25.504834003827));
#41691=CARTESIAN_POINT('Ctrl Pts',(3.00475544206156,-3.3741675088233,25.4783767071426));
#41692=CARTESIAN_POINT('Ctrl Pts',(2.44404554694452,-3.87348952065733,25.4519194104581));
#41693=CARTESIAN_POINT('Ctrl Pts',(1.7561812683028,-4.23002447452067,25.4254621137736));
#41694=CARTESIAN_POINT('Ctrl Pts',(1.0249437139941,-4.40034680762112,25.3990048170892));
#41695=CARTESIAN_POINT('Ctrl Pts',(0.293706159685441,-4.57066914072155,
25.3725475204047));
#41696=CARTESIAN_POINT('Ctrl Pts',(-0.4809046702902,-4.55477885305912,25.3460902237202));
#41697=CARTESIAN_POINT('Ctrl Pts',(-1.20454203412779,-4.35461136408482,
25.3196329270358));
#41698=CARTESIAN_POINT('Ctrl Pts',(-1.92817939796537,-4.15444387511052,
25.2931756303513));
#41699=CARTESIAN_POINT('Ctrl Pts',(-2.60084329566491,-3.76999918482436,
25.2667183336669));
#41700=CARTESIAN_POINT('Ctrl Pts',(-3.14060400894472,-3.24810223102625,
25.2402610369824));
#41701=CARTESIAN_POINT('Ctrl Pts',(-3.68036472222457,-2.72620527722811,
25.2138037402979));
#41702=CARTESIAN_POINT('Ctrl Pts',(-4.08722225108469,-2.066856059918,25.1873464436134));
#41703=CARTESIAN_POINT('Ctrl Pts',(-4.31162179879184,-1.35036258404192,
25.1608891469289));
#41704=CARTESIAN_POINT('Ctrl Pts',(-4.53602134649897,-0.633869108165933,
25.1344318502445));
#41705=CARTESIAN_POINT('Ctrl Pts',(-4.57796291305318,0.139768626276003,
25.1079745535601));
#41706=CARTESIAN_POINT('Ctrl Pts',(-4.4323380620662,0.876322399437911,25.0815172568756));
#41707=CARTESIAN_POINT('Ctrl Pts',(-4.28671321107921,1.6128761725999,25.0550599601911));
#41708=CARTESIAN_POINT('Ctrl Pts',(-3.95352194255099,2.31234598448186,25.0286026635066));
#41709=CARTESIAN_POINT('Ctrl Pts',(-3.4733465842351,2.88953718612163,25.0021453668221));
#41710=CARTESIAN_POINT('Ctrl Pts',(-2.99317122591925,3.46672838776137,24.9756880701377));
#41711=CARTESIAN_POINT('Ctrl Pts',(-2.36601177781574,3.92164097915893,24.9492307734532));
#41712=CARTESIAN_POINT('Ctrl Pts',(-1.66825556660664,4.19886711014808,24.9227734767688));
#41713=CARTESIAN_POINT('Ctrl Pts',(-0.970499355397546,4.47609324113723,
24.8963161800843));
#41714=CARTESIAN_POINT('Ctrl Pts',(-0.202146381082855,4.57563291171796,
24.8698588833998));
#41715=CARTESIAN_POINT('Ctrl Pts',(0.543218814426126,4.4853623001772,24.8434015867153));
#41716=CARTESIAN_POINT('Ctrl Pts',(1.28858400993515,4.39509168863642,24.8169442900309));
#41717=CARTESIAN_POINT('Ctrl Pts',(2.01096142663846,4.11501079497414,24.7904869933464));
#41718=CARTESIAN_POINT('Ctrl Pts',(2.62236629465924,3.67923316206414,24.7640296966619));
#41719=CARTESIAN_POINT('Ctrl Pts',(3.23377116267999,3.24345552915417,24.7375723999775));
#41720=CARTESIAN_POINT('Ctrl Pts',(3.73420348201823,2.65198115699651,24.711115103293));
#41721=CARTESIAN_POINT('Ctrl Pts',(4.06271115002261,1.97685096951678,24.6846578066085));
#41722=CARTESIAN_POINT('Ctrl Pts',(4.36101609468216,1.3637916931913,24.660632971903));
#41723=CARTESIAN_POINT('Ctrl Pts',(4.51755636187948,0.681751967669245,24.6366081371975));
#41724=CARTESIAN_POINT('Ctrl Pts',(4.51805179992706,-6.79869438786201E-5,
24.612583302492));
#41725=CARTESIAN_POINT('Origin',(0.,0.,20.5));
#41726=CARTESIAN_POINT('',(4.5173631353831,-4.88662610135722E-6,23.612583302492));
#41727=CARTESIAN_POINT('',(4.51813699104787,9.0065690785813E-7,23.8874166975081));
#41728=CARTESIAN_POINT('',(4.51775,5.53264807684796E-16,20.5));
#41729=CARTESIAN_POINT('Ctrl Pts',(4.51813695063288,9.0056284873609E-7,
23.8874166975081));
#41730=CARTESIAN_POINT('Ctrl Pts',(4.51814591729222,0.751660275924123,23.9139038680762));
#41731=CARTESIAN_POINT('Ctrl Pts',(4.32649937043261,1.5033152188212,23.9403910386443));
#41732=CARTESIAN_POINT('Ctrl Pts',(3.96661538289285,2.16322075812818,23.9668782092125));
#41733=CARTESIAN_POINT('Ctrl Pts',(3.6071372949696,2.8223820147924,23.9933355058969));
#41734=CARTESIAN_POINT('Ctrl Pts',(3.07980110896882,3.39000071259223,24.0197928025814));
#41735=CARTESIAN_POINT('Ctrl Pts',(2.44883578872663,3.7969415223372,24.0462500992659));
#41736=CARTESIAN_POINT('Ctrl Pts',(1.81787046848448,4.20388233208215,24.0727073959503));
#41737=CARTESIAN_POINT('Ctrl Pts',(1.08327601400093,4.45014525377226,24.0991646926348));
#41738=CARTESIAN_POINT('Ctrl Pts',(0.334525216833109,4.50573573609242,24.1256219893193));
#41739=CARTESIAN_POINT('Ctrl Pts',(-0.414225580334709,4.56132621841258,
24.1520792860037));
#41740=CARTESIAN_POINT('Ctrl Pts',(-1.17713272018679,4.4262442613628,24.1785365826882));
#41741=CARTESIAN_POINT('Ctrl Pts',(-1.86127495742213,4.11694269781237,24.2049938793727));
#41742=CARTESIAN_POINT('Ctrl Pts',(-2.54541719465748,3.80764113426195,24.2314511760572));
#41743=CARTESIAN_POINT('Ctrl Pts',(-3.15079452927609,3.32411996421088,24.2579084727416));
#41744=CARTESIAN_POINT('Ctrl Pts',(-3.6036726719115,2.72527153104338,24.2843657694261));
#41745=CARTESIAN_POINT('Ctrl Pts',(-4.05655081454692,2.12642309787588,24.3108230661106));
#41746=CARTESIAN_POINT('Ctrl Pts',(-4.35692976519914,1.41224740159195,24.337280362795));
#41747=CARTESIAN_POINT('Ctrl Pts',(-4.46822370011745,0.669730251598438,
24.3637376594795));
#41748=CARTESIAN_POINT('Ctrl Pts',(-4.57951763503577,-0.0727868983951169,
24.390194956164));
#41749=CARTESIAN_POINT('Ctrl Pts',(-4.50172655422016,-0.843645502098255,
24.4166522528484));
#41750=CARTESIAN_POINT('Ctrl Pts',(-4.24432532522016,-1.54895583471323,
24.4431095495329));
#41751=CARTESIAN_POINT('Ctrl Pts',(-3.98692409622017,-2.25426616732816,
24.4695668462174));
#41752=CARTESIAN_POINT('Ctrl Pts',(-3.54991271903582,-2.89402822885493,
24.4960241429018));
#41753=CARTESIAN_POINT('Ctrl Pts',(-2.98651869575401,-3.39031970824422,
24.5224814395863));
#41754=CARTESIAN_POINT('Ctrl Pts',(-2.42312467247219,-3.88661118763352,
24.5489387362708));
#41755=CARTESIAN_POINT('Ctrl Pts',(-1.73334800309291,-4.23943208488534,
24.5753960329552));
#41756=CARTESIAN_POINT('Ctrl Pts',(-1.00120272254919,-4.40580920519233,
24.6018533296397));
#41757=CARTESIAN_POINT('Ctrl Pts',(-0.269057442005433,-4.57218632549932,
24.6283106263242));
#41758=CARTESIAN_POINT('Ctrl Pts',(0.505456449702776,-4.55211966886146,
24.6547679230086));
#41759=CARTESIAN_POINT('Ctrl Pts',(1.22800401774408,-4.34805333184884,24.6812252196931));
#41760=CARTESIAN_POINT('Ctrl Pts',(1.95055158578534,-4.14398699483623,24.7076825163776));
#41761=CARTESIAN_POINT('Ctrl Pts',(2.6211328301597,-3.75592097744887,24.7341398130621));
#41762=CARTESIAN_POINT('Ctrl Pts',(3.15807169745557,-3.23112129111977,24.7605971097465));
#41763=CARTESIAN_POINT('Ctrl Pts',(3.69501056475143,-2.70632160479067,24.787054406431));
#41764=CARTESIAN_POINT('Ctrl Pts',(4.0983070549688,-2.04478824951983,24.8135117031154));
#41765=CARTESIAN_POINT('Ctrl Pts',(4.31884010194003,-1.32709525583961,24.8399689997999));
#41766=CARTESIAN_POINT('Ctrl Pts',(4.45067248416388,-0.898065782199879,
24.855784899036));
#41767=CARTESIAN_POINT('Ctrl Pts',(4.51719389013711,-0.448967520484957,
24.871600798272));
#41768=CARTESIAN_POINT('Ctrl Pts',(4.51742159705025,6.47500723078405E-5,
24.8874166975081));
#41769=CARTESIAN_POINT('Ctrl Pts',(4.51805179992706,-6.79869438786201E-5,
24.612583302492));
#41770=CARTESIAN_POINT('Ctrl Pts',(4.51810196194601,-0.0691007664161157,
24.610150840513));
#41771=CARTESIAN_POINT('Ctrl Pts',(4.51655248974293,-0.13813129299046,24.6077183785341));
#41772=CARTESIAN_POINT('Ctrl Pts',(4.51338856189906,-0.207087743519482,
24.6052859165551));
#41773=CARTESIAN_POINT('Ctrl Pts',(4.47897528910062,-0.957110266274211,
24.5788286198707));
#41774=CARTESIAN_POINT('Ctrl Pts',(4.25356572683319,-1.69836930898188,24.5523713231862));
#41775=CARTESIAN_POINT('Ctrl Pts',(3.8646145103131,-2.3405803406153,24.5259140265017));
#41776=CARTESIAN_POINT('Ctrl Pts',(3.47566329379301,-2.98279137224871,24.4994567298173));
#41777=CARTESIAN_POINT('Ctrl Pts',(2.92317042302025,-3.52595439280789,24.4729994331328));
#41778=CARTESIAN_POINT('Ctrl Pts',(2.27442891819395,-3.90391274752403,24.4465421364483));
#41779=CARTESIAN_POINT('Ctrl Pts',(1.62568741336761,-4.2818711022402,24.4200848397639));
#41780=CARTESIAN_POINT('Ctrl Pts',(0.88069727448771,-4.49462479111332,24.3936275430794));
#41781=CARTESIAN_POINT('Ctrl Pts',(0.130197475965773,-4.51626065030008,
24.3671702463949));
#41782=CARTESIAN_POINT('Ctrl Pts',(-0.620302322556121,-4.53789650948684,
24.3407129497104));
#41783=CARTESIAN_POINT('Ctrl Pts',(-1.37631178072007,-4.36841453898727,
24.314255653026));
#41784=CARTESIAN_POINT('Ctrl Pts',(-2.04574978322055,-4.02845745523667,
24.2877983563415));
#41785=CARTESIAN_POINT('Ctrl Pts',(-2.71518778572104,-3.68850037148608,
24.2613410596571));
#41786=CARTESIAN_POINT('Ctrl Pts',(-3.29805433255807,-3.17806817448446,
24.2348837629726));
#41787=CARTESIAN_POINT('Ctrl Pts',(-3.72335692340428,-2.55933094091641,
24.2084264662881));
#41788=CARTESIAN_POINT('Ctrl Pts',(-4.14865951425051,-1.94059370734831,
24.1819691696036));
#41789=CARTESIAN_POINT('Ctrl Pts',(-4.41639814910591,-1.21355143721374,
24.1555118729192));
#41790=CARTESIAN_POINT('Ctrl Pts',(-4.49396255855832,-0.466757074372799,
24.1290545762347));
#41791=CARTESIAN_POINT('Ctrl Pts',(-4.57152696801073,0.280037288468098,
24.1025972795502));
#41792=CARTESIAN_POINT('Ctrl Pts',(-4.4589171520602,1.04658374401527,24.0761399828658));
#41793=CARTESIAN_POINT('Ctrl Pts',(-4.16984886166344,1.73951778234053,24.0496826861813));
#41794=CARTESIAN_POINT('Ctrl Pts',(-3.88078057126667,2.43245182066584,24.0232253894968));
#41795=CARTESIAN_POINT('Ctrl Pts',(-3.41525380642364,3.05177344176913,23.9967680928124));
#41796=CARTESIAN_POINT('Ctrl Pts',(-2.82996921187404,3.52204995762946,23.9703107961279));
#41797=CARTESIAN_POINT('Ctrl Pts',(-2.24468461732448,3.99232647348976,23.9438534994434));
#41798=CARTESIAN_POINT('Ctrl Pts',(-1.53964219306833,4.31355788410714,23.917396202759));
#41799=CARTESIAN_POINT('Ctrl Pts',(-0.800715326097399,4.44661855917222,
23.8909389060745));
#41800=CARTESIAN_POINT('Ctrl Pts',(-0.0617884591264724,4.5796792342373,
23.86448160939));
#41801=CARTESIAN_POINT('Ctrl Pts',(0.711022850559258,4.5245691737501,23.8380243127056));
#41802=CARTESIAN_POINT('Ctrl Pts',(1.42359104075306,4.28800072211045,23.8115670160211));
#41803=CARTESIAN_POINT('Ctrl Pts',(2.13615923094691,4.05143227047079,23.7851097193366));
#41804=CARTESIAN_POINT('Ctrl Pts',(2.78848430164884,3.63340542767864,23.7586524226522));
#41805=CARTESIAN_POINT('Ctrl Pts',(3.30111378116074,3.08483540049647,23.7321951259677));
#41806=CARTESIAN_POINT('Ctrl Pts',(3.81374326067261,2.53626537331434,23.7057378292832));
#41807=CARTESIAN_POINT('Ctrl Pts',(4.18667714899447,1.85715216174218,23.6792805325988));
#41808=CARTESIAN_POINT('Ctrl Pts',(4.37449251133263,1.13021100344109,23.6528232359143));
#41809=CARTESIAN_POINT('Ctrl Pts',(4.46971107890219,0.761666625925485,23.6394099247735));
#41810=CARTESIAN_POINT('Ctrl Pts',(4.51734893340559,0.380829109202114,23.6259966136328));
#41811=CARTESIAN_POINT('Ctrl Pts',(4.51736327228765,-4.88489681080284E-6,
23.612583302492));
#41812=CARTESIAN_POINT('Origin',(0.,0.,20.5));
#41813=CARTESIAN_POINT('',(4.51802736372575,7.65320072124154E-5,22.612583302492));
#41814=CARTESIAN_POINT('',(4.51742427980126,-6.60698246896739E-5,22.8874166975081));
#41815=CARTESIAN_POINT('',(4.51775,5.53264807684796E-16,20.5));
#41816=CARTESIAN_POINT('Ctrl Pts',(4.51742427980126,-6.60698246896739E-5,
22.8874166975081));
#41817=CARTESIAN_POINT('Ctrl Pts',(4.51719087600353,0.450661745130009,22.9032923445115));
#41818=CARTESIAN_POINT('Ctrl Pts',(4.450158091451,0.901457458944964,22.9191679915148));
#41819=CARTESIAN_POINT('Ctrl Pts',(4.31734276296,1.3319583722546,22.9350436385182));
#41820=CARTESIAN_POINT('Ctrl Pts',(4.09600157608532,2.04940254217993,22.9615009352027));
#41821=CARTESIAN_POINT('Ctrl Pts',(3.69196031163168,2.71048127828687,22.9879582318872));
#41822=CARTESIAN_POINT('Ctrl Pts',(3.15443074594463,3.23467592132643,23.0144155285716));
#41823=CARTESIAN_POINT('Ctrl Pts',(2.61690118025762,3.75887056436596,23.0408728252561));
#41824=CARTESIAN_POINT('Ctrl Pts',(1.94588331333721,4.14618111433815,23.0673301219406));
#41825=CARTESIAN_POINT('Ctrl Pts',(1.22310638006181,4.34943357534335,23.093787418625));
#41826=CARTESIAN_POINT('Ctrl Pts',(0.500329446786407,4.55268603634856,23.1202447153095));
#41827=CARTESIAN_POINT('Ctrl Pts',(-0.274206552844009,4.5718804083868,23.146702011994));
#41828=CARTESIAN_POINT('Ctrl Pts',(-1.00616399197876,4.4046788379547,23.1731593086784));
#41829=CARTESIAN_POINT('Ctrl Pts',(-1.73812143111355,4.23747726752258,23.1996166053629));
#41830=CARTESIAN_POINT('Ctrl Pts',(-2.4275003097527,3.88387975462009,23.2260739020474));
#41831=CARTESIAN_POINT('Ctrl Pts',(-2.99033504306372,3.38695408510429,23.2525311987318));
#41832=CARTESIAN_POINT('Ctrl Pts',(-3.55316977637471,2.89002841558852,23.2789884954163));
#41833=CARTESIAN_POINT('Ctrl Pts',(-3.98946036435762,2.24977458945944,23.3054457921008));
#41834=CARTESIAN_POINT('Ctrl Pts',(-4.24606709644918,1.54417481408558,23.3319030887853));
#41835=CARTESIAN_POINT('Ctrl Pts',(-4.50267382854076,0.838575038711681,
23.3583603854697));
#41836=CARTESIAN_POINT('Ctrl Pts',(-4.57959670474098,0.0676293140930979,
23.3848176821541));
#41837=CARTESIAN_POINT('Ctrl Pts',(-4.46746660375748,-0.674762023707061,
23.4112749788386));
#41838=CARTESIAN_POINT('Ctrl Pts',(-4.35533650277398,-1.41715336150718,
23.4377322755231));
#41839=CARTESIAN_POINT('Ctrl Pts',(-4.05415342460676,-2.13099031248878,
23.4641895722076));
#41840=CARTESIAN_POINT('Ctrl Pts',(-3.60060113490302,-2.72932832606618,
23.4906468688921));
#41841=CARTESIAN_POINT('Ctrl Pts',(-3.14704884519929,-3.32766633964359,
23.5171041655765));
#41842=CARTESIAN_POINT('Ctrl Pts',(-2.54112734395902,-3.81050541581682,
23.543561462261));
#41843=CARTESIAN_POINT('Ctrl Pts',(-1.85663719941186,-4.11903628947138,
23.5700187589454));
#41844=CARTESIAN_POINT('Ctrl Pts',(-1.17214705486469,-4.42756716312594,
23.5964760556299));
#41845=CARTESIAN_POINT('Ctrl Pts',(-0.409088267010601,-4.56178983426184,
23.6229333523144));
#41846=CARTESIAN_POINT('Ctrl Pts',(0.339599448275288,-4.50535613008826,
23.6493906489989));
#41847=CARTESIAN_POINT('Ctrl Pts',(1.08828716356118,-4.44892242591468,23.6758479456834));
#41848=CARTESIAN_POINT('Ctrl Pts',(1.82260380627889,-4.20183234643162,23.7023052423678));
#41849=CARTESIAN_POINT('Ctrl Pts',(2.45311042204474,-3.7941811898551,23.7287625390522));
#41850=CARTESIAN_POINT('Ctrl Pts',(3.08361703781062,-3.38653003327857,23.7552198357367));
#41851=CARTESIAN_POINT('Ctrl Pts',(3.61031362662464,-2.81831779960855,23.7816771324212));
#41852=CARTESIAN_POINT('Ctrl Pts',(3.96904912687646,-2.15875211004929,23.8081344291057));
#41853=CARTESIAN_POINT('Ctrl Pts',(4.32737956599415,-1.49993115979256,23.8345618519065));
#41854=CARTESIAN_POINT('Ctrl Pts',(4.51812800419987,-0.749962938110063,
23.8609892747073));
#41855=CARTESIAN_POINT('Ctrl Pts',(4.51813695063288,9.0056284873609E-7,
23.8874166975081));
#41856=CARTESIAN_POINT('Ctrl Pts',(4.51736327228765,-4.88489681080284E-6,
23.612583302492));
#41857=CARTESIAN_POINT('Ctrl Pts',(4.51737721635919,-0.370352896766723,
23.5995393169483));
#41858=CARTESIAN_POINT('Ctrl Pts',(4.47235409625982,-0.740697577327283,
23.5864953314046));
#41859=CARTESIAN_POINT('Ctrl Pts',(4.38225454858748,-1.09973029228254,23.5734513458609));
#41860=CARTESIAN_POINT('Ctrl Pts',(4.19950438714968,-1.82796132467507,23.5469940491764));
#41861=CARTESIAN_POINT('Ctrl Pts',(3.83130722791959,-2.50965428443002,23.5205367524919));
#41862=CARTESIAN_POINT('Ctrl Pts',(3.3225090776327,-3.06177972318861,23.4940794558075));
#41863=CARTESIAN_POINT('Ctrl Pts',(2.81371092734586,-3.61390516194714,23.467622159123));
#41864=CARTESIAN_POINT('Ctrl Pts',(2.16431178600224,-4.03646307970933,23.4411648624385));
#41865=CARTESIAN_POINT('Ctrl Pts',(1.45340774986053,-4.27798639033802,23.4147075657541));
#41866=CARTESIAN_POINT('Ctrl Pts',(0.742503713718783,-4.51950970096672,
23.3882502690696));
#41867=CARTESIAN_POINT('Ctrl Pts',(-0.0299052172210591,-4.5799984044619,
23.3617929723851));
#41868=CARTESIAN_POINT('Ctrl Pts',(-0.769740489176251,-4.4520850425719,
23.3353356757007));
#41869=CARTESIAN_POINT('Ctrl Pts',(-1.50957576113144,-4.32417168068191,
23.3088783790162));
#41870=CARTESIAN_POINT('Ctrl Pts',(-2.21683737410199,-4.00785625340675,
23.2824210823318));
#41871=CARTESIAN_POINT('Ctrl Pts',(-2.80538164796902,-3.54166563180954,
23.2559637856473));
#41872=CARTESIAN_POINT('Ctrl Pts',(-3.39392592183609,-3.0754750102123,23.2295064889628));
#41873=CARTESIAN_POINT('Ctrl Pts',(-3.86375285659963,-2.459409194293,23.2030491922783));
#41874=CARTESIAN_POINT('Ctrl Pts',(-4.15763804857074,-1.76850431465145,
23.1765918955939));
#41875=CARTESIAN_POINT('Ctrl Pts',(-4.45152324054182,-1.07759943500997,
23.1501345989094));
#41876=CARTESIAN_POINT('Ctrl Pts',(-4.56946668972051,-0.311855491646258,
23.123677302225));
#41877=CARTESIAN_POINT('Ctrl Pts',(-4.49710302020607,0.435460743133651,
23.0972200055405));
#41878=CARTESIAN_POINT('Ctrl Pts',(-4.42473935069162,1.18277697791365,23.070762708856));
#41879=CARTESIAN_POINT('Ctrl Pts',(-4.162068562484,1.91166550410983,23.0443054121715));
#41880=CARTESIAN_POINT('Ctrl Pts',(-3.74108365616062,2.53334852003347,23.017848115487));
#41881=CARTESIAN_POINT('Ctrl Pts',(-3.32009874983724,3.15503153595711,22.9913908188026));
#41882=CARTESIAN_POINT('Ctrl Pts',(-2.74079972539808,3.66950904160819,22.9649335221181));
#41883=CARTESIAN_POINT('Ctrl Pts',(-2.07374458313369,4.01411821952858,22.9384762254337));
#41884=CARTESIAN_POINT('Ctrl Pts',(-1.40668944086933,4.35872739744894,22.9120189287492));
#41885=CARTESIAN_POINT('Ctrl Pts',(-0.651878180779734,4.53346824763863,
22.8855616320647));
#41886=CARTESIAN_POINT('Ctrl Pts',(0.0987540592506666,4.51705757827173,
22.8591043353802));
#41887=CARTESIAN_POINT('Ctrl Pts',(0.849386299281067,4.50064690890482,22.8326470386958));
#41888=CARTESIAN_POINT('Ctrl Pts',(1.59583951925228,4.29308471998132,22.8061897420113));
#41889=CARTESIAN_POINT('Ctrl Pts',(2.24719647092532,3.91965176135188,22.7797324453269));
#41890=CARTESIAN_POINT('Ctrl Pts',(2.89855342259837,3.54621880272245,22.7532751486424));
#41891=CARTESIAN_POINT('Ctrl Pts',(3.45481410597325,3.00691507438708,22.7268178519579));
#41892=CARTESIAN_POINT('Ctrl Pts',(3.8482267217168,2.3674273530564,22.7003605552734));
#41893=CARTESIAN_POINT('Ctrl Pts',(4.24163933746037,1.72793963172568,22.673903258589));
#41894=CARTESIAN_POINT('Ctrl Pts',(4.47220388557259,0.988267917399649,22.6474459619045));
#41895=CARTESIAN_POINT('Ctrl Pts',(4.51183760195935,0.238503067401548,22.6209886652201));
#41896=CARTESIAN_POINT('Ctrl Pts',(4.51603475238966,0.159104107382582,22.618186877644));
#41897=CARTESIAN_POINT('Ctrl Pts',(4.51809071117569,0.0795919580082339,
22.615385090068));
#41898=CARTESIAN_POINT('Ctrl Pts',(4.51802736372575,7.65320072124154E-5,
22.612583302492));
#41899=CARTESIAN_POINT('Origin',(0.,0.,20.5));
#41900=CARTESIAN_POINT('',(4.51732076945549,-0.00048196737157627,21.612583302492));
#41901=CARTESIAN_POINT('',(4.51782520267197,0.000113471772791779,21.8874166975081));
#41902=CARTESIAN_POINT('',(4.51775,5.53264807684796E-16,20.5));
#41903=CARTESIAN_POINT('Ctrl Pts',(4.51782520267197,0.000113471772791779,
21.8874166975081));
#41904=CARTESIAN_POINT('Ctrl Pts',(4.51797972979194,0.149530198200455,21.8926808209467));
#41905=CARTESIAN_POINT('Ctrl Pts',(4.51071347097486,0.298931999583376,21.8979449443854));
#41906=CARTESIAN_POINT('Ctrl Pts',(4.49591510340165,0.447583892947329,21.903209067824));
#41907=CARTESIAN_POINT('Ctrl Pts',(4.4215390356869,1.19470300808371,21.9296663645084));
#41908=CARTESIAN_POINT('Ctrl Pts',(4.15689950898611,1.92287920852908,21.9561236611929));
#41909=CARTESIAN_POINT('Ctrl Pts',(3.73423901960025,2.54342464869698,21.9825809578774));
#41910=CARTESIAN_POINT('Ctrl Pts',(3.3115785302144,3.16397008886483,22.0090382545618));
#41911=CARTESIAN_POINT('Ctrl Pts',(2.7308970781435,3.67688476875521,22.0354955512463));
#41912=CARTESIAN_POINT('Ctrl Pts',(2.06291588716907,4.0196945481291,22.0619528479308));
#41913=CARTESIAN_POINT('Ctrl Pts',(1.39493469619467,4.36250432750298,22.0884101446153));
#41914=CARTESIAN_POINT('Ctrl Pts',(0.639653766316767,4.53520920636039,22.1148674412997));
#41915=CARTESIAN_POINT('Ctrl Pts',(-0.110931801888053,4.51677482186132,
22.1413247379842));
#41916=CARTESIAN_POINT('Ctrl Pts',(-0.861517370093001,4.49834043736225,
22.1677820346687));
#41917=CARTESIAN_POINT('Ctrl Pts',(-1.60740757662484,4.28876678950664,22.1942393313531));
#41918=CARTESIAN_POINT('Ctrl Pts',(-2.25775525993264,3.91357923987666,22.2206966280376));
#41919=CARTESIAN_POINT('Ctrl Pts',(-2.90810294324037,3.53839169024672,22.2471539247221));
#41920=CARTESIAN_POINT('Ctrl Pts',(-3.46290810332406,2.99759023884246,22.2736112214065));
#41921=CARTESIAN_POINT('Ctrl Pts',(-3.85459532302061,2.35704415643024,22.300068518091));
#41922=CARTESIAN_POINT('Ctrl Pts',(-4.24628254271713,1.71649807401806,22.3265258147755));
#41923=CARTESIAN_POINT('Ctrl Pts',(-4.4748518220265,0.976207360597959,22.3529831114599));
#41924=CARTESIAN_POINT('Ctrl Pts',(-4.51246407961468,0.226338472032797,
22.3794404081444));
#41925=CARTESIAN_POINT('Ctrl Pts',(-4.55007633720287,-0.523530416532452,
22.4058977048289));
#41926=CARTESIAN_POINT('Ctrl Pts',(-4.39673157306978,-1.28297748024285,
22.4323550015133));
#41927=CARTESIAN_POINT('Ctrl Pts',(-4.07110679585725,-1.95950283641873,
22.4588122981978));
#41928=CARTESIAN_POINT('Ctrl Pts',(-3.74548201864475,-2.63602819259453,
22.4852695948823));
#41929=CARTESIAN_POINT('Ctrl Pts',(-3.24757722835284,-3.22963184123592,
22.5117268915668));
#41930=CARTESIAN_POINT('Ctrl Pts',(-2.63803679068419,-3.66801355240642,
22.5381841882512));
#41931=CARTESIAN_POINT('Ctrl Pts',(-2.02849635301547,-4.10639526357697,
22.5646414849357));
#41932=CARTESIAN_POINT('Ctrl Pts',(-1.30732026797,-4.38955503727659,22.5910987816201));
#41933=CARTESIAN_POINT('Ctrl Pts',(-0.562346924558367,-4.48300430658586,
22.6175560783046));
#41934=CARTESIAN_POINT('Ctrl Pts',(0.182626418853268,-4.57645357589513,
22.6440133749891));
#41935=CARTESIAN_POINT('Ctrl Pts',(0.951397020631046,-4.48019234081406,
22.6704706716736));
#41936=CARTESIAN_POINT('Ctrl Pts',(1.65032944052472,-4.20594512376056,22.696927968358));
#41937=CARTESIAN_POINT('Ctrl Pts',(2.34926186041832,-3.93169790670708,22.7233852650425));
#41938=CARTESIAN_POINT('Ctrl Pts',(2.97835609842781,-3.47946470768123,22.749842561727));
#41939=CARTESIAN_POINT('Ctrl Pts',(3.46098918943069,-2.90432702425209,22.7762998584114));
#41940=CARTESIAN_POINT('Ctrl Pts',(3.94362228043359,-2.32918934082292,22.8027571550959));
#41941=CARTESIAN_POINT('Ctrl Pts',(4.27979422442984,-1.63114717299047,22.8292144517804));
#41942=CARTESIAN_POINT('Ctrl Pts',(4.42855964178011,-0.89522128720241,22.8556717484648));
#41943=CARTESIAN_POINT('Ctrl Pts',(4.48805867336429,-0.600886230695128,
22.8662533981459));
#41944=CARTESIAN_POINT('Ctrl Pts',(4.51757985123852,-0.300491232865703,
22.876835047827));
#41945=CARTESIAN_POINT('Ctrl Pts',(4.51742427980126,-6.60698246896739E-5,
22.8874166975081));
#41946=CARTESIAN_POINT('Ctrl Pts',(4.51802736372575,7.65320072124154E-5,
22.612583302492));
#41947=CARTESIAN_POINT('Ctrl Pts',(4.51749252083047,-0.671272680948583,
22.5889277933835));
#41948=CARTESIAN_POINT('Ctrl Pts',(4.36588431242158,-1.34285546610394,22.5652722842751));
#41949=CARTESIAN_POINT('Ctrl Pts',(4.07637456299432,-1.94852038806885,22.5416167751666));
#41950=CARTESIAN_POINT('Ctrl Pts',(3.75257492298122,-2.62592100787102,22.5151594784822));
#41951=CARTESIAN_POINT('Ctrl Pts',(3.2562727582937,-3.22086426180528,22.4887021817977));
#41952=CARTESIAN_POINT('Ctrl Pts',(2.64791620593777,-3.66088792814019,22.4622448851133));
#41953=CARTESIAN_POINT('Ctrl Pts',(2.03955965358178,-4.10091159447515,22.4357875884288));
#41954=CARTESIAN_POINT('Ctrl Pts',(1.31914871355735,-4.38601567321071,22.4093302917443));
#41955=CARTESIAN_POINT('Ctrl Pts',(0.574430373257849,-4.48147252184727,
22.3828729950598));
#41956=CARTESIAN_POINT('Ctrl Pts',(-0.17028796704161,-4.57692937048383,
22.3564156983754));
#41957=CARTESIAN_POINT('Ctrl Pts',(-0.939313707616121,-4.48273898902142,
22.3299584016909));
#41958=CARTESIAN_POINT('Ctrl Pts',(-1.63898363511379,-4.21037796912979,
22.3035011050064));
#41959=CARTESIAN_POINT('Ctrl Pts',(-2.33865356261146,-3.93801694923817,
22.277043808322));
#41960=CARTESIAN_POINT('Ctrl Pts',(-2.96896767703227,-3.48748529091735,
22.2505865116375));
#41961=CARTESIAN_POINT('Ctrl Pts',(-3.4531482409959,-2.91364911818973,22.224129214953));
#41962=CARTESIAN_POINT('Ctrl Pts',(-3.93732880495957,-2.33981294546208,
22.1976719182685));
#41963=CARTESIAN_POINT('Ctrl Pts',(-4.27537581846602,-1.64267225832765,
22.1712146215841));
#41964=CARTESIAN_POINT('Ctrl Pts',(-4.42612719062429,-0.907153378338295,
22.1447573248996));
#41965=CARTESIAN_POINT('Ctrl Pts',(-4.57687856278254,-0.171634498348981,
22.1183000282152));
#41966=CARTESIAN_POINT('Ctrl Pts',(-4.5403342935926,0.602262574495347,22.0918427315307));
#41967=CARTESIAN_POINT('Ctrl Pts',(-4.32092341583129,1.32030703112007,22.0653854348462));
#41968=CARTESIAN_POINT('Ctrl Pts',(-4.10151253806998,2.03835148774475,22.0389281381617));
#41969=CARTESIAN_POINT('Ctrl Pts',(-3.69923505173734,2.70054332814993,22.0124708414773));
#41970=CARTESIAN_POINT('Ctrl Pts',(-3.16312948534619,3.2261735651419,21.9860135447928));
#41971=CARTESIAN_POINT('Ctrl Pts',(-2.62702391895502,3.7518038021339,21.9595562481083));
#41972=CARTESIAN_POINT('Ctrl Pts',(-1.95709027250536,4.14087243571266,21.9330989514239));
#41973=CARTESIAN_POINT('Ctrl Pts',(-1.23484721910289,4.34609472311248,21.9066416547394));
#41974=CARTESIAN_POINT('Ctrl Pts',(-0.512604165700429,4.5513170105123,21.880184358055));
#41975=CARTESIAN_POINT('Ctrl Pts',(0.261948294654812,4.57269295173318,21.8537270613705));
#41976=CARTESIAN_POINT('Ctrl Pts',(0.994322299916156,4.40742376897541,21.827269764686));
#41977=CARTESIAN_POINT('Ctrl Pts',(1.72669630517754,4.24215458621763,21.8008124680015));
#41978=CARTESIAN_POINT('Ctrl Pts',(2.41689185534501,3.89024027948119,21.7743551713171));
#41979=CARTESIAN_POINT('Ctrl Pts',(2.9811237744369,3.39491220205643,21.7478978746326));
#41980=CARTESIAN_POINT('Ctrl Pts',(3.54535569352876,2.8995841246317,21.7214405779481));
#41981=CARTESIAN_POINT('Ctrl Pts',(3.98362398154505,2.26084227651867,21.6949832812637));
#41982=CARTESIAN_POINT('Ctrl Pts',(4.24201965646871,1.55578891217676,21.6685259845792));
#41983=CARTESIAN_POINT('Ctrl Pts',(4.42414140114732,1.05885509606931,21.6498784238835));
#41984=CARTESIAN_POINT('Ctrl Pts',(4.51690828804801,0.528979877711725,21.6312308631877));
#41985=CARTESIAN_POINT('Ctrl Pts',(4.51732076945549,-0.00048196737157627,
21.612583302492));
#41986=CARTESIAN_POINT('Origin',(0.,0.,20.5));
#41987=CARTESIAN_POINT('',(4.52133925202235,0.00376432143610439,20.612583302492));
#41988=CARTESIAN_POINT('',(4.50983715083838,-0.000439487622834945,20.8874166975081));
#41989=CARTESIAN_POINT('',(4.51775,5.53264807684796E-16,20.5));
#41990=CARTESIAN_POINT('Ctrl Pts',(4.50983715083838,-0.000439487622834945,
20.8874166975081));
#41991=CARTESIAN_POINT('Ctrl Pts',(4.51223989494407,0.600272225419278,20.9085265940664));
#41992=CARTESIAN_POINT('Ctrl Pts',(4.40045147683232,1.20075832380094,20.9296364906248));
#41993=CARTESIAN_POINT('Ctrl Pts',(4.16995632188889,1.7527710518725,20.9507463871831));
#41994=CARTESIAN_POINT('Ctrl Pts',(3.88107386896856,2.44461548985082,20.9772036838676));
#41995=CARTESIAN_POINT('Ctrl Pts',(3.40572780474968,3.06031833788172,21.0036609805521));
#41996=CARTESIAN_POINT('Ctrl Pts',(2.81753981467946,3.528620768205,21.0301182772365));
#41997=CARTESIAN_POINT('Ctrl Pts',(2.22935182460931,3.99692319852822,21.056575573921));
#41998=CARTESIAN_POINT('Ctrl Pts',(1.52832190868785,4.31782521114387,21.0830328706055));
#41999=CARTESIAN_POINT('Ctrl Pts',(0.790149843231595,4.44924273175288,21.1094901672899));
#42000=CARTESIAN_POINT('Ctrl Pts',(0.051977777775257,4.58066025236192,21.1359474639744));
#42001=CARTESIAN_POINT('Ctrl Pts',(-0.723336437215882,4.52259328096428,
21.1624047606589));
#42002=CARTESIAN_POINT('Ctrl Pts',(-1.43588412720356,4.28390166798379,21.1888620573433));
#42003=CARTESIAN_POINT('Ctrl Pts',(-2.14843181719121,4.04521005500332,21.2153193540278));
#42004=CARTESIAN_POINT('Ctrl Pts',(-2.7982129821754,3.62589380044002,21.2417766507123));
#42005=CARTESIAN_POINT('Ctrl Pts',(-3.30902952393807,3.07605344225317,21.2682339473967));
#42006=CARTESIAN_POINT('Ctrl Pts',(-3.81984606570073,2.52621308406631,21.2946912440812));
#42007=CARTESIAN_POINT('Ctrl Pts',(-4.19169798424187,1.84584862225589,21.3211485407657));
#42008=CARTESIAN_POINT('Ctrl Pts',(-4.37772925931563,1.11834540158705,21.3476058374502));
#42009=CARTESIAN_POINT('Ctrl Pts',(-4.56376053438938,0.390842180918212,
21.3740631341346));
#42010=CARTESIAN_POINT('Ctrl Pts',(-4.56397116599575,-0.383799798609046,
21.4005204308191));
#42011=CARTESIAN_POINT('Ctrl Pts',(-4.37916492462626,-1.11150455739398,
21.4269777275035));
#42012=CARTESIAN_POINT('Ctrl Pts',(-4.19435868325677,-1.83920931617892,
21.453435024188));
#42013=CARTESIAN_POINT('Ctrl Pts',(-3.82453556891143,-2.51997685422154,
21.4798923208725));
#42014=CARTESIAN_POINT('Ctrl Pts',(-3.31430027943462,-3.07074498667336,
21.5063496175569));
#42015=CARTESIAN_POINT('Ctrl Pts',(-2.80406498995777,-3.62151311912521,
21.5328069142414));
#42016=CARTESIAN_POINT('Ctrl Pts',(-2.15341752534944,-4.04228184598626,
21.5592642109259));
#42017=CARTESIAN_POINT('Ctrl Pts',(-1.44183871719702,-4.28187903967218,
21.5857215076104));
#42018=CARTESIAN_POINT('Ctrl Pts',(-0.730259909044641,-4.5214762333581,
21.6121788042948));
#42019=CARTESIAN_POINT('Ctrl Pts',(0.0422502426518133,-4.57990189386891,
21.6386361009793));
#42020=CARTESIAN_POINT('Ctrl Pts',(0.781724091400323,-4.44999904027082,
21.6650933976638));
#42021=CARTESIAN_POINT('Ctrl Pts',(1.52119794014883,-4.32009618667273,21.6915506943482));
#42022=CARTESIAN_POINT('Ctrl Pts',(2.2276354859494,-4.00186481896572,21.7180079910327));
#42023=CARTESIAN_POINT('Ctrl Pts',(2.81492815165366,-3.53408677354305,21.7444652877172));
#42024=CARTESIAN_POINT('Ctrl Pts',(3.40222081735796,-3.06630872812035,21.7709225844016));
#42025=CARTESIAN_POINT('Ctrl Pts',(3.87036860296593,-2.44898400498197,21.7973798810861));
#42026=CARTESIAN_POINT('Ctrl Pts',(4.16238619140555,-1.75729062849908,21.8238371777706));
#42027=CARTESIAN_POINT('Ctrl Pts',(4.39630197715038,-1.20322126398217,21.8450303510164));
#42028=CARTESIAN_POINT('Ctrl Pts',(4.51720308199739,-0.601432940640185,
21.8662235242623));
#42029=CARTESIAN_POINT('Ctrl Pts',(4.51782520267197,0.000113471772791779,
21.8874166975081));
#42030=CARTESIAN_POINT('Ctrl Pts',(4.51732076945549,-0.00048196737157627,
21.612583302492));
#42031=CARTESIAN_POINT('Ctrl Pts',(4.51749351971195,-0.222224494111391,
21.6047735665033));
#42032=CARTESIAN_POINT('Ctrl Pts',(4.50146734240306,-0.44389451533626,21.5969638305145));
#42033=CARTESIAN_POINT('Ctrl Pts',(4.46902189478939,-0.663041834113329,
21.5891540945258));
#42034=CARTESIAN_POINT('Ctrl Pts',(4.35910539635538,-1.40545433549076,21.5626967978413));
#42035=CARTESIAN_POINT('Ctrl Pts',(4.06074933765633,-2.11891445767478,21.5362395011569));
#42036=CARTESIAN_POINT('Ctrl Pts',(3.60841564297682,-2.71899122382358,21.5097822044724));
#42037=CARTESIAN_POINT('Ctrl Pts',(3.15608194829734,-3.31906798997234,21.4833249077879));
#42038=CARTESIAN_POINT('Ctrl Pts',(2.54977061763742,-3.80576140008588,21.4568676111035));
#42039=CARTESIAN_POINT('Ctrl Pts',(1.86683275295722,-4.11521969441498,21.430410314419));
#42040=CARTESIAN_POINT('Ctrl Pts',(1.18389488827701,-4.42467798874409,21.4039530177345));
#42041=CARTESIAN_POINT('Ctrl Pts',(0.424330489576522,-4.55690116728877,
21.37749572105));
#42042=CARTESIAN_POINT('Ctrl Pts',(-0.325633495564533,-4.50373822059831,
21.3510384243656));
#42043=CARTESIAN_POINT('Ctrl Pts',(-1.07559748070559,-4.45057527390784,
21.3245811276811));
#42044=CARTESIAN_POINT('Ctrl Pts',(-1.81596105228721,-4.21202620198225,
21.2981238309967));
#42045=CARTESIAN_POINT('Ctrl Pts',(-2.44569775560519,-3.80516814017082,
21.2716665343122));
#42046=CARTESIAN_POINT('Ctrl Pts',(-3.70517116224116,-2.99145201654798,
21.2187519409433));
#42047=CARTESIAN_POINT('Ctrl Pts',(-4.52213709582257,-1.50449993338184,
21.1658373475743));
#42048=CARTESIAN_POINT('Ctrl Pts',(-4.5251392293927,-0.0110172863203392,
21.1129227542054));
#42049=CARTESIAN_POINT('Ctrl Pts',(-4.52814136296284,1.4824653607412,21.0600081608364));
#42050=CARTESIAN_POINT('Ctrl Pts',(-3.71717969652165,2.98247857169809,21.0070935674675));
#42051=CARTESIAN_POINT('Ctrl Pts',(-2.46290199004371,3.79700220422752,20.9541789740986));
#42052=CARTESIAN_POINT('Ctrl Pts',(-1.20862428356581,4.61152583675692,20.9012643807296));
#42053=CARTESIAN_POINT('Ctrl Pts',(0.488969462948824,4.7405598908589,20.8483497873607));
#42054=CARTESIAN_POINT('Ctrl Pts',(1.85305394748095,4.12790602103174,20.7954351939918));
#42055=CARTESIAN_POINT('Ctrl Pts',(3.21713843201311,3.51525215120457,20.7425206006228));
#42056=CARTESIAN_POINT('Ctrl Pts',(4.24771365456276,2.16091035744822,20.6896060072539));
#42057=CARTESIAN_POINT('Ctrl Pts',(4.47332054780559,0.68305737845925,20.636691413885));
#42058=CARTESIAN_POINT('Ctrl Pts',(4.5075830310957,0.458618699879782,20.628655376754));
#42059=CARTESIAN_POINT('Ctrl Pts',(4.52327979691323,0.231331370382945,20.620619339623));
#42060=CARTESIAN_POINT('Ctrl Pts',(4.52133925202235,0.00376432143610439,
20.612583302492));
#42061=CARTESIAN_POINT('Origin',(0.,0.,20.5));
#42062=CARTESIAN_POINT('',(4.51048356578783,0.00141370502139415,19.612583302492));
#42063=CARTESIAN_POINT('',(4.51474283421141,-0.0038924084009401,19.8874166975081));
#42064=CARTESIAN_POINT('',(4.51775,5.53264807684796E-16,20.5));
#42065=CARTESIAN_POINT('Ctrl Pts',(4.51474283421141,-0.00389240840094011,
19.8874166975081));
#42066=CARTESIAN_POINT('Ctrl Pts',(4.50621483686762,1.04654996357473,19.9243723671861));
#42067=CARTESIAN_POINT('Ctrl Pts',(4.14085607956887,2.10234645737149,19.9613280368642));
#42068=CARTESIAN_POINT('Ctrl Pts',(3.4708839066554,2.90334883526624,19.9982837065423));
#42069=CARTESIAN_POINT('Ctrl Pts',(2.51159118088301,4.05025580469952,20.0511982999112));
#42070=CARTESIAN_POINT('Ctrl Pts',(0.927790752426727,4.6747928461432,20.1041128932802));
#42071=CARTESIAN_POINT('Ctrl Pts',(-0.556105607180406,4.49092827001162,
20.1570274866491));
#42072=CARTESIAN_POINT('Ctrl Pts',(-2.04000196678754,4.30706369388004,20.209942080018));
#42073=CARTESIAN_POINT('Ctrl Pts',(-3.42399425754553,3.3147975001732,20.262856673387));
#42074=CARTESIAN_POINT('Ctrl Pts',(-4.07445610293379,1.9687487323051,20.3157712667559));
#42075=CARTESIAN_POINT('Ctrl Pts',(-4.72491794832207,0.622699964436965,
20.3686858601248));
#42076=CARTESIAN_POINT('Ctrl Pts',(-4.64184934834058,-1.07713137759245,
20.4216004534938));
#42077=CARTESIAN_POINT('Ctrl Pts',(-3.86404219126196,-2.3542716484918,20.4745150468627));
#42078=CARTESIAN_POINT('Ctrl Pts',(-3.08623503418336,-3.63141191939111,
20.5274296402316));
#42079=CARTESIAN_POINT('Ctrl Pts',(-1.61368932000766,-4.48586111916038,
20.5803442336006));
#42080=CARTESIAN_POINT('Ctrl Pts',(-0.118635503777389,-4.52427204848619,
20.6332588269695));
#42081=CARTESIAN_POINT('Ctrl Pts',(1.37641831245292,-4.56268297781199,20.6861734203384));
#42082=CARTESIAN_POINT('Ctrl Pts',(2.89398023073781,-3.78505563669429,20.7390880137074));
#42083=CARTESIAN_POINT('Ctrl Pts',(3.73680595955696,-2.55211434826229,20.7920026070763));
#42084=CARTESIAN_POINT('Ctrl Pts',(4.24339242394412,-1.81104612176332,20.8238073038869));
#42085=CARTESIAN_POINT('Ctrl Pts',(4.50621711662441,-0.905486741220779,
20.8556120006975));
#42086=CARTESIAN_POINT('Ctrl Pts',(4.50983715083838,-0.000439487622834945,
20.8874166975081));
#42087=CARTESIAN_POINT('Ctrl Pts',(4.52133925202235,0.00376432143610439,
20.612583302492));
#42088=CARTESIAN_POINT('Ctrl Pts',(4.51050196349347,-1.26712087204873,20.567704746254));
#42089=CARTESIAN_POINT('Ctrl Pts',(3.94958417430038,-2.54673008347757,20.5228261900161));
#42090=CARTESIAN_POINT('Ctrl Pts',(3.00029299713898,-3.38761451526673,20.4779476337781));
#42091=CARTESIAN_POINT('Ctrl Pts',(1.88101998929342,-4.37906926578227,20.4250330404092));
#42092=CARTESIAN_POINT('Ctrl Pts',(0.221835409666229,-4.76061460259175,
20.3721184470403));
#42093=CARTESIAN_POINT('Ctrl Pts',(-1.21815646492133,-4.35804593593179,
20.3192038536714));
#42094=CARTESIAN_POINT('Ctrl Pts',(-2.65814833950885,-3.95547726927185,
20.2662892603024));
#42095=CARTESIAN_POINT('Ctrl Pts',(-3.87894750905677,-2.76879459914251,
20.2133746669335));
#42096=CARTESIAN_POINT('Ctrl Pts',(-4.32195458228653,-1.34081481536639,
20.1604600735645));
#42097=CARTESIAN_POINT('Ctrl Pts',(-4.76496165551631,0.0871649684097867,
20.1075454801956));
#42098=CARTESIAN_POINT('Ctrl Pts',(-4.43017663242789,1.75644186583272,20.0546308868267));
#42099=CARTESIAN_POINT('Ctrl Pts',(-3.47088390665552,2.90334883526609,20.0017162934577));
#42100=CARTESIAN_POINT('Ctrl Pts',(-2.51159118088318,4.05025580469941,19.9488017000888));
#42101=CARTESIAN_POINT('Ctrl Pts',(-0.927790752426926,4.67479284614316,
19.8958871067198));
#42102=CARTESIAN_POINT('Ctrl Pts',(0.556105607180211,4.49092827001165,19.8429725133509));
#42103=CARTESIAN_POINT('Ctrl Pts',(2.04000196678735,4.30706369388013,19.790057919982));
#42104=CARTESIAN_POINT('Ctrl Pts',(3.42399425754539,3.31479750017334,19.737143326613));
#42105=CARTESIAN_POINT('Ctrl Pts',(4.07445610293371,1.96874873230528,19.6842287332441));
#42106=CARTESIAN_POINT('Ctrl Pts',(4.36802741054216,1.36123992961467,19.6603469229934));
#42107=CARTESIAN_POINT('Ctrl Pts',(4.51218113590681,0.681666855829588,19.6364651127427));
#42108=CARTESIAN_POINT('Ctrl Pts',(4.51048356578783,0.00141370502139415,
19.612583302492));
#42109=CARTESIAN_POINT('Origin',(0.,0.,20.5));
#42110=CARTESIAN_POINT('',(4.51751172608841,-5.0340792907555E-5,18.612583302492));
#42111=CARTESIAN_POINT('',(4.52514732618828,-0.0014363825736758,18.8874166975081));
#42112=CARTESIAN_POINT('',(4.51775,5.53264807684796E-16,20.5));
#42113=CARTESIAN_POINT('Ctrl Pts',(4.52514732618828,-0.0014363825736758,
18.8874166975081));
#42114=CARTESIAN_POINT('Ctrl Pts',(4.52467107616349,1.48887736965158,18.9402181403059));
#42115=CARTESIAN_POINT('Ctrl Pts',(3.71449759637046,2.98422031831989,18.9930195831037));
#42116=CARTESIAN_POINT('Ctrl Pts',(2.46290199004355,3.79700220422763,19.0458210259014));
#42117=CARTESIAN_POINT('Ctrl Pts',(1.20862428356557,4.611525836757,19.0987356192704));
#42118=CARTESIAN_POINT('Ctrl Pts',(-0.488969462949119,4.74055989085888,
19.1516502126393));
#42119=CARTESIAN_POINT('Ctrl Pts',(-1.85305394748124,4.12790602103161,19.2045648060083));
#42120=CARTESIAN_POINT('Ctrl Pts',(-3.21713843201331,3.51525215120436,19.2574793993772));
#42121=CARTESIAN_POINT('Ctrl Pts',(-4.24771365456286,2.16091035744797,19.3103939927461));
#42122=CARTESIAN_POINT('Ctrl Pts',(-4.47332054780562,0.683057378459056,
19.3633085861151));
#42123=CARTESIAN_POINT('Ctrl Pts',(-4.69892744104839,-0.794795600529883,
19.416223179484));
#42124=CARTESIAN_POINT('Ctrl Pts',(-4.1195660049844,-2.3961597647514,19.4691377728529));
#42125=CARTESIAN_POINT('Ctrl Pts',(-3.00029299713883,-3.38761451526686,
19.5220523662219));
#42126=CARTESIAN_POINT('Ctrl Pts',(-1.8810199892932,-4.37906926578239,19.5749669595908));
#42127=CARTESIAN_POINT('Ctrl Pts',(-0.221835409665938,-4.76061460259178,
19.6278815529597));
#42128=CARTESIAN_POINT('Ctrl Pts',(1.21815646492164,-4.35804593593171,19.6807961463287));
#42129=CARTESIAN_POINT('Ctrl Pts',(2.6581483395091,-3.95547726927166,19.7337107396976));
#42130=CARTESIAN_POINT('Ctrl Pts',(3.8789475090569,-2.76879459914231,19.7866253330665));
#42131=CARTESIAN_POINT('Ctrl Pts',(4.32195458228659,-1.3408148153662,19.8395399264355));
#42132=CARTESIAN_POINT('Ctrl Pts',(4.45556453043254,-0.910139288059504,
19.8554988501263));
#42133=CARTESIAN_POINT('Ctrl Pts',(4.51842556165299,-0.457515081242471,
19.8714577738172));
#42134=CARTESIAN_POINT('Ctrl Pts',(4.51474283421141,-0.00389240840094011,
19.8874166975081));
#42135=CARTESIAN_POINT('Ctrl Pts',(4.51048356578783,0.00141370502139415,
19.612583302492));
#42136=CARTESIAN_POINT('Ctrl Pts',(4.50841985350745,-0.825560548001291,
19.5835505193738));
#42137=CARTESIAN_POINT('Ctrl Pts',(4.29080360170741,-1.65353988177363,19.5545177362555));
#42138=CARTESIAN_POINT('Ctrl Pts',(3.86404219126206,-2.35427164849163,19.5254849531373));
#42139=CARTESIAN_POINT('Ctrl Pts',(3.08623503418352,-3.63141191939097,19.4725703597684));
#42140=CARTESIAN_POINT('Ctrl Pts',(1.61368932000785,-4.48586111916031,19.4196557663994));
#42141=CARTESIAN_POINT('Ctrl Pts',(0.118635503777585,-4.52427204848618,
19.3667411730305));
#42142=CARTESIAN_POINT('Ctrl Pts',(-1.37641831245272,-4.56268297781205,
19.3138265796616));
#42143=CARTESIAN_POINT('Ctrl Pts',(-2.89398023073765,-3.78505563669441,
19.2609119862926));
#42144=CARTESIAN_POINT('Ctrl Pts',(-3.73680595955685,-2.55211434826245,
19.2079973929237));
#42145=CARTESIAN_POINT('Ctrl Pts',(-4.57963168837605,-1.3191730598305,19.1550827995547));
#42146=CARTESIAN_POINT('Ctrl Pts',(-4.74772122772955,0.369082175915713,
19.1021682061858));
#42147=CARTESIAN_POINT('Ctrl Pts',(-4.16995632188897,1.75277105187232,19.0492536128169));
#42148=CARTESIAN_POINT('Ctrl Pts',(-3.88107386896868,2.44461548985061,19.0227963161324));
#42149=CARTESIAN_POINT('Ctrl Pts',(-3.40572780474986,3.0603183378815,18.9963390194479));
#42150=CARTESIAN_POINT('Ctrl Pts',(-2.81753981467971,3.5286207682048,18.9698817227635));
#42151=CARTESIAN_POINT('Ctrl Pts',(-2.22935182460953,3.99692319852811,18.943424426079));
#42152=CARTESIAN_POINT('Ctrl Pts',(-1.52832190868799,4.31782521114383,18.9169671293945));
#42153=CARTESIAN_POINT('Ctrl Pts',(-0.790149843231659,4.44924273175287,
18.8905098327101));
#42154=CARTESIAN_POINT('Ctrl Pts',(-0.0519777777753676,4.58066025236191,
18.8640525360256));
#42155=CARTESIAN_POINT('Ctrl Pts',(0.72333643721573,4.5225932809643,18.8375952393411));
#42156=CARTESIAN_POINT('Ctrl Pts',(1.43588412720338,4.28390166798386,18.8111379426567));
#42157=CARTESIAN_POINT('Ctrl Pts',(2.14843181719103,4.04521005500342,18.7846806459722));
#42158=CARTESIAN_POINT('Ctrl Pts',(2.79821298217524,3.62589380044014,18.7582233492877));
#42159=CARTESIAN_POINT('Ctrl Pts',(3.30902952393793,3.07605344225331,18.7317660526033));
#42160=CARTESIAN_POINT('Ctrl Pts',(3.81984606570062,2.52621308406647,18.7053087559188));
#42161=CARTESIAN_POINT('Ctrl Pts',(4.19169798424179,1.84584862225607,18.6788514592343));
#42162=CARTESIAN_POINT('Ctrl Pts',(4.37772925931557,1.11834540158724,18.6523941625499));
#42163=CARTESIAN_POINT('Ctrl Pts',(4.47103767181987,0.753448850803234,18.6391238758639));
#42164=CARTESIAN_POINT('Ctrl Pts',(4.51759801973486,0.3766933068382,18.625853589178));
#42165=CARTESIAN_POINT('Ctrl Pts',(4.51751172608841,-5.0340792907555E-5,
18.612583302492));
#42166=CARTESIAN_POINT('Origin',(0.,0.,20.5));
#42167=CARTESIAN_POINT('',(4.51803700570725,7.32895604327321E-5,17.612583302492));
#42168=CARTESIAN_POINT('',(4.51742050630483,-6.62530376704942E-5,17.8874166975081));
#42169=CARTESIAN_POINT('',(4.51775,5.53264807684796E-16,20.5));
#42170=CARTESIAN_POINT('Ctrl Pts',(4.51742050630483,-6.62530376705099E-5,
17.8874166975081));
#42171=CARTESIAN_POINT('Ctrl Pts',(4.5172038153436,0.446598657046559,17.9031493200567));
#42172=CARTESIAN_POINT('Ctrl Pts',(4.4513943616742,0.893327565156709,17.9188819426052));
#42173=CARTESIAN_POINT('Ctrl Pts',(4.32092341583127,1.32030703112013,17.9346145651538));
#42174=CARTESIAN_POINT('Ctrl Pts',(4.10151253806993,2.03835148774488,17.9610718618383));
#42175=CARTESIAN_POINT('Ctrl Pts',(3.6992350517372,2.70054332815014,17.9875291585227));
#42176=CARTESIAN_POINT('Ctrl Pts',(3.16312948534596,3.22617356514213,18.0139864552072));
#42177=CARTESIAN_POINT('Ctrl Pts',(2.62702391895476,3.75180380213408,18.0404437518917));
#42178=CARTESIAN_POINT('Ctrl Pts',(1.95709027250505,4.1408724357128,18.0669010485761));
#42179=CARTESIAN_POINT('Ctrl Pts',(1.23484721910258,4.34609472311257,18.0933583452606));
#42180=CARTESIAN_POINT('Ctrl Pts',(0.51260416570011,4.55131701051233,18.1198156419451));
#42181=CARTESIAN_POINT('Ctrl Pts',(-0.261948294655145,4.57269295173316,
18.1462729386295));
#42182=CARTESIAN_POINT('Ctrl Pts',(-0.994322299916471,4.40742376897534,
18.172730235314));
#42183=CARTESIAN_POINT('Ctrl Pts',(-1.72669630517784,4.24215458621751,18.1991875319985));
#42184=CARTESIAN_POINT('Ctrl Pts',(-2.41689185534529,3.89024027948101,18.225644828683));
#42185=CARTESIAN_POINT('Ctrl Pts',(-2.98112377443714,3.39491220205621,18.2521021253674));
#42186=CARTESIAN_POINT('Ctrl Pts',(-3.54535569352893,2.89958412463147,18.2785594220519));
#42187=CARTESIAN_POINT('Ctrl Pts',(-3.98362398154516,2.26084227651845,18.3050167187363));
#42188=CARTESIAN_POINT('Ctrl Pts',(-4.24201965646877,1.55578891217658,18.3314740154208));
#42189=CARTESIAN_POINT('Ctrl Pts',(-4.50041533139241,0.85073554783464,18.3579313121053));
#42190=CARTESIAN_POINT('Ctrl Pts',(-4.5789383932234,0.0793706672638789,
18.3843886087897));
#42191=CARTESIAN_POINT('Ctrl Pts',(-4.46902189478936,-0.663041834113523,
18.4108459054742));
#42192=CARTESIAN_POINT('Ctrl Pts',(-4.35910539635533,-1.4054543354909,18.4373032021587));
#42193=CARTESIAN_POINT('Ctrl Pts',(-4.06074933765627,-2.11891445767488,
18.4637604988432));
#42194=CARTESIAN_POINT('Ctrl Pts',(-3.60841564297678,-2.71899122382363,
18.4902177955276));
#42195=CARTESIAN_POINT('Ctrl Pts',(-3.15608194829727,-3.31906798997241,
18.5166750922121));
#42196=CARTESIAN_POINT('Ctrl Pts',(-2.54977061763729,-3.80576140008597,
18.5431323888965));
#42197=CARTESIAN_POINT('Ctrl Pts',(-1.86683275295704,-4.11521969441507,
18.569589685581));
#42198=CARTESIAN_POINT('Ctrl Pts',(-1.18389488827682,-4.42467798874415,
18.5960469822655));
#42199=CARTESIAN_POINT('Ctrl Pts',(-0.424330489576326,-4.55690116728879,
18.62250427895));
#42200=CARTESIAN_POINT('Ctrl Pts',(0.325633495564726,-4.5037382205983,18.6489615756344));
#42201=CARTESIAN_POINT('Ctrl Pts',(1.07559748070578,-4.4505752739078,18.6754188723189));
#42202=CARTESIAN_POINT('Ctrl Pts',(1.8159610522874,-4.21202620198217,18.7018761690034));
#42203=CARTESIAN_POINT('Ctrl Pts',(2.44569775560536,-3.80516814017072,18.7283334656878));
#42204=CARTESIAN_POINT('Ctrl Pts',(3.70517116224129,-2.99145201654782,18.7812480590567));
#42205=CARTESIAN_POINT('Ctrl Pts',(4.52213709582263,-1.50449993338164,18.8341626524257));
#42206=CARTESIAN_POINT('Ctrl Pts',(4.5251392293927,-0.0110172863201459,
18.8870772457947));
#42207=CARTESIAN_POINT('Ctrl Pts',(4.52514564904193,-0.00782367934410926,
18.8871903963658));
#42208=CARTESIAN_POINT('Ctrl Pts',(4.52514834676573,-0.00463004250646042,
18.887303546937));
#42209=CARTESIAN_POINT('Ctrl Pts',(4.52514732618828,-0.00143638257367575,
18.8874166975081));
#42210=CARTESIAN_POINT('Ctrl Pts',(4.51751172608841,-5.0340792907555E-5,
18.612583302492));
#42211=CARTESIAN_POINT('Ctrl Pts',(4.51742597397124,-0.374429761958339,
18.5993962924935));
#42212=CARTESIAN_POINT('Ctrl Pts',(4.47127719829474,-0.748797435630456,
18.586209282495));
#42213=CARTESIAN_POINT('Ctrl Pts',(4.37916492462631,-1.11150455739379,18.5730222724965));
#42214=CARTESIAN_POINT('Ctrl Pts',(4.19435868325684,-1.83920931617878,18.546564975812));
#42215=CARTESIAN_POINT('Ctrl Pts',(3.8245355689115,-2.51997685422145,18.5201076791275));
#42216=CARTESIAN_POINT('Ctrl Pts',(3.31430027943466,-3.07074498667331,18.493650382443));
#42217=CARTESIAN_POINT('Ctrl Pts',(2.80406498995785,-3.62151311912514,18.4671930857586));
#42218=CARTESIAN_POINT('Ctrl Pts',(2.15341752534957,-4.04228184598617,18.4407357890741));
#42219=CARTESIAN_POINT('Ctrl Pts',(1.4418387171972,-4.28187903967212,18.4142784923896));
#42220=CARTESIAN_POINT('Ctrl Pts',(0.730259909044834,-4.52147623335806,
18.3878211957052));
#42221=CARTESIAN_POINT('Ctrl Pts',(-0.0422502426516132,-4.57990189386892,
18.3613638990207));
#42222=CARTESIAN_POINT('Ctrl Pts',(-0.781724091400131,-4.44999904027085,
18.3349066023362));
#42223=CARTESIAN_POINT('Ctrl Pts',(-1.52119794014869,-4.32009618667279,
18.3084493056518));
#42224=CARTESIAN_POINT('Ctrl Pts',(-2.2276354859493,-4.00186481896578,18.2819920089673));
#42225=CARTESIAN_POINT('Ctrl Pts',(-2.81492815165361,-3.53408677354309,
18.2555347122828));
#42226=CARTESIAN_POINT('Ctrl Pts',(-3.40222081735788,-3.06630872812042,
18.2290774155984));
#42227=CARTESIAN_POINT('Ctrl Pts',(-3.87036860296584,-2.4489840049821,18.2026201189139));
#42228=CARTESIAN_POINT('Ctrl Pts',(-4.16238619140547,-1.75729062849926,
18.1761628222294));
#42229=CARTESIAN_POINT('Ctrl Pts',(-4.45440377984509,-1.06559725201643,
18.149705525545));
#42230=CARTESIAN_POINT('Ctrl Pts',(-4.57029117111638,-0.299535222189059,
18.1232482288605));
#42231=CARTESIAN_POINT('Ctrl Pts',(-4.49591510340165,0.447583892947263,
18.096790932176));
#42232=CARTESIAN_POINT('Ctrl Pts',(-4.42153903568692,1.19470300808361,18.0703336354916));
#42233=CARTESIAN_POINT('Ctrl Pts',(-4.15689950898618,1.92287920852894,18.0438763388071));
#42234=CARTESIAN_POINT('Ctrl Pts',(-3.73423901960036,2.54342464869681,18.0174190421226));
#42235=CARTESIAN_POINT('Ctrl Pts',(-3.31157853021454,3.16397008886469,17.9909617454381));
#42236=CARTESIAN_POINT('Ctrl Pts',(-2.73089707814366,3.67688476875509,17.9645044487537));
#42237=CARTESIAN_POINT('Ctrl Pts',(-2.06291588716924,4.01969454812901,17.9380471520692));
#42238=CARTESIAN_POINT('Ctrl Pts',(-1.39493469619478,4.36250432750296,17.9115898553848));
#42239=CARTESIAN_POINT('Ctrl Pts',(-0.639653766316788,4.53520920636039,
17.8851325587003));
#42240=CARTESIAN_POINT('Ctrl Pts',(0.110931801888114,4.51677482186132,17.8586752620158));
#42241=CARTESIAN_POINT('Ctrl Pts',(0.861517370092973,4.49834043736224,17.8322179653313));
#42242=CARTESIAN_POINT('Ctrl Pts',(1.60740757662473,4.28876678950667,17.8057606686469));
#42243=CARTESIAN_POINT('Ctrl Pts',(2.25775525993247,3.91357923987676,17.7793033719624));
#42244=CARTESIAN_POINT('Ctrl Pts',(2.90810294324022,3.53839169024685,17.7528460752779));
#42245=CARTESIAN_POINT('Ctrl Pts',(3.46290810332394,2.99759023884261,17.7263887785935));
#42246=CARTESIAN_POINT('Ctrl Pts',(3.8545953230205,2.35704415643041,17.699931481909));
#42247=CARTESIAN_POINT('Ctrl Pts',(4.24628254271708,1.71649807401819,17.6734741852245));
#42248=CARTESIAN_POINT('Ctrl Pts',(4.47485182202649,0.976207360598019,17.6470168885401));
#42249=CARTESIAN_POINT('Ctrl Pts',(4.51246407961468,0.226338472032798,17.6205595918556));
#42250=CARTESIAN_POINT('Ctrl Pts',(4.51624383400808,0.150982181084616,17.6179008287344));
#42251=CARTESIAN_POINT('Ctrl Pts',(4.5180951579083,0.0755291623761646,17.6152420656132));
#42252=CARTESIAN_POINT('Ctrl Pts',(4.51803700570725,7.32895604327322E-5,
17.612583302492));
#42253=CARTESIAN_POINT('Origin',(0.,0.,20.5));
#42254=CARTESIAN_POINT('',(4.51759135405446,-0.000109312323752775,16.612583302492));
#42255=CARTESIAN_POINT('',(4.51783748975292,0.000112199089269072,16.8874166975081));
#42256=CARTESIAN_POINT('',(4.51775,5.53264807684796E-16,20.5));
#42257=CARTESIAN_POINT('Ctrl Pts',(4.51783748975292,0.000112199089269072,
16.8874166975081));
#42258=CARTESIAN_POINT('Ctrl Pts',(4.5179865637855,0.145467881021208,16.8925377964919));
#42259=CARTESIAN_POINT('Ctrl Pts',(4.51110979946378,0.290809516813962,16.8976588954757));
#42260=CARTESIAN_POINT('Ctrl Pts',(4.49710302020602,0.435460743134165,16.9027799944596));
#42261=CARTESIAN_POINT('Ctrl Pts',(4.42473935069149,1.18277697791411,16.929237291144));
#42262=CARTESIAN_POINT('Ctrl Pts',(4.16206856248382,1.91166550411022,16.9556945878285));
#42263=CARTESIAN_POINT('Ctrl Pts',(3.7410836561604,2.53334852003379,16.9821518845129));
#42264=CARTESIAN_POINT('Ctrl Pts',(3.320098749837,3.15503153595733,17.0086091811974));
#42265=CARTESIAN_POINT('Ctrl Pts',(2.74079972539787,3.66950904160833,17.0350664778819));
#42266=CARTESIAN_POINT('Ctrl Pts',(2.07374458313351,4.01411821952866,17.0615237745663));
#42267=CARTESIAN_POINT('Ctrl Pts',(1.40668944086914,4.358727397449,17.0879810712508));
#42268=CARTESIAN_POINT('Ctrl Pts',(0.651878180779539,4.53346824763866,17.1144383679353));
#42269=CARTESIAN_POINT('Ctrl Pts',(-0.0987540592508608,4.51705757827172,
17.1408956646198));
#42270=CARTESIAN_POINT('Ctrl Pts',(-0.849386299281262,4.50064690890479,
17.1673529613042));
#42271=CARTESIAN_POINT('Ctrl Pts',(-1.59583951925246,4.29308471998125,17.1938102579887));
#42272=CARTESIAN_POINT('Ctrl Pts',(-2.24719647092549,3.91965176135179,17.2202675546731));
#42273=CARTESIAN_POINT('Ctrl Pts',(-2.89855342259852,3.54621880272232,17.2467248513576));
#42274=CARTESIAN_POINT('Ctrl Pts',(-3.45481410597338,3.00691507438693,17.2731821480421));
#42275=CARTESIAN_POINT('Ctrl Pts',(-3.8482267217169,2.36742735305624,17.2996394447266));
#42276=CARTESIAN_POINT('Ctrl Pts',(-4.24163933746045,1.7279396317255,17.326096741411));
#42277=CARTESIAN_POINT('Ctrl Pts',(-4.47220388557264,0.988267917399458,
17.3525540380955));
#42278=CARTESIAN_POINT('Ctrl Pts',(-4.51183760195937,0.238503067401354,
17.37901133478));
#42279=CARTESIAN_POINT('Ctrl Pts',(-4.55147131834609,-0.511261782596708,
17.4054686314644));
#42280=CARTESIAN_POINT('Ctrl Pts',(-4.40017420300738,-1.27111976826683,
17.4319259281489));
#42281=CARTESIAN_POINT('Ctrl Pts',(-4.07637456299423,-1.94852038806902,
17.4583832248334));
#42282=CARTESIAN_POINT('Ctrl Pts',(-3.75257492298108,-2.62592100787122,
17.4848405215178));
#42283=CARTESIAN_POINT('Ctrl Pts',(-3.25627275829351,-3.22086426180549,
17.5112978182023));
#42284=CARTESIAN_POINT('Ctrl Pts',(-2.64791620593751,-3.66088792814038,
17.5377551148868));
#42285=CARTESIAN_POINT('Ctrl Pts',(-2.0395596535815,-4.10091159447528,17.5642124115712));
#42286=CARTESIAN_POINT('Ctrl Pts',(-1.31914871355708,-4.38601567321079,
17.5906697082557));
#42287=CARTESIAN_POINT('Ctrl Pts',(-0.574430373257593,-4.48147252184731,
17.6171270049402));
#42288=CARTESIAN_POINT('Ctrl Pts',(0.17028796704189,-4.57692937048383,17.6435843016246));
#42289=CARTESIAN_POINT('Ctrl Pts',(0.939313707616428,-4.48273898902136,
17.6700415983091));
#42290=CARTESIAN_POINT('Ctrl Pts',(1.63898363511409,-4.21037796912968,17.6964988949936));
#42291=CARTESIAN_POINT('Ctrl Pts',(2.33865356261174,-3.93801694923801,17.7229561916781));
#42292=CARTESIAN_POINT('Ctrl Pts',(2.96896767703252,-3.48748529091713,17.7494134883625));
#42293=CARTESIAN_POINT('Ctrl Pts',(3.45314824099611,-2.91364911818949,17.775870785047));
#42294=CARTESIAN_POINT('Ctrl Pts',(3.9373288049597,-2.33981294546184,17.8023280817315));
#42295=CARTESIAN_POINT('Ctrl Pts',(4.27537581846611,-1.64267225832742,17.8287853784159));
#42296=CARTESIAN_POINT('Ctrl Pts',(4.42612719062433,-0.907153378338104,
17.8552426751004));
#42297=CARTESIAN_POINT('Ctrl Pts',(4.48723544976425,-0.609004992176015,
17.8659673492363));
#42298=CARTESIAN_POINT('Ctrl Pts',(4.51756822102564,-0.304550492318464,
17.8766920233722));
#42299=CARTESIAN_POINT('Ctrl Pts',(4.51742050630483,-6.62530376704943E-5,
17.8874166975081));
#42300=CARTESIAN_POINT('Ctrl Pts',(4.51803700570725,7.32895604327322E-5,
17.612583302492));
#42301=CARTESIAN_POINT('Ctrl Pts',(4.5175164865615,-0.675330663287972,17.5887847689287));
#42302=CARTESIAN_POINT('Ctrl Pts',(4.36400868534142,-1.35096328729663,17.5649862353655));
#42303=CARTESIAN_POINT('Ctrl Pts',(4.07110679585739,-1.95950283641844,17.5411877018022));
#42304=CARTESIAN_POINT('Ctrl Pts',(3.74548201864491,-2.63602819259433,17.5147304051177));
#42305=CARTESIAN_POINT('Ctrl Pts',(3.24757722835295,-3.22963184123583,17.4882731084333));
#42306=CARTESIAN_POINT('Ctrl Pts',(2.63803679068424,-3.66801355240638,17.4618158117488));
#42307=CARTESIAN_POINT('Ctrl Pts',(2.02849635301557,-4.10639526357692,17.4353585150643));
#42308=CARTESIAN_POINT('Ctrl Pts',(1.30732026797015,-4.38955503727653,17.4089012183799));
#42309=CARTESIAN_POINT('Ctrl Pts',(0.562346924558562,-4.48300430658583,
17.3824439216954));
#42310=CARTESIAN_POINT('Ctrl Pts',(-0.182626418853022,-4.57645357589513,
17.3559866250109));
#42311=CARTESIAN_POINT('Ctrl Pts',(-0.95139702063077,-4.48019234081411,
17.3295293283265));
#42312=CARTESIAN_POINT('Ctrl Pts',(-1.65032944052442,-4.20594512376068,
17.303072031642));
#42313=CARTESIAN_POINT('Ctrl Pts',(-2.34926186041808,-3.93169790670724,
17.2766147349575));
#42314=CARTESIAN_POINT('Ctrl Pts',(-2.97835609842763,-3.47946470768139,
17.2501574382731));
#42315=CARTESIAN_POINT('Ctrl Pts',(-3.46098918943056,-2.90432702425224,
17.2237001415886));
#42316=CARTESIAN_POINT('Ctrl Pts',(-3.94362228043348,-2.32918934082309,
17.1972428449041));
#42317=CARTESIAN_POINT('Ctrl Pts',(-4.27979422442977,-1.63114717299066,
17.1707855482197));
#42318=CARTESIAN_POINT('Ctrl Pts',(-4.42855964178007,-0.895221287202602,
17.1443282515352));
#42319=CARTESIAN_POINT('Ctrl Pts',(-4.57732505913038,-0.159295401414506,
17.1178709548507));
#42320=CARTESIAN_POINT('Ctrl Pts',(-4.53868394983468,0.614514202329214,
17.0914136581662));
#42321=CARTESIAN_POINT('Ctrl Pts',(-4.31734276296002,1.33195837225454,17.0649563614818));
#42322=CARTESIAN_POINT('Ctrl Pts',(-4.09600157608536,2.04940254217985,17.0384990647973));
#42323=CARTESIAN_POINT('Ctrl Pts',(-3.69196031163174,2.71048127828677,17.0120417681128));
#42324=CARTESIAN_POINT('Ctrl Pts',(-3.15443074594472,3.23467592132634,16.9855844714284));
#42325=CARTESIAN_POINT('Ctrl Pts',(-2.61690118025774,3.75887056436587,16.9591271747439));
#42326=CARTESIAN_POINT('Ctrl Pts',(-1.94588331333737,4.14618111433807,16.9326698780594));
#42327=CARTESIAN_POINT('Ctrl Pts',(-1.223106380062,4.3494335753433,16.906212581375));
#42328=CARTESIAN_POINT('Ctrl Pts',(-0.500329446786581,4.55268603634855,
16.8797552846905));
#42329=CARTESIAN_POINT('Ctrl Pts',(0.274206552843852,4.57188040838682,16.853297988006));
#42330=CARTESIAN_POINT('Ctrl Pts',(1.00616399197863,4.40467883795473,16.8268406913216));
#42331=CARTESIAN_POINT('Ctrl Pts',(1.73812143111341,4.23747726752264,16.8003833946371));
#42332=CARTESIAN_POINT('Ctrl Pts',(2.42750030975254,3.88387975462018,16.7739260979526));
#42333=CARTESIAN_POINT('Ctrl Pts',(2.99033504306357,3.38695408510442,16.7474688012682));
#42334=CARTESIAN_POINT('Ctrl Pts',(3.55316977637459,2.89002841558867,16.7210115045837));
#42335=CARTESIAN_POINT('Ctrl Pts',(3.98946036435752,2.24977458945961,16.6945542078992));
#42336=CARTESIAN_POINT('Ctrl Pts',(4.24606709644911,1.54417481408576,16.6680969112148));
#42337=CARTESIAN_POINT('Ctrl Pts',(4.42554078305754,1.05067025197154,16.6495923749738));
#42338=CARTESIAN_POINT('Ctrl Pts',(4.51711737210933,0.525199995180907,16.6310878387329));
#42339=CARTESIAN_POINT('Ctrl Pts',(4.51759135405446,-0.000109312323752775,
16.612583302492));
#42340=CARTESIAN_POINT('Origin',(0.,0.,20.5));
#42341=CARTESIAN_POINT('',(4.51759608459634,0.0001098887360651,15.612583302492));
#42342=CARTESIAN_POINT('',(4.5178043285159,-0.000114763987914418,15.8874166975081));
#42343=CARTESIAN_POINT('',(4.51775,5.53264807684796E-16,20.5));
#42344=CARTESIAN_POINT('Ctrl Pts',(4.5178043285159,-0.000114763987914418,
15.8874166975081));
#42345=CARTESIAN_POINT('Ctrl Pts',(4.51719021324072,0.595015005655344,15.9083835696116));
#42346=CARTESIAN_POINT('Ctrl Pts',(4.39892963080694,1.19038158256103,15.9293504417152));
#42347=CARTESIAN_POINT('Ctrl Pts',(4.16984886166331,1.73951778234083,15.9503173138187));
#42348=CARTESIAN_POINT('Ctrl Pts',(3.88078057126651,2.43245182066608,15.9767746105032));
#42349=CARTESIAN_POINT('Ctrl Pts',(3.41525380642348,3.05177344176931,16.0032319071877));
#42350=CARTESIAN_POINT('Ctrl Pts',(2.82996921187389,3.52204995762958,16.0296892038721));
#42351=CARTESIAN_POINT('Ctrl Pts',(2.2446846173243,3.99232647348986,16.0561465005566));
#42352=CARTESIAN_POINT('Ctrl Pts',(1.53964219306814,4.3135578841072,16.082603797241));
#42353=CARTESIAN_POINT('Ctrl Pts',(0.800715326097207,4.44661855917225,16.1090610939255));
#42354=CARTESIAN_POINT('Ctrl Pts',(0.0617884591262693,4.57967923423731,
16.13551839061));
#42355=CARTESIAN_POINT('Ctrl Pts',(-0.711022850559448,4.52456917375008,
16.1619756872944));
#42356=CARTESIAN_POINT('Ctrl Pts',(-1.42359104075325,4.28800072211039,16.1884329839789));
#42357=CARTESIAN_POINT('Ctrl Pts',(-2.13615923094709,4.0514322704707,16.2148902806634));
#42358=CARTESIAN_POINT('Ctrl Pts',(-2.788484301649,3.63340542767853,16.2413475773478));
#42359=CARTESIAN_POINT('Ctrl Pts',(-3.30111378116087,3.08483540049633,16.2678048740323));
#42360=CARTESIAN_POINT('Ctrl Pts',(-3.81374326067272,2.53626537331417,16.2942621707168));
#42361=CARTESIAN_POINT('Ctrl Pts',(-4.18667714899455,1.857152161742,16.3207194674013));
#42362=CARTESIAN_POINT('Ctrl Pts',(-4.37449251133268,1.1302110034409,16.3471767640857));
#42363=CARTESIAN_POINT('Ctrl Pts',(-4.56230787367082,0.403269845139789,
16.3736340607702));
#42364=CARTESIAN_POINT('Ctrl Pts',(-4.56500471002526,-0.371499259890255,
16.4000913574546));
#42365=CARTESIAN_POINT('Ctrl Pts',(-4.38225454858744,-1.09973029228273,
16.4265486541391));
#42366=CARTESIAN_POINT('Ctrl Pts',(-4.19950438714961,-1.82796132467523,
16.4530059508236));
#42367=CARTESIAN_POINT('Ctrl Pts',(-3.8313072279195,-2.50965428443015,16.4794632475081));
#42368=CARTESIAN_POINT('Ctrl Pts',(-3.3225090776326,-3.06177972318871,16.5059205441925));
#42369=CARTESIAN_POINT('Ctrl Pts',(-2.81371092734571,-3.61390516194727,
16.532377840877));
#42370=CARTESIAN_POINT('Ctrl Pts',(-2.16431178600201,-4.03646307970946,
16.5588351375615));
#42371=CARTESIAN_POINT('Ctrl Pts',(-1.45340774986022,-4.27798639033812,
16.5852924342459));
#42372=CARTESIAN_POINT('Ctrl Pts',(-0.742503713718461,-4.51950970096678,
16.6117497309304));
#42373=CARTESIAN_POINT('Ctrl Pts',(0.0299052172213853,-4.5799984044619,
16.6382070276149));
#42374=CARTESIAN_POINT('Ctrl Pts',(0.769740489176569,-4.45208504257185,
16.6646643242993));
#42375=CARTESIAN_POINT('Ctrl Pts',(1.50957576113175,-4.32417168068181,16.6911216209838));
#42376=CARTESIAN_POINT('Ctrl Pts',(2.21683737410228,-4.00785625340658,16.7175789176683));
#42377=CARTESIAN_POINT('Ctrl Pts',(2.80538164796928,-3.54166563180933,16.7440362143527));
#42378=CARTESIAN_POINT('Ctrl Pts',(3.39392592183629,-3.07547501021207,16.7704935110372));
#42379=CARTESIAN_POINT('Ctrl Pts',(3.86375285659978,-2.45940919429276,16.7969508077217));
#42380=CARTESIAN_POINT('Ctrl Pts',(4.15763804857084,-1.76850431465121,16.8234081044061));
#42381=CARTESIAN_POINT('Ctrl Pts',(4.39463854911208,-1.21133162689784,16.8447443021068));
#42382=CARTESIAN_POINT('Ctrl Pts',(4.51721639786597,-0.605487805208481,
16.8660804998074));
#42383=CARTESIAN_POINT('Ctrl Pts',(4.51783748975292,0.000112199089269072,
16.8874166975081));
#42384=CARTESIAN_POINT('Ctrl Pts',(4.51759135405446,-0.000109312323752775,
16.612583302492));
#42385=CARTESIAN_POINT('Ctrl Pts',(4.51779505896309,-0.225873364281351,
16.6046305420484));
#42386=CARTESIAN_POINT('Ctrl Pts',(4.50117162820754,-0.451607688050524,
16.5966777816049));
#42387=CARTESIAN_POINT('Ctrl Pts',(4.46746660375751,-0.674762023706868,
16.5887250211614));
#42388=CARTESIAN_POINT('Ctrl Pts',(4.35533650277404,-1.417153361507,16.5622677244769));
#42389=CARTESIAN_POINT('Ctrl Pts',(4.05415342460685,-2.1309903124886,16.5358104277924));
#42390=CARTESIAN_POINT('Ctrl Pts',(3.60060113490314,-2.72932832606603,16.509353131108));
#42391=CARTESIAN_POINT('Ctrl Pts',(3.14704884519943,-3.32766633964346,16.4828958344235));
#42392=CARTESIAN_POINT('Ctrl Pts',(2.54112734395919,-3.81050541581671,16.456438537739));
#42393=CARTESIAN_POINT('Ctrl Pts',(1.85663719941204,-4.1190362894713,16.4299812410546));
#42394=CARTESIAN_POINT('Ctrl Pts',(1.17214705486486,-4.4275671631259,16.4035239443701));
#42395=CARTESIAN_POINT('Ctrl Pts',(0.409088267010757,-4.56178983426182,
16.3770666476856));
#42396=CARTESIAN_POINT('Ctrl Pts',(-0.33959944827516,-4.50535613008826,
16.3506093510012));
#42397=CARTESIAN_POINT('Ctrl Pts',(-1.08828716356108,-4.4489224259147,16.3241520543167));
#42398=CARTESIAN_POINT('Ctrl Pts',(-1.82260380627881,-4.20183234643166,
16.2976947576322));
#42399=CARTESIAN_POINT('Ctrl Pts',(-2.45311042204468,-3.79418118985514,
16.2712374609477));
#42400=CARTESIAN_POINT('Ctrl Pts',(-3.08361703781053,-3.38653003327864,
16.2447801642633));
#42401=CARTESIAN_POINT('Ctrl Pts',(-3.61031362662454,-2.81831779960867,
16.2183228675788));
#42402=CARTESIAN_POINT('Ctrl Pts',(-3.96904912687637,-2.15875211004946,
16.1918655708943));
#42403=CARTESIAN_POINT('Ctrl Pts',(-4.3277846271282,-1.49918642049025,16.1654082742099));
#42404=CARTESIAN_POINT('Ctrl Pts',(-4.51855903881786,-0.748267275041791,
16.1389509775254));
#42405=CARTESIAN_POINT('Ctrl Pts',(-4.51813624973985,0.00254420544672257,
16.1124936808409));
#42406=CARTESIAN_POINT('Ctrl Pts',(-4.51771346066184,0.753355685935258,
16.0860363841565));
#42407=CARTESIAN_POINT('Ctrl Pts',(-4.32609347081614,1.50405950146385,16.059579087472));
#42408=CARTESIAN_POINT('Ctrl Pts',(-3.96661538289292,2.16322075812806,16.0331217907875));
#42409=CARTESIAN_POINT('Ctrl Pts',(-3.6071372949697,2.82238201479228,16.0066644941031));
#42410=CARTESIAN_POINT('Ctrl Pts',(-3.07980110896895,3.39000071259211,15.9802071974186));
#42411=CARTESIAN_POINT('Ctrl Pts',(-2.4488357887268,3.7969415223371,15.9537499007341));
#42412=CARTESIAN_POINT('Ctrl Pts',(-1.81787046848466,4.20388233208208,15.9272926040497));
#42413=CARTESIAN_POINT('Ctrl Pts',(-1.08327601400112,4.45014525377221,15.9008353073652));
#42414=CARTESIAN_POINT('Ctrl Pts',(-0.334525216833305,4.50573573609241,
15.8743780106807));
#42415=CARTESIAN_POINT('Ctrl Pts',(0.41422558033451,4.5613262184126,15.8479207139963));
#42416=CARTESIAN_POINT('Ctrl Pts',(1.1771327201866,4.42624426136285,15.8214634173118));
#42417=CARTESIAN_POINT('Ctrl Pts',(1.86127495742196,4.11694269781245,15.7950061206273));
#42418=CARTESIAN_POINT('Ctrl Pts',(2.54541719465734,3.80764113426205,15.7685488239429));
#42419=CARTESIAN_POINT('Ctrl Pts',(3.15079452927597,3.32411996421099,15.7420915272584));
#42420=CARTESIAN_POINT('Ctrl Pts',(3.60367267191142,2.72527153104349,15.7156342305739));
#42421=CARTESIAN_POINT('Ctrl Pts',(4.05655081454687,2.12642309787598,15.6891769338895));
#42422=CARTESIAN_POINT('Ctrl Pts',(4.35692976519912,1.41224740159204,15.662719637205));
#42423=CARTESIAN_POINT('Ctrl Pts',(4.46822370011744,0.669730251598505,15.6362623405205));
#42424=CARTESIAN_POINT('Ctrl Pts',(4.50142605066627,0.448214903788299,15.6283693278443));
#42425=CARTESIAN_POINT('Ctrl Pts',(4.51779965427679,0.224177139537577,15.6204763151682));
#42426=CARTESIAN_POINT('Ctrl Pts',(4.51759608459634,0.0001098887360651,
15.612583302492));
#42427=CARTESIAN_POINT('Origin',(0.,0.,20.5));
#42428=CARTESIAN_POINT('',(4.51803303654689,-7.46219232266102E-5,14.612583302492));
#42429=CARTESIAN_POINT('',(4.51743493951217,7.09613961932946E-5,14.8874166975081));
#42430=CARTESIAN_POINT('',(4.51775,5.53264807684796E-16,20.5));
#42431=CARTESIAN_POINT('Ctrl Pts',(4.51743493951217,7.09613961932946E-5,
14.8874166975081));
#42432=CARTESIAN_POINT('Ctrl Pts',(4.51759894908653,0.294069189408427,14.8977720460469));
#42433=CARTESIAN_POINT('Ctrl Pts',(4.48933542297813,0.588036293354993,14.9081273945857));
#42434=CARTESIAN_POINT('Ctrl Pts',(4.43233806206614,0.876322399438229,14.9184827431245));
#42435=CARTESIAN_POINT('Ctrl Pts',(4.2867132110791,1.61287617260017,14.9449400398089));
#42436=CARTESIAN_POINT('Ctrl Pts',(3.95352194255086,2.31234598448206,14.9713973364934));
#42437=CARTESIAN_POINT('Ctrl Pts',(3.47334658423498,2.88953718612178,14.9978546331779));
#42438=CARTESIAN_POINT('Ctrl Pts',(2.99317122591908,3.46672838776151,15.0243119298623));
#42439=CARTESIAN_POINT('Ctrl Pts',(2.36601177781554,3.92164097915906,15.0507692265468));
#42440=CARTESIAN_POINT('Ctrl Pts',(1.6682555666064,4.19886711014818,15.0772265232313));
#42441=CARTESIAN_POINT('Ctrl Pts',(0.97049935539727,4.4760932411373,15.1036838199157));
#42442=CARTESIAN_POINT('Ctrl Pts',(0.20214638108255,4.57563291171798,15.1301411166002));
#42443=CARTESIAN_POINT('Ctrl Pts',(-0.543218814426446,4.48536230017716,
15.1565984132847));
#42444=CARTESIAN_POINT('Ctrl Pts',(-1.28858400993542,4.39509168863634,15.1830557099691));
#42445=CARTESIAN_POINT('Ctrl Pts',(-2.01096142663867,4.11501079497402,15.2095130066536));
#42446=CARTESIAN_POINT('Ctrl Pts',(-2.6223662946594,3.67923316206403,15.2359703033381));
#42447=CARTESIAN_POINT('Ctrl Pts',(-3.23377116268013,3.24345552915403,15.2624276000225));
#42448=CARTESIAN_POINT('Ctrl Pts',(-3.73420348201834,2.65198115699635,15.288884896707));
#42449=CARTESIAN_POINT('Ctrl Pts',(-4.06271115002269,1.9768509695166,15.3153421933915));
#42450=CARTESIAN_POINT('Ctrl Pts',(-4.39121881802704,1.30172078203686,15.3417994900759));
#42451=CARTESIAN_POINT('Ctrl Pts',(-4.54780183469754,0.542934779235054,
15.3682567867604));
#42452=CARTESIAN_POINT('Ctrl Pts',(-4.51338856189906,-0.207087743519677,
15.3947140834449));
#42453=CARTESIAN_POINT('Ctrl Pts',(-4.47897528910057,-0.957110266274451,
15.4211713801293));
#42454=CARTESIAN_POINT('Ctrl Pts',(-4.2535657268331,-1.69836930898215,15.4476286768138));
#42455=CARTESIAN_POINT('Ctrl Pts',(-3.86461451031294,-2.34058034061557,
15.4740859734983));
#42456=CARTESIAN_POINT('Ctrl Pts',(-3.4756632937928,-2.98279137224897,15.5005432701827));
#42457=CARTESIAN_POINT('Ctrl Pts',(-2.92317042302,-3.5259543928081,15.5270005668672));
#42458=CARTESIAN_POINT('Ctrl Pts',(-2.27442891819367,-3.9039127475242,15.5534578635517));
#42459=CARTESIAN_POINT('Ctrl Pts',(-1.62568741336734,-4.28187110224029,
15.5799151602362));
#42460=CARTESIAN_POINT('Ctrl Pts',(-0.880697274487477,-4.49462479111335,
15.6063724569206));
#42461=CARTESIAN_POINT('Ctrl Pts',(-0.130197475965578,-4.51626065030008,
15.6328297536051));
#42462=CARTESIAN_POINT('Ctrl Pts',(0.620302322556342,-4.53789650948681,
15.6592870502896));
#42463=CARTESIAN_POINT('Ctrl Pts',(1.3763117807203,-4.3684145389872,15.685744346974));
#42464=CARTESIAN_POINT('Ctrl Pts',(2.04574978322079,-4.02845745523656,15.7122016436585));
#42465=CARTESIAN_POINT('Ctrl Pts',(2.71518778572125,-3.68850037148593,15.738658940343));
#42466=CARTESIAN_POINT('Ctrl Pts',(3.29805433255825,-3.17806817448428,15.7651162370274));
#42467=CARTESIAN_POINT('Ctrl Pts',(3.72335692340443,-2.55933094091619,15.7915735337119));
#42468=CARTESIAN_POINT('Ctrl Pts',(4.14865951425061,-1.94059370734809,15.8180308303964));
#42469=CARTESIAN_POINT('Ctrl Pts',(4.41639814910596,-1.21355143721353,15.8444881270808));
#42470=CARTESIAN_POINT('Ctrl Pts',(4.49396255855834,-0.466757074372606,
15.8709454237653));
#42471=CARTESIAN_POINT('Ctrl Pts',(4.51005874349141,-0.311782128309925,
15.8764358483462));
#42472=CARTESIAN_POINT('Ctrl Pts',(4.51796514189739,-0.155956565280692,
15.8819262729272));
#42473=CARTESIAN_POINT('Ctrl Pts',(4.5178043285159,-0.000114763987914418,
15.8874166975081));
#42474=CARTESIAN_POINT('Ctrl Pts',(4.51759608459634,0.0001098887360651,
15.612583302492));
#42475=CARTESIAN_POINT('Ctrl Pts',(4.5171172908178,-0.526893962833933,15.5940190184837));
#42476=CARTESIAN_POINT('Ctrl Pts',(4.42493597400368,-1.05406092973462,15.5754547344754));
#42477=CARTESIAN_POINT('Ctrl Pts',(4.24432532522022,-1.54895583471304,15.5568904504671));
#42478=CARTESIAN_POINT('Ctrl Pts',(3.98692409622027,-2.25426616732798,15.5304331537826));
#42479=CARTESIAN_POINT('Ctrl Pts',(3.54991271903595,-2.89402822885477,15.5039758570982));
#42480=CARTESIAN_POINT('Ctrl Pts',(2.98651869575415,-3.39031970824409,15.4775185604137));
#42481=CARTESIAN_POINT('Ctrl Pts',(2.42312467247236,-3.88661118763341,15.4510612637292));
#42482=CARTESIAN_POINT('Ctrl Pts',(1.73334800309309,-4.23943208488526,15.4246039670448));
#42483=CARTESIAN_POINT('Ctrl Pts',(1.00120272254938,-4.40580920519228,15.3981466703603));
#42484=CARTESIAN_POINT('Ctrl Pts',(0.269057442005672,-4.5721863254993,15.3716893736758));
#42485=CARTESIAN_POINT('Ctrl Pts',(-0.505456449702493,-4.55211966886149,
15.3452320769914));
#42486=CARTESIAN_POINT('Ctrl Pts',(-1.22800401774377,-4.34805333184893,
15.3187747803069));
#42487=CARTESIAN_POINT('Ctrl Pts',(-1.95055158578508,-4.14398699483636,
15.2923174836224));
#42488=CARTESIAN_POINT('Ctrl Pts',(-2.62113283015951,-3.75592097744901,
15.265860186938));
#42489=CARTESIAN_POINT('Ctrl Pts',(-3.15807169745543,-3.23112129111991,
15.2394028902535));
#42490=CARTESIAN_POINT('Ctrl Pts',(-3.69501056475133,-2.70632160479082,
15.212945593569));
#42491=CARTESIAN_POINT('Ctrl Pts',(-4.09830705496871,-2.04478824952003,
15.1864882968846));
#42492=CARTESIAN_POINT('Ctrl Pts',(-4.31884010193997,-1.3270952558398,15.1600310002001));
#42493=CARTESIAN_POINT('Ctrl Pts',(-4.53937314891122,-0.609402262159613,
15.1335737035156));
#42494=CARTESIAN_POINT('Ctrl Pts',(-4.57714275263633,0.164450369930026,
15.1071164068312));
#42495=CARTESIAN_POINT('Ctrl Pts',(-4.42754861718238,0.90020824628735,15.0806591101467));
#42496=CARTESIAN_POINT('Ctrl Pts',(-4.27795448172842,1.63596612264472,15.0542018134622));
#42497=CARTESIAN_POINT('Ctrl Pts',(-3.94099660709542,2.33362924326977,15.0277445167778));
#42498=CARTESIAN_POINT('Ctrl Pts',(-3.45771608949183,2.90822301219606,15.0012872200933));
#42499=CARTESIAN_POINT('Ctrl Pts',(-2.97443557188824,3.48281678112233,14.9748299234088));
#42500=CARTESIAN_POINT('Ctrl Pts',(-2.34483241131409,3.93434119834979,14.9483726267244));
#42501=CARTESIAN_POINT('Ctrl Pts',(-1.64559157592583,4.20780108957628,14.9219153300399));
#42502=CARTESIAN_POINT('Ctrl Pts',(-0.946350740537523,4.4812609808028,14.8954580333554));
#42503=CARTESIAN_POINT('Ctrl Pts',(-0.17747223033509,4.57665634602833,14.8690007366709));
#42504=CARTESIAN_POINT('Ctrl Pts',(0.567395403080653,4.48236813534546,14.8425434399865));
#42505=CARTESIAN_POINT('Ctrl Pts',(1.31226303649637,4.38807992466259,14.816086143302));
#42506=CARTESIAN_POINT('Ctrl Pts',(2.03311979312542,4.10410813807131,14.7896288466175));
#42507=CARTESIAN_POINT('Ctrl Pts',(2.64216611780504,3.665040224898,14.7631715499331));
#42508=CARTESIAN_POINT('Ctrl Pts',(3.25121244248463,3.22597231172472,14.7367142532486));
#42509=CARTESIAN_POINT('Ctrl Pts',(3.74844833521482,2.63180827196943,14.7102569565641));
#42510=CARTESIAN_POINT('Ctrl Pts',(4.07331101456755,1.95491662809442,14.6837996598797));
#42511=CARTESIAN_POINT('Ctrl Pts',(4.36479376317213,1.347576205805,14.6600608740838));
#42512=CARTESIAN_POINT('Ctrl Pts',(4.51750642932664,0.673635432917883,14.6363220882879));
#42513=CARTESIAN_POINT('Ctrl Pts',(4.51803303654689,-7.46219232266102E-5,
14.612583302492));
#42514=CARTESIAN_POINT('Origin',(0.,0.,20.5));
#42515=CARTESIAN_POINT('',(4.51736301819297,2.68279993319077E-6,13.612583302492));
#42516=CARTESIAN_POINT('',(4.51813640225623,-7.72658854479727E-6,13.8874166975081));
#42517=CARTESIAN_POINT('',(4.51775,5.53264807684796E-16,20.5));
#42518=CARTESIAN_POINT('Ctrl Pts',(4.51813584929441,-7.71553139285741E-6,
13.8874166975081));
#42519=CARTESIAN_POINT('Ctrl Pts',(4.5180616865618,0.743534623094937,13.9136178191666));
#42520=CARTESIAN_POINT('Ctrl Pts',(4.33069406362294,1.48711296925487,13.9398189408251));
#42521=CARTESIAN_POINT('Ctrl Pts',(3.97822152575483,2.14180184335953,13.9660200624836));
#42522=CARTESIAN_POINT('Ctrl Pts',(3.62230277429653,2.80289177698769,13.9924773591681));
#42523=CARTESIAN_POINT('Ctrl Pts',(3.0980347793188,3.37334555127586,14.0189346558525));
#42524=CARTESIAN_POINT('Ctrl Pts',(2.46927280238618,3.78368252785474,14.045391952537));
#42525=CARTESIAN_POINT('Ctrl Pts',(1.84051082545358,4.19401950443362,14.0718492492215));
#42526=CARTESIAN_POINT('Ctrl Pts',(1.10725486656609,4.44423968330323,14.0983065459059));
#42527=CARTESIAN_POINT('Ctrl Pts',(0.358814689998941,4.50386652360373,14.1247638425904));
#42528=CARTESIAN_POINT('Ctrl Pts',(-0.389625486568206,4.56349336390423,
14.1512211392749));
#42529=CARTESIAN_POINT('Ctrl Pts',(-1.15324988081502,4.43252686563563,14.1776784359594));
#42530=CARTESIAN_POINT('Ctrl Pts',(-1.83904988664919,4.12691860334233,14.2041357326438));
#42531=CARTESIAN_POINT('Ctrl Pts',(-2.52484989248339,3.82131034104901,14.2305930293283));
#42532=CARTESIAN_POINT('Ctrl Pts',(-3.13282550990494,3.34106031473099,14.2570503260128));
#42533=CARTESIAN_POINT('Ctrl Pts',(-3.58892598157751,2.74466244608609,14.2835076226972));
#42534=CARTESIAN_POINT('Ctrl Pts',(-4.04502645325008,2.14826457744119,14.3099649193817));
#42535=CARTESIAN_POINT('Ctrl Pts',(-4.34925177917366,1.43571886646941,14.3364222160662));
#42536=CARTESIAN_POINT('Ctrl Pts',(-4.46454765134644,0.693812592170538,
14.3628795127506));
#42537=CARTESIAN_POINT('Ctrl Pts',(-4.57984352351921,-0.0480936821283345,
14.3893368094351));
#42538=CARTESIAN_POINT('Ctrl Pts',(-4.50620994194118,-0.819360519754252,
14.4157941061196));
#42539=CARTESIAN_POINT('Ctrl Pts',(-4.25261539535597,-1.52604847346958,
14.442251402804));
#42540=CARTESIAN_POINT('Ctrl Pts',(-3.99902084877075,-2.23273642718488,
14.4687086994885));
#42541=CARTESIAN_POINT('Ctrl Pts',(-3.56546533717836,-2.87484549698955,
14.495165996173));
#42542=CARTESIAN_POINT('Ctrl Pts',(-3.00475544206132,-3.37416750882351,
14.5216232928574));
#42543=CARTESIAN_POINT('Ctrl Pts',(-2.44404554694427,-3.87348952065748,
14.5480805895419));
#42544=CARTESIAN_POINT('Ctrl Pts',(-1.75618126830258,-4.23002447452076,
14.5745378862264));
#42545=CARTESIAN_POINT('Ctrl Pts',(-1.02494371399391,-4.40034680762116,
14.6009951829108));
#42546=CARTESIAN_POINT('Ctrl Pts',(-0.293706159685227,-4.57066914072157,
14.6274524795953));
#42547=CARTESIAN_POINT('Ctrl Pts',(0.480904670290444,-4.5547788530591,14.6539097762798));
#42548=CARTESIAN_POINT('Ctrl Pts',(1.20454203412804,-4.35461136408475,14.6803670729642));
#42549=CARTESIAN_POINT('Ctrl Pts',(1.92817939796561,-4.15444387511041,14.7068243696487));
#42550=CARTESIAN_POINT('Ctrl Pts',(2.60084329566512,-3.76999918482422,14.7332816663332));
#42551=CARTESIAN_POINT('Ctrl Pts',(3.14060400894491,-3.24810223102607,14.7597389630176));
#42552=CARTESIAN_POINT('Ctrl Pts',(3.68036472222471,-2.72620527722791,14.7861962597021));
#42553=CARTESIAN_POINT('Ctrl Pts',(4.08722225108478,-2.0668560599178,14.8126535563866));
#42554=CARTESIAN_POINT('Ctrl Pts',(4.3116217987919,-1.35036258404174,14.839110853071));
#42555=CARTESIAN_POINT('Ctrl Pts',(4.44819168059748,-0.91430364223594,14.8552128012167));
#42556=CARTESIAN_POINT('Ctrl Pts',(4.51717991442519,-0.457078713927616,
14.8713147493624));
#42557=CARTESIAN_POINT('Ctrl Pts',(4.51743493951217,7.09613961932946E-5,
14.8874166975081));
#42558=CARTESIAN_POINT('Ctrl Pts',(4.51803303654689,-7.46219232266102E-5,
14.612583302492));
#42559=CARTESIAN_POINT('Ctrl Pts',(4.51809334238876,-0.0772263404472327,
14.6098647916034));
#42560=CARTESIAN_POINT('Ctrl Pts',(4.51615783443211,-0.154375033265316,
14.6071462807148));
#42561=CARTESIAN_POINT('Ctrl Pts',(4.51220636430248,-0.231420332178498,
14.6044277698263));
#42562=CARTESIAN_POINT('Ctrl Pts',(4.47374956870936,-0.981246400581585,
14.5779704731418));
#42563=CARTESIAN_POINT('Ctrl Pts',(4.24434651154784,-1.72127928939297,14.5515131764573));
#42564=CARTESIAN_POINT('Ctrl Pts',(3.85193823129266,-2.36138381177295,14.5250558797729));
#42565=CARTESIAN_POINT('Ctrl Pts',(3.4595299510375,-3.0014883341529,14.4985985830884));
#42566=CARTESIAN_POINT('Ctrl Pts',(2.90411644768869,-3.54166449010144,14.4721412864039));
#42567=CARTESIAN_POINT('Ctrl Pts',(2.25334647126064,-3.91611942165386,14.4456839897195));
#42568=CARTESIAN_POINT('Ctrl Pts',(1.60257649483259,-4.29057435320629,14.419226693035));
#42569=CARTESIAN_POINT('Ctrl Pts',(0.856450045325319,-4.49930806036259,
14.3927693963505));
#42570=CARTESIAN_POINT('Ctrl Pts',(0.10584449852735,-4.51689700860324,14.3663120996661));
#42571=CARTESIAN_POINT('Ctrl Pts',(-0.644761048270598,-4.53448595684389,
14.3398548029816));
#42572=CARTESIAN_POINT('Ctrl Pts',(-1.39984569235923,-4.36093014616891,
14.3133975062971));
#42573=CARTESIAN_POINT('Ctrl Pts',(-2.06744095976432,-4.01736848223886,
14.2869402096127));
#42574=CARTESIAN_POINT('Ctrl Pts',(-2.73503622716945,-3.67380681830879,
14.2604829129282));
#42575=CARTESIAN_POINT('Ctrl Pts',(-3.31514211789102,-3.16023930112366,
14.2340256162437));
#42576=CARTESIAN_POINT('Ctrl Pts',(-3.73710237646046,-2.53921788589538,
14.2075683195593));
#42577=CARTESIAN_POINT('Ctrl Pts',(-4.15906263502989,-1.91819647066709,
14.1811110228748));
#42578=CARTESIAN_POINT('Ctrl Pts',(-4.42287726144721,-1.18972115739562,
14.1546537261903));
#42579=CARTESIAN_POINT('Ctrl Pts',(-4.49641392618661,-0.442519433011148,
14.1281964295058));
#42580=CARTESIAN_POINT('Ctrl Pts',(-4.56995059092601,0.3046822913733,14.1017391328214));
#42581=CARTESIAN_POINT('Ctrl Pts',(-4.45320929398754,1.07061042687079,14.0752818361369));
#42582=CARTESIAN_POINT('Ctrl Pts',(-4.16040899613706,1.76197577425433,14.0488245394525));
#42583=CARTESIAN_POINT('Ctrl Pts',(-3.86760869828659,2.45334112163787,14.022367242768));
#42584=CARTESIAN_POINT('Ctrl Pts',(-3.39874939952411,3.07014368090745,13.9959099460835));
#42585=CARTESIAN_POINT('Ctrl Pts',(-2.81093764353767,3.53725758297869,13.969452649399));
#42586=CARTESIAN_POINT('Ctrl Pts',(-2.22312588755121,4.00437148504995,13.9429953527146));
#42587=CARTESIAN_POINT('Ctrl Pts',(-1.51636167434084,4.32179672992284,13.9165380560301));
#42588=CARTESIAN_POINT('Ctrl Pts',(-0.776728102877452,4.45087127407632,
13.8900807593456));
#42589=CARTESIAN_POINT('Ctrl Pts',(-0.0370945314140622,4.5799458182298,
13.8636234626612));
#42590=CARTESIAN_POINT('Ctrl Pts',(0.735408398302354,4.52066966166384,13.8371661659767));
#42591=CARTESIAN_POINT('Ctrl Pts',(1.44669068438533,4.2802625746454,13.8107088692922));
#42592=CARTESIAN_POINT('Ctrl Pts',(2.15797297046829,4.03985548762697,13.7842515726078));
#42593=CARTESIAN_POINT('Ctrl Pts',(2.80803461291788,3.61831747015607,13.7577942759233));
#42594=CARTESIAN_POINT('Ctrl Pts',(3.31769882312725,3.06699138623137,13.7313369792388));
#42595=CARTESIAN_POINT('Ctrl Pts',(3.82736303333661,2.51566530230669,13.7048796825544));
#42596=CARTESIAN_POINT('Ctrl Pts',(4.19662981130577,1.83455115192822,13.6784223858699));
#42597=CARTESIAN_POINT('Ctrl Pts',(4.38052287215716,1.10660788480175,13.6519650891854));
#42598=CARTESIAN_POINT('Ctrl Pts',(4.47176471220886,0.745425777992701,13.6388378269543));
#42599=CARTESIAN_POINT('Ctrl Pts',(4.5173707651647,0.372715156596874,13.6257105647231));
#42600=CARTESIAN_POINT('Ctrl Pts',(4.51736305946108,2.68251383689355E-6,
13.612583302492));
#42601=CARTESIAN_POINT('Origin',(0.,0.,20.5));
#42602=CARTESIAN_POINT('',(4.51804648040592,6.99590604930078E-5,12.612583302492));
#42603=CARTESIAN_POINT('',(4.51741195309898,-5.96473381690886E-5,12.8874166975081));
#42604=CARTESIAN_POINT('',(4.51775,5.53264807684796E-16,20.5));
#42605=CARTESIAN_POINT('Ctrl Pts',(4.51741195309898,-5.96473381690886E-5,
12.8874166975081));
#42606=CARTESIAN_POINT('Ctrl Pts',(4.51720574953279,0.442550368129689,12.9030062956018));
#42607=CARTESIAN_POINT('Ctrl Pts',(4.45260272288938,0.885219283315433,12.9185958936956));
#42608=CARTESIAN_POINT('Ctrl Pts',(4.32446175047221,1.30866046509405,12.9341854917894));
#42609=CARTESIAN_POINT('Ctrl Pts',(4.10699214642681,2.02728764889691,12.9606427884738));
#42610=CARTESIAN_POINT('Ctrl Pts',(3.70652120381657,2.69053531250561,12.9871000851583));
#42611=CARTESIAN_POINT('Ctrl Pts',(3.1718258402377,3.21762062452953,13.0135573818428));
#42612=CARTESIAN_POINT('Ctrl Pts',(2.63713047665883,3.74470593655345,13.0400146785272));
#42613=CARTESIAN_POINT('Ctrl Pts',(1.96821069211135,4.13562889699258,13.0664719752117));
#42614=CARTESIAN_POINT('Ctrl Pts',(1.24654017603871,4.34277552191208,13.0929292718962));
#42615=CARTESIAN_POINT('Ctrl Pts',(0.524869659966072,4.54992214683159,13.1193865685806));
#42616=CARTESIAN_POINT('Ctrl Pts',(-0.249551587631711,4.57329243623147,
13.1458438652651));
#42617=CARTESIAN_POINT('Ctrl Pts',(-0.98239991587342,4.41003991472745,13.1723011619496));
#42618=CARTESIAN_POINT('Ctrl Pts',(-1.71524824411517,4.24678739322342,13.198758458634));
#42619=CARTESIAN_POINT('Ctrl Pts',(-2.40652365300083,3.89691206081547,13.2252157553185));
#42620=CARTESIAN_POINT('Ctrl Pts',(-2.97202956278422,3.40302834577293,13.251673052003));
#42621=CARTESIAN_POINT('Ctrl Pts',(-3.53753547256757,2.90914463073042,13.2781303486874));
#42622=CARTESIAN_POINT('Ctrl Pts',(-3.97727188324865,2.27125253305334,13.3045876453719));
#42623=CARTESIAN_POINT('Ctrl Pts',(-4.23767938667653,1.56704660426365,13.3310449420564));
#42624=CARTESIAN_POINT('Ctrl Pts',(-4.49808689010441,0.862840675473956,
13.3575022387408));
#42625=CARTESIAN_POINT('Ctrl Pts',(-4.57916548627907,0.0923209155716644,
13.3839595354253));
#42626=CARTESIAN_POINT('Ctrl Pts',(-4.47103989191868,-0.650664221445422,
13.4104168321098));
#42627=CARTESIAN_POINT('Ctrl Pts',(-4.36291429755829,-1.39364935846249,
13.4368741287942));
#42628=CARTESIAN_POINT('Ctrl Pts',(-4.06558451266282,-2.1090998725944,13.4633314254787));
#42629=CARTESIAN_POINT('Ctrl Pts',(-3.61526497596841,-2.70987468303122,
13.4897887221632));
#42630=CARTESIAN_POINT('Ctrl Pts',(-3.16494543927398,-3.31064949346807,
13.5162460188477));
#42631=CARTESIAN_POINT('Ctrl Pts',(-2.56163615078063,-3.79674860020983,
13.5427033155321));
#42632=CARTESIAN_POINT('Ctrl Pts',(-1.87881951412554,-4.10896567003649,
13.5691606122166));
#42633=CARTESIAN_POINT('Ctrl Pts',(-1.19600287747047,-4.42118273986315,
13.5956179089011));
#42634=CARTESIAN_POINT('Ctrl Pts',(-0.43367889265364,-4.55951777277468,
13.6220752055855));
#42635=CARTESIAN_POINT('Ctrl Pts',(0.315302222661903,-4.50712171486214,
13.64853250227));
#42636=CARTESIAN_POINT('Ctrl Pts',(1.06428333797747,-4.4547256569496,13.6749897989545));
#42637=CARTESIAN_POINT('Ctrl Pts',(1.7999215837918,-4.211598508213,13.7014470956389));
#42638=CARTESIAN_POINT('Ctrl Pts',(2.43261703591854,-3.80735288629203,13.7279043923234));
#42639=CARTESIAN_POINT('Ctrl Pts',(3.06531248804526,-3.40310726437108,13.7543616890079));
#42640=CARTESIAN_POINT('Ctrl Pts',(3.59506514648438,-2.8377431692658,13.7808189856923));
#42641=CARTESIAN_POINT('Ctrl Pts',(3.95735172373184,-2.18012132205388,13.8072762823768));
#42642=CARTESIAN_POINT('Ctrl Pts',(4.3196383009793,-1.52249947484199,13.8337335790613));
#42643=CARTESIAN_POINT('Ctrl Pts',(4.51445879703509,-0.772619875523486,
13.8601908757457));
#42644=CARTESIAN_POINT('Ctrl Pts',(4.51808429109356,-0.0218170293801791,
13.8866481724302));
#42645=CARTESIAN_POINT('Ctrl Pts',(4.51811939524822,-0.0145473169490636,
13.8869043474562));
#42646=CARTESIAN_POINT('Ctrl Pts',(4.5181365744023,-0.0072775179612929,
13.8871605224821));
#42647=CARTESIAN_POINT('Ctrl Pts',(4.51813584929441,-7.71553139285741E-6,
13.8874166975081));
#42648=CARTESIAN_POINT('Ctrl Pts',(4.51736305946108,2.68251383689355E-6,
13.612583302492));
#42649=CARTESIAN_POINT('Ctrl Pts',(4.51735523473014,-0.378466950622669,
13.5992532680387));
#42650=CARTESIAN_POINT('Ctrl Pts',(4.47031360843327,-0.756938494124053,
13.5859232335853));
#42651=CARTESIAN_POINT('Ctrl Pts',(4.37626124565255,-1.12334284793068,13.572593199132));
#42652=CARTESIAN_POINT('Ctrl Pts',(4.18958721456293,-1.85057792966208,13.5461359024476));
#42653=CARTESIAN_POINT('Ctrl Pts',(3.81771980865007,-2.53027570925035,13.5196786057631));
#42654=CARTESIAN_POINT('Ctrl Pts',(3.3059520663969,-3.07964974938441,13.4932213090786));
#42655=CARTESIAN_POINT('Ctrl Pts',(2.79418432414376,-3.62902378951843,13.4667640123941));
#42656=CARTESIAN_POINT('Ctrl Pts',(2.14251624555032,-4.04807409019825,13.4403067157097));
#42657=CARTESIAN_POINT('Ctrl Pts',(1.43032028136785,-4.28576078857712,13.4138494190252));
#42658=CARTESIAN_POINT('Ctrl Pts',(0.718124317185353,-4.523447486956,13.3873921223408));
#42659=CARTESIAN_POINT('Ctrl Pts',(-0.0545995325861841,-4.57977058303392,
13.3609348256563));
#42660=CARTESIAN_POINT('Ctrl Pts',(-0.793734358242206,-4.44786998604312,
13.3344775289718));
#42661=CARTESIAN_POINT('Ctrl Pts',(-1.53286918389827,-4.31596938905231,
13.3080202322873));
#42662=CARTESIAN_POINT('Ctrl Pts',(-2.23841498543881,-3.99584509899276,
13.2815629356029));
#42663=CARTESIAN_POINT('Ctrl Pts',(-2.82443706508576,-3.52648790010218,
13.2551056389184));
#42664=CARTESIAN_POINT('Ctrl Pts',(-3.41045914473268,-3.05713070121163,
13.2286483422339));
#42665=CARTESIAN_POINT('Ctrl Pts',(-3.87695750248602,-2.43854059349005,
13.2021910455495));
#42666=CARTESIAN_POINT('Ctrl Pts',(-4.16711315465972,-1.74606116744496,
13.175733748865));
#42667=CARTESIAN_POINT('Ctrl Pts',(-4.45726880683343,-1.05358174139987,
13.1492764521805));
#42668=CARTESIAN_POINT('Ctrl Pts',(-4.57108175342749,-0.287212997031258,
13.1228191554961));
#42669=CARTESIAN_POINT('Ctrl Pts',(-4.49468970350711,0.459702200761001,
13.0963618588116));
#42670=CARTESIAN_POINT('Ctrl Pts',(-4.41829765358673,1.20661739855328,13.0699045621271));
#42671=CARTESIAN_POINT('Ctrl Pts',(-4.15170060715189,1.93407904976921,13.0434472654427));
#42672=CARTESIAN_POINT('Ctrl Pts',(-3.72736978940707,2.5534831303952,13.0169899687582));
#42673=CARTESIAN_POINT('Ctrl Pts',(-3.30303897166226,3.1728872110212,12.9905326720737));
#42674=CARTESIAN_POINT('Ctrl Pts',(-2.72097438260746,3.68423372105726,12.9640753753893));
#42675=CARTESIAN_POINT('Ctrl Pts',(-2.05207084500052,4.02524122150415,12.9376180787048));
#42676=CARTESIAN_POINT('Ctrl Pts',(-1.3831673073936,4.36624872195103,12.9111607820203));
#42677=CARTESIAN_POINT('Ctrl Pts',(-0.627424821234523,4.53691721280875,
12.8847034853359));
#42678=CARTESIAN_POINT('Ctrl Pts',(0.123108015066336,4.51645946077498,12.8582461886514));
#42679=CARTESIAN_POINT('Ctrl Pts',(0.873640851367194,4.49600170874121,12.8317888919669));
#42680=CARTESIAN_POINT('Ctrl Pts',(1.61896403780984,4.28441771381596,12.8053315952824));
#42681=CARTESIAN_POINT('Ctrl Pts',(2.268298035158,3.9074781724145,12.778874298598));
#42682=CARTESIAN_POINT('Ctrl Pts',(2.91763203250619,3.53053863101303,12.7524170019135));
#42683=CARTESIAN_POINT('Ctrl Pts',(3.47097684075988,2.98824354313534,12.7259597052291));
#42684=CARTESIAN_POINT('Ctrl Pts',(3.86093567467777,2.34664385031004,12.6995024085446));
#42685=CARTESIAN_POINT('Ctrl Pts',(4.25089450859566,1.70504415748472,12.6730451118601));
#42686=CARTESIAN_POINT('Ctrl Pts',(4.47746736817774,0.964139859711776,12.6465878151756));
#42687=CARTESIAN_POINT('Ctrl Pts',(4.51305792988216,0.214172280478037,12.6201305184912));
#42688=CARTESIAN_POINT('Ctrl Pts',(4.51644212114351,0.142860291950876,12.6176147798248));
#42689=CARTESIAN_POINT('Ctrl Pts',(4.51809954743677,0.0714663578345357,
12.6150990411584));
#42690=CARTESIAN_POINT('Ctrl Pts',(4.51804648040592,6.99590604930078E-5,
12.612583302492));
#42691=CARTESIAN_POINT('Origin',(0.,0.,20.5));
#42692=CARTESIAN_POINT('',(4.5175801641472,-0.000107849321499542,11.612583302492));
#42693=CARTESIAN_POINT('',(4.5178502562812,0.000110962492481057,11.8874166975081));
#42694=CARTESIAN_POINT('',(4.51775,5.53264807684796E-16,20.5));
#42695=CARTESIAN_POINT('Ctrl Pts',(4.5178502562812,0.000110962492481057,
11.8874166975081));
#42696=CARTESIAN_POINT('Ctrl Pts',(4.51799453028332,0.141405931765494,11.8923947720371));
#42697=CARTESIAN_POINT('Ctrl Pts',(4.51149711848843,0.282687684813822,11.8973728465661));
#42698=CARTESIAN_POINT('Ctrl Pts',(4.49826065670895,0.423335220010937,11.9023509210951));
#42699=CARTESIAN_POINT('Ctrl Pts',(4.42791197182862,1.17084382900464,11.9288082177796));
#42700=CARTESIAN_POINT('Ctrl Pts',(4.16720717585505,1.90043785893767,11.955265514464));
#42701=CARTESIAN_POINT('Ctrl Pts',(3.7478998244077,2.5232535644287,11.9817228111485));
#42702=CARTESIAN_POINT('Ctrl Pts',(3.32859247296032,3.14606926991974,12.008180107833));
#42703=CARTESIAN_POINT('Ctrl Pts',(2.75068256603915,3.66210665096878,12.0346374045175));
#42704=CARTESIAN_POINT('Ctrl Pts',(2.08455889071624,4.00851292567871,12.0610947012019));
#42705=CARTESIAN_POINT('Ctrl Pts',(1.41843521539332,4.35491920038864,12.0875519978864));
#42706=CARTESIAN_POINT('Ctrl Pts',(0.664097771668666,4.53169436875946,12.1140092945709));
#42707=CARTESIAN_POINT('Ctrl Pts',(-0.0865759746608722,4.51730741092621,
12.1404665912553));
#42708=CARTESIAN_POINT('Ctrl Pts',(-0.83724972099039,4.50292045309296,12.1669238879398));
#42709=CARTESIAN_POINT('Ctrl Pts',(-1.58425976992479,4.29737136905566,12.1933811846243));
#42710=CARTESIAN_POINT('Ctrl Pts',(-2.23662112424321,3.92569580976245,12.2198384813087));
#42711=CARTESIAN_POINT('Ctrl Pts',(-2.88898247856163,3.55402025046923,12.2462957779932));
#42712=CARTESIAN_POINT('Ctrl Pts',(-3.44669513826407,3.01621821592011,12.2727530746777));
#42713=CARTESIAN_POINT('Ctrl Pts',(-3.84183031863679,2.37779339872086,12.2992103713621));
#42714=CARTESIAN_POINT('Ctrl Pts',(-4.23696549900952,1.7393685815216,12.3256676680466));
#42715=CARTESIAN_POINT('Ctrl Pts',(-4.46952320005253,1.00032098167222,12.3521249647311));
#42716=CARTESIAN_POINT('Ctrl Pts',(-4.51117815115765,0.250665778907295,
12.3785822614155));
#42717=CARTESIAN_POINT('Ctrl Pts',(-4.55283310226278,-0.498989423857626,
12.4050395581));
#42718=CARTESIAN_POINT('Ctrl Pts',(-4.40358530343001,-1.25925222953809,
12.4314968547845));
#42719=CARTESIAN_POINT('Ctrl Pts',(-4.08161297138,-1.93752346980879,12.4579541514689));
#42720=CARTESIAN_POINT('Ctrl Pts',(-3.75964063932998,-2.61579471007952,
12.4844114481534));
#42721=CARTESIAN_POINT('Ctrl Pts',(-3.26494377406269,-3.21207438494048,
12.5108687448379));
#42722=CARTESIAN_POINT('Ctrl Pts',(-2.65777590627122,-3.65373628991496,
12.5373260415223));
#42723=CARTESIAN_POINT('Ctrl Pts',(-2.05060803847976,-4.09539819488944,
12.5637833382068));
#42724=CARTESIAN_POINT('Ctrl Pts',(-1.33096916816412,-4.38244232997743,
12.5902406348913));
#42725=CARTESIAN_POINT('Ctrl Pts',(-0.586510513281939,-4.47990703720592,
12.6166979315757));
#42726=CARTESIAN_POINT('Ctrl Pts',(0.15794814160022,-4.57737174443441,12.6431552282602));
#42727=CARTESIAN_POINT('Ctrl Pts',(0.927226581048916,-4.48525702380341,
12.6696125249447));
#42728=CARTESIAN_POINT('Ctrl Pts',(1.62762754252377,-4.21478234633953,12.6960698216291));
#42729=CARTESIAN_POINT('Ctrl Pts',(2.32802850399863,-3.94430766887566,12.7225271183136));
#42730=CARTESIAN_POINT('Ctrl Pts',(2.95955198749964,-3.49547303457892,12.7489844149981));
#42731=CARTESIAN_POINT('Ctrl Pts',(3.44527913166315,-2.92294600516735,12.7754417116826));
#42732=CARTESIAN_POINT('Ctrl Pts',(3.93100627582668,-2.35041897575576,12.801899008367));
#42733=CARTESIAN_POINT('Ctrl Pts',(4.2709370806527,-1.65419955122932,12.8283563050515));
#42734=CARTESIAN_POINT('Ctrl Pts',(4.42366835032544,-0.919086486967588,
12.854813601736));
#42735=CARTESIAN_POINT('Ctrl Pts',(4.48640482049374,-0.617128682745771,
12.8656813003267));
#42736=CARTESIAN_POINT('Ctrl Pts',(4.51755570011492,-0.308608476653881,
12.8765489989174));
#42737=CARTESIAN_POINT('Ctrl Pts',(4.51741195309898,-5.96473381690886E-5,
12.8874166975081));
#42738=CARTESIAN_POINT('Ctrl Pts',(4.51804648040592,6.99590604930078E-5,
12.612583302492));
#42739=CARTESIAN_POINT('Ctrl Pts',(4.51754145680588,-0.679388939577024,
12.5886417444739));
#42740=CARTESIAN_POINT('Ctrl Pts',(4.36212083370235,-1.35907105681478,12.5647001864558));
#42741=CARTESIAN_POINT('Ctrl Pts',(4.06580926285153,-1.97047118281595,12.5407586284378));
#42742=CARTESIAN_POINT('Ctrl Pts',(3.73836177028969,-2.64611620618181,12.5143013317533));
#42743=CARTESIAN_POINT('Ctrl Pts',(3.23885852133923,-3.23837539221903,12.4878440350688));
#42744=CARTESIAN_POINT('Ctrl Pts',(2.62813845890645,-3.67511222754003,12.4613867383844));
#42745=CARTESIAN_POINT('Ctrl Pts',(2.01741839647366,-4.11184906286103,12.4349294416999));
#42746=CARTESIAN_POINT('Ctrl Pts',(1.29548152055856,-4.3930635474658,12.4084721450154));
#42747=CARTESIAN_POINT('Ctrl Pts',(0.550258943657521,-4.48450406835832,
12.382014848331));
#42748=CARTESIAN_POINT('Ctrl Pts',(-0.194963633243496,-4.57594458925083,
12.3555575516465));
#42749=CARTESIAN_POINT('Ctrl Pts',(-0.963471911130448,-4.47761114643111,
12.329100254962));
#42750=CARTESIAN_POINT('Ctrl Pts',(-1.66166243228881,-4.2014806444059,12.3026429582776));
#42751=CARTESIAN_POINT('Ctrl Pts',(-2.35985295344718,-3.92535014238069,
12.2761856615931));
#42752=CARTESIAN_POINT('Ctrl Pts',(-2.98772571787696,-3.47142258114999,
12.2497283649086));
#42753=CARTESIAN_POINT('Ctrl Pts',(-3.46880651775701,-2.89498583529589,
12.2232710682242));
#42754=CARTESIAN_POINT('Ctrl Pts',(-3.94988731763707,-2.31854908944178,
12.1968137715397));
#42755=CARTESIAN_POINT('Ctrl Pts',(-4.28417615296739,-1.61960315896426,
12.1703564748552));
#42756=CARTESIAN_POINT('Ctrl Pts',(-4.43095701357263,-0.883278884650216,
12.1438991781708));
#42757=CARTESIAN_POINT('Ctrl Pts',(-4.57773787417786,-0.146954610336191,
12.1174418814863));
#42758=CARTESIAN_POINT('Ctrl Pts',(-4.53701076005802,0.626748007814359,
12.0909845848018));
#42759=CARTESIAN_POINT('Ctrl Pts',(-4.31373618863893,1.34359284719155,12.0645272881174));
#42760=CARTESIAN_POINT('Ctrl Pts',(-4.09046161721984,2.06043768656874,12.0380699914329));
#42761=CARTESIAN_POINT('Ctrl Pts',(-3.6846395885015,2.72042474717257,12.0116126947484));
#42762=CARTESIAN_POINT('Ctrl Pts',(-3.1456987764459,3.24316833544978,11.985155398064));
#42763=CARTESIAN_POINT('Ctrl Pts',(-2.60675796439029,3.76591192372701,11.9586981013795));
#42764=CARTESIAN_POINT('Ctrl Pts',(-1.9346983689974,4.15141203967762,11.932240804695));
#42765=CARTESIAN_POINT('Ctrl Pts',(-1.21137610519676,4.35271519582384,11.9057835080105));
#42766=CARTESIAN_POINT('Ctrl Pts',(-0.488053841396109,4.55401835197005,
11.8793262113261));
#42767=CARTESIAN_POINT('Ctrl Pts',(0.286531090812296,4.57112454831187,11.8528689146416));
#42768=CARTESIAN_POINT('Ctrl Pts',(1.0180351039428,4.40195026906683,11.8264116179572));
#42769=CARTESIAN_POINT('Ctrl Pts',(1.74953911707329,4.2327759898218,11.7999543212727));
#42770=CARTESIAN_POINT('Ctrl Pts',(2.43796221112589,3.8773212349899,11.7734970245882));
#42771=CARTESIAN_POINT('Ctrl Pts',(2.99945521514432,3.37888000031681,11.7470397279037));
#42772=CARTESIAN_POINT('Ctrl Pts',(3.56094821916276,2.88043876564371,11.7205824312193));
#42773=CARTESIAN_POINT('Ctrl Pts',(3.99551113314703,2.23901105112941,11.6941251345348));
#42774=CARTESIAN_POINT('Ctrl Pts',(4.2502146751182,1.53272204251365,11.6676678378503));
#42775=CARTESIAN_POINT('Ctrl Pts',(4.42698035695052,1.0425535226241,11.6493063260642));
#42776=CARTESIAN_POINT('Ctrl Pts',(4.51711789485057,0.521144965264365,11.6309448142781));
#42777=CARTESIAN_POINT('Ctrl Pts',(4.5175801641472,-0.000107849321499542,
11.612583302492));
#42778=CARTESIAN_POINT('Origin',(0.,0.,20.5));
#42779=CARTESIAN_POINT('',(4.517607537138,0.000111184246189833,10.612583302492));
#42780=CARTESIAN_POINT('',(4.51779144669394,-0.000115517084662978,10.8874166975081));
#42781=CARTESIAN_POINT('',(4.51775,5.53264807684796E-16,20.5));
#42782=CARTESIAN_POINT('Ctrl Pts',(4.51779144669394,-0.000115517084662978,
10.8874166975081));
#42783=CARTESIAN_POINT('Ctrl Pts',(4.51718124885461,0.590959459307199,10.9082405451568));
#42784=CARTESIAN_POINT('Ctrl Pts',(4.40057028871007,1.18226809182004,10.9290643928055));
#42785=CARTESIAN_POINT('Ctrl Pts',(4.17452335103026,1.72826978099499,10.9498882404543));
#42786=CARTESIAN_POINT('Ctrl Pts',(3.88732422262257,2.42198061313325,10.9763455371387));
#42787=CARTESIAN_POINT('Ctrl Pts',(3.42346880605941,3.0425550177638,11.0028028338232));
#42788=CARTESIAN_POINT('Ctrl Pts',(2.83945417771489,3.51440771921171,11.0292601305077));
#42789=CARTESIAN_POINT('Ctrl Pts',(2.25543954937037,3.98626042065963,11.0557174271921));
#42790=CARTESIAN_POINT('Ctrl Pts',(1.55126570924448,4.30939141892491,11.0821747238766));
#42791=CARTESIAN_POINT('Ctrl Pts',(0.812700251733397,4.44444371603802,11.1086320205611));
#42792=CARTESIAN_POINT('Ctrl Pts',(0.0741347942222902,4.57949601315113,
11.1350893172455));
#42793=CARTESIAN_POINT('Ctrl Pts',(-0.698822280674023,4.52646960911206,
11.16154661393));
#42794=CARTESIAN_POINT('Ctrl Pts',(-1.41202565668891,4.29182306124677,11.1880039106145));
#42795=CARTESIAN_POINT('Ctrl Pts',(-2.12522903270377,4.0571765133815,11.2144612072989));
#42796=CARTESIAN_POINT('Ctrl Pts',(-2.7786787098372,3.64090982169003,11.2409185039834));
#42797=CARTESIAN_POINT('Ctrl Pts',(-3.29278524060752,3.09372380852504,11.2673758006679));
#42798=CARTESIAN_POINT('Ctrl Pts',(-3.80689177137783,2.54653779536005,11.2938330973523));
#42799=CARTESIAN_POINT('Ctrl Pts',(-4.18165515578503,1.86843246072154,11.3202903940368));
#42800=CARTESIAN_POINT('Ctrl Pts',(-4.37142962837066,1.14200028388812,11.3467476907213));
#42801=CARTESIAN_POINT('Ctrl Pts',(-4.56120410095629,0.415568107054687,
11.3732049874058));
#42802=CARTESIAN_POINT('Ctrl Pts',(-4.56598966172034,-0.359190911973653,
11.3996622840902));
#42803=CARTESIAN_POINT('Ctrl Pts',(-4.38520343465808,-1.08791198212924,
11.4261195807747));
#42804=CARTESIAN_POINT('Ctrl Pts',(-4.20441720759582,-1.81663305228484,
11.4525768774592));
#42805=CARTESIAN_POINT('Ctrl Pts',(-3.83805919270723,-2.49931617356768,
11.4790341741436));
#42806=CARTESIAN_POINT('Ctrl Pts',(-3.33075139074592,-3.05281129735225,
11.5054914708281));
#42807=CARTESIAN_POINT('Ctrl Pts',(-2.82344358878461,-3.6063064211368,11.5319487675126));
#42808=CARTESIAN_POINT('Ctrl Pts',(-2.17518599975058,-4.03061354742309,
11.558406064197));
#42809=CARTESIAN_POINT('Ctrl Pts',(-1.46493568054124,-4.27405253782339,
11.5848633608815));
#42810=CARTESIAN_POINT('Ctrl Pts',(-0.7546853613319,-4.51749152822369,11.611320657566));
#42811=CARTESIAN_POINT('Ctrl Pts',(0.017557688052746,-4.580062382738,11.6377779542504));
#42812=CARTESIAN_POINT('Ctrl Pts',(0.757735118863148,-4.4541440405356,11.6642352509349));
#42813=CARTESIAN_POINT('Ctrl Pts',(1.49791254967357,-4.3282256983332,11.6906925476194));
#42814=CARTESIAN_POINT('Ctrl Pts',(2.20602436190975,-4.01381815941408,11.7171498443038));
#42815=CARTESIAN_POINT('Ctrl Pts',(2.79582332053076,-3.54921591405394,11.7436071409883));
#42816=CARTESIAN_POINT('Ctrl Pts',(3.38562227915178,-3.0846136686938,11.7700644376728));
#42817=CARTESIAN_POINT('Ctrl Pts',(3.85710838415764,-2.46981671689265,11.7965217343572));
#42818=CARTESIAN_POINT('Ctrl Pts',(4.15285514976701,-1.77970664696488,11.8229790310417));
#42819=CARTESIAN_POINT('Ctrl Pts',(4.39295566177474,-1.21944428605644,11.8444582531972));
#42820=CARTESIAN_POINT('Ctrl Pts',(4.51722774785459,-0.609543637247958,
11.8659374753526));
#42821=CARTESIAN_POINT('Ctrl Pts',(4.5178502562812,0.000110962492481057,
11.8874166975081));
#42822=CARTESIAN_POINT('Ctrl Pts',(4.5175801641472,-0.000107849321499542,
11.612583302492));
#42823=CARTESIAN_POINT('Ctrl Pts',(4.51778398357309,-0.229933732598545,
11.6044875175936));
#42824=CARTESIAN_POINT('Ctrl Pts',(4.50055473854231,-0.45972933914648,11.5963917326953));
#42825=CARTESIAN_POINT('Ctrl Pts',(4.46563124792392,-0.686803612223187,
11.5882959477969));
#42826=CARTESIAN_POINT('Ctrl Pts',(4.35150010880038,-1.42888995562703,11.5618386511125));
#42827=CARTESIAN_POINT('Ctrl Pts',(4.04839366059521,-2.14191233971748,11.535381354428));
#42828=CARTESIAN_POINT('Ctrl Pts',(3.59322993324244,-2.73902542723646,11.5089240577435));
#42829=CARTESIAN_POINT('Ctrl Pts',(3.13806620588969,-3.33613851475543,11.4824667610591));
#42830=CARTESIAN_POINT('Ctrl Pts',(2.53084519938934,-3.81734230570294,11.4560094643746));
#42831=CARTESIAN_POINT('Ctrl Pts',(1.84552576030269,-4.12402671090484,11.4295521676901));
#42832=CARTESIAN_POINT('Ctrl Pts',(1.16020632121604,-4.43071111610674,11.4030948710056));
#42833=CARTESIAN_POINT('Ctrl Pts',(0.396788449543078,-4.56287613556304,
11.3766375743212));
#42834=CARTESIAN_POINT('Ctrl Pts',(-0.351744402844812,-4.50442421617511,
11.3501802776367));
#42835=CARTESIAN_POINT('Ctrl Pts',(-1.10027725523272,-4.44597229678718,
11.3237229809523));
#42836=CARTESIAN_POINT('Ctrl Pts',(-1.83392508833558,-4.196903438555,11.2972656842678));
#42837=CARTESIAN_POINT('Ctrl Pts',(-2.4633304080324,-3.787553952759,11.2708083875833));
#42838=CARTESIAN_POINT('Ctrl Pts',(-3.0927357277292,-3.378204466963,11.2443510908988));
#42839=CARTESIAN_POINT('Ctrl Pts',(-3.61789853401999,-2.80857435360317,
11.2178937942144));
#42840=CARTESIAN_POINT('Ctrl Pts',(-3.97485457831262,-2.1480439300593,11.1914364975299));
#42841=CARTESIAN_POINT('Ctrl Pts',(-4.33181062260526,-1.48751350651541,
11.1649792008454));
#42842=CARTESIAN_POINT('Ctrl Pts',(-4.52055990489972,-0.736082772787468,
11.138521904161));
#42843=CARTESIAN_POINT('Ctrl Pts',(-4.51811297150728,0.0147248393883086,
11.1120646074765));
#42844=CARTESIAN_POINT('Ctrl Pts',(-4.51566603811484,0.765532451564064,
11.085607310792));
#42845=CARTESIAN_POINT('Ctrl Pts',(-4.32202288903552,1.5157169421876,11.0591500141076));
#42846=CARTESIAN_POINT('Ctrl Pts',(-3.96076904551623,2.17390667055369,11.0326927174231));
#42847=CARTESIAN_POINT('Ctrl Pts',(-3.59951520199693,2.83209639891979,11.0062354207386));
#42848=CARTESIAN_POINT('Ctrl Pts',(-3.07065066403766,3.3982913650284,10.9797781240542));
#42849=CARTESIAN_POINT('Ctrl Pts',(-2.43859054705097,3.8035296486331,10.9533208273697));
#42850=CARTESIAN_POINT('Ctrl Pts',(-1.8065304300643,4.20876793223779,10.9268635306852));
#42851=CARTESIAN_POINT('Ctrl Pts',(-1.0712747340502,4.4530495333386,10.9004062340008));
#42852=CARTESIAN_POINT('Ctrl Pts',(-0.322376789052762,4.50662122327553,
10.8739489373163));
#42853=CARTESIAN_POINT('Ctrl Pts',(0.426521155944698,4.56019291321245,10.8474916406318));
#42854=CARTESIAN_POINT('Ctrl Pts',(1.18906134992551,4.42305469198549,10.8210343439474));
#42855=CARTESIAN_POINT('Ctrl Pts',(1.87236724118984,4.11190984316492,10.7945770472629));
#42856=CARTESIAN_POINT('Ctrl Pts',(2.55567313245417,3.80076499434435,10.7681197505784));
#42857=CARTESIAN_POINT('Ctrl Pts',(3.15974472100203,3.31561351793017,10.741662453894));
#42858=CARTESIAN_POINT('Ctrl Pts',(3.61100675589317,2.71554632681736,10.7152051572095));
#42859=CARTESIAN_POINT('Ctrl Pts',(4.0622687907843,2.11547913570456,10.688747860525));
#42860=CARTESIAN_POINT('Ctrl Pts',(4.36072127201872,1.40049622989312,10.6622905638405));
#42861=CARTESIAN_POINT('Ctrl Pts',(4.47001301768877,0.657681736016976,10.6358332671561));
#42862=CARTESIAN_POINT('Ctrl Pts',(4.5020272386327,0.440093233047143,10.6280832789347));
#42863=CARTESIAN_POINT('Ctrl Pts',(4.51781057668589,0.220116648612125,10.6203332907133));
#42864=CARTESIAN_POINT('Ctrl Pts',(4.517607537138,0.000111184246189833,
10.612583302492));
#42865=CARTESIAN_POINT('Origin',(0.,0.,20.5));
#42866=CARTESIAN_POINT('',(4.51802315729813,-7.77880120685776E-5,9.61258330249199));
#42867=CARTESIAN_POINT('',(4.5174420818448,7.39595355181285E-5,9.88741669750808));
#42868=CARTESIAN_POINT('',(4.51775,5.53264807684796E-16,20.5));
#42869=CARTESIAN_POINT('Ctrl Pts',(4.5174420818448,7.39595355181285E-5,
9.88741669750808));
#42870=CARTESIAN_POINT('Ctrl Pts',(4.51761100468578,0.290010274247371,9.89762902159206));
#42871=CARTESIAN_POINT('Ctrl Pts',(4.49012793116805,0.579914973420611,9.90784134567604));
#42872=CARTESIAN_POINT('Ctrl Pts',(4.43468447094956,0.864369878764984,9.91805366976002));
#42873=CARTESIAN_POINT('Ctrl Pts',(4.29104585704042,1.60131357171471,9.94451096644449));
#42874=CARTESIAN_POINT('Ctrl Pts',(3.95974153092839,2.30167910674412,9.97096826312895));
#42875=CARTESIAN_POINT('Ctrl Pts',(3.48112399286906,2.88016273680304,9.99742555981342));
#42876=CARTESIAN_POINT('Ctrl Pts',(3.00250645480973,3.45864636686196,10.0238828564979));
#42877=CARTESIAN_POINT('Ctrl Pts',(2.3765757048031,3.91524809195038,10.0503401531824));
#42878=CARTESIAN_POINT('Ctrl Pts',(1.67956941546288,4.19435432728793,10.0767974498668));
#42879=CARTESIAN_POINT('Ctrl Pts',(0.982563126122689,4.47346056262548,10.1032547465513));
#42880=CARTESIAN_POINT('Ctrl Pts',(0.214481297448898,4.57507130821216,10.1297120432358));
#42881=CARTESIAN_POINT('Ctrl Pts',(-0.531124553886154,4.4868104876913,10.1561693399202));
#42882=CARTESIAN_POINT('Ctrl Pts',(-1.27673040522121,4.39854966717044,10.1826266366047));
#42883=CARTESIAN_POINT('Ctrl Pts',(-1.99986027921753,4.12041728054204,10.2090839332892));
#42884=CARTESIAN_POINT('Ctrl Pts',(-2.61243775753278,3.68628954467964,10.2355412299736));
#42885=CARTESIAN_POINT('Ctrl Pts',(-3.22501523584806,3.25216180881724,10.2619985266581));
#42886=CARTESIAN_POINT('Ctrl Pts',(-3.72704031848226,2.66203872372082,10.2884558233426));
#42887=CARTESIAN_POINT('Ctrl Pts',(-4.05736690597737,1.9877966280475,10.314913120027));
#42888=CARTESIAN_POINT('Ctrl Pts',(-4.38769349347249,1.31355453237416,10.3413704167115));
#42889=CARTESIAN_POINT('Ctrl Pts',(-4.54632158582851,0.555193426123966,
10.367827713396));
#42890=CARTESIAN_POINT('Ctrl Pts',(-4.51393045695515,-0.194919147263826,
10.3942850100804));
#42891=CARTESIAN_POINT('Ctrl Pts',(-4.48153932808179,-0.945031720651576,
10.4207423067649));
#42892=CARTESIAN_POINT('Ctrl Pts',(-4.25812897797905,-1.68689576117688,
10.4471996034494));
#42893=CARTESIAN_POINT('Ctrl Pts',(-3.87091054003425,-2.33015304974784,
10.4736569001339));
#42894=CARTESIAN_POINT('Ctrl Pts',(-3.48369210208944,-2.9734103383188,10.5001141968183));
#42895=CARTESIAN_POINT('Ctrl Pts',(-2.93266557630255,-3.51806087493544,
10.5265714935028));
#42896=CARTESIAN_POINT('Ctrl Pts',(-2.28494538367617,-3.89776682701959,
10.5530287901872));
#42897=CARTESIAN_POINT('Ctrl Pts',(-1.63722519104977,-4.27747277910375,
10.5794860868717));
#42898=CARTESIAN_POINT('Ctrl Pts',(-0.892811331583869,-4.49223414665542,
10.6059433835562));
#42899=CARTESIAN_POINT('Ctrl Pts',(-0.142372589495352,-4.51589323278992,
10.6324006802407));
#42900=CARTESIAN_POINT('Ctrl Pts',(0.608066152593165,-4.53955231892441,
10.6588579769251));
#42901=CARTESIAN_POINT('Ctrl Pts',(1.36452977730431,-4.37210912364174,10.6853152736096));
#42902=CARTESIAN_POINT('Ctrl Pts',(2.03488185235016,-4.03395804281271,10.7117725702941));
#42903=CARTESIAN_POINT('Ctrl Pts',(2.70523392739599,-3.6958069619837,10.7382298669785));
#42904=CARTESIAN_POINT('Ctrl Pts',(3.28947445277654,-3.18694799560833,10.764687163663));
#42905=CARTESIAN_POINT('Ctrl Pts',(3.71644357909769,-2.56935960262103,10.7911444603475));
#42906=CARTESIAN_POINT('Ctrl Pts',(4.14341270541885,-1.95177120963373,10.8176017570319));
#42907=CARTESIAN_POINT('Ctrl Pts',(4.41311043268061,-1.22545339003449,10.8440590537164));
#42908=CARTESIAN_POINT('Ctrl Pts',(4.49268787618539,-0.478870850411892,
10.8705163504009));
#42909=CARTESIAN_POINT('Ctrl Pts',(4.50963199098762,-0.319903940901298,
10.8761497994366));
#42910=CARTESIAN_POINT('Ctrl Pts',(4.51795652273981,-0.160018279147252,
10.8817832484723));
#42911=CARTESIAN_POINT('Ctrl Pts',(4.51779144669394,-0.000115517084662978,
10.8874166975081));
#42912=CARTESIAN_POINT('Ctrl Pts',(4.517607537138,0.000111184246189833,
10.612583302492));
#42913=CARTESIAN_POINT('Ctrl Pts',(4.51711743014117,-0.530948988737395,
10.5938759940289));
#42914=CARTESIAN_POINT('Ctrl Pts',(4.42347995325767,-1.06217743558981,10.5751686855658));
#42915=CARTESIAN_POINT('Ctrl Pts',(4.24013400258143,-1.56039266992325,10.5564613771027));
#42916=CARTESIAN_POINT('Ctrl Pts',(3.98083223169834,-2.26500650004656,10.5300040804182));
#42917=CARTESIAN_POINT('Ctrl Pts',(3.54209767982647,-2.90358807835227,10.5035467837338));
#42918=CARTESIAN_POINT('Ctrl Pts',(2.9773677298226,-3.39835887534092,10.4770894870493));
#42919=CARTESIAN_POINT('Ctrl Pts',(2.41263777981875,-3.89312967232955,10.4506321903648));
#42920=CARTESIAN_POINT('Ctrl Pts',(1.7219124316829,-4.24408968800111,10.4241748936803));
#42921=CARTESIAN_POINT('Ctrl Pts',(0.989321268370679,-4.40849238086523,
10.3977175969959));
#42922=CARTESIAN_POINT('Ctrl Pts',(0.256730105058482,-4.57289507372935,
10.3712603003114));
#42923=CARTESIAN_POINT('Ctrl Pts',(-0.517726873430066,-4.55074044378602,
10.3448030036269));
#42924=CARTESIAN_POINT('Ctrl Pts',(-1.2397216642308,-4.34472690044313,10.3183457069425));
#42925=CARTESIAN_POINT('Ctrl Pts',(-1.96171645503154,-4.13871335710024,
10.291888410258));
#42926=CARTESIAN_POINT('Ctrl Pts',(-2.63124905814445,-3.74884090035779,
10.2654311135735));
#42927=CARTESIAN_POINT('Ctrl Pts',(-3.16677114350303,-3.22259556396298,
10.2389738168891));
#42928=CARTESIAN_POINT('Ctrl Pts',(-3.70229322886161,-2.69635022756818,
10.2125165202046));
#42929=CARTESIAN_POINT('Ctrl Pts',(-4.10380479646586,-2.033732011521,10.1860592235201));
#42930=CARTESIAN_POINT('Ctrl Pts',(-4.32240218174696,-1.31544708119576,
10.1596019268357));
#42931=CARTESIAN_POINT('Ctrl Pts',(-4.54099956702807,-0.597162150870509,
10.1331446301512));
#42932=CARTESIAN_POINT('Ctrl Pts',(-4.57668276998605,0.176789493732823,
10.1066873334667));
#42933=CARTESIAN_POINT('Ctrl Pts',(-4.42510561599232,0.912141398858014,
10.0802300367823));
#42934=CARTESIAN_POINT('Ctrl Pts',(-4.27352846199858,1.64749330398323,10.0537727400978));
#42935=CARTESIAN_POINT('Ctrl Pts',(-3.93469095105313,2.34424546963029,10.0273154434133));
#42936=CARTESIAN_POINT('Ctrl Pts',(-3.44986311698706,2.91753425314077,10.0008581467289));
#42937=CARTESIAN_POINT('Ctrl Pts',(-2.965035282921,3.49082303665126,9.97440085004439));
#42938=CARTESIAN_POINT('Ctrl Pts',(-2.33421712573433,3.94064843802516,9.94794355335992));
#42939=CARTESIAN_POINT('Ctrl Pts',(-1.63424159882622,4.21222222121095,9.92148625667545));
#42940=CARTESIAN_POINT('Ctrl Pts',(-0.93426607191815,4.48379600439673,9.89502895999098));
#42941=CARTESIAN_POINT('Ctrl Pts',(-0.165133175288626,4.57711816939442,
9.86857166330652));
#42942=CARTESIAN_POINT('Ctrl Pts',(0.579477555476215,4.48082217978985,9.84211436662205));
#42943=CARTESIAN_POINT('Ctrl Pts',(1.32408828624107,4.38452619018528,9.81565706993759));
#42944=CARTESIAN_POINT('Ctrl Pts',(2.04417685114126,4.09861204597845,9.78919977325312));
#42945=CARTESIAN_POINT('Ctrl Pts',(2.65203725991646,3.65790377350364,9.76274247656865));
#42946=CARTESIAN_POINT('Ctrl Pts',(3.25989766869166,3.21719550102883,9.73628517988418));
#42947=CARTESIAN_POINT('Ctrl Pts',(3.75552992134187,2.62169310028604,9.70982788319971));
#42948=CARTESIAN_POINT('Ctrl Pts',(4.07856655802598,1.94392810462463,9.68337058651525));
#42949=CARTESIAN_POINT('Ctrl Pts',(4.36666460048778,1.33946797123696,9.65977482517416));
#42950=CARTESIAN_POINT('Ctrl Pts',(4.51748278690866,0.669577455247932,9.63617906383307));
#42951=CARTESIAN_POINT('Ctrl Pts',(4.51802315729813,-7.77880120685776E-5,
9.61258330249199));
#42952=CARTESIAN_POINT('Origin',(0.,0.,20.5));
#42953=CARTESIAN_POINT('',(4.51736326149566,6.46810088806768E-6,8.61258330249198));
#42954=CARTESIAN_POINT('',(4.51813428255233,-1.20076389504314E-5,8.88741669750808));
#42955=CARTESIAN_POINT('',(4.51775,5.53264807684796E-16,20.5));
#42956=CARTESIAN_POINT('Ctrl Pts',(4.51813428255233,-1.20076389504314E-5,
8.88741669750808));
#42957=CARTESIAN_POINT('Ctrl Pts',(4.51802118875718,0.73947229319191,8.91347479471178));
#42958=CARTESIAN_POINT('Ctrl Pts',(4.3327730937107,1.47901118956561,8.93953289191547));
#42959=CARTESIAN_POINT('Ctrl Pts',(3.9839812468855,2.13106899669204,8.96559098911917));
#42960=CARTESIAN_POINT('Ctrl Pts',(3.62984605042663,2.79311606496825,8.99204828580364));
#42961=CARTESIAN_POINT('Ctrl Pts',(3.10711787221281,3.36498116344761,9.01850558248812));
#42962=CARTESIAN_POINT('Ctrl Pts',(2.47946442583089,3.77701175603631,9.04496287917258));
#42963=CARTESIAN_POINT('Ctrl Pts',(1.85181097944898,4.189042348625,9.07142017585705));
#42964=CARTESIAN_POINT('Ctrl Pts',(1.11923226489897,4.44123843532303,9.09787747254152));
#42965=CARTESIAN_POINT('Ctrl Pts',(0.370955558845314,4.50288281188386,9.12433476922598));
#42966=CARTESIAN_POINT('Ctrl Pts',(-0.377321147208358,4.5645271884447,9.15079206591045));
#42967=CARTESIAN_POINT('Ctrl Pts',(-1.14129584476571,4.43561985486832,9.17724936259492));
#42968=CARTESIAN_POINT('Ctrl Pts',(-1.82791726117885,4.13186158171856,9.20370665927939));
#42969=CARTESIAN_POINT('Ctrl Pts',(-2.51453867759199,3.82810330856881,9.23016395596386));
#42970=CARTESIAN_POINT('Ctrl Pts',(-3.12380681286095,3.34949409584567,9.25662125264832));
#42971=CARTESIAN_POINT('Ctrl Pts',(-3.58151348240605,2.75432801596707,9.28307854933279));
#42972=CARTESIAN_POINT('Ctrl Pts',(-4.03922015195113,2.15916193608848,9.30953584601726));
#42973=CARTESIAN_POINT('Ctrl Pts',(-4.34536535577235,1.44743898905445,9.33599314270173));
#42974=CARTESIAN_POINT('Ctrl Pts',(-4.46266094686473,0.705846242127692,
9.3624504393862));
#42975=CARTESIAN_POINT('Ctrl Pts',(-4.57995653795712,-0.0357465047990668,
9.38890773607066));
#42976=CARTESIAN_POINT('Ctrl Pts',(-4.50840251632067,-0.807209051618545,
9.41536503275513));
#42977=CARTESIAN_POINT('Ctrl Pts',(-4.25671408259964,-1.51457811392983,
9.4418223294396));
#42978=CARTESIAN_POINT('Ctrl Pts',(-4.00502564887861,-2.22194717624114,
9.46827962612407));
#42979=CARTESIAN_POINT('Ctrl Pts',(-3.57320280307299,-2.86522275404424,
9.49473692280854));
#42980=CARTESIAN_POINT('Ctrl Pts',(-3.01384108989007,-3.36605459389589,
9.521194219493));
#42981=CARTESIAN_POINT('Ctrl Pts',(-2.45447937670717,-3.86688643374753,
9.54765151617747));
#42982=CARTESIAN_POINT('Ctrl Pts',(-1.76757879614698,-4.22527453564772,
9.57410881286193));
#42983=CARTESIAN_POINT('Ctrl Pts',(-1.03680307870741,-4.39756762542433,
9.6005661095464));
#42984=CARTESIAN_POINT('Ctrl Pts',(-0.306027361267855,-4.56986071520094,
9.62702340623087));
#42985=CARTESIAN_POINT('Ctrl Pts',(0.468623493051109,-4.55605879285398,
9.65348070291534));
#42986=CARTESIAN_POINT('Ctrl Pts',(1.19279786752367,-4.35784291725027,9.67993799959981));
#42987=CARTESIAN_POINT('Ctrl Pts',(1.91697224199627,-4.15962704164656,9.70639529628428));
#42988=CARTESIAN_POINT('Ctrl Pts',(2.59067013662248,-3.7769972127861,9.73285259296875));
#42989=CARTESIAN_POINT('Ctrl Pts',(3.13183589343935,-3.25655732035571,9.75930988965321));
#42990=CARTESIAN_POINT('Ctrl Pts',(3.67300165025619,-2.73611742792533,9.78576718633768));
#42991=CARTESIAN_POINT('Ctrl Pts',(4.08163526926369,-2.07786747192505,9.81222448302215));
#42992=CARTESIAN_POINT('Ctrl Pts',(4.30796562791432,-1.3619815684899,9.83868177970662));
#42993=CARTESIAN_POINT('Ctrl Pts',(4.44693411433176,-0.922422416809593,
9.8549267523071));
#42994=CARTESIAN_POINT('Ctrl Pts',(4.51717337249904,-0.461134228693464,
9.87117172490759));
#42995=CARTESIAN_POINT('Ctrl Pts',(4.5174420818448,7.39595355181285E-5,
9.88741669750808));
#42996=CARTESIAN_POINT('Ctrl Pts',(4.51802315729813,-7.77880120685776E-5,
9.61258330249199));
#42997=CARTESIAN_POINT('Ctrl Pts',(4.51808868978702,-0.081289075021137,
9.60972176714861));
#42998=CARTESIAN_POINT('Ctrl Pts',(4.51594405515544,-0.162496901825208,
9.60686023180522));
#42999=CARTESIAN_POINT('Ctrl Pts',(4.51156607035433,-0.243584147729178,
9.60399869646184));
#43000=CARTESIAN_POINT('Ctrl Pts',(4.47108792528055,-0.993303813841435,
9.57754139977738));
#43001=CARTESIAN_POINT('Ctrl Pts',(4.23969061441499,-1.73271555548592,9.5510841030929));
#43002=CARTESIAN_POINT('Ctrl Pts',(3.84555807412645,-2.37175984086041,9.52462680640843));
#43003=CARTESIAN_POINT('Ctrl Pts',(3.45142553383792,-3.0108041262349,9.49816950972396));
#43004=CARTESIAN_POINT('Ctrl Pts',(2.8945577641264,-3.54948095533939,9.47171221303951));
#43005=CARTESIAN_POINT('Ctrl Pts',(2.24278064303981,-3.92218008655942,9.44525491635504));
#43006=CARTESIAN_POINT('Ctrl Pts',(1.59100352195321,-4.29487921777947,9.41879761967057));
#43007=CARTESIAN_POINT('Ctrl Pts',(0.844317049491529,-4.50160065111505,
9.3923403229861));
#43008=CARTESIAN_POINT('Ctrl Pts',(0.0936668116193721,-4.51716594477095,
9.36588302630163));
#43009=CARTESIAN_POINT('Ctrl Pts',(-0.656983426252764,-4.53273123842686,
9.33942572961716));
#43010=CARTESIAN_POINT('Ctrl Pts',(-1.41159742953537,-4.3571403924031,9.3129684329327));
#43011=CARTESIAN_POINT('Ctrl Pts',(-2.07826404778352,-4.01178017741349,
9.28651113624823));
#43012=CARTESIAN_POINT('Ctrl Pts',(-2.74493066603167,-3.66641996242389,
9.26005383956376));
#43013=CARTESIAN_POINT('Ctrl Pts',(-3.32364989924536,-3.15129037846845,
9.23359654287929));
#43014=CARTESIAN_POINT('Ctrl Pts',(-3.7439343853058,-2.52913363876293,9.20713924619482));
#43015=CARTESIAN_POINT('Ctrl Pts',(-4.16421887136626,-1.9069768990574,9.18068194951035));
#43016=CARTESIAN_POINT('Ctrl Pts',(-4.42606861027347,-1.1777930036018,9.15422465282589));
#43017=CARTESIAN_POINT('Ctrl Pts',(-4.49759059362582,-0.430395743852028,
9.12776735614142));
#43018=CARTESIAN_POINT('Ctrl Pts',(-4.56911257697816,0.317001515897712,
9.10131005945695));
#43019=CARTESIAN_POINT('Ctrl Pts',(-4.45030680477565,1.08261213994165,9.07485276277248));
#43020=CARTESIAN_POINT('Ctrl Pts',(-4.15564368858649,1.77318560159636,9.04839546608801));
#43021=CARTESIAN_POINT('Ctrl Pts',(-3.86098057239734,2.46375906325108,9.02193816940354));
#43022=CARTESIAN_POINT('Ctrl Pts',(-3.39046011222153,3.0792953625166,8.99548087271908));
#43023=CARTESIAN_POINT('Ctrl Pts',(-2.8013911793688,3.54482285937563,8.96902357603462));
#43024=CARTESIAN_POINT('Ctrl Pts',(-2.21232224651606,4.01035035623468,8.94256627935015));
#43025=CARTESIAN_POINT('Ctrl Pts',(-1.50470484098639,4.32586905068723,8.91610898266568));
#43026=CARTESIAN_POINT('Ctrl Pts',(-0.76472597963103,4.45294911494335,8.88965168598121));
#43027=CARTESIAN_POINT('Ctrl Pts',(-0.0247471182756658,4.58002917919947,
8.86319438929674));
#43028=CARTESIAN_POINT('Ctrl Pts',(0.747593198905389,4.51867061325916,8.83673709261227));
#43029=CARTESIAN_POINT('Ctrl Pts',(1.45822477605263,4.27634682254651,8.8102797959278));
#43030=CARTESIAN_POINT('Ctrl Pts',(2.16885635319985,4.03402303183387,8.78382249924334));
#43031=CARTESIAN_POINT('Ctrl Pts',(2.81777919031325,3.6107340163489,8.75736520255887));
#43032=CARTESIAN_POINT('Ctrl Pts',(3.3259552040156,3.0580359097105,8.7309079058744));
#43033=CARTESIAN_POINT('Ctrl Pts',(3.83413121771795,2.5053378030721,8.70445060918993));
#43034=CARTESIAN_POINT('Ctrl Pts',(4.20156040800925,1.82323060528026,8.67799331250546));
#43035=CARTESIAN_POINT('Ctrl Pts',(4.38349030615737,1.0947942181167,8.65153601582099));
#43036=CARTESIAN_POINT('Ctrl Pts',(4.47277460017851,0.737305266442263,8.63855177804465));
#43037=CARTESIAN_POINT('Ctrl Pts',(4.51738186963902,0.368658049377594,8.62556754026832));
#43038=CARTESIAN_POINT('Ctrl Pts',(4.51736350124836,6.46409108656654E-6,
8.61258330249198));
#43039=CARTESIAN_POINT('Origin',(0.,0.,20.5));
#43040=CARTESIAN_POINT('',(4.51805554098247,6.65521552928316E-5,7.61258330249197));
#43041=CARTESIAN_POINT('',(4.51740628246061,-5.63430382605529E-5,7.88741669750807));
#43042=CARTESIAN_POINT('',(4.51775,5.53264807684796E-16,20.5));
#43043=CARTESIAN_POINT('Ctrl Pts',(4.51740628246061,-5.63430382605529E-5,
7.88741669750807));
#43044=CARTESIAN_POINT('Ctrl Pts',(4.51721359264065,0.438494588092411,7.90286327114702));
#43045=CARTESIAN_POINT('Ctrl Pts',(4.45380791076361,0.877100051477632,7.91830984478598));
#43046=CARTESIAN_POINT('Ctrl Pts',(4.32797411068275,1.29699720179238,7.93375641842493));
#43047=CARTESIAN_POINT('Ctrl Pts',(4.1124426757192,2.01620805997421,7.9602137151094));
#43048=CARTESIAN_POINT('Ctrl Pts',(3.71376126713352,2.68053296061069,7.98667101179386));
#43049=CARTESIAN_POINT('Ctrl Pts',(3.18048883925826,3.20905786603343,8.01312830847833));
#43050=CARTESIAN_POINT('Ctrl Pts',(2.64721641138298,3.73758277145619,8.0395856051628));
#43051=CARTESIAN_POINT('Ctrl Pts',(1.97935296421813,4.13030768166519,8.06604290184727));
#43052=CARTESIAN_POINT('Ctrl Pts',(1.25824352648304,4.33939913723789,8.09250019853174));
#43053=CARTESIAN_POINT('Ctrl Pts',(0.53713408874796,4.54849059281059,8.11895749521621));
#43054=CARTESIAN_POINT('Ctrl Pts',(-0.237221339557352,4.57394859374699,
8.14541479190067));
#43055=CARTESIAN_POINT('Ctrl Pts',(-0.970507124268639,4.41267238370822,
8.17187208858514));
#43056=CARTESIAN_POINT('Ctrl Pts',(-1.70379290897991,4.25139617366945,8.19832938526961));
#43057=CARTESIAN_POINT('Ctrl Pts',(-2.39600905009715,3.90338575265551,8.22478668195408));
#43058=CARTESIAN_POINT('Ctrl Pts',(-2.96284438772951,3.4110284047919,8.25124397863854));
#43059=CARTESIAN_POINT('Ctrl Pts',(-3.52967972536187,2.91867105692828,8.27770127532301));
#43060=CARTESIAN_POINT('Ctrl Pts',(-3.97113425950935,2.28196678221498,8.30415857200748));
#43061=CARTESIAN_POINT('Ctrl Pts',(-4.2334393164843,1.57846545665159,8.33061586869195));
#43062=CARTESIAN_POINT('Ctrl Pts',(-4.49574437345926,0.874964131088192,
8.35707316537641));
#43063=CARTESIAN_POINT('Ctrl Pts',(-4.57889995326168,0.104665754674698,
8.38353046206088));
#43064=CARTESIAN_POINT('Ctrl Pts',(-4.47277779830253,-0.638608182855007,
8.40998775874535));
#43065=CARTESIAN_POINT('Ctrl Pts',(-4.36665564334337,-1.38188212038471,
8.43644505542982));
#43066=CARTESIAN_POINT('Ctrl Pts',(-4.07125575362263,-2.09813161903063,
8.46290235211428));
#43067=CARTESIAN_POINT('Ctrl Pts',(-3.62255750878001,-2.70011828255337,
8.48935964879875));
#43068=CARTESIAN_POINT('Ctrl Pts',(-3.17385926393738,-3.30210494607612,
8.51581694548322));
#43069=CARTESIAN_POINT('Ctrl Pts',(-2.57186266397286,-3.78982877447569,
8.54227424216769));
#43070=CARTESIAN_POINT('Ctrl Pts',(-1.88989022851369,-4.10388554523221,
8.56873153885216));
#43071=CARTESIAN_POINT('Ctrl Pts',(-1.20791779305452,-4.41794231598872,
8.59518883553663));
#43072=CARTESIAN_POINT('Ctrl Pts',(-0.445969522100707,-4.55833202910218,
8.62164613222109));
#43073=CARTESIAN_POINT('Ctrl Pts',(0.30315012821752,-4.50795537288903,8.64810342890556));
#43074=CARTESIAN_POINT('Ctrl Pts',(1.05226977853573,-4.45757871667589,8.67456072559003));
#43075=CARTESIAN_POINT('Ctrl Pts',(1.78856080821834,-4.21643569113615,8.7010180222745));
#43076=CARTESIAN_POINT('Ctrl Pts',(2.42234378472631,-3.81389724990005,8.72747531895897));
#43077=CARTESIAN_POINT('Ctrl Pts',(3.05612676123428,-3.41135880866395,8.75393261564343));
#43078=CARTESIAN_POINT('Ctrl Pts',(3.58740168456759,-2.84742495173149,8.78038991232789));
#43079=CARTESIAN_POINT('Ctrl Pts',(3.95145985704281,-2.19078219875382,8.80684720901236));
#43080=CARTESIAN_POINT('Ctrl Pts',(4.31551802951803,-1.53413944577613,8.83330450569683));
#43081=CARTESIAN_POINT('Ctrl Pts',(4.51235945113515,-0.78478779675323,8.85976180238131));
#43082=CARTESIAN_POINT('Ctrl Pts',(4.51800905459174,-0.0339974532052447,
8.88621909906578));
#43083=CARTESIAN_POINT('Ctrl Pts',(4.51809429832594,-0.0226691939774265,
8.88661829854654));
#43084=CARTESIAN_POINT('Ctrl Pts',(4.5181360151034,-0.0113406072147017,
8.88701749802731));
#43085=CARTESIAN_POINT('Ctrl Pts',(4.51813428255233,-1.20076389504314E-5,
8.88741669750808));
#43086=CARTESIAN_POINT('Ctrl Pts',(4.51736350124836,6.46409108656654E-6,
8.61258330249198));
#43087=CARTESIAN_POINT('Ctrl Pts',(4.5173444413379,-0.382523847714403,8.59911024358385));
#43088=CARTESIAN_POINT('Ctrl Pts',(4.46927642784078,-0.765058862836159,
8.58563718467573));
#43089=CARTESIAN_POINT('Ctrl Pts',(4.37321687241043,-1.13513692172449,8.5721641257676));
#43090=CARTESIAN_POINT('Ctrl Pts',(4.18458293451042,-1.86186609786678,8.54570682908313));
#43091=CARTESIAN_POINT('Ctrl Pts',(3.81088445270546,-2.54055887361605,8.51924953239865));
#43092=CARTESIAN_POINT('Ctrl Pts',(3.29763748849563,-3.08855122001653,8.49279223571418));
#43093=CARTESIAN_POINT('Ctrl Pts',(2.78439052428581,-3.636543566417,8.46633493902971));
#43094=CARTESIAN_POINT('Ctrl Pts',(2.13159507767111,-4.05383548346868,8.43987764234525));
#43095=CARTESIAN_POINT('Ctrl Pts',(1.4187609115801,-4.28960127750468,8.41342034566079));
#43096=CARTESIAN_POINT('Ctrl Pts',(0.705926745489094,-4.52536707154067,
8.38696304897632));
#43097=CARTESIAN_POINT('Ctrl Pts',(-0.0669461400782259,-4.57960674256099,
8.36050575229184));
#43098=CARTESIAN_POINT('Ctrl Pts',(-0.805722683022316,-4.44571395866409,
8.33404845560738));
#43099=CARTESIAN_POINT('Ctrl Pts',(-1.54449922596642,-4.31182117476718,
8.30759115892291));
#43100=CARTESIAN_POINT('Ctrl Pts',(-2.24917942628729,-3.98979593595305,
8.28113386223845));
#43101=CARTESIAN_POINT('Ctrl Pts',(-2.83393401547744,-3.51886055991386,
8.25467656555398));
#43102=CARTESIAN_POINT('Ctrl Pts',(-3.41868860466758,-3.04792518387468,
8.22821926886951));
#43103=CARTESIAN_POINT('Ctrl Pts',(-3.88351758272698,-2.42807967061047,
8.20176197218504));
#43104=CARTESIAN_POINT('Ctrl Pts',(-4.17180529456878,-1.73482051763438,
8.17530467550057));
#43105=CARTESIAN_POINT('Ctrl Pts',(-4.46009300641058,-1.0415613646583,8.1488473788161));
#43106=CARTESIAN_POINT('Ctrl Pts',(-4.57183945203477,-0.274888571970355,
8.12239008213164));
#43107=CARTESIAN_POINT('Ctrl Pts',(-4.49343403803759,0.471817962780769,
8.09593278544718));
#43108=CARTESIAN_POINT('Ctrl Pts',(-4.41502862404041,1.21852449753188,8.06947548876271));
#43109=CARTESIAN_POINT('Ctrl Pts',(-4.14647135042187,1.94526477434618,8.04301819207824));
#43110=CARTESIAN_POINT('Ctrl Pts',(-3.72047219588799,2.56352263181385,8.01656089539377));
#43111=CARTESIAN_POINT('Ctrl Pts',(-3.2944730413541,3.18178048928153,7.9901035987093));
#43112=CARTESIAN_POINT('Ctrl Pts',(-2.71103200590485,3.69155592740257,7.96364630202483));
#43113=CARTESIAN_POINT('Ctrl Pts',(-2.04121156194556,4.03075886199821,7.93718900534037));
#43114=CARTESIAN_POINT('Ctrl Pts',(-1.37139111798628,4.36996179659386,7.9107317086559));
#43115=CARTESIAN_POINT('Ctrl Pts',(-0.615191265516958,4.53859222766412,
7.88427441197143));
#43116=CARTESIAN_POINT('Ctrl Pts',(0.135283690341632,4.5161111553332,7.85781711528696));
#43117=CARTESIAN_POINT('Ctrl Pts',(0.885758646200222,4.49363008300228,7.83135981860249));
#43118=CARTESIAN_POINT('Ctrl Pts',(1.63050870544808,4.28003750727018,7.80490252191802));
#43119=CARTESIAN_POINT('Ctrl Pts',(2.27882413510697,3.90134876747149,7.77844522523355));
#43120=CARTESIAN_POINT('Ctrl Pts',(2.92713956476585,3.52266002767282,7.75198792854908));
#43121=CARTESIAN_POINT('Ctrl Pts',(3.47902036483576,2.97887512380756,7.72553063186463));
#43122=CARTESIAN_POINT('Ctrl Pts',(3.8672480646519,2.33622645534278,7.69907333518016));
#43123=CARTESIAN_POINT('Ctrl Pts',(4.25547576446805,1.69357778687799,7.67261603849569));
#43124=CARTESIAN_POINT('Ctrl Pts',(4.48005036403042,0.952065353813674,7.64615874181121));
#43125=CARTESIAN_POINT('Ctrl Pts',(4.51361892565605,0.202004549842097,7.61970144512674));
#43126=CARTESIAN_POINT('Ctrl Pts',(4.51662938451667,0.134738420941428,7.61732873091515));
#43127=CARTESIAN_POINT('Ctrl Pts',(4.51810364598245,0.0674035403653694,
7.61495601670356));
#43128=CARTESIAN_POINT('Ctrl Pts',(4.51805554098247,6.65521552928316E-5,
7.61258330249197));
#43129=CARTESIAN_POINT('Origin',(0.,0.,20.5));
#43130=CARTESIAN_POINT('',(4.51756917096255,-0.000106270599391639,6.61258330249198));
#43131=CARTESIAN_POINT('',(4.5178629555887,0.000109594847417262,6.88741669750807));
#43132=CARTESIAN_POINT('',(4.51775,5.53264807684796E-16,20.5));
#43133=CARTESIAN_POINT('Ctrl Pts',(4.5178629555887,0.000109594847417262,
6.88741669750807));
#43134=CARTESIAN_POINT('Ctrl Pts',(4.51800230500779,0.137343923060939,6.89225174758228));
#43135=CARTESIAN_POINT('Ctrl Pts',(4.5118734339612,0.274565850873291,6.89708679765648));
#43136=CARTESIAN_POINT('Ctrl Pts',(4.4993855978694,0.411206621885887,6.90192184773068));
#43137=CARTESIAN_POINT('Ctrl Pts',(4.43105241013461,1.15890217051388,6.92837914441515));
#43138=CARTESIAN_POINT('Ctrl Pts',(4.17231550636749,1.88919639463632,6.95483644109962));
#43139=CARTESIAN_POINT('Ctrl Pts',(3.75468875509468,2.51314026599451,6.98129373778408));
#43140=CARTESIAN_POINT('Ctrl Pts',(3.33706200382187,3.13708413735269,7.00775103446855));
#43141=CARTESIAN_POINT('Ctrl Pts',(2.76054540504339,3.6546776559466,7.03420833115302));
#43142=CARTESIAN_POINT('Ctrl Pts',(2.09535804244149,4.00287850404845,7.06066562783749));
#43143=CARTESIAN_POINT('Ctrl Pts',(1.4301706798396,4.35107935215029,7.08712292452196));
#43144=CARTESIAN_POINT('Ctrl Pts',(0.676312553414283,4.52988752976006,7.11358022120642));
#43145=CARTESIAN_POINT('Ctrl Pts',(-0.074397251354124,4.51752439873747,
7.14003751789089));
#43146=CARTESIAN_POINT('Ctrl Pts',(-0.82510705612252,4.50516126771487,7.16649481457536));
#43147=CARTESIAN_POINT('Ctrl Pts',(-1.57266853923404,4.30162682805993,7.19295211125983));
#43148=CARTESIAN_POINT('Ctrl Pts',(-2.22602953939534,3.93171134926469,7.2194094079443));
#43149=CARTESIAN_POINT('Ctrl Pts',(-2.87939053955664,3.56179587046945,7.24586670462877));
#43150=CARTESIAN_POINT('Ctrl Pts',(-3.43855105676772,3.0254993525339,7.27232400131323));
#43151=CARTESIAN_POINT('Ctrl Pts',(-3.83540595887268,2.38814211780651,7.2987812979977));
#43152=CARTESIAN_POINT('Ctrl Pts',(-4.23226086097764,1.7507848830791,7.32523859468216));
#43153=CARTESIAN_POINT('Ctrl Pts',(-4.46681014797648,1.01236693155982,7.35169589136664));
#43154=CARTESIAN_POINT('Ctrl Pts',(-4.51048597629575,0.26282675251353,7.37815318805111));
#43155=CARTESIAN_POINT('Ctrl Pts',(-4.55416180461501,-0.486713426532748,
7.40461048473557));
#43156=CARTESIAN_POINT('Ctrl Pts',(-4.40696417425471,-1.24737583310602,
7.43106778142003));
#43157=CARTESIAN_POINT('Ctrl Pts',(-4.08682159368453,-1.92651262793454,
7.4575250781045));
#43158=CARTESIAN_POINT('Ctrl Pts',(-3.76667901311434,-2.60564942276306,
7.48398237478897));
#43159=CARTESIAN_POINT('Ctrl Pts',(-3.27359148233425,-3.20326060584682,
7.51043967147344));
#43160=CARTESIAN_POINT('Ctrl Pts',(-2.66761651687792,-3.64655779648116,
7.53689696815791));
#43161=CARTESIAN_POINT('Ctrl Pts',(-2.06164155142159,-4.0898549871155,7.56335426484238));
#43162=CARTESIAN_POINT('Ctrl Pts',(-1.342779151289,-4.37883818530042,7.58981156152685));
#43163=CARTESIAN_POINT('Ctrl Pts',(-0.59858596122885,-4.47830955732374,
7.61626885821132));
#43164=CARTESIAN_POINT('Ctrl Pts',(0.145607228831289,-4.57778092934705,
7.64272615489578));
#43165=CARTESIAN_POINT('Ctrl Pts',(0.915131208818995,-4.48774047520876,
7.66918345158024));
#43166=CARTESIAN_POINT('Ctrl Pts',(1.61625880962798,-4.21915502257233,7.69564074826471));
#43167=CARTESIAN_POINT('Ctrl Pts',(2.31738641043699,-3.95056956993589,7.72209804494918));
#43168=CARTESIAN_POINT('Ctrl Pts',(2.95011763206728,-3.5034391188013,7.74855534163365));
#43169=CARTESIAN_POINT('Ctrl Pts',(3.43738651198769,-2.93222366326352,7.77501263831812));
#43170=CARTESIAN_POINT('Ctrl Pts',(3.92465539190809,-2.36100820772573,7.80146993500259));
#43171=CARTESIAN_POINT('Ctrl Pts',(4.2664619301186,-1.66570774778476,7.82792723168706));
#43172=CARTESIAN_POINT('Ctrl Pts',(4.42117446855315,-0.931009109950678,
7.85438452837153));
#43173=CARTESIAN_POINT('Ctrl Pts',(4.4855611265208,-0.625249858747316,7.86539525141704));
#43174=CARTESIAN_POINT('Ctrl Pts',(4.51754363682092,-0.312666955391513,
7.87640597446256));
#43175=CARTESIAN_POINT('Ctrl Pts',(4.51740628246061,-5.63430382605529E-5,
7.88741669750807));
#43176=CARTESIAN_POINT('Ctrl Pts',(4.51805554098247,6.65521552928316E-5,
7.61258330249197));
#43177=CARTESIAN_POINT('Ctrl Pts',(4.51756724414766,-0.683447390694716,
7.58849872001909));
#43178=CARTESIAN_POINT('Ctrl Pts',(4.36022097756292,-1.36717849491845,7.56441413754622));
#43179=CARTESIAN_POINT('Ctrl Pts',(4.06048220709641,-1.98142521687064,7.54032955507335));
#43180=CARTESIAN_POINT('Ctrl Pts',(3.73121440322227,-2.65618500473295,7.51387225838888));
#43181=CARTESIAN_POINT('Ctrl Pts',(3.23011627178511,-3.24709540557874,7.48741496170441));
#43182=CARTESIAN_POINT('Ctrl Pts',(2.61822101061302,-3.68218418656399,7.46095766501995));
#43183=CARTESIAN_POINT('Ctrl Pts',(2.00632574944092,-4.11727296754925,7.43450036833548));
#43184=CARTESIAN_POINT('Ctrl Pts',(1.28363335853389,-4.39654012867397,7.40804307165101));
#43185=CARTESIAN_POINT('Ctrl Pts',(0.538166971278164,-4.48597123878683,
7.38158577496654));
#43186=CARTESIAN_POINT('Ctrl Pts',(-0.207299415977548,-4.57540234889969,
7.35512847828207));
#43187=CARTESIAN_POINT('Ctrl Pts',(-0.975539799581951,-4.47499740800071,
7.3286711815976));
#43188=CARTESIAN_POINT('Ctrl Pts',(-1.67298335104765,-4.1969856267701,7.30221388491313));
#43189=CARTESIAN_POINT('Ctrl Pts',(-2.37042690251334,-3.91897384553948,
7.27575658822867));
#43190=CARTESIAN_POINT('Ctrl Pts',(-2.99707362184033,-3.46335522397723,
7.2492992915442));
#43191=CARTESIAN_POINT('Ctrl Pts',(-3.47659863214408,-2.88562360594227,
7.22284199485973));
#43192=CARTESIAN_POINT('Ctrl Pts',(-3.95612364244783,-2.30789198790732,
7.19638469817527));
#43193=CARTESIAN_POINT('Ctrl Pts',(-4.28852694372834,-1.60804737339967,
7.1699274014908));
#43194=CARTESIAN_POINT('Ctrl Pts',(-4.43332218177076,-0.871330061926449,
7.14347010480633));
#43195=CARTESIAN_POINT('Ctrl Pts',(-4.57811741981318,-0.134612750453221,
7.11701280812186));
#43196=CARTESIAN_POINT('Ctrl Pts',(-4.53530459461751,0.63897725798557,7.09055551143739));
#43197=CARTESIAN_POINT('Ctrl Pts',(-4.31009826091029,1.3552175565183,7.06409821475293));
#43198=CARTESIAN_POINT('Ctrl Pts',(-4.08489192720307,2.07145785505103,7.03764091806846));
#43199=CARTESIAN_POINT('Ctrl Pts',(-3.67729208498431,2.7303484436777,7.01118362138399));
#43200=CARTESIAN_POINT('Ctrl Pts',(-3.13694394393276,3.25163717791837,6.98472632469952));
#43201=CARTESIAN_POINT('Ctrl Pts',(-2.59659580288121,3.77292591215904,6.95826902801505));
#43202=CARTESIAN_POINT('Ctrl Pts',(-1.92349936299689,4.15661279201372,6.93181173133059));
#43203=CARTESIAN_POINT('Ctrl Pts',(-1.19963702572085,4.35596518015434,6.90535443464612));
#43204=CARTESIAN_POINT('Ctrl Pts',(-0.475774688444814,4.55531756829496,
6.87889713796165));
#43205=CARTESIAN_POINT('Ctrl Pts',(0.298853546222961,4.57033546472154,6.85243984127718));
#43206=CARTESIAN_POINT('Ctrl Pts',(1.02989881660515,4.39918970627009,6.82598254459271));
#43207=CARTESIAN_POINT('Ctrl Pts',(1.76094408698735,4.22804394781863,6.79952524790824));
#43208=CARTESIAN_POINT('Ctrl Pts',(2.44840639308396,3.87073453448917,6.77306795122378));
#43209=CARTESIAN_POINT('Ctrl Pts',(3.00855358684847,3.37078135737971,6.74661065453931));
#43210=CARTESIAN_POINT('Ctrl Pts',(3.56870078061298,2.87082818027025,6.72015335785485));
#43211=CARTESIAN_POINT('Ctrl Pts',(4.00153286204536,2.22823123938082,6.69369606117038));
#43212=CARTESIAN_POINT('Ctrl Pts',(4.25433136265593,1.52125813092963,6.66723876448591));
#43213=CARTESIAN_POINT('Ctrl Pts',(4.42840834170919,1.03443663992461,6.6490202771546));
#43214=CARTESIAN_POINT('Ctrl Pts',(4.51711887209743,0.517089928133967,6.63080178982329));
#43215=CARTESIAN_POINT('Ctrl Pts',(4.51756917096255,-0.000106270599391639,
6.61258330249198));
#43216=CARTESIAN_POINT('Origin',(0.,0.,20.5));
#43217=CARTESIAN_POINT('',(4.51761916309611,0.000112359330087797,5.61258330249198));
#43218=CARTESIAN_POINT('',(4.51777856404949,-0.00011613542669066,5.88741669750807));
#43219=CARTESIAN_POINT('',(4.51775,5.53264807684796E-16,20.5));
#43220=CARTESIAN_POINT('Ctrl Pts',(4.51777856404949,-0.00011613542669066,
5.88741669750807));
#43221=CARTESIAN_POINT('Ctrl Pts',(4.51717292408202,0.586903980160037,5.90809752070199));
#43222=CARTESIAN_POINT('Ctrl Pts',(4.40219918284471,1.17415437942607,5.92877834389592));
#43223=CARTESIAN_POINT('Ctrl Pts',(4.17916749942524,1.71700921836349,5.94945916708984));
#43224=CARTESIAN_POINT('Ctrl Pts',(3.89383962040738,2.41149180233464,5.97591646377431));
#43225=CARTESIAN_POINT('Ctrl Pts',(3.43165892348727,3.03331448007484,6.00237376045877));
#43226=CARTESIAN_POINT('Ctrl Pts',(2.84891850603996,3.50673993762589,6.02883105714324));
#43227=CARTESIAN_POINT('Ctrl Pts',(2.26617808859264,3.98016539517695,6.05528835382771));
#43228=CARTESIAN_POINT('Ctrl Pts',(1.56287795061812,4.30519363253886,6.08174565051218));
#43229=CARTESIAN_POINT('Ctrl Pts',(0.82467927055748,4.44223657011985,6.10820294719664));
#43230=CARTESIAN_POINT('Ctrl Pts',(0.086480590496836,4.57927950770083,6.13466024388111));
#43231=CARTESIAN_POINT('Ctrl Pts',(-0.686616631649936,4.5283371455009,6.16111754056558));
#43232=CARTESIAN_POINT('Ctrl Pts',(-1.4004500098362,4.29561420685648,6.18757483725005));
#43233=CARTESIAN_POINT('Ctrl Pts',(-2.11428338802246,4.06289126821206,6.21403213393451));
#43234=CARTESIAN_POINT('Ctrl Pts',(-2.76885292224821,3.64838775312316,6.24048943061899));
#43235=CARTESIAN_POINT('Ctrl Pts',(-3.28443276767729,3.10258973098363,6.26694672730345));
#43236=CARTESIAN_POINT('Ctrl Pts',(-3.80001261310638,2.5567917088441,6.29340402398792));
#43237=CARTESIAN_POINT('Ctrl Pts',(-4.1766027697388,1.87969917965394,6.31986132067238));
#43238=CARTESIAN_POINT('Ctrl Pts',(-4.36833497328082,1.15378126410905,6.34631861735685));
#43239=CARTESIAN_POINT('Ctrl Pts',(-4.56006717682283,0.427863348564182,
6.37277591404132));
#43240=CARTESIAN_POINT('Ctrl Pts',(-4.56694142727444,-0.346879953335408,
6.39923321072579));
#43241=CARTESIAN_POINT('Ctrl Pts',(-4.38812044853859,-1.07608576485095,
6.42569050741026));
#43242=CARTESIAN_POINT('Ctrl Pts',(-4.20929946980274,-1.80529157636651,
6.45214780409473));
#43243=CARTESIAN_POINT('Ctrl Pts',(-3.84478326187941,-2.48895989749803,
6.4786051007792));
#43244=CARTESIAN_POINT('Ctrl Pts',(-3.33896949547221,-3.04382068336875,
6.50506239746367));
#43245=CARTESIAN_POINT('Ctrl Pts',(-2.83315572906502,-3.59868146923946,
6.53151969414813));
#43246=CARTESIAN_POINT('Ctrl Pts',(-2.18604440417397,-4.02473471984939,
6.55797699083259));
#43247=CARTESIAN_POINT('Ctrl Pts',(-1.47645296399246,-4.27008762080069,
6.58443428751706));
#43248=CARTESIAN_POINT('Ctrl Pts',(-0.766861523810935,-4.51544052175199,
6.61089158420153));
#43249=CARTESIAN_POINT('Ctrl Pts',(0.00521003166104095,-4.58009307304465,
6.637348880886));
#43250=CARTESIAN_POINT('Ctrl Pts',(0.745724241442684,-4.45617066548422,
6.66380617757047));
#43251=CARTESIAN_POINT('Ctrl Pts',(1.48623845122433,-4.3322482579238,6.69026347425494));
#43252=CARTESIAN_POINT('Ctrl Pts',(2.19519531531564,-4.01975089151029,6.7167207709394));
#43253=CARTESIAN_POINT('Ctrl Pts',(2.78624467229499,-3.55674039962227,6.74317806762387));
#43254=CARTESIAN_POINT('Ctrl Pts',(3.37729402927435,-3.09372990773424,6.76963536430834));
#43255=CARTESIAN_POINT('Ctrl Pts',(3.85043587914176,-2.4802062903717,6.79609266099281));
#43256=CARTESIAN_POINT('Ctrl Pts',(4.14804206822422,-1.79089604512366,6.82254995767728));
#43257=CARTESIAN_POINT('Ctrl Pts',(4.39126096128897,-1.22755670280584,6.84417220428754));
#43258=CARTESIAN_POINT('Ctrl Pts',(4.51723978779142,-0.613599558623174,
6.86579445089781));
#43259=CARTESIAN_POINT('Ctrl Pts',(4.5178629555887,0.000109594847417262,
6.88741669750807));
#43260=CARTESIAN_POINT('Ctrl Pts',(4.51756917096255,-0.000106270599391639,
6.61258330249198));
#43261=CARTESIAN_POINT('Ctrl Pts',(4.51777280622788,-0.233994013420898,
6.60434449313882));
#43262=CARTESIAN_POINT('Ctrl Pts',(4.49992676845961,-0.467850975545092,
6.59610568378566));
#43263=CARTESIAN_POINT('Ctrl Pts',(4.46376343532316,-0.698840208967197,
6.5878668744325));
#43264=CARTESIAN_POINT('Ctrl Pts',(4.34763208759105,-1.44061616439985,6.56140957774804));
#43265=CARTESIAN_POINT('Ctrl Pts',(4.04260447233807,-2.15281879925221,6.53495228106357));
#43266=CARTESIAN_POINT('Ctrl Pts',(3.58583261551844,-2.74870262081615,6.5084949843791));
#43267=CARTESIAN_POINT('Ctrl Pts',(3.1290607586988,-3.3445864423801,6.48203768769463));
#43268=CARTESIAN_POINT('Ctrl Pts',(2.52054466031253,-3.82415145065562,6.45558039101016));
#43269=CARTESIAN_POINT('Ctrl Pts',(1.83440090767928,-4.12898715838434,6.42912309432569));
#43270=CARTESIAN_POINT('Ctrl Pts',(1.14825715504604,-4.43382286611306,6.40266579764122));
#43271=CARTESIAN_POINT('Ctrl Pts',(0.384485748165844,-4.56392927329498,
6.37620850095676));
#43272=CARTESIAN_POINT('Ctrl Pts',(-0.363886800892981,-4.50345956352816,
6.34975120427229));
#43273=CARTESIAN_POINT('Ctrl Pts',(-1.11225934995183,-4.44298985376135,
6.32329390758782));
#43274=CARTESIAN_POINT('Ctrl Pts',(-1.84523304118933,-4.19194402704577,
6.29683661090335));
#43275=CARTESIAN_POINT('Ctrl Pts',(-2.47353249021757,-3.78089918723516,
6.27037931421889));
#43276=CARTESIAN_POINT('Ctrl Pts',(-3.10183193924579,-3.36985434742456,
6.24392201753442));
#43277=CARTESIAN_POINT('Ctrl Pts',(-3.62545714606476,-2.79881049451895,
6.21746472084996));
#43278=CARTESIAN_POINT('Ctrl Pts',(-3.98063113999636,-2.13732013781012,
6.19100742416549));
#43279=CARTESIAN_POINT('Ctrl Pts',(-4.33580513392796,-1.47582978110128,
6.16455012748102));
#43280=CARTESIAN_POINT('Ctrl Pts',(-4.52252791497214,-0.723892920589236,
6.13809283079655));
#43281=CARTESIAN_POINT('Ctrl Pts',(-4.51805685504966,0.0269053663076428,
6.11163553411208));
#43282=CARTESIAN_POINT('Ctrl Pts',(-4.51358579512718,0.777703653204501,
6.08517823742761));
#43283=CARTESIAN_POINT('Ctrl Pts',(-4.31792089423804,1.52736336648619,6.05872094074314));
#43284=CARTESIAN_POINT('Ctrl Pts',(-3.95489392076209,2.18457678274683,6.03226364405868));
#43285=CARTESIAN_POINT('Ctrl Pts',(-3.59186694728612,2.84179019900748,6.00580634737421));
#43286=CARTESIAN_POINT('Ctrl Pts',(-3.06147790122333,3.40655731824708,5.97934905068974));
#43287=CARTESIAN_POINT('Ctrl Pts',(-2.42832758138604,3.81009013038763,5.95289175400527));
#43288=CARTESIAN_POINT('Ctrl Pts',(-1.79517726154877,4.21362294252816,5.9264344573208));
#43289=CARTESIAN_POINT('Ctrl Pts',(-1.05926566793702,4.45592144756967,5.89997716063634));
#43290=CARTESIAN_POINT('Ctrl Pts',(-0.310226018196338,4.50747395575742,
5.87351986395187));
#43291=CARTESIAN_POINT('Ctrl Pts',(0.438813631544363,4.55902646394516,5.8470625672674));
#43292=CARTESIAN_POINT('Ctrl Pts',(1.20098133741399,4.41983297527914,5.82060527058293));
#43293=CARTESIAN_POINT('Ctrl Pts',(1.88344591635241,4.10684710262907,5.79414797389846));
#43294=CARTESIAN_POINT('Ctrl Pts',(2.56591049529081,3.79386122997902,5.767690677214));
#43295=CARTESIAN_POINT('Ctrl Pts',(3.16867194729802,3.30708297334494,5.74123338052953));
#43296=CARTESIAN_POINT('Ctrl Pts',(3.61831459461448,2.70580138565218,5.71477608384506));
#43297=CARTESIAN_POINT('Ctrl Pts',(4.06795724193093,2.10451979795941,5.68831878716059));
#43298=CARTESIAN_POINT('Ctrl Pts',(4.36448108455665,1.38873487920795,5.66186149047613));
#43299=CARTESIAN_POINT('Ctrl Pts',(4.47176984663199,0.645628440320207,5.63540419379166));
#43300=CARTESIAN_POINT('Ctrl Pts',(4.50261735669319,0.431971549265432,5.6277972300251));
#43301=CARTESIAN_POINT('Ctrl Pts',(4.51782138536506,0.216056072273327,5.62019026625854));
#43302=CARTESIAN_POINT('Ctrl Pts',(4.51761916309611,0.000112359330087797,
5.61258330249198));
#43303=CARTESIAN_POINT('Origin',(0.,0.,20.5));
#43304=CARTESIAN_POINT('',(4.51801297056466,-8.08487039419617E-5,4.61258330249197));
#43305=CARTESIAN_POINT('',(4.51744953111884,7.68816669171638E-5,4.88741669750807));
#43306=CARTESIAN_POINT('',(4.51775,5.53264807684796E-16,20.5));
#43307=CARTESIAN_POINT('Ctrl Pts',(4.51744953111884,7.68816669171638E-5,
4.88741669750807));
#43308=CARTESIAN_POINT('Ctrl Pts',(4.51762304095457,0.28595126409645,4.89748599713724));
#43309=CARTESIAN_POINT('Ctrl Pts',(4.49090928481679,0.571793625338861,4.90755529676642));
#43310=CARTESIAN_POINT('Ctrl Pts',(4.43699864797727,0.852411075740623,4.91762459639559));
#43311=CARTESIAN_POINT('Ctrl Pts',(4.2953473151299,1.58973933227679,4.94408189308006));
#43312=CARTESIAN_POINT('Ctrl Pts',(3.96593233939643,2.29099550010712,4.97053918976452));
#43313=CARTESIAN_POINT('Ctrl Pts',(3.48887610024735,2.87076735409198,4.99699648644899));
#43314=CARTESIAN_POINT('Ctrl Pts',(3.01181986109827,3.45053920807684,5.02345378313346));
#43315=CARTESIAN_POINT('Ctrl Pts',(2.38712235853358,3.90882674821622,5.04991107981793));
#43316=CARTESIAN_POINT('Ctrl Pts',(1.69087105699343,4.18981105932229,5.0763683765024));
#43317=CARTESIAN_POINT('Ctrl Pts',(0.994619755453274,4.47079537042835,5.10282567318686));
#43318=CARTESIAN_POINT('Ctrl Pts',(0.226814654937662,4.57447645250109,5.12928296987133));
#43319=CARTESIAN_POINT('Ctrl Pts',(-0.519026433064492,4.48822606449115,
5.1557402665558));
#43320=CARTESIAN_POINT('Ctrl Pts',(-1.26486752106665,4.40197567648121,5.18219756324027));
#43321=CARTESIAN_POINT('Ctrl Pts',(-1.98874459655534,4.12579381838858,5.20865485992474));
#43322=CARTESIAN_POINT('Ctrl Pts',(-2.60249023287342,3.69331913486986,5.2351121566092));
#43323=CARTESIAN_POINT('Ctrl Pts',(-3.21623586919149,3.26084445135114,5.26156945329367));
#43324=CARTESIAN_POINT('Ctrl Pts',(-3.71985006633895,2.67207694240634,5.28802674997814));
#43325=CARTESIAN_POINT('Ctrl Pts',(-4.05199317246879,1.99872783901753,5.31448404666261));
#43326=CARTESIAN_POINT('Ctrl Pts',(-4.38413627859864,1.32537873562872,5.34094134334707));
#43327=CARTESIAN_POINT('Ctrl Pts',(-4.54480829371086,0.567448037795898,
5.36739864003154));
#43328=CARTESIAN_POINT('Ctrl Pts',(-4.51443954418554,-0.182749134310455,
5.39385593671601));
#43329=CARTESIAN_POINT('Ctrl Pts',(-4.48407079466022,-0.932946306416809,
5.42031323340048));
#43330=CARTESIAN_POINT('Ctrl Pts',(-4.26266128049735,-1.6754099527967,5.44677053008495));
#43331=CARTESIAN_POINT('Ctrl Pts',(-3.87717843548113,-2.31970882302876,
5.47322782676942));
#43332=CARTESIAN_POINT('Ctrl Pts',(-3.49169559046492,-2.96400769326083,
5.49968512345388));
#43333=CARTESIAN_POINT('Ctrl Pts',(-2.94213941459537,-3.51014178734505,
5.52614242013835));
#43334=CARTESIAN_POINT('Ctrl Pts',(-2.29544524188241,-3.89159257704565,
5.55259971682282));
#43335=CARTESIAN_POINT('Ctrl Pts',(-1.64875106916946,-4.27304336674624,
5.57905701350729));
#43336=CARTESIAN_POINT('Ctrl Pts',(-0.904918899613081,-4.48981085206321,
5.60551431019175));
#43337=CARTESIAN_POINT('Ctrl Pts',(-0.154546668242997,-4.51549299318827,
5.63197160687622));
#43338=CARTESIAN_POINT('Ctrl Pts',(0.595825563127097,-4.54117513431334,
5.65842890356069));
#43339=CARTESIAN_POINT('Ctrl Pts',(1.35273785631093,-4.37577193124651,5.68488620024516));
#43340=CARTESIAN_POINT('Ctrl Pts',(2.02399913169717,-4.03942931106444,5.71134349692963));
#43341=CARTESIAN_POINT('Ctrl Pts',(2.69526040708341,-3.70308669088236,5.73780079361409));
#43342=CARTESIAN_POINT('Ctrl Pts',(3.28087066467206,-3.19580465358505,5.76425809029856));
#43343=CARTESIAN_POINT('Ctrl Pts',(3.70950322320198,-2.57936958989042,5.79071538698303));
#43344=CARTESIAN_POINT('Ctrl Pts',(4.13813578173191,-1.9629345261958,5.8171726836675));
#43345=CARTESIAN_POINT('Ctrl Pts',(4.40979064120311,-1.23734643610387,5.84362998035196));
#43346=CARTESIAN_POINT('Ctrl Pts',(4.49138054038091,-0.490981145956846,
5.87008727703643));
#43347=CARTESIAN_POINT('Ctrl Pts',(4.50919422313609,-0.328025747897277,
5.87586375052698));
#43348=CARTESIAN_POINT('Ctrl Pts',(4.51794772865112,-0.164079924696943,
5.88164022401752));
#43349=CARTESIAN_POINT('Ctrl Pts',(4.51777856404949,-0.00011613542669066,
5.88741669750807));
#43350=CARTESIAN_POINT('Ctrl Pts',(4.51761916309611,0.000112359330087797,
5.61258330249198));
#43351=CARTESIAN_POINT('Ctrl Pts',(4.51711804895781,-0.535004016325972,
5.59373296957407));
#43352=CARTESIAN_POINT('Ctrl Pts',(4.42201232003226,-1.07029377947848,5.57488263665616));
#43353=CARTESIAN_POINT('Ctrl Pts',(4.23591186210463,-1.57181816399948,5.55603230373826));
#43354=CARTESIAN_POINT('Ctrl Pts',(3.97471143397694,-2.27573037040736,5.52957500705379));
#43355=CARTESIAN_POINT('Ctrl Pts',(3.5342568961966,-2.91312682419909,5.50311771036932));
#43356=CARTESIAN_POINT('Ctrl Pts',(2.96819512400045,-3.40637334272939,5.47666041368485));
#43357=CARTESIAN_POINT('Ctrl Pts',(2.4021333518043,-3.89961986125968,5.45020311700038));
#43358=CARTESIAN_POINT('Ctrl Pts',(1.71046434519234,-4.24871644452854,5.42374582031592));
#43359=CARTESIAN_POINT('Ctrl Pts',(0.977432623678222,-4.41114351504991,
5.39728852363145));
#43360=CARTESIAN_POINT('Ctrl Pts',(0.244400902164107,-4.57357058557128,
5.37083122694698));
#43361=CARTESIAN_POINT('Ctrl Pts',(-0.529993534252169,-4.54932814334517,
5.34437393026251));
#43362=CARTESIAN_POINT('Ctrl Pts',(-1.2514303002616,-4.34136889100483,5.31791663357804));
#43363=CARTESIAN_POINT('Ctrl Pts',(-1.97286706627105,-4.1334096386645,5.29145933689358));
#43364=CARTESIAN_POINT('Ctrl Pts',(-2.64134616187366,-3.74173357620994,
5.2650020402091));
#43365=CARTESIAN_POINT('Ctrl Pts',(-3.17544757305171,-3.214046414568,5.23854474352464));
#43366=CARTESIAN_POINT('Ctrl Pts',(-3.70954898422975,-2.68635925292607,
5.21208744684017));
#43367=CARTESIAN_POINT('Ctrl Pts',(-4.10927271098324,-2.02266099209677,
5.1856301501557));
#43368=CARTESIAN_POINT('Ctrl Pts',(-4.32593284578035,-1.3037893457135,5.15917285347124));
#43369=CARTESIAN_POINT('Ctrl Pts',(-4.54259298057747,-0.584917699330228,
5.13271555678677));
#43370=CARTESIAN_POINT('Ctrl Pts',(-4.57618952341819,0.189127332607011,
5.1062582601023));
#43371=CARTESIAN_POINT('Ctrl Pts',(-4.42263045256687,0.924067921868061,
5.07980096341783));
#43372=CARTESIAN_POINT('Ctrl Pts',(-4.26907138171554,1.65900851112912,5.05334366673336));
#43373=CARTESIAN_POINT('Ctrl Pts',(-3.92835669717217,2.35484465771397,5.0268863700489));
#43374=CARTESIAN_POINT('Ctrl Pts',(-3.44198507043455,2.92682428907221,5.00042907336443));
#43375=CARTESIAN_POINT('Ctrl Pts',(-2.95561344369694,3.49880392043043,4.97397177667996));
#43376=CARTESIAN_POINT('Ctrl Pts',(-2.3235848747651,3.94692703656203,4.9475144799955));
#43377=CARTESIAN_POINT('Ctrl Pts',(-1.62287974384915,4.21661273787403,4.92105718331103));
#43378=CARTESIAN_POINT('Ctrl Pts',(-0.922174612933183,4.48629843918604,
4.89459988662656));
#43379=CARTESIAN_POINT('Ctrl Pts',(-0.152792920033106,4.57754672567842,
4.86814258994209));
#43380=CARTESIAN_POINT('Ctrl Pts',(0.591555496154586,4.47924365704375,4.84168529325762));
#43381=CARTESIAN_POINT('Ctrl Pts',(1.33590391234227,4.38094058840908,4.81522799657315));
#43382=CARTESIAN_POINT('Ctrl Pts',(2.05521905181757,4.09308616464735,4.78877069988869));
#43383=CARTESIAN_POINT('Ctrl Pts',(2.66188912668092,3.65074073599527,4.76231340320422));
#43384=CARTESIAN_POINT('Ctrl Pts',(3.26855920154427,3.20839530734318,4.73585610651975));
#43385=CARTESIAN_POINT('Ctrl Pts',(3.76258421179568,2.61155887380074,4.70939880983528));
#43386=CARTESIAN_POINT('Ctrl Pts',(4.08379245793942,1.93292545243589,4.68294151315081));
#43387=CARTESIAN_POINT('Ctrl Pts',(4.36852345568096,1.33135941704992,4.65948877626453));
#43388=CARTESIAN_POINT('Ctrl Pts',(4.51746001083452,0.665519661321642,4.63603603937825));
#43389=CARTESIAN_POINT('Ctrl Pts',(4.51801297056466,-8.08487039419617E-5,
4.61258330249197));
#43390=CARTESIAN_POINT('Origin',(0.,0.,20.5));
#43391=CARTESIAN_POINT('',(4.51736370604735,1.02551535238581E-5,3.61258330249198));
#43392=CARTESIAN_POINT('',(4.51813206731963,-1.62797693238861E-5,3.88741669750807));
#43393=CARTESIAN_POINT('',(4.51775,5.53264807684796E-16,20.5));
#43394=CARTESIAN_POINT('Ctrl Pts',(4.51813206731963,-1.62797693238861E-5,
3.88741669750807));
#43395=CARTESIAN_POINT('Ctrl Pts',(4.51798177204935,0.735410282480124,3.91333177025696));
#43396=CARTESIAN_POINT('Ctrl Pts',(4.33483992986086,1.47090898249386,3.93924684300585));
#43397=CARTESIAN_POINT('Ctrl Pts',(3.98971201192936,2.12032066114161,3.96516191575474));
#43398=CARTESIAN_POINT('Ctrl Pts',(3.63736294436994,2.78332005222287,3.99161921243921));
#43399=CARTESIAN_POINT('Ctrl Pts',(3.11617838217547,3.35659231850456,4.01807650912368));
#43400=CARTESIAN_POINT('Ctrl Pts',(2.48963802820999,3.77031353241187,4.04453380580815));
#43401=CARTESIAN_POINT('Ctrl Pts',(1.86309767424454,4.18403474631916,4.07099110249262));
#43402=CARTESIAN_POINT('Ctrl Pts',(1.13120152850809,4.4382049078521,4.09744839917709));
#43403=CARTESIAN_POINT('Ctrl Pts',(0.383093731539025,4.50186637263401,4.12390569586155));
#43404=CARTESIAN_POINT('Ctrl Pts',(-0.365014065430051,4.56552783741592,
4.15036299254602));
#43405=CARTESIAN_POINT('Ctrl Pts',(-1.12933351363175,4.43868060544681,4.17682028923049));
#43406=CARTESIAN_POINT('Ctrl Pts',(-1.81677135017129,4.13677452919472,4.20327758591496));
#43407=CARTESIAN_POINT('Ctrl Pts',(-2.50420918671083,3.83486845294263,4.22973488259942));
#43408=CARTESIAN_POINT('Ctrl Pts',(-3.11476541158823,3.35790353240755,4.25619217928389));
#43409=CARTESIAN_POINT('Ctrl Pts',(-3.57407495233505,2.7639735670387,4.28264947596836));
#43410=CARTESIAN_POINT('Ctrl Pts',(-4.03338449308186,2.17004360166985,4.30910677265283));
#43411=CARTESIAN_POINT('Ctrl Pts',(-4.3414473496981,1.45914859146723,4.3355640693373));
#43412=CARTESIAN_POINT('Ctrl Pts',(-4.4607418071907,0.717874761903797,4.36202136602176));
#43413=CARTESIAN_POINT('Ctrl Pts',(-4.5800362646833,-0.0233990676596439,
4.38847866270623));
#43414=CARTESIAN_POINT('Ctrl Pts',(-4.51056232305225,-0.795051716583895,
4.4149359593907));
#43415=CARTESIAN_POINT('Ctrl Pts',(-4.26078183149923,-1.50309674624206,
4.44139325607517));
#43416=CARTESIAN_POINT('Ctrl Pts',(-4.01100133994621,-2.21114177590023,
4.46785055275963));
#43417=CARTESIAN_POINT('Ctrl Pts',(-3.58091429847122,-2.85557918629231,
4.4943078494441));
#43418=CARTESIAN_POINT('Ctrl Pts',(-3.02290483273516,-3.35791721405156,
4.52076514612857));
#43419=CARTESIAN_POINT('Ctrl Pts',(-2.4648953669991,-3.86025524181081,4.54722244281304));
#43420=CARTESIAN_POINT('Ctrl Pts',(-1.77896347700197,-4.22049388693723,
4.57367973949751));
#43421=CARTESIAN_POINT('Ctrl Pts',(-1.04865490780318,-4.39475648114178,
4.60013703618198));
#43422=CARTESIAN_POINT('Ctrl Pts',(-0.318346338604368,-4.56901907534634,
4.62659433286644));
#43423=CARTESIAN_POINT('Ctrl Pts',(0.456338909796113,-4.55730561862902,
4.65305162955091));
#43424=CARTESIAN_POINT('Ctrl Pts',(1.18104503151144,-4.36104279705434,4.67950892623538));
#43425=CARTESIAN_POINT('Ctrl Pts',(1.90575115322676,-4.16477997547966,4.70596622291985));
#43426=CARTESIAN_POINT('Ctrl Pts',(2.58047814825693,-3.78396778904763,4.73242351960431));
#43427=CARTESIAN_POINT('Ctrl Pts',(3.1230450153487,-3.26498874060892,4.75888081628878));
#43428=CARTESIAN_POINT('Ctrl Pts',(3.66561188244045,-2.74600969217023,4.78533811297325));
#43429=CARTESIAN_POINT('Ctrl Pts',(4.07601862159381,-2.08886378172488,4.81179540965772));
#43430=CARTESIAN_POINT('Ctrl Pts',(4.30427814618986,-1.37359065388121,4.83825270634219));
#43431=CARTESIAN_POINT('Ctrl Pts',(4.4456650936749,-0.930541084129997,4.85464070339748));
#43432=CARTESIAN_POINT('Ctrl Pts',(4.51716714020965,-0.465189691975021,
4.87102870045278));
#43433=CARTESIAN_POINT('Ctrl Pts',(4.51744953111884,7.68816669171638E-5,
4.88741669750807));
#43434=CARTESIAN_POINT('Ctrl Pts',(4.51801297056466,-8.08487039419617E-5,
4.61258330249197));
#43435=CARTESIAN_POINT('Ctrl Pts',(4.51808381093537,-0.0853517722542952,
4.60957874269379));
#43436=CARTESIAN_POINT('Ctrl Pts',(4.51571930609417,-0.170618769185437,
4.6065741828956));
#43437=CARTESIAN_POINT('Ctrl Pts',(4.51089298576516,-0.255746192878958,
4.60356962309741));
#43438=CARTESIAN_POINT('Ctrl Pts',(4.46839378541107,-1.00535400764169,4.57711232641294));
#43439=CARTESIAN_POINT('Ctrl Pts',(4.23500390266681,-1.74413922797991,4.55065502972848));
#43440=CARTESIAN_POINT('Ctrl Pts',(3.83914996695076,-2.38211863169309,4.52419773304401));
#43441=CARTESIAN_POINT('Ctrl Pts',(3.44329603123471,-3.02009803540626,4.49774043635954));
#43442=CARTESIAN_POINT('Ctrl Pts',(2.88497804254688,-3.55727162249439,4.47128313967507));
#43443=CARTESIAN_POINT('Ctrl Pts',(2.23219851400147,-3.92821224455693,4.4448258429906));
#43444=CARTESIAN_POINT('Ctrl Pts',(1.57941898545608,-4.29915286661947,4.41836854630613));
#43445=CARTESIAN_POINT('Ctrl Pts',(0.832177917053118,-4.50386052365641,
4.39191124962167));
#43446=CARTESIAN_POINT('Ctrl Pts',(0.0814884439290546,-4.51740204959703,
4.3654539529372));
#43447=CARTESIAN_POINT('Ctrl Pts',(-0.66920102919502,-4.53094357553764,
4.33899665625273));
#43448=CARTESIAN_POINT('Ctrl Pts',(-1.42333890704021,-4.35331897038192,
4.31253935956826));
#43449=CARTESIAN_POINT('Ctrl Pts',(-2.08907203071289,-4.00616271445513,
4.28608206288379));
#43450=CARTESIAN_POINT('Ctrl Pts',(-2.75480515438558,-3.65900645852834,
4.25962476619933));
#43451=CARTESIAN_POINT('Ctrl Pts',(-3.33213352388578,-3.14231855183048,
4.23316746951486));
#43452=CARTESIAN_POINT('Ctrl Pts',(-3.75073918275569,-2.51903100956272,
4.20671017283039));
#43453=CARTESIAN_POINT('Ctrl Pts',(-4.1693448416256,-1.89574346729495,4.18025287614593));
#43454=CARTESIAN_POINT('Ctrl Pts',(-4.42922778986523,-1.16585628945725,
4.15379557946146));
#43455=CARTESIAN_POINT('Ctrl Pts',(-4.49873457199956,-0.418268926521358,
4.12733828277699));
#43456=CARTESIAN_POINT('Ctrl Pts',(-4.56824135413388,0.329318436414523,
4.10088098609252));
#43457=CARTESIAN_POINT('Ctrl Pts',(-4.44737197016292,1.0946059844486,4.07442368940805));
#43458=CARTESIAN_POINT('Ctrl Pts',(-4.1508481772844,1.78438254119798,4.04796639272359));
#43459=CARTESIAN_POINT('Ctrl Pts',(-3.85432438440588,2.47415909794737,4.02150909603912));
#43460=CARTESIAN_POINT('Ctrl Pts',(-3.3821461826198,3.08842466341204,3.99505179935465));
#43461=CARTESIAN_POINT('Ctrl Pts',(-2.79182435432936,3.55236237154529,3.96859450267018));
#43462=CARTESIAN_POINT('Ctrl Pts',(-2.20150252603891,4.01630007967853,3.94213720598571));
#43463=CARTESIAN_POINT('Ctrl Pts',(-1.49303707124409,4.32990993048035,3.91567990930125));
#43464=CARTESIAN_POINT('Ctrl Pts',(-0.752718298258071,4.45499459120489,
3.88922261261678));
#43465=CARTESIAN_POINT('Ctrl Pts',(-0.0123995252720613,4.58007925192944,
3.86276531593231));
#43466=CARTESIAN_POINT('Ctrl Pts',(0.759772565905157,4.51663872257671,3.83630801924784));
#43467=CARTESIAN_POINT('Ctrl Pts',(1.46974826915516,4.27239998941026,3.80985072256337));
#43468=CARTESIAN_POINT('Ctrl Pts',(2.17972397240517,4.02816125624381,3.78339342587891));
#43469=CARTESIAN_POINT('Ctrl Pts',(2.82750328772796,3.60312431926363,3.75693612919444));
#43470=CARTESIAN_POINT('Ctrl Pts',(3.33418741143483,3.04905820699226,3.73047883250997));
#43471=CARTESIAN_POINT('Ctrl Pts',(3.84087153514169,2.49499209472089,3.7040215358255));
#43472=CARTESIAN_POINT('Ctrl Pts',(4.20646046723263,1.81189680715833,3.67756423914103));
#43473=CARTESIAN_POINT('Ctrl Pts',(4.38642588038764,1.08297259432681,3.65110694245657));
#43474=CARTESIAN_POINT('Ctrl Pts',(4.47377321176399,0.729184698918257,3.63826572913504));
#43475=CARTESIAN_POINT('Ctrl Pts',(4.51739308950363,0.364600853640814,3.62542451581351));
#43476=CARTESIAN_POINT('Ctrl Pts',(4.51736430815743,1.02391689833781E-5,
3.61258330249198));
#43477=CARTESIAN_POINT('Origin',(0.,0.,20.5));
#43478=CARTESIAN_POINT('',(4.51806423128285,6.30519293007281E-5,2.61258330249198));
#43479=CARTESIAN_POINT('',(4.5174009456275,-5.29814202112051E-5,2.88741669750807));
#43480=CARTESIAN_POINT('',(4.51775,5.53264807684796E-16,20.5));
#43481=CARTESIAN_POINT('Ctrl Pts',(4.5174009456275,-5.29814202112051E-5,
2.88741669750807));
#43482=CARTESIAN_POINT('Ctrl Pts',(4.5172216944486,0.434438744202657,2.90272024669221));
#43483=CARTESIAN_POINT('Ctrl Pts',(4.45500169120217,0.868980727030553,2.91802379587635));
#43484=CARTESIAN_POINT('Ctrl Pts',(4.33145501462215,1.28532451174868,2.9333273450605));
#43485=CARTESIAN_POINT('Ctrl Pts',(4.11786331525058,2.00511381699269,2.95978464174497));
#43486=CARTESIAN_POINT('Ctrl Pts',(3.72097433835707,2.67051112625836,2.98624193842943));
#43487=CARTESIAN_POINT('Ctrl Pts',(3.18912872207782,3.2004717836931,3.0126992351139));
#43488=CARTESIAN_POINT('Ctrl Pts',(2.65728310579859,3.73043244112782,3.03915653179837));
#43489=CARTESIAN_POINT('Ctrl Pts',(1.99048085013363,4.12495644673162,3.06561382848284));
#43490=CARTESIAN_POINT('Ctrl Pts',(1.26993773185205,4.33599121325399,3.0920711251673));
#43491=CARTESIAN_POINT('Ctrl Pts',(0.54939461357047,4.54702597977637,3.11852842185177));
#43492=CARTESIAN_POINT('Ctrl Pts',(-0.22488936732773,4.57457150721731,3.14498571853624));
#43493=CARTESIAN_POINT('Ctrl Pts',(-0.958607278893408,4.41527278082,3.17144301522071));
#43494=CARTESIAN_POINT('Ctrl Pts',(-1.69232519045908,4.25597405442269,3.19790031190518));
#43495=CARTESIAN_POINT('Ctrl Pts',(-2.38547703269224,3.90983107418713,3.22435760858964));
#43496=CARTESIAN_POINT('Ctrl Pts',(-2.95363767834166,3.41900367201878,3.25081490527411));
#43497=CARTESIAN_POINT('Ctrl Pts',(-3.52179832399109,2.92817626985041,3.27727220195858));
#43498=CARTESIAN_POINT('Ctrl Pts',(-3.96496777305678,2.29266444574925,3.30372949864305));
#43499=CARTESIAN_POINT('Ctrl Pts',(-4.229168477112,1.58987283655001,3.33018679532752));
#43500=CARTESIAN_POINT('Ctrl Pts',(-4.49336918116721,0.887081227350804,
3.35664409201199));
#43501=CARTESIAN_POINT('Ctrl Pts',(-4.57860114021196,0.117009833053533,
3.38310138869645));
#43502=CARTESIAN_POINT('Ctrl Pts',(-4.47448319596347,-0.62654750277845,
3.40955868538092));
#43503=CARTESIAN_POINT('Ctrl Pts',(-4.37036525171498,-1.37010483861044,
3.43601598206539));
#43504=CARTESIAN_POINT('Ctrl Pts',(-4.07689740417324,-2.08714811597715,
3.46247327874986));
#43505=CARTESIAN_POINT('Ctrl Pts',(-3.62982371237881,-2.69034225726949,
3.48893057543432));
#43506=CARTESIAN_POINT('Ctrl Pts',(-3.18275002058438,-3.29353639856183,
3.51538787211879));
#43507=CARTESIAN_POINT('Ctrl Pts',(-2.58207048453726,-3.7828814037798,3.54184516880326));
#43508=CARTESIAN_POINT('Ctrl Pts',(-1.90094720693718,-4.09877559286125,
3.56830246548773));
#43509=CARTESIAN_POINT('Ctrl Pts',(-1.2198239293371,-4.41466978194271,3.59475976217219));
#43510=CARTESIAN_POINT('Ctrl Pts',(-0.45825691018407,-4.55711315488765,
3.62121705885666));
#43511=CARTESIAN_POINT('Ctrl Pts',(0.290995830439079,-4.5087562665179,3.64767435554113));
#43512=CARTESIAN_POINT('Ctrl Pts',(1.04024857106223,-4.46039937814816,3.6741316522256));
#43513=CARTESIAN_POINT('Ctrl Pts',(1.77718703315549,-4.22124222846373,3.70058894891007));
#43514=CARTESIAN_POINT('Ctrl Pts',(2.41205292762872,-3.8204138936135,3.72704624559453));
#43515=CARTESIAN_POINT('Ctrl Pts',(3.04691882210195,-3.41958555876328,3.753503542279));
#43516=CARTESIAN_POINT('Ctrl Pts',(3.57971214895514,-2.85708603874726,3.77996083896347));
#43517=CARTESIAN_POINT('Ctrl Pts',(3.94553927063659,-2.2014271525676,3.80641813564794));
#43518=CARTESIAN_POINT('Ctrl Pts',(4.31136639231804,-1.54576826638794,3.83287543233241));
#43519=CARTESIAN_POINT('Ctrl Pts',(4.51022730882776,-0.796950014044647,
3.85933272901687));
#43520=CARTESIAN_POINT('Ctrl Pts',(4.51790098062045,-0.0461776299325883,
3.88579002570134));
#43521=CARTESIAN_POINT('Ctrl Pts',(4.51805824719871,-0.0307910709167367,
3.88633224963692));
#43522=CARTESIAN_POINT('Ctrl Pts',(4.5181352119642,-0.0154036911331415,
3.88687447357249));
#43523=CARTESIAN_POINT('Ctrl Pts',(4.51813206731963,-1.62797693238861E-5,
3.88741669750807));
#43524=CARTESIAN_POINT('Ctrl Pts',(4.51736430815743,1.02391689833781E-5,
3.61258330249198));
#43525=CARTESIAN_POINT('Ctrl Pts',(4.51733379007481,-0.386580659657543,
3.59896721912904));
#43526=CARTESIAN_POINT('Ctrl Pts',(4.46822794652789,-0.773179169265813,
3.5853511357661));
#43527=CARTESIAN_POINT('Ctrl Pts',(4.370140714067,-1.14692274519747,3.57173505240317));
#43528=CARTESIAN_POINT('Ctrl Pts',(4.17954824037228,-1.87314073378976,3.5452777557187));
#43529=CARTESIAN_POINT('Ctrl Pts',(3.80402139876375,-2.55082357287386,3.51882045903423));
#43530=CARTESIAN_POINT('Ctrl Pts',(3.28929894294204,-3.09743024266209,3.49236316234976));
#43531=CARTESIAN_POINT('Ctrl Pts',(2.77457648712035,-3.64403691245031,3.46590586566529));
#43532=CARTESIAN_POINT('Ctrl Pts',(2.12065841708548,-4.05956741294266,3.43944856898082));
#43533=CARTESIAN_POINT('Ctrl Pts',(1.40719123005614,-4.29341058905976,3.41299127229636));
#43534=CARTESIAN_POINT('Ctrl Pts',(0.693724043026795,-4.52725376517686,
3.38653397561189));
#43535=CARTESIAN_POINT('Ctrl Pts',(-0.0792922609970231,-4.5794096169187,
3.36007667892742));
#43536=CARTESIAN_POINT('Ctrl Pts',(-0.8177051517065,-4.44352561926563,3.33361938224295));
#43537=CARTESIAN_POINT('Ctrl Pts',(-1.55611804241598,-4.30764162161257,
3.30716208555848));
#43538=CARTESIAN_POINT('Ctrl Pts',(-2.2599275198111,-3.9837177745646,3.28070478887401));
#43539=CARTESIAN_POINT('Ctrl Pts',(-2.84341036847309,-3.51120764419552,
3.25424749218955));
#43540=CARTESIAN_POINT('Ctrl Pts',(-3.42689321713508,-3.03869751382645,
3.22779019550508));
#43541=CARTESIAN_POINT('Ctrl Pts',(-3.89004943706392,-2.41760110013629,
3.20133289882062));
#43542=CARTESIAN_POINT('Ctrl Pts',(-4.17646711326174,-1.72356725892568,
3.17487560213615));
#43543=CARTESIAN_POINT('Ctrl Pts',(-4.46288478945955,-1.02953341771508,
3.14841830545168));
#43544=CARTESIAN_POINT('Ctrl Pts',(-4.57256392192634,-0.262562148984027,
3.12196100876721));
#43545=CARTESIAN_POINT('Ctrl Pts',(-4.49214571371297,0.483930295567052,
3.09550371208274));
#43546=CARTESIAN_POINT('Ctrl Pts',(-4.41172750549959,1.23042274011814,3.06904641539827));
#43547=CARTESIAN_POINT('Ctrl Pts',(-4.14121195660606,1.95643636048925,3.04258911871381));
#43548=CARTESIAN_POINT('Ctrl Pts',(-3.71354756149959,2.57354350122118,3.01613182202934));
#43549=CARTESIAN_POINT('Ctrl Pts',(-3.28588316639313,3.1906506419531,2.98967452534487));
#43550=CARTESIAN_POINT('Ctrl Pts',(-2.70106992507374,3.69885130304582,2.9632172286604));
#43551=CARTESIAN_POINT('Ctrl Pts',(-2.03033744310303,4.03624720641976,2.93675993197593));
#43552=CARTESIAN_POINT('Ctrl Pts',(-1.35960496113232,4.3736431097937,2.91030263529147));
#43553=CARTESIAN_POINT('Ctrl Pts',(-0.602953238510295,4.54023425544885,
2.883845338607));
#43554=CARTESIAN_POINT('Ctrl Pts',(0.147458382357749,4.5157300262161,2.85738804192253));
#43555=CARTESIAN_POINT('Ctrl Pts',(0.897870003225787,4.49122579698336,2.83093074523806));
#43556=CARTESIAN_POINT('Ctrl Pts',(1.64204152233985,4.27562619286271,2.80447344855359));
#43557=CARTESIAN_POINT('Ctrl Pts',(2.28933367226974,3.89519100702514,2.77801615186913));
#43558=CARTESIAN_POINT('Ctrl Pts',(2.93662582219963,3.51475582118756,2.75155885518466));
#43559=CARTESIAN_POINT('Ctrl Pts',(3.48703860294536,2.96948505363305,2.72510155850019));
#43560=CARTESIAN_POINT('Ctrl Pts',(3.873532346971,2.32579208038178,2.69864426181572));
#43561=CARTESIAN_POINT('Ctrl Pts',(4.26002609099665,1.68209910713051,2.67218696513126));
#43562=CARTESIAN_POINT('Ctrl Pts',(4.48260079830222,0.939983928182504,2.64572966844679));
#43563=CARTESIAN_POINT('Ctrl Pts',(4.51414711586846,0.189835351011121,2.61927237176232));
#43564=CARTESIAN_POINT('Ctrl Pts',(4.51680568306753,0.126616549085492,2.61704268200554));
#43565=CARTESIAN_POINT('Ctrl Pts',(4.51810751267774,0.063340691696271,2.61481299224876));
#43566=CARTESIAN_POINT('Ctrl Pts',(4.51806423128285,6.30519293007281E-5,
2.61258330249198));
#43567=CARTESIAN_POINT('Origin',(0.,0.,20.5));
#43568=CARTESIAN_POINT('',(4.51755838390264,-0.00010457874560596,1.61258330249198));
#43569=CARTESIAN_POINT('',(4.51787557461174,0.000108094638884985,1.88741669750807));
#43570=CARTESIAN_POINT('',(4.51775,5.53264807684796E-16,20.5));
#43571=CARTESIAN_POINT('Ctrl Pts',(4.51787557461174,0.000108094638884985,
1.88741669750807));
#43572=CARTESIAN_POINT('Ctrl Pts',(4.51800988663209,0.133281854142107,1.89210872312746));
#43573=CARTESIAN_POINT('Ctrl Pts',(4.5122387502371,0.266444013117212,1.89680074874686));
#43574=CARTESIAN_POINT('Ctrl Pts',(4.50047783691867,0.399075035061228,1.90149277436625));
#43575=CARTESIAN_POINT('Ctrl Pts',(4.43416064298431,1.14695208897868,1.92795007105072));
#43576=CARTESIAN_POINT('Ctrl Pts',(4.17739351195545,1.87794119941301,1.95440736773518));
#43577=CARTESIAN_POINT('Ctrl Pts',(3.76145039622174,2.50300870173296,1.98086466441965));
#43578=CARTESIAN_POINT('Ctrl Pts',(3.34550728048802,3.1280762040529,2.00732196110412));
#43579=CARTESIAN_POINT('Ctrl Pts',(2.77038818004944,3.64722209825845,2.03377925778859));
#43580=CARTESIAN_POINT('Ctrl Pts',(2.10614196483581,3.99721498898444,2.06023655447306));
#43581=CARTESIAN_POINT('Ctrl Pts',(1.44189574962217,4.34720787971043,2.08669385115753));
#43582=CARTESIAN_POINT('Ctrl Pts',(0.688522419633492,4.52804776695686,2.11315114784199));
#43583=CARTESIAN_POINT('Ctrl Pts',(-0.0622179873186998,4.51770855260139,
2.13960844452646));
#43584=CARTESIAN_POINT('Ctrl Pts',(-0.812958394270891,4.50736933824591,
2.16606574121093));
#43585=CARTESIAN_POINT('Ctrl Pts',(-1.56106587818659,4.30585102228854,2.1925230378954));
#43586=CARTESIAN_POINT('Ctrl Pts',(-2.21542177547916,3.9376983125846,2.21898033457986));
#43587=CARTESIAN_POINT('Ctrl Pts',(-2.86977767277172,3.56954560288067,2.24543763126433));
#43588=CARTESIAN_POINT('Ctrl Pts',(-3.43038198344116,3.03475849943017,2.2718949279488));
#43589=CARTESIAN_POINT('Ctrl Pts',(-3.82895372288602,2.39847347956868,2.29835222463327));
#43590=CARTESIAN_POINT('Ctrl Pts',(-4.22752546233088,1.76218845970719,2.32480952131774));
#43591=CARTESIAN_POINT('Ctrl Pts',(-4.46406463055117,1.0244055234347,2.35126681800221));
#43592=CARTESIAN_POINT('Ctrl Pts',(-4.50976101864305,0.274985815861316,
2.37772411468667));
#43593=CARTESIAN_POINT('Ctrl Pts',(-4.55545740673492,-0.474433891712066,
2.40418141137114));
#43594=CARTESIAN_POINT('Ctrl Pts',(-4.41031101469838,-1.23549037058635,
2.43063870805561));
#43595=CARTESIAN_POINT('Ctrl Pts',(-4.09200051244538,-1.91548778391935,
2.45709600474008));
#43596=CARTESIAN_POINT('Ctrl Pts',(-3.77369001019238,-2.59548519725235,
2.48355330142454));
#43597=CARTESIAN_POINT('Ctrl Pts',(-3.28221539772292,-3.19442354504408,
2.51001059810901));
#43598=CARTESIAN_POINT('Ctrl Pts',(-2.67743773890551,-3.63935279939741,
2.53646789479348));
#43599=CARTESIAN_POINT('Ctrl Pts',(-2.07266008008808,-4.08428205375076,
2.56292519147795));
#43600=CARTESIAN_POINT('Ctrl Pts',(-1.35457937492269,-4.37520221466569,
2.58938248816241));
#43601=CARTESIAN_POINT('Ctrl Pts',(-0.610657058576137,-4.47667952851314,
2.61583978484688));
#43602=CARTESIAN_POINT('Ctrl Pts',(0.133265257770398,-4.57815684236058,
2.64229708153135));
#43603=CARTESIAN_POINT('Ctrl Pts',(0.9030291852981,-4.49019130914055,2.66875437821582));
#43604=CARTESIAN_POINT('Ctrl Pts',(1.60487832955586,-4.22349703344507,2.69521167490029));
#43605=CARTESIAN_POINT('Ctrl Pts',(2.30672747381364,-3.95680275774959,2.72166897158476));
#43606=CARTESIAN_POINT('Ctrl Pts',(2.94066183480147,-3.51137973957866,2.74812626826922));
#43607=CARTESIAN_POINT('Ctrl Pts',(3.42946890894601,-2.94148000958192,2.77458356495369));
#43608=CARTESIAN_POINT('Ctrl Pts',(3.91827598309054,-2.37158027958518,2.80104086163816));
#43609=CARTESIAN_POINT('Ctrl Pts',(4.26195577039178,-1.67720383776263,2.82749815832263));
#43610=CARTESIAN_POINT('Ctrl Pts',(4.41864845311758,-0.94292496624017,2.85395545500709));
#43611=CARTESIAN_POINT('Ctrl Pts',(4.4847062457604,-0.633370999882247,2.86510920250742));
#43612=CARTESIAN_POINT('Ctrl Pts',(4.51753158998749,-0.316725338941023,
2.87626295000774));
#43613=CARTESIAN_POINT('Ctrl Pts',(4.5174009456275,-5.29814202112051E-5,
2.88741669750807));
#43614=CARTESIAN_POINT('Ctrl Pts',(4.51806423128285,6.30519293007281E-5,
2.61258330249198));
#43615=CARTESIAN_POINT('Ctrl Pts',(4.51759393956657,-0.687506049970836,
2.58835569556429));
#43616=CARTESIAN_POINT('Ctrl Pts',(4.35830909853907,-1.37528559362468,2.5641280886366));
#43617=CARTESIAN_POINT('Ctrl Pts',(4.0551256392357,-1.9923648496729,2.53990048170891));
#43618=CARTESIAN_POINT('Ctrl Pts',(3.72403991720982,-2.66623449779077,2.51344318502445));
#43619=CARTESIAN_POINT('Ctrl Pts',(3.22135054533116,-3.25579181863177,2.48698588833998));
#43620=CARTESIAN_POINT('Ctrl Pts',(2.60828453275314,-3.68922938300052,2.46052859165551));
#43621=CARTESIAN_POINT('Ctrl Pts',(1.99521852017512,-4.12266694736928,2.43407129497105));
#43622=CARTESIAN_POINT('Ctrl Pts',(1.27177586689775,-4.3999847552658,2.40761399828658));
#43623=CARTESIAN_POINT('Ctrl Pts',(0.526071087432441,-4.48740580460158,
2.38115670160211));
#43624=CARTESIAN_POINT('Ctrl Pts',(-0.219633692032863,-4.57482685393736,
2.35469940491764));
#43625=CARTESIAN_POINT('Ctrl Pts',(-0.987600597686097,-4.47235114471241,
2.32824210823317));
#43626=CARTESIAN_POINT('Ctrl Pts',(-1.68429211034942,-4.19246010490287,
2.3017848115487));
#43627=CARTESIAN_POINT('Ctrl Pts',(-2.38098362301274,-3.91256906509334,
2.27532751486424));
#43628=CARTESIAN_POINT('Ctrl Pts',(-3.00639974268614,-3.45526269469925,
2.24887021817977));
#43629=CARTESIAN_POINT('Ctrl Pts',(-3.48436547816518,-2.87624040350871,
2.2224129214953));
#43630=CARTESIAN_POINT('Ctrl Pts',(-3.96233121364423,-2.29721811231817,
2.19595562481083));
#43631=CARTESIAN_POINT('Ctrl Pts',(-4.29284656492891,-1.59647990033118,
2.16949832812637));
#43632=CARTESIAN_POINT('Ctrl Pts',(-4.43565512801646,-0.859374906258969,
2.1430410314419));
#43633=CARTESIAN_POINT('Ctrl Pts',(-4.578463691104,-0.122269912186753,2.11658373475743));
#43634=CARTESIAN_POINT('Ctrl Pts',(-4.53356546599441,0.651201863970698,
2.09012643807296));
#43635=CARTESIAN_POINT('Ctrl Pts',(-4.30642900683079,1.36683241594063,2.06366914138849));
#43636=CARTESIAN_POINT('Ctrl Pts',(-4.07929254766716,2.08246296791056,2.03721184470403));
#43637=CARTESIAN_POINT('Ctrl Pts',(-3.66991785444949,2.74025229569297,2.01075454801956));
#43638=CARTESIAN_POINT('Ctrl Pts',(-3.12816631171559,3.26008238708848,1.98429725133509));
#43639=CARTESIAN_POINT('Ctrl Pts',(-2.58641476898168,3.77991247848399,1.95783995465062));
#43640=CARTESIAN_POINT('Ctrl Pts',(-1.91228637673154,4.16178333349259,1.93138265796616));
#43641=CARTESIAN_POINT('Ctrl Pts',(-1.18788922711582,4.3591835047376,1.90492536128169));
#43642=CARTESIAN_POINT('Ctrl Pts',(-0.463492077500105,4.55658367598262,
1.87846806459722));
#43643=CARTESIAN_POINT('Ctrl Pts',(0.311173829481187,4.56951316346406,1.85201076791275));
#43644=CARTESIAN_POINT('Ctrl Pts',(1.04175504380577,4.39639716966128,1.82555347122828));
#43645=CARTESIAN_POINT('Ctrl Pts',(1.77233625813035,4.2232811758585,1.79909617454381));
#43646=CARTESIAN_POINT('Ctrl Pts',(2.45883277979823,3.86411970077152,1.77263887785935));
#43647=CARTESIAN_POINT('Ctrl Pts',(3.01763009204651,3.36265821505193,1.74618158117488));
#43648=CARTESIAN_POINT('Ctrl Pts',(3.57642740429479,2.86119672933234,1.71972428449041));
#43649=CARTESIAN_POINT('Ctrl Pts',(4.00752550712348,2.21743523298015,1.69326698780594));
#43650=CARTESIAN_POINT('Ctrl Pts',(4.2584171290782,1.50978316287142,1.66680969112148));
#43651=CARTESIAN_POINT('Ctrl Pts',(4.42982474689917,1.02631960741915,1.64873422824498));
#43652=CARTESIAN_POINT('Ctrl Pts',(4.51712029378003,0.513034879908299,1.63065876536848));
#43653=CARTESIAN_POINT('Ctrl Pts',(4.51755838390264,-0.00010457874560596,
1.61258330249198));
#43654=CARTESIAN_POINT('Origin',(0.,0.,20.5));
#43655=CARTESIAN_POINT('',(4.51763087883895,0.00011359767064345,0.612583302491977));
#43656=CARTESIAN_POINT('',(4.5177656910975,-0.000116631996953637,0.887416697508071));
#43657=CARTESIAN_POINT('',(4.51775,5.53264807684796E-16,20.5));
#43658=CARTESIAN_POINT('',(-3.4337878873619,2.93584158412996,0.));
#43659=CARTESIAN_POINT('Ctrl Pts',(4.51763087883895,0.00011359767064345,
0.612583302491977));
#43660=CARTESIAN_POINT('Ctrl Pts',(4.51711863846112,-0.539057740350668,
0.59358994511926));
#43661=CARTESIAN_POINT('Ctrl Pts',(4.42053200733307,-1.07840729234144,0.574596587746541));
#43662=CARTESIAN_POINT('Ctrl Pts',(4.23165828048039,-1.58323058504537,0.555603230373824));
#43663=CARTESIAN_POINT('Ctrl Pts',(3.96856165521391,-2.28643746765176,0.529145933689356));
#43664=CARTESIAN_POINT('Ctrl Pts',(3.52639272074203,-2.92265018460396,0.502688637004889));
#43665=CARTESIAN_POINT('Ctrl Pts',(2.95900217961999,-3.41436616507663,0.476231340320421));
#43666=CARTESIAN_POINT('Ctrl Pts',(2.39161163849795,-3.90608214554931,0.449774043635953));
#43667=CARTESIAN_POINT('Ctrl Pts',(1.69899949072575,-4.25330138954245,0.423316746951485));
#43668=CARTESIAN_POINT('Ctrl Pts',(0.965534545329656,-4.41375671437595,
0.396859450267017));
#43669=CARTESIAN_POINT('Ctrl Pts',(0.232069599933564,-4.57421203920944,
0.370402153582549));
#43670=CARTESIAN_POINT('Ctrl Pts',(-0.542248143086422,-4.54790344488329,
0.343944856898081));
#43671=CARTESIAN_POINT('Ctrl Pts',(-1.26312545635881,-4.33799038903376,
0.317487560213613));
#43672=CARTESIAN_POINT('Ctrl Pts',(-1.9840027696312,-4.12807733318424,0.291030263529145));
#43673=CARTESIAN_POINT('Ctrl Pts',(-2.651439653156,-3.73455981581135,0.264572966844678));
#43674=CARTESIAN_POINT('Ctrl Pts',(-3.18410908512135,-3.20545326780586,
0.23811567016021));
#43675=CARTESIAN_POINT('Ctrl Pts',(-3.71677851708671,-2.67634671980037,
0.211658373475742));
#43676=CARTESIAN_POINT('Ctrl Pts',(-4.11468049749262,-2.01165114116227,
0.185201076791274));
#43677=CARTESIAN_POINT('Ctrl Pts',(-4.32941757999959,-1.29215909736801,
0.158743780106806));
#43678=CARTESIAN_POINT('Ctrl Pts',(-4.54415466250656,-0.572667053573755,
0.132286483422338));
#43679=CARTESIAN_POINT('Ctrl Pts',(-4.57572684711458,0.201621455376676,
0.10582918673787));
#43680=CARTESIAN_POINT('Ctrl Pts',(-4.42014586550132,0.936043740039453,
0.0793718900534021));
#43681=CARTESIAN_POINT('Ctrl Pts',(-4.26456488388806,1.67046602470223,0.0529145933689342));
#43682=CARTESIAN_POINT('Ctrl Pts',(-3.92183073605352,2.36502208507736,0.0264572966844666));
#43683=CARTESIAN_POINT('Ctrl Pts',(-3.43378788736187,2.93584158412999,-1.38777878078145E-15));
#43684=CARTESIAN_POINT('',(3.43409108914489,2.93606647242259,-1.66533453693773E-15));
#43685=CARTESIAN_POINT('Origin',(0.,0.,0.));
#43686=CARTESIAN_POINT('Ctrl Pts',(3.43409108914489,2.93606647242259,-1.66533453693773E-15));
#43687=CARTESIAN_POINT('Ctrl Pts',(2.96705577784701,3.48188002612677,0.0253131010459874));
#43688=CARTESIAN_POINT('Ctrl Pts',(2.36757358452891,3.91460873741651,0.0506262020919764));
#43689=CARTESIAN_POINT('Ctrl Pts',(1.70215900486043,4.18523117809474,0.0759393031379656));
#43690=CARTESIAN_POINT('Ctrl Pts',(1.00666654344788,4.46808621784236,0.102396599822434));
#43691=CARTESIAN_POINT('Ctrl Pts',(0.23914646876357,4.57384880856985,0.128853896506902));
#43692=CARTESIAN_POINT('Ctrl Pts',(-0.506923795872801,4.48961228541997,
0.15531119319137));
#43693=CARTESIAN_POINT('Ctrl Pts',(-1.25299406050917,4.40537576227008,0.181768489875837));
#43694=CARTESIAN_POINT('Ctrl Pts',(-1.9776145150976,4.13114012524282,0.208225786560305));
#43695=CARTESIAN_POINT('Ctrl Pts',(-2.59252418705973,3.70032015205329,0.234683083244772));
#43696=CARTESIAN_POINT('Ctrl Pts',(-3.20743385902187,3.26950017886376,0.26114037992924));
#43697=CARTESIAN_POINT('Ctrl Pts',(-3.71263274835771,2.68209586951196,0.287597676613709));
#43698=CARTESIAN_POINT('Ctrl Pts',(-4.04658977984313,2.00964543895375,0.314054973298177));
#43699=CARTESIAN_POINT('Ctrl Pts',(-4.38054681132855,1.33719500839555,0.340512269982645));
#43700=CARTESIAN_POINT('Ctrl Pts',(-4.54326198496355,0.579698456630952,
0.366969566667112));
#43701=CARTESIAN_POINT('Ctrl Pts',(-4.51491593042486,-0.170578278221808,
0.39342686335158));
#43702=CARTESIAN_POINT('Ctrl Pts',(-4.48656987588618,-0.920855013074566,
0.419884160036048));
#43703=CARTESIAN_POINT('Ctrl Pts',(-4.26716259317382,-1.66391193101549,
0.446341456720516));
#43704=CARTESIAN_POINT('Ctrl Pts',(-3.88341809255795,-2.30924747945238,
0.472798753404984));
#43705=CARTESIAN_POINT('Ctrl Pts',(-3.49967359194208,-2.95458302788927,
0.499256050089452));
#43706=CARTESIAN_POINT('Ctrl Pts',(-2.95159187342268,-3.50219720682213,
0.52571334677392));
#43707=CARTESIAN_POINT('Ctrl Pts',(-2.30592844750098,-3.88539017854139,
0.552170643458388));
#43708=CARTESIAN_POINT('Ctrl Pts',(-1.66026502157927,-4.26858315026064,
0.578627940142856));
#43709=CARTESIAN_POINT('Ctrl Pts',(-0.91701988825525,-4.48735491476628,
0.605085236827324));
#43710=CARTESIAN_POINT('Ctrl Pts',(-0.166719607306316,-4.51505986234428,
0.631542533511792));
#43711=CARTESIAN_POINT('Ctrl Pts',(0.583580673642613,-4.54276480992227,
0.65799983019626));
#43712=CARTESIAN_POINT('Ctrl Pts',(1.34093610221646,-4.37940294057262,0.684457126880727));
#43713=CARTESIAN_POINT('Ctrl Pts',(2.01310169166318,-4.04487125838886,0.710914423565195));
#43714=CARTESIAN_POINT('Ctrl Pts',(2.68526728110991,-3.7103395762051,0.737371720249663));
#43715=CARTESIAN_POINT('Ctrl Pts',(3.27224303142951,-3.20463808118722,0.763829016934131));
#43716=CARTESIAN_POINT('Ctrl Pts',(3.70253591076623,-2.58936080975925,0.790286313618599));
#43717=CARTESIAN_POINT('Ctrl Pts',(4.13282879010294,-1.9740835383313,0.816743610303067));
#43718=CARTESIAN_POINT('Ctrl Pts',(4.40643879845678,-1.24923049049327,0.843200906987535));
#43719=CARTESIAN_POINT('Ctrl Pts',(4.49004055820744,-0.503087883691874,
0.869658203672002));
#43720=CARTESIAN_POINT('Ctrl Pts',(4.50874543387838,-0.336147561686243,
0.875577701617358));
#43721=CARTESIAN_POINT('Ctrl Pts',(4.51793876013751,-0.168141513884366,
0.881497199562714));
#43722=CARTESIAN_POINT('Ctrl Pts',(4.5177656910975,-0.000116631996953637,
0.887416697508071));
#43723=CARTESIAN_POINT('Origin',(0.,0.,-2.20833684463713));
#43724=CARTESIAN_POINT('',(5.07403060246553,1.54698778687123E-5,39.208336844637));
#43725=CARTESIAN_POINT('',(5.07396752856948,-6.48011021279027E-5,39.2916631553629));
#43726=CARTESIAN_POINT('',(5.0736,-1.85409460923845E-12,-2.20833684463713));
#43727=CARTESIAN_POINT('',(-1.31303618635666,-4.90075024188317,40.));
#43728=CARTESIAN_POINT('Ctrl Pts',(5.07396752856948,-6.48011021277175E-5,
39.2916631553629));
#43729=CARTESIAN_POINT('Ctrl Pts',(5.07347424400433,0.779307331517198,39.3161170634328));
#43730=CARTESIAN_POINT('Ctrl Pts',(4.69381943413572,2.40236770827343,39.3670282681872));
#43731=CARTESIAN_POINT('Ctrl Pts',(3.03470961035893,4.33144609848054,39.4443967696262));
#43732=CARTESIAN_POINT('Ctrl Pts',(0.593383061700927,5.25537632570972,39.5237686596795));
#43733=CARTESIAN_POINT('Ctrl Pts',(-1.99247705733066,4.8990504464678,39.603140549733));
#43734=CARTESIAN_POINT('Ctrl Pts',(-4.09299916691649,3.34943642687039,39.6825124397864));
#43735=CARTESIAN_POINT('Ctrl Pts',(-5.19642846461573,0.983699440459269,
39.7618843298398));
#43736=CARTESIAN_POINT('Ctrl Pts',(-5.03410925482033,-1.62126816458454,
39.8412562198932));
#43737=CARTESIAN_POINT('Ctrl Pts',(-3.6453165085118,-3.83208153227987,39.9206281099466));
#43738=CARTESIAN_POINT('Ctrl Pts',(-2.12771778283764,-4.68247622999901,
39.9735427033155));
#43739=CARTESIAN_POINT('Ctrl Pts',(-1.31303618635638,-4.90075024188325,
40.));
#43740=CARTESIAN_POINT('',(1.31317395760221,-4.90115117757563,40.));
#43741=CARTESIAN_POINT('Origin',(0.,0.,40.));
#43742=CARTESIAN_POINT('Ctrl Pts',(5.07403060246553,1.54698778688793E-5,
39.208336844637));
#43743=CARTESIAN_POINT('Ctrl Pts',(5.07403315687698,0.0146420671929676,
39.2087957918851));
#43744=CARTESIAN_POINT('Ctrl Pts',(5.07040151797183,0.872458469457581,39.2357120358177));
#43745=CARTESIAN_POINT('Ctrl Pts',(4.62253485344793,2.56965255248844,39.2890855764349));
#43746=CARTESIAN_POINT('Ctrl Pts',(2.83047200092405,4.46759066254981,39.3684574664882));
#43747=CARTESIAN_POINT('Ctrl Pts',(0.34891291852996,5.27723479734496,39.4478293565417));
#43748=CARTESIAN_POINT('Ctrl Pts',(-2.21764149317963,4.80135391043001,39.527201246595));
#43749=CARTESIAN_POINT('Ctrl Pts',(-4.24398161873814,3.15587819282133,39.6065731366485));
#43750=CARTESIAN_POINT('Ctrl Pts',(-5.23650047694821,0.74162931109825,39.6859450267018));
#43751=CARTESIAN_POINT('Ctrl Pts',(-4.9534132521342,-1.85326330477585,39.7653169167553));
#43752=CARTESIAN_POINT('Ctrl Pts',(-3.46369715057683,-3.99673439595749,
39.8446888068086));
#43753=CARTESIAN_POINT('Ctrl Pts',(-1.1638488125998,-5.14969078544563,39.9229165012236));
#43754=CARTESIAN_POINT('Ctrl Pts',(0.533836595431815,-5.10962665469158,
39.974686898954));
#43755=CARTESIAN_POINT('Ctrl Pts',(1.31317395760221,-4.90115117757563,40.));
#43756=CARTESIAN_POINT('Origin',(0.,0.,-2.20833684463713));
#43757=CARTESIAN_POINT('',(5.07325764975804,-8.44407784307555E-5,38.208336844637));
#43758=CARTESIAN_POINT('',(5.07316912366228,-1.81818814078922E-5,38.2916631553629));
#43759=CARTESIAN_POINT('',(5.0736,-1.85409460923845E-12,-2.20833684463713));
#43760=CARTESIAN_POINT('Ctrl Pts',(5.07316912366228,-1.81818814076751E-5,
38.2916631553629));
#43761=CARTESIAN_POINT('Ctrl Pts',(5.07311400239361,0.441352830351579,38.3055055398681));
#43762=CARTESIAN_POINT('Ctrl Pts',(4.90711571561459,1.72636801461904,38.3458052210578));
#43763=CARTESIAN_POINT('Ctrl Pts',(3.83482475204887,3.64212307300276,38.4125621989319));
#43764=CARTESIAN_POINT('Ctrl Pts',(1.62575061805696,5.03268082057242,38.4919340889853));
#43765=CARTESIAN_POINT('Ctrl Pts',(-0.979352771366501,5.19728867487039,
38.5713059790387));
#43766=CARTESIAN_POINT('Ctrl Pts',(-3.3458879870052,4.09584848370752,38.6506778690921));
#43767=CARTESIAN_POINT('Ctrl Pts',(-4.89737230716795,1.99666872129193,38.7300497591456));
#43768=CARTESIAN_POINT('Ctrl Pts',(-5.2558675504918,-0.588895222855594,
38.809421649199));
#43769=CARTESIAN_POINT('Ctrl Pts',(-4.33404513553914,-3.03100540392653,
38.8887935392523));
#43770=CARTESIAN_POINT('Ctrl Pts',(-2.35645883694701,-4.73476973691708,
38.9681654293058));
#43771=CARTESIAN_POINT('Ctrl Pts',(0.195155463808245,-5.28515396379923,
39.0475373193592));
#43772=CARTESIAN_POINT('Ctrl Pts',(2.69923061743519,-4.54808766460433,39.1269092094126));
#43773=CARTESIAN_POINT('Ctrl Pts',(4.5457786161602,-2.70311485851688,39.2062810994659));
#43774=CARTESIAN_POINT('Ctrl Pts',(5.05724155748156,-0.970965988519946,
39.2611990814494));
#43775=CARTESIAN_POINT('Ctrl Pts',(5.07400794095178,-0.063914933051532,
39.2896597667484));
#43776=CARTESIAN_POINT('Ctrl Pts',(5.07396752856948,-6.48011021277175E-5,
39.2916631553629));
#43777=CARTESIAN_POINT('Ctrl Pts',(5.07325764975804,-8.44407784305126E-5,
38.208336844637));
#43778=CARTESIAN_POINT('Ctrl Pts',(5.07294945930103,0.51977335908998,38.2246415650049));
#43779=CARTESIAN_POINT('Ctrl Pts',(4.86451980067584,1.88343404898941,38.2674035820572));
#43780=CARTESIAN_POINT('Ctrl Pts',(3.66171031660113,3.81612616476472,38.336622895794));
#43781=CARTESIAN_POINT('Ctrl Pts',(1.39049711694169,5.10269135980963,38.4159947858473));
#43782=CARTESIAN_POINT('Ctrl Pts',(-1.21943810235573,5.14625223481529,38.4953666759008));
#43783=CARTESIAN_POINT('Ctrl Pts',(-3.53232089954511,3.93619745533324,38.5747385659542));
#43784=CARTESIAN_POINT('Ctrl Pts',(-4.98473814342406,1.76729369047725,38.6541104560076));
#43785=CARTESIAN_POINT('Ctrl Pts',(-5.22288421068334,-0.832118909543577,
38.733482346061));
#43786=CARTESIAN_POINT('Ctrl Pts',(-4.18874724188046,-3.22882917750522,
38.8128542361144));
#43787=CARTESIAN_POINT('Ctrl Pts',(-2.13424072225093,-4.83900381899058,
38.8922261261678));
#43788=CARTESIAN_POINT('Ctrl Pts',(0.440162123945958,-5.27040781417516,
38.9715980162212));
#43789=CARTESIAN_POINT('Ctrl Pts',(2.90734243084964,-4.41795218255951,39.0509699062746));
#43790=CARTESIAN_POINT('Ctrl Pts',(4.65612987828293,-2.500445050276,39.1298828490799));
#43791=CARTESIAN_POINT('Ctrl Pts',(5.07388590069044,-0.828549010266373,
39.1823384952007));
#43792=CARTESIAN_POINT('Ctrl Pts',(5.07403060246553,1.54698778688793E-5,
39.208336844637));
#43793=CARTESIAN_POINT('Origin',(0.,0.,-2.20833684463713));
#43794=CARTESIAN_POINT('',(5.07364050160013,0.000130038443658109,37.208336844637));
#43795=CARTESIAN_POINT('',(5.07387656802193,9.59844669708175E-5,37.2916631553629));
#43796=CARTESIAN_POINT('',(5.0736,-1.85409460923845E-12,-2.20833684463713));
#43797=CARTESIAN_POINT('Ctrl Pts',(5.07387656802193,9.59844669710073E-5,
37.2916631553629));
#43798=CARTESIAN_POINT('Ctrl Pts',(5.07396569861154,0.103072231247123,37.2948940163033));
#43799=CARTESIAN_POINT('Ctrl Pts',(5.04574853055582,1.04926503651591,37.3245821739283));
#43800=CARTESIAN_POINT('Ctrl Pts',(4.48202491545551,2.80756015154514,37.3807276282377));
#43801=CARTESIAN_POINT('Ctrl Pts',(2.59328691715162,4.6093171199916,37.4600995182911));
#43802=CARTESIAN_POINT('Ctrl Pts',(0.0728299659736646,5.28825464055466,
37.5394714083445));
#43803=CARTESIAN_POINT('Ctrl Pts',(-2.46536820371075,4.67898503603898,37.6188432983979));
#43804=CARTESIAN_POINT('Ctrl Pts',(-4.40300813596802,2.92992503348812,37.6982151884513));
#43805=CARTESIAN_POINT('Ctrl Pts',(-5.26808503220261,0.467141778084607,
37.7775870785047));
#43806=CARTESIAN_POINT('Ctrl Pts',(-4.84986807528987,-2.10943618050861,
37.8569589685581));
#43807=CARTESIAN_POINT('Ctrl Pts',(-3.2502339902585,-4.17216015459505,37.9363308586115));
#43808=CARTESIAN_POINT('Ctrl Pts',(-0.858850099431265,-5.21855515011692,
38.0157027486649));
#43809=CARTESIAN_POINT('Ctrl Pts',(1.74174777450972,-4.99372166181591,38.0950746387183));
#43810=CARTESIAN_POINT('Ctrl Pts',(3.91805974601555,-3.55242863073569,38.1744465287717));
#43811=CARTESIAN_POINT('Ctrl Pts',(4.92684606433671,-1.64805066527608,38.2399760343199));
#43812=CARTESIAN_POINT('Ctrl Pts',(5.0732193570569,-0.402250655317197,38.2790482431836));
#43813=CARTESIAN_POINT('Ctrl Pts',(5.07316912366228,-1.81818814076751E-5,
38.2916631553629));
#43814=CARTESIAN_POINT('Ctrl Pts',(5.07364050160013,0.000130038443658265,
37.208336844637));
#43815=CARTESIAN_POINT('Ctrl Pts',(5.07382783063862,0.181611936494348,37.2140300414401));
#43816=CARTESIAN_POINT('Ctrl Pts',(5.01990561118457,1.20636170521342,37.2461805349277));
#43817=CARTESIAN_POINT('Ctrl Pts',(4.34693493313475,3.01249033764469,37.3047883250998));
#43818=CARTESIAN_POINT('Ctrl Pts',(2.37663436681862,4.72467463787371,37.3841602151531));
#43819=CARTESIAN_POINT('Ctrl Pts',(-0.17260907066365,5.28593865420645,37.4635321052065));
#43820=CARTESIAN_POINT('Ctrl Pts',(-2.67980532059584,4.55955971460153,37.54290399526));
#43821=CARTESIAN_POINT('Ctrl Pts',(-4.53420692607955,2.72248212093334,37.6222758853133));
#43822=CARTESIAN_POINT('Ctrl Pts',(-5.28408576066665,0.222213908718847,
37.7016477753668));
#43823=CARTESIAN_POINT('Ctrl Pts',(-4.74677300008161,-2.33218511979937,
37.7810196654201));
#43824=CARTESIAN_POINT('Ctrl Pts',(-3.05315684347904,-4.31846901533503,
37.8603915554736));
#43825=CARTESIAN_POINT('Ctrl Pts',(-0.615798437855754,-5.25278341751105,
37.9397634455269));
#43826=CARTESIAN_POINT('Ctrl Pts',(1.97156710418767,-4.90753140600709,38.0191353355804));
#43827=CARTESIAN_POINT('Ctrl Pts',(4.07866326363087,-3.36681560666115,38.0985072256337));
#43828=CARTESIAN_POINT('Ctrl Pts',(4.96346005639167,-1.49092415374923,38.1615743953193));
#43829=CARTESIAN_POINT('Ctrl Pts',(5.07344955290414,-0.323787998268402,
38.1981842683204));
#43830=CARTESIAN_POINT('Ctrl Pts',(5.07325764975804,-8.44407784305126E-5,
38.208336844637));
#43831=CARTESIAN_POINT('Origin',(0.,0.,-2.20833684463713));
#43832=CARTESIAN_POINT('',(5.07371855919287,-0.000123991516001801,36.208336844637));
#43833=CARTESIAN_POINT('',(5.07347409402005,-0.000127990615926579,36.2916631553629));
#43834=CARTESIAN_POINT('',(5.0736,-1.85409460923845E-12,-2.20833684463713));
#43835=CARTESIAN_POINT('Ctrl Pts',(5.07347409402005,-0.00012799061592652,
36.2916631553629));
#43836=CARTESIAN_POINT('Ctrl Pts',(5.07289252391416,0.608034774450749,36.3107397894231));
#43837=CARTESIAN_POINT('Ctrl Pts',(4.81166108430775,2.06014185956918,36.3562737201677));
#43838=CARTESIAN_POINT('Ctrl Pts',(3.45741385862894,4.002153265115,36.4282649475969));
#43839=CARTESIAN_POINT('Ctrl Pts',(1.12210854951209,5.16834729390565,36.5076368376502));
#43840=CARTESIAN_POINT('Ctrl Pts',(-1.4865399185207,5.07554336184357,36.5870087277037));
#43841=CARTESIAN_POINT('Ctrl Pts',(-3.73307055280216,3.74634830136112,36.666380617757));
#43842=CARTESIAN_POINT('Ctrl Pts',(-5.07023346343257,1.50455108706837,36.7457525078105));
#43843=CARTESIAN_POINT('Ctrl Pts',(-5.17229872514219,-1.10375144176689,
36.8251243978638));
#43844=CARTESIAN_POINT('Ctrl Pts',(-4.01440346609619,-3.44318256250012,
36.9044962879173));
#43845=CARTESIAN_POINT('Ctrl Pts',(-1.87860840844056,-4.94386203236358,
36.9838681779707));
#43846=CARTESIAN_POINT('Ctrl Pts',(0.71481149928202,-5.24022765419639,37.0632400680241));
#43847=CARTESIAN_POINT('Ctrl Pts',(3.13410490798792,-4.26008541851396,37.1426119580775));
#43848=CARTESIAN_POINT('Ctrl Pts',(4.72253605350391,-2.32433471697507,37.2187529871904));
#43849=CARTESIAN_POINT('Ctrl Pts',(5.07323581438062,-0.740193128270358,
37.2684367196189));
#43850=CARTESIAN_POINT('Ctrl Pts',(5.07387656802193,9.59844669710073E-5,
37.2916631553629));
#43851=CARTESIAN_POINT('Ctrl Pts',(5.07371855919287,-0.000123991516001801,
36.208336844637));
#43852=CARTESIAN_POINT('Ctrl Pts',(5.07301904482133,0.686442797877024,36.2298758145598));
#43853=CARTESIAN_POINT('Ctrl Pts',(4.76024594010631,2.21696867292356,36.2778720811671));
#43854=CARTESIAN_POINT('Ctrl Pts',(3.26800144929601,4.15825779320007,36.3523256444589));
#43855=CARTESIAN_POINT('Ctrl Pts',(0.881102883784141,5.2148441065383,36.4316975345123));
#43856=CARTESIAN_POINT('Ctrl Pts',(-1.72043039392939,5.00110593838543,36.5110694245656));
#43857=CARTESIAN_POINT('Ctrl Pts',(-3.90287063578981,3.56910943340206,36.5904413146191));
#43858=CARTESIAN_POINT('Ctrl Pts',(-5.13458022962944,1.26768577053169,36.6698132046725));
#43859=CARTESIAN_POINT('Ctrl Pts',(-5.11551744473188,-1.34254334006536,
36.7491850947259));
#43860=CARTESIAN_POINT('Ctrl Pts',(-3.85032593330342,-3.62573186469175,
36.8285569847793));
#43861=CARTESIAN_POINT('Ctrl Pts',(-1.64720354707418,-5.02570013250056,
36.9079288748327));
#43862=CARTESIAN_POINT('Ctrl Pts',(0.957173977199105,-5.20141897223083,
36.9873007648861));
#43863=CARTESIAN_POINT('Ctrl Pts',(3.32838603929536,-4.11008366347129,37.0666726549395));
#43864=CARTESIAN_POINT('Ctrl Pts',(4.77688430036561,-2.16763522711972,37.1403513481898));
#43865=CARTESIAN_POINT('Ctrl Pts',(5.07295727932621,-0.661766675847902,
37.1875727447556));
#43866=CARTESIAN_POINT('Ctrl Pts',(5.07364050160013,0.000130038443658265,
37.208336844637));
#43867=CARTESIAN_POINT('Origin',(0.,0.,-2.20833684463713));
#43868=CARTESIAN_POINT('',(5.07321765521711,6.54440514302745E-5,35.208336844637));
#43869=CARTESIAN_POINT('',(5.07337786466077,0.000116280867786642,35.2916631553629));
#43870=CARTESIAN_POINT('',(5.0736,-1.85409460923845E-12,-2.20833684463713));
#43871=CARTESIAN_POINT('Ctrl Pts',(5.07337786466077,0.000116280867786742,
35.2916631553629));
#43872=CARTESIAN_POINT('Ctrl Pts',(5.07360553071623,0.269998548266127,35.3001282658583));
#43873=CARTESIAN_POINT('Ctrl Pts',(4.98629871182508,1.38323904612086,35.3350506730382));
#43874=CARTESIAN_POINT('Ctrl Pts',(4.18367369924664,3.23540039647985,35.3964303769026));
#43875=CARTESIAN_POINT('Ctrl Pts',(2.12664217080567,4.8423480280398,35.4758022669559));
#43876=CARTESIAN_POINT('Ctrl Pts',(-0.448434683200953,5.2697103983248,35.5551741570095));
#43877=CARTESIAN_POINT('Ctrl Pts',(-2.91427384097317,4.41338297988397,35.6345460470627));
#43878=CARTESIAN_POINT('Ctrl Pts',(-4.67020234172003,2.48196523640092,35.7139179371163));
#43879=CARTESIAN_POINT('Ctrl Pts',(-5.28847988934142,-0.0540537449324728,
35.7932898271696));
#43880=CARTESIAN_POINT('Ctrl Pts',(-4.61849544177097,-2.57690535364626,
35.872661717223));
#43881=CARTESIAN_POINT('Ctrl Pts',(-2.82345572745135,-4.47202852209511,
35.9520336072764));
#43882=CARTESIAN_POINT('Ctrl Pts',(-0.340628447537815,-5.27777544122882,
36.0314054973298));
#43883=CARTESIAN_POINT('Ctrl Pts',(2.22517516822766,-4.79786794503694,36.1107773873833));
#43884=CARTESIAN_POINT('Ctrl Pts',(4.2489310383545,-3.14921043733466,36.1901492774366));
#43885=CARTESIAN_POINT('Ctrl Pts',(5.00002147582269,-1.31403716914749,36.2504445334299));
#43886=CARTESIAN_POINT('Ctrl Pts',(5.07369910083888,-0.235423387877496,
36.2842824927386));
#43887=CARTESIAN_POINT('Ctrl Pts',(5.07347409402005,-0.00012799061592652,
36.2916631553629));
#43888=CARTESIAN_POINT('Ctrl Pts',(5.07321765521711,6.54440514305868E-5,
35.208336844637));
#43889=CARTESIAN_POINT('Ctrl Pts',(5.07337613287412,0.348482730653562,35.2192642909951));
#43890=CARTESIAN_POINT('Ctrl Pts',(4.95236148577976,1.54037186125541,35.2566490340376));
#43891=CARTESIAN_POINT('Ctrl Pts',(4.02905439992751,3.42602714375337,35.3204910737646));
#43892=CARTESIAN_POINT('Ctrl Pts',(1.8996801667365,4.93580354262787,35.3998629638181));
#43893=CARTESIAN_POINT('Ctrl Pts',(-0.69245195020073,5.24322912373406,35.4792348538714));
#43894=CARTESIAN_POINT('Ctrl Pts',(-3.11590430478548,4.27341569598948,35.5586067439249));
#43895=CARTESIAN_POINT('Ctrl Pts',(-4.78032926766171,2.26260766374704,35.6379786339782));
#43896=CARTESIAN_POINT('Ctrl Pts',(-5.28027660201491,-0.299366587187078,
35.7173505240316));
#43897=CARTESIAN_POINT('Ctrl Pts',(-4.49396024381123,-2.78841580011912,
35.7967224140851));
#43898=CARTESIAN_POINT('Ctrl Pts',(-2.61292511742748,-4.59821309619579,
35.8760943041384));
#43899=CARTESIAN_POINT('Ctrl Pts',(-0.0953872160500441,-5.28789586001125,
35.9554661941919));
#43900=CARTESIAN_POINT('Ctrl Pts',(2.4453868000212,-4.68945889688694,36.0348380842453));
#43901=CARTESIAN_POINT('Ctrl Pts',(4.39047000437915,-2.94868012642215,36.1142099742987));
#43902=CARTESIAN_POINT('Ctrl Pts',(5.02844178521537,-1.15692185290368,36.1720428944293));
#43903=CARTESIAN_POINT('Ctrl Pts',(5.07387829014872,-0.156898425299628,
36.2034185178754));
#43904=CARTESIAN_POINT('Ctrl Pts',(5.07371855919287,-0.000123991516001801,
36.208336844637));
#43905=CARTESIAN_POINT('Origin',(0.,0.,-2.20833684463713));
#43906=CARTESIAN_POINT('',(5.07403267809782,1.0680673442065E-5,34.208336844637));
#43907=CARTESIAN_POINT('',(5.07395837593185,-6.84743504405761E-5,34.2916631553629));
#43908=CARTESIAN_POINT('',(5.0736,-1.85409460923845E-12,-2.20833684463713));
#43909=CARTESIAN_POINT('Ctrl Pts',(5.07395837593184,-6.84743504405106E-5,
34.2916631553629));
#43910=CARTESIAN_POINT('Ctrl Pts',(5.07344266957576,0.774748712740892,34.315974038978));
#43911=CARTESIAN_POINT('Ctrl Pts',(4.69722240792898,2.39327548011594,34.3667422192777));
#43912=CARTESIAN_POINT('Ctrl Pts',(3.04637426047967,4.32325632045994,34.4439676962618));
#43913=CARTESIAN_POINT('Ctrl Pts',(0.607552238322964,5.25374358196314,34.5233395863151));
#43914=CARTESIAN_POINT('Ctrl Pts',(-1.97926816429518,4.90443053586424,34.6027114763686));
#43915=CARTESIAN_POINT('Ctrl Pts',(-4.08394322312674,3.36040906700167,34.6820833664219));
#43916=CARTESIAN_POINT('Ctrl Pts',(-5.19377875245966,0.997799387556786,
34.7614552564754));
#43917=CARTESIAN_POINT('Ctrl Pts',(-5.03842127392763,-1.60787201410546,
34.8408271465287));
#43918=CARTESIAN_POINT('Ctrl Pts',(-3.65571552542313,-3.82186935209593,
34.9201990365822));
#43919=CARTESIAN_POINT('Ctrl Pts',(-1.38248556671468,-5.10486777548014,
34.9995709266355));
#43920=CARTESIAN_POINT('Ctrl Pts',(1.22751481596557,-5.14433170819057,35.078942816689));
#43921=CARTESIAN_POINT('Ctrl Pts',(3.53849530653457,-3.93064782357091,35.1583147067423));
#43922=CARTESIAN_POINT('Ctrl Pts',(4.83296736710027,-1.99102597475866,35.2292214863004));
#43923=CARTESIAN_POINT('Ctrl Pts',(5.07289397138366,-0.573505529121166,
35.2736709691739));
#43924=CARTESIAN_POINT('Ctrl Pts',(5.07337786466077,0.000116280867786742,
35.2916631553629));
#43925=CARTESIAN_POINT('Ctrl Pts',(5.07403267809783,1.06806734422689E-5,
34.208336844637));
#43926=CARTESIAN_POINT('Ctrl Pts',(5.07403390825189,0.0100790925016438,
34.2086527674304));
#43927=CARTESIAN_POINT('Ctrl Pts',(5.07154731505229,0.863336953552071,34.2354259869081));
#43928=CARTESIAN_POINT('Ctrl Pts',(4.62944563286023,2.55718096342464,34.2886565030704));
#43929=CARTESIAN_POINT('Ctrl Pts',(2.84250620674923,4.45994392474861,34.3680283931238));
#43930=CARTESIAN_POINT('Ctrl Pts',(0.363138560454883,5.27627441792225,34.4474002831772));
#43931=CARTESIAN_POINT('Ctrl Pts',(-2.20468883537271,4.80731614172534,34.5267721732306));
#43932=CARTESIAN_POINT('Ctrl Pts',(-4.23545891089946,3.1673062942179,34.606144063284));
#43933=CARTESIAN_POINT('Ctrl Pts',(-5.23448057076036,0.755747644152594,
34.6855159533374));
#43934=CARTESIAN_POINT('Ctrl Pts',(-4.95839434991029,-1.83990945920924,
34.7648878433908));
#43935=CARTESIAN_POINT('Ctrl Pts',(-3.47445424064183,-3.98736869087822,
34.8442597334442));
#43936=CARTESIAN_POINT('Ctrl Pts',(-1.14414476892706,-5.16351373534018,
34.9236316234976));
#43937=CARTESIAN_POINT('Ctrl Pts',(1.4648758359769,-5.0818382631171,35.003003513551));
#43938=CARTESIAN_POINT('Ctrl Pts',(3.71705592968454,-3.76223823845686,35.0823754036044));
#43939=CARTESIAN_POINT('Ctrl Pts',(4.87836197951498,-1.83401443292226,35.1508198472998));
#43940=CARTESIAN_POINT('Ctrl Pts',(5.07299243019996,-0.495097664945923,
35.1928069943106));
#43941=CARTESIAN_POINT('Ctrl Pts',(5.07321765521711,6.54440514305868E-5,
35.208336844637));
#43942=CARTESIAN_POINT('Origin',(0.,0.,-2.20833684463713));
#43943=CARTESIAN_POINT('',(5.07324948390142,-8.11089730112791E-5,33.208336844637));
#43944=CARTESIAN_POINT('',(5.07316757009266,-1.39624117367057E-5,33.2916631553629));
#43945=CARTESIAN_POINT('',(5.0736,-1.85409460923845E-12,-2.20833684463713));
#43946=CARTESIAN_POINT('Ctrl Pts',(5.07316757009266,-1.39624117367898E-5,
33.2916631553629));
#43947=CARTESIAN_POINT('Ctrl Pts',(5.07312569317602,0.436797029802116,33.3053625154133));
#43948=CARTESIAN_POINT('Ctrl Pts',(4.90946580291021,1.7172430470973,33.3455191721481));
#43949=CARTESIAN_POINT('Ctrl Pts',(3.84462977702742,3.63177136187071,33.4121331255675));
#43950=CARTESIAN_POINT('Ctrl Pts',(1.63931253580255,5.02827960213734,33.4915050156209));
#43951=CARTESIAN_POINT('Ctrl Pts',(-0.965337610587002,5.19991006123145,
33.5708769056743));
#43952=CARTESIAN_POINT('Ctrl Pts',(-3.33483365177614,4.1048539392153,33.6502487957277));
#43953=CARTESIAN_POINT('Ctrl Pts',(-4.89197159692173,2.00986448354636,33.7296206857811));
#43954=CARTESIAN_POINT('Ctrl Pts',(-5.25743608925264,-0.574723511554913,
33.8089925758345));
#43955=CARTESIAN_POINT('Ctrl Pts',(-4.34220078737896,-3.01931013137032,
33.888364465888));
#43956=CARTESIAN_POINT('Ctrl Pts',(-2.36921498499824,-4.72839948631349,
33.9677363559413));
#43957=CARTESIAN_POINT('Ctrl Pts',(0.18090634355963,-5.28566119252548,34.0471082459947));
#43958=CARTESIAN_POINT('Ctrl Pts',(2.68695928725581,-4.55534753185087,34.1264801360481));
#43959=CARTESIAN_POINT('Ctrl Pts',(4.53847489605999,-2.71536129550809,34.2058520261016));
#43960=CARTESIAN_POINT('Ctrl Pts',(5.05594943598948,-0.980087925357289,
34.2609130325398));
#43961=CARTESIAN_POINT('Ctrl Pts',(5.07400390775537,-0.0684772480926434,
34.2895167422936));
#43962=CARTESIAN_POINT('Ctrl Pts',(5.07395837593184,-6.84743504405106E-5,
34.2916631553629));
#43963=CARTESIAN_POINT('Ctrl Pts',(5.07324948390142,-8.1108973011175E-5,
33.208336844637));
#43964=CARTESIAN_POINT('Ctrl Pts',(5.07295666213735,0.515218890813949,33.22449854055));
#43965=CARTESIAN_POINT('Ctrl Pts',(4.86710522495599,1.87431284273704,33.2671175331475));
#43966=CARTESIAN_POINT('Ctrl Pts',(3.67198507285579,3.80624052997629,33.3361938224296));
#43967=CARTESIAN_POINT('Ctrl Pts',(1.40424863498483,5.09892411381589,33.4155657124829));
#43968=CARTESIAN_POINT('Ctrl Pts',(-1.20555966211678,5.14952106980705,33.4949376025364));
#43969=CARTESIAN_POINT('Ctrl Pts',(-3.52169629398785,3.94570609146478,33.5743094925897));
#43970=CARTESIAN_POINT('Ctrl Pts',(-4.979955503786,1.78072584291395,33.6536813826432));
#43971=CARTESIAN_POINT('Ctrl Pts',(-5.22510857580638,-0.818035279400921,
33.7330532726965));
#43972=CARTESIAN_POINT('Ctrl Pts',(-4.19743676434199,-3.2175248183441,33.81242516275));
#43973=CARTESIAN_POINT('Ctrl Pts',(-2.14727864795256,-4.83323243340904,
33.8917970528034));
#43974=CARTESIAN_POINT('Ctrl Pts',(0.425951794157462,-5.27157532587404,
33.9711689428568));
#43975=CARTESIAN_POINT('Ctrl Pts',(2.89542132203897,-4.4257741373902,34.0505408329101));
#43976=CARTESIAN_POINT('Ctrl Pts',(4.6525507987008,-2.50952187653605,34.1295968001703));
#43977=CARTESIAN_POINT('Ctrl Pts',(5.07393088766675,-0.833110966960862,
34.1821954707459));
#43978=CARTESIAN_POINT('Ctrl Pts',(5.07403267809783,1.06806734422689E-5,
34.208336844637));
#43979=CARTESIAN_POINT('Origin',(0.,0.,-2.20833684463713));
#43980=CARTESIAN_POINT('',(5.07365497060222,0.000129255909634973,32.208336844637));
#43981=CARTESIAN_POINT('',(5.0738885135215,9.2741528424134E-5,32.2916631553629));
#43982=CARTESIAN_POINT('',(5.0736,-1.85409460923845E-12,-2.20833684463713));
#43983=CARTESIAN_POINT('Ctrl Pts',(5.0738885135215,9.27415284240896E-5,
32.2916631553629));
#43984=CARTESIAN_POINT('Ctrl Pts',(5.07397157552195,0.0985097427010157,
32.2947509918485));
#43985=CARTESIAN_POINT('Ctrl Pts',(5.04713500973232,1.0401410882179,32.3242961250187));
#43986=CARTESIAN_POINT('Ctrl Pts',(4.48957765297736,2.79546665964672,32.3802985548733));
#43987=CARTESIAN_POINT('Ctrl Pts',(2.60570395470567,4.60230901263064,32.4596704449267));
#43988=CARTESIAN_POINT('Ctrl Pts',(0.0870865406955613,5.28803907717593,
32.5390423349801));
#43989=CARTESIAN_POINT('Ctrl Pts',(-2.45274496186521,4.68561452739711,32.6184142250335));
#43990=CARTESIAN_POINT('Ctrl Pts',(-4.39509322077448,2.94178465017617,32.6977861150869));
#43991=CARTESIAN_POINT('Ctrl Pts',(-5.26680649947691,0.48134254370224,32.7771580051403));
#43992=CARTESIAN_POINT('Ctrl Pts',(-4.85553737278523,-2.09635354098391,
32.8565298951937));
#43993=CARTESIAN_POINT('Ctrl Pts',(-3.26147008963279,-4.16338254328624,
32.9359017852471));
#43994=CARTESIAN_POINT('Ctrl Pts',(-0.8729159117874,-5.21622077353502,33.0152736753005));
#43995=CARTESIAN_POINT('Ctrl Pts',(1.72827865000283,-4.99839916925953,33.0946455653539));
#43996=CARTESIAN_POINT('Ctrl Pts',(3.9084683581323,-3.5629785911213,33.1740174554073));
#43997=CARTESIAN_POINT('Ctrl Pts',(4.92459807825024,-1.65717664129123,33.2396899854103));
#43998=CARTESIAN_POINT('Ctrl Pts',(5.07320656921722,-0.406807195031642,
33.2789052187288));
#43999=CARTESIAN_POINT('Ctrl Pts',(5.07316757009266,-1.39624117367898E-5,
33.2916631553629));
#44000=CARTESIAN_POINT('Ctrl Pts',(5.07365497060222,0.000129255909635077,
32.208336844637));
#44001=CARTESIAN_POINT('Ctrl Pts',(5.07383759281576,0.177050513766622,32.2138870169853));
#44002=CARTESIAN_POINT('Ctrl Pts',(5.02150924629178,1.19723596214486,32.2458944860181));
#44003=CARTESIAN_POINT('Ctrl Pts',(4.35504064192764,3.00076029606972,32.3043592517354));
#44004=CARTESIAN_POINT('Ctrl Pts',(2.3893631891323,4.71825019448202,32.3837311417886));
#44005=CARTESIAN_POINT('Ctrl Pts',(-0.158357847769981,5.28638478918814,
32.4631030318421));
#44006=CARTESIAN_POINT('Ctrl Pts',(-2.66750326347463,4.56676775046226,32.5424749218955));
#44007=CARTESIAN_POINT('Ctrl Pts',(-4.52685078861515,2.73469619609277,32.6218468119489));
#44008=CARTESIAN_POINT('Ctrl Pts',(-5.28346748166331,0.23645870150246,32.7012187020024));
#44009=CARTESIAN_POINT('Ctrl Pts',(-4.75304319093522,-2.31937960938145,
32.7805905920557));
#44010=CARTESIAN_POINT('Ctrl Pts',(-3.06478809957792,-4.3102221812797,32.8599624821091));
#44011=CARTESIAN_POINT('Ctrl Pts',(-0.629957410956834,-5.25110417033318,
32.9393343721625));
#44012=CARTESIAN_POINT('Ctrl Pts',(1.95832950858626,-4.91282880661543,33.0187062622159));
#44013=CARTESIAN_POINT('Ctrl Pts',(4.06957169452659,-3.37779921996823,33.0980781522693));
#44014=CARTESIAN_POINT('Ctrl Pts',(4.96144058461863,-1.50005120370765,33.1612883464097));
#44015=CARTESIAN_POINT('Ctrl Pts',(5.07343602224469,-0.328346354394994,
33.1980412438656));
#44016=CARTESIAN_POINT('Ctrl Pts',(5.07324948390142,-8.1108973011175E-5,
33.208336844637));
#44017=CARTESIAN_POINT('Origin',(0.,0.,-2.20833684463713));
#44018=CARTESIAN_POINT('',(5.073704252564,-0.000125440355911652,31.2083368446371));
#44019=CARTESIAN_POINT('',(5.07346075270687,-0.000126888963244813,31.2916631553629));
#44020=CARTESIAN_POINT('',(5.0736,-1.85409460923845E-12,-2.20833684463713));
#44021=CARTESIAN_POINT('Ctrl Pts',(5.07346075270687,-0.000126888963244594,
31.2916631553629));
#44022=CARTESIAN_POINT('Ctrl Pts',(5.07289095298355,0.60348081698673,31.3105967649683));
#44023=CARTESIAN_POINT('Ctrl Pts',(4.81451756387892,2.05102782258644,31.3559876712581));
#44024=CARTESIAN_POINT('Ctrl Pts',(3.46819087602115,3.99281772621712,31.4278358742324));
#44025=CARTESIAN_POINT('Ctrl Pts',(1.13603804757386,5.16530336977167,31.5072077642858));
#44026=CARTESIAN_POINT('Ctrl Pts',(-1.47285113468488,5.07953254565492,31.5865796543392));
#44027=CARTESIAN_POINT('Ctrl Pts',(-3.72295704063504,3.75639883677117,31.6659515443926));
#44028=CARTESIAN_POINT('Ctrl Pts',(-5.06615885211213,1.51821468589782,31.745323434446));
#44029=CARTESIAN_POINT('Ctrl Pts',(-5.17525558096714,-1.08980320194903,
31.8246953244994));
#44030=CARTESIAN_POINT('Ctrl Pts',(-4.02367150553249,-3.43234744203962,
31.9040672145529));
#44031=CARTESIAN_POINT('Ctrl Pts',(-1.89192995759591,-4.93877944262154,
31.9834391046062));
#44032=CARTESIAN_POINT('Ctrl Pts',(0.70068154029511,-5.24213570278371,32.0628109946597));
#44033=CARTESIAN_POINT('Ctrl Pts',(3.12260856590247,-4.26851930901834,32.142182884713));
#44034=CARTESIAN_POINT('Ctrl Pts',(4.71924613978307,-2.33342987779042,32.2184669382808));
#44035=CARTESIAN_POINT('Ctrl Pts',(5.07325988110442,-0.74474986994901,32.2682936951641));
#44036=CARTESIAN_POINT('Ctrl Pts',(5.0738885135215,9.27415284240896E-5,
32.2916631553629));
#44037=CARTESIAN_POINT('Ctrl Pts',(5.073704252564,-0.000125440355911652,
31.2083368446371));
#44038=CARTESIAN_POINT('Ctrl Pts',(5.0730059773177,0.681887909050636,31.2297327901051));
#44039=CARTESIAN_POINT('Ctrl Pts',(4.76334894417968,2.20786416800771,31.2775860322575));
#44040=CARTESIAN_POINT('Ctrl Pts',(3.27920000412114,4.14943233229341,31.3518965710945));
#44041=CARTESIAN_POINT('Ctrl Pts',(0.895158610487983,5.21244975125701,31.4312684611478));
#44042=CARTESIAN_POINT('Ctrl Pts',(-1.70694143926006,5.00572594837619,31.5106403512013));
#44043=CARTESIAN_POINT('Ctrl Pts',(-3.89323433265515,3.57961838445739,31.5900122412546));
#44044=CARTESIAN_POINT('Ctrl Pts',(-5.13114396014345,1.28152370543563,31.6693841313081));
#44045=CARTESIAN_POINT('Ctrl Pts',(-5.11911827653528,-1.32874731162563,
31.7487560213615));
#44046=CARTESIAN_POINT('Ctrl Pts',(-3.86008671173927,-3.61533842470713,
31.8281279114149));
#44047=CARTESIAN_POINT('Ctrl Pts',(-1.6607465681206,-5.02124109994587,31.9074998014683));
#44048=CARTESIAN_POINT('Ctrl Pts',(0.943147763492109,-5.20398055756647,
31.9868716915216));
#44049=CARTESIAN_POINT('Ctrl Pts',(3.31729338754031,-4.11904187017945,32.0662435815751));
#44050=CARTESIAN_POINT('Ctrl Pts',(4.77384508508688,-2.17674249303873,32.1400652992802));
#44051=CARTESIAN_POINT('Ctrl Pts',(5.07296704505946,-0.666321171863868,
32.1874297203008));
#44052=CARTESIAN_POINT('Ctrl Pts',(5.07365497060222,0.000129255909635077,
32.208336844637));
#44053=CARTESIAN_POINT('Origin',(0.,0.,-2.20833684463713));
#44054=CARTESIAN_POINT('',(5.0732242396654,6.91156314036601E-5,30.208336844637));
#44055=CARTESIAN_POINT('',(5.07338983982448,0.000118254562807938,30.2916631553629));
#44056=CARTESIAN_POINT('',(5.0736,-1.85409460923845E-12,-2.20833684463713));
#44057=CARTESIAN_POINT('Ctrl Pts',(5.07338983982448,0.000118254562808118,
30.2916631553629));
#44058=CARTESIAN_POINT('Ctrl Pts',(5.07361825292341,0.265438860321299,30.2999852414035));
#44059=CARTESIAN_POINT('Ctrl Pts',(4.98815112489718,1.37411209267241,30.3347646241286));
#44060=CARTESIAN_POINT('Ctrl Pts',(4.19238095442003,3.22410968801099,30.3960013035382));
#44061=CARTESIAN_POINT('Ctrl Pts',(2.13968914249988,4.83659712202475,30.4753731935916));
#44062=CARTESIAN_POINT('Ctrl Pts',(-0.434226208411599,5.27090020273941,
30.554745083645));
#44063=CARTESIAN_POINT('Ctrl Pts',(-2.90236501609743,4.4212236610065,30.6341169736984));
#44064=CARTESIAN_POINT('Ctrl Pts',(-4.66349413013793,2.49454682166501,30.7134888637518));
#44065=CARTESIAN_POINT('Ctrl Pts',(-5.28860639654603,-0.0397961018483339,
30.7928607538052));
#44066=CARTESIAN_POINT('Ctrl Pts',(-4.62542585088724,-2.56444478303865,
30.8722326438586));
#44067=CARTESIAN_POINT('Ctrl Pts',(-2.83550180615875,-4.46440039138299,
30.951604533912));
#44068=CARTESIAN_POINT('Ctrl Pts',(-0.354855797726762,-5.27683794616905,
31.0309764239654));
#44069=CARTESIAN_POINT('Ctrl Pts',(2.21223229757146,-4.80384945735102,31.1103483140188));
#44070=CARTESIAN_POINT('Ctrl Pts',(4.24042550187443,-3.16065387386267,31.1897202040722));
#44071=CARTESIAN_POINT('Ctrl Pts',(4.99825410162456,-1.32316383571886,31.2501584845202));
#44072=CARTESIAN_POINT('Ctrl Pts',(5.07368717518548,-0.239983714616348,
31.2841394682838));
#44073=CARTESIAN_POINT('Ctrl Pts',(5.07346075270687,-0.000126888963244594,
31.2916631553629));
#44074=CARTESIAN_POINT('Ctrl Pts',(5.0732242396654,6.91156314035213E-5,
30.208336844637));
#44075=CARTESIAN_POINT('Ctrl Pts',(5.07338968774506,0.343924846945636,30.2191212665403));
#44076=CARTESIAN_POINT('Ctrl Pts',(4.95443916911164,1.53124494231641,30.256362985128));
#44077=CARTESIAN_POINT('Ctrl Pts',(4.0382761360698,3.41515258753676,30.3200620004003));
#44078=CARTESIAN_POINT('Ctrl Pts',(1.91297991407722,4.93066417388641,30.3994338904535));
#44079=CARTESIAN_POINT('Ctrl Pts',(-0.678313980675348,5.24507688131741,
30.4788057805071));
#44080=CARTESIAN_POINT('Ctrl Pts',(-3.10437209115798,4.28180047024023,30.5581776705604));
#44081=CARTESIAN_POINT('Ctrl Pts',(-4.77421203164559,2.2754869422171,30.6375495606138));
#44082=CARTESIAN_POINT('Ctrl Pts',(-5.28106448876339,-0.285130168225216,
30.7169214506672));
#44083=CARTESIAN_POINT('Ctrl Pts',(-4.50146132585641,-2.77629020081278,
30.7962933407206));
#44084=CARTESIAN_POINT('Ctrl Pts',(-2.62531214778642,-4.59115208569648,
30.8756652307741));
#44085=CARTESIAN_POINT('Ctrl Pts',(-0.109642741545517,-5.28761948484725,
30.9550371208274));
#44086=CARTESIAN_POINT('Ctrl Pts',(2.43273539384572,-4.69603448143646,31.0344090108809));
#44087=CARTESIAN_POINT('Ctrl Pts',(4.38250457206463,-2.96050587284378,31.1137809009342));
#44088=CARTESIAN_POINT('Ctrl Pts',(5.02689419953704,-1.16604718553494,31.1717568455196));
#44089=CARTESIAN_POINT('Ctrl Pts',(5.07386943415284,-0.161460170846308,
31.2032754934206));
#44090=CARTESIAN_POINT('Ctrl Pts',(5.073704252564,-0.000125440355911652,
31.2083368446371));
#44091=CARTESIAN_POINT('Origin',(0.,0.,-2.20833684463713));
#44092=CARTESIAN_POINT('',(5.07403430731529,5.85510781675173E-6,29.2083368446371));
#44093=CARTESIAN_POINT('',(5.07394886825829,-7.2464216758803E-5,29.2916631553629));
#44094=CARTESIAN_POINT('',(5.0736,-1.85409460923845E-12,-2.20833684463713));
#44095=CARTESIAN_POINT('Ctrl Pts',(5.07394886825829,-7.24642167588933E-5,
29.2916631553629));
#44096=CARTESIAN_POINT('Ctrl Pts',(5.07341208948874,0.770190548650157,29.3158310145232));
#44097=CARTESIAN_POINT('Ctrl Pts',(4.70060969038705,2.3841859592787,29.3664561703681));
#44098=CARTESIAN_POINT('Ctrl Pts',(3.05801844753361,4.31502775447088,29.4435386228973));
#44099=CARTESIAN_POINT('Ctrl Pts',(0.621713829942241,5.25208656259286,29.5229105129507));
#44100=CARTESIAN_POINT('Ctrl Pts',(-1.96603890048284,4.90974870936366,29.6022824030042));
#44101=CARTESIAN_POINT('Ctrl Pts',(-4.07486890650364,3.37140693807791,29.6816542930575));
#44102=CARTESIAN_POINT('Ctrl Pts',(-5.19106986646947,1.01179789915904,29.7610261831109));
#44103=CARTESIAN_POINT('Ctrl Pts',(-5.04273769720158,-1.59428286841832,
29.8403980731643));
#44104=CARTESIAN_POINT('Ctrl Pts',(-3.66600578680595,-3.81199985813419,
29.9197699632177));
#44105=CARTESIAN_POINT('Ctrl Pts',(-1.39624298131062,-5.10112212012718,
29.9991418532712));
#44106=CARTESIAN_POINT('Ctrl Pts',(1.21364152390063,-5.1476223247995,30.0785137433246));
#44107=CARTESIAN_POINT('Ctrl Pts',(3.52788564023963,-3.94017312521939,30.157885633378));
#44108=CARTESIAN_POINT('Ctrl Pts',(4.83020369710336,-2.00014283583164,30.2289354373907));
#44109=CARTESIAN_POINT('Ctrl Pts',(5.07289208966392,-0.578059506409542,
30.2735279447191));
#44110=CARTESIAN_POINT('Ctrl Pts',(5.07338983982448,0.000118254562808118,
30.2916631553629));
#44111=CARTESIAN_POINT('Ctrl Pts',(5.07403400238361,5.85099688312179E-6,
29.2083368446371));
#44112=CARTESIAN_POINT('Ctrl Pts',(5.07403437680669,0.00551609080175396,
29.2085097429756));
#44113=CARTESIAN_POINT('Ctrl Pts',(5.07268078911905,0.854215563279166,29.2351399379985));
#44114=CARTESIAN_POINT('Ctrl Pts',(4.6363228263275,2.54469094339263,29.2882274297059));
#44115=CARTESIAN_POINT('Ctrl Pts',(2.85451963682592,4.45226447892365,29.3675993197594));
#44116=CARTESIAN_POINT('Ctrl Pts',(0.377361782165573,5.2752762423091,29.4469712098127));
#44117=CARTESIAN_POINT('Ctrl Pts',(-2.19172056735417,4.81324238969394,29.5263430998662));
#44118=CARTESIAN_POINT('Ctrl Pts',(-4.22690463795758,3.17871334488069,29.6057149899195));
#44119=CARTESIAN_POINT('Ctrl Pts',(-5.23242409484928,0.769856765217166,
29.6850868799731));
#44120=CARTESIAN_POINT('Ctrl Pts',(-4.96333662400999,-1.82653521840426,
29.7644587700263));
#44121=CARTESIAN_POINT('Ctrl Pts',(-3.48519133772112,-3.97798726578954,
29.8438306600798));
#44122=CARTESIAN_POINT('Ctrl Pts',(-1.15806115590354,-5.16041042035391,
29.9232025501331));
#44123=CARTESIAN_POINT('Ctrl Pts',(1.45117016016719,-5.08576901889481,30.0025744401866));
#44124=CARTESIAN_POINT('Ctrl Pts',(3.70689963733188,-3.77224554159173,30.08194633024));
#44125=CARTESIAN_POINT('Ctrl Pts',(4.87583741971579,-1.84313681714053,30.1505337983901));
#44126=CARTESIAN_POINT('Ctrl Pts',(5.07298379589765,-0.499652414928338,
30.1926639698558));
#44127=CARTESIAN_POINT('Ctrl Pts',(5.0732242396654,6.91156314035213E-5,
30.208336844637));
#44128=CARTESIAN_POINT('Origin',(0.,0.,-2.20833684463713));
#44129=CARTESIAN_POINT('',(5.07324166632265,-7.76939179139569E-5,28.2083368446371));
#44130=CARTESIAN_POINT('',(5.07316594158954,-9.7399319174236E-6,28.2916631553629));
#44131=CARTESIAN_POINT('',(5.0736,-1.85409460923845E-12,-2.20833684463713));
#44132=CARTESIAN_POINT('Ctrl Pts',(5.0731664254358,-9.72907478691276E-6,
28.2916631553629));
#44133=CARTESIAN_POINT('Ctrl Pts',(5.07313755787372,0.432241135355033,28.3052194909585));
#44134=CARTESIAN_POINT('Ctrl Pts',(4.91180237168408,1.70811792520993,28.3452331232385));
#44135=CARTESIAN_POINT('Ctrl Pts',(3.85440685831077,3.62139325645763,28.4117040522031));
#44136=CARTESIAN_POINT('Ctrl Pts',(1.6528625396316,5.02384183393471,28.4910759422564));
#44137=CARTESIAN_POINT('Ctrl Pts',(-0.951315435152638,5.20249366075061,
28.5704478323099));
#44138=CARTESIAN_POINT('Ctrl Pts',(-3.32375507563475,4.11382954733206,28.6498197223633));
#44139=CARTESIAN_POINT('Ctrl Pts',(-4.8865353366993,2.02304566199065,28.7291916124167));
#44140=CARTESIAN_POINT('Ctrl Pts',(-5.25896640590637,-0.560547668676075,
28.8085635024701));
#44141=CARTESIAN_POINT('Ctrl Pts',(-4.35032489915935,-3.00759282800452,
28.8879353925235));
#44142=CARTESIAN_POINT('Ctrl Pts',(-2.38195387625792,-4.72199503162487,
28.9673072825769));
#44143=CARTESIAN_POINT('Ctrl Pts',(0.166655838534471,-5.28612969750008,
29.0466791726303));
#44144=CARTESIAN_POINT('Ctrl Pts',(2.67466855994625,-4.56257486971391,29.1260510626837));
#44145=CARTESIAN_POINT('Ctrl Pts',(4.53113794043359,-2.72758690275364,29.2054229527372));
#44146=CARTESIAN_POINT('Ctrl Pts',(5.05464511995301,-0.989211078787786,
29.2606269836302));
#44147=CARTESIAN_POINT('Ctrl Pts',(5.07399971767151,-0.0730399965665694,
29.2893737178388));
#44148=CARTESIAN_POINT('Ctrl Pts',(5.07394886825829,-7.24642167588933E-5,
29.2916631553629));
#44149=CARTESIAN_POINT('Ctrl Pts',(5.07324166632265,-7.76939179139916E-5,
28.2083368446371));
#44150=CARTESIAN_POINT('Ctrl Pts',(5.07296420662618,0.510664363139913,28.2243555160953));
#44151=CARTESIAN_POINT('Ctrl Pts',(4.86967684263928,1.86519135610718,28.266831484238));
#44152=CARTESIAN_POINT('Ctrl Pts',(3.68223314068176,3.79632723101881,28.3357647490651));
#44153=CARTESIAN_POINT('Ctrl Pts',(1.41798994671214,5.09511980804509,28.4151366391186));
#44154=CARTESIAN_POINT('Ctrl Pts',(-1.19167245960906,5.15275247768794,28.4945085291719));
#44155=CARTESIAN_POINT('Ctrl Pts',(-3.51104609249168,3.9551860491902,28.5738804192253));
#44156=CARTESIAN_POINT('Ctrl Pts',(-4.97513666881207,1.79414505376557,28.6532523092787));
#44157=CARTESIAN_POINT('Ctrl Pts',(-5.22729496488809,-0.803945705483672,
28.7326241993322));
#44158=CARTESIAN_POINT('Ctrl Pts',(-4.2060957779385,-3.20619707038074,28.8119960893855));
#44159=CARTESIAN_POINT('Ctrl Pts',(-2.16030096951815,-4.82742592572986,
28.891367979439));
#44160=CARTESIAN_POINT('Ctrl Pts',(0.41173837333167,-5.27270451089724,28.9707398694923));
#44161=CARTESIAN_POINT('Ctrl Pts',(2.88347915980534,-4.43356394814356,29.0501117595458));
#44162=CARTESIAN_POINT('Ctrl Pts',(4.64895661344711,-2.51859756056696,29.1293107512606));
#44163=CARTESIAN_POINT('Ctrl Pts',(5.07397708173548,-0.837673326665985,
29.1820524462911));
#44164=CARTESIAN_POINT('Ctrl Pts',(5.07403400238361,5.85099688312179E-6,
29.2083368446371));
#44165=CARTESIAN_POINT('Origin',(0.,0.,-2.20833684463713));
#44166=CARTESIAN_POINT('',(5.07366942975965,0.000128322057781627,27.2083368446371));
#44167=CARTESIAN_POINT('',(5.07390014538872,8.93747992460227E-5,27.2916631553629));
#44168=CARTESIAN_POINT('',(5.0736,-1.85409460923845E-12,-2.20833684463713));
#44169=CARTESIAN_POINT('Ctrl Pts',(5.07390014538872,8.93747992459192E-5,
27.2916631553629));
#44170=CARTESIAN_POINT('Ctrl Pts',(5.07397720165276,0.0939472090868575,
27.2946079673937));
#44171=CARTESIAN_POINT('Ctrl Pts',(5.04850897709501,1.03101725778952,27.324010076109));
#44172=CARTESIAN_POINT('Ctrl Pts',(4.49709775967288,2.7833528499375,27.3798694815089));
#44173=CARTESIAN_POINT('Ctrl Pts',(2.61810205366886,4.59526745509821,27.4592413715622));
#44174=CARTESIAN_POINT('Ctrl Pts',(0.101342482461748,5.28778507964899,27.5386132616156));
#44175=CARTESIAN_POINT('Ctrl Pts',(-2.44010389315526,4.69220996311103,27.617985151669));
#44176=CARTESIAN_POINT('Ctrl Pts',(-4.38714636147802,2.95362288558985,27.6973570417224));
#44177=CARTESIAN_POINT('Ctrl Pts',(-5.26548968692851,0.495539810872365,
27.7767289317758));
#44178=CARTESIAN_POINT('Ctrl Pts',(-4.86117137960698,-2.08325566491491,
27.8561008218293));
#44179=CARTESIAN_POINT('Ctrl Pts',(-3.27268248423349,-4.15457467193712,
27.9354727118826));
#44180=CARTESIAN_POINT('Ctrl Pts',(-0.886975379660524,-5.21384848487045,
28.0148446019361));
#44181=CARTESIAN_POINT('Ctrl Pts',(1.71479696411104,-5.00304034754724,28.0942164919895));
#44182=CARTESIAN_POINT('Ctrl Pts',(3.89884856306386,-3.57350265560346,28.1735883820429));
#44183=CARTESIAN_POINT('Ctrl Pts',(4.92233667869786,-1.66630250443567,28.2394039365007));
#44184=CARTESIAN_POINT('Ctrl Pts',(5.07319389740952,-0.411363633920409,
28.278762194274));
#44185=CARTESIAN_POINT('Ctrl Pts',(5.0731664254358,-9.72907478691276E-6,
28.2916631553629));
#44186=CARTESIAN_POINT('Ctrl Pts',(5.07366942975965,0.000128322057781714,
27.2083368446371));
#44187=CARTESIAN_POINT('Ctrl Pts',(5.07384715626772,0.172489015223486,27.2137439925305));
#44188=CARTESIAN_POINT('Ctrl Pts',(5.02310017357893,1.18811030837938,27.2456084371085));
#44189=CARTESIAN_POINT('Ctrl Pts',(4.36311469772634,2.98900844458398,27.3039301783709));
#44190=CARTESIAN_POINT('Ctrl Pts',(2.40207464524773,4.7117914582426,27.3833020684242));
#44191=CARTESIAN_POINT('Ctrl Pts',(-0.144105473911181,5.28679250204684,
27.4626739584777));
#44192=CARTESIAN_POINT('Ctrl Pts',(-2.65518181859737,4.57394259446923,27.542045848531));
#44193=CARTESIAN_POINT('Ctrl Pts',(-4.51946174941854,2.74689039512913,27.6214177385845));
#44194=CARTESIAN_POINT('Ctrl Pts',(-5.28281080174027,0.25070177567431,27.7007896286378));
#44195=CARTESIAN_POINT('Ctrl Pts',(-4.75927883606144,-2.30655724141581,
27.7801615186913));
#44196=CARTESIAN_POINT('Ctrl Pts',(-3.07639708040302,-4.30194401997489,
27.8595334087447));
#44197=CARTESIAN_POINT('Ctrl Pts',(-0.644111805447875,-5.24938675745965,
27.9389052987981));
#44198=CARTESIAN_POINT('Ctrl Pts',(1.94507767959709,-4.91809050014772,28.0182771888515));
#44199=CARTESIAN_POINT('Ctrl Pts',(4.06045054724861,-3.38875828300845,28.0976490789049));
#44200=CARTESIAN_POINT('Ctrl Pts',(4.95940796121397,-1.50917823199387,28.1610022975001));
#44201=CARTESIAN_POINT('Ctrl Pts',(5.07342247393797,-0.332904603741066,
28.1978982194108));
#44202=CARTESIAN_POINT('Ctrl Pts',(5.07324166632265,-7.76939179139916E-5,
28.2083368446371));
#44203=CARTESIAN_POINT('Origin',(0.,0.,-2.20833684463713));
#44204=CARTESIAN_POINT('',(5.07368988190431,-0.000126739092140837,26.2083368446371));
#44205=CARTESIAN_POINT('',(5.07344758812249,-0.000125648970980255,26.2916631553629));
#44206=CARTESIAN_POINT('',(5.0736,-1.85409460923845E-12,-2.20833684463713));
#44207=CARTESIAN_POINT('Ctrl Pts',(5.07344758812249,-0.000125648970980205,
26.2916631553629));
#44208=CARTESIAN_POINT('Ctrl Pts',(5.0728899391017,0.598926868258771,26.3104537405135));
#44209=CARTESIAN_POINT('Ctrl Pts',(4.81735989282913,2.0419133290656,26.3557016223485));
#44210=CARTESIAN_POINT('Ctrl Pts',(3.47894268615705,3.98345316700778,26.427406800868));
#44211=CARTESIAN_POINT('Ctrl Pts',(1.14995928876529,5.16222190355009,26.5067786909214));
#44212=CARTESIAN_POINT('Ctrl Pts',(-1.45915164597797,5.08348481077201,26.5861505809748));
#44213=CARTESIAN_POINT('Ctrl Pts',(-3.71281646953845,3.76642207019263,26.6655224710282));
#44214=CARTESIAN_POINT('Ctrl Pts',(-5.06204741929919,1.53186725014815,26.7448943610816));
#44215=CARTESIAN_POINT('Ctrl Pts',(-5.17817482237054,-1.07584704130177,
26.824266251135));
#44216=CARTESIAN_POINT('Ctrl Pts',(-4.032910300408,-3.42148737483758,26.9036381411884));
#44217=CARTESIAN_POINT('Ctrl Pts',(-1.90523775596165,-4.93366095719681,
26.9830100312419));
#44218=CARTESIAN_POINT('Ctrl Pts',(0.686546488664775,-5.24400565085624,
27.0623819212952));
#44219=CARTESIAN_POINT('Ctrl Pts',(3.11108952829732,-4.27692217537667,27.1417538113486));
#44220=CARTESIAN_POINT('Ctrl Pts',(4.71594148821095,-2.34252421969056,27.2181808893712));
#44221=CARTESIAN_POINT('Ctrl Pts',(5.07328489925194,-0.749306805737992,
27.2681506707093));
#44222=CARTESIAN_POINT('Ctrl Pts',(5.07390014538872,8.93747992459192E-5,
27.2916631553629));
#44223=CARTESIAN_POINT('Ctrl Pts',(5.07368988190431,-0.000126739092140768,
26.2083368446371));
#44224=CARTESIAN_POINT('Ctrl Pts',(5.07299367900981,0.677333119387493,26.2295897656503));
#44225=CARTESIAN_POINT('Ctrl Pts',(4.76643747661854,2.19875901809265,26.2772999833479));
#44226=CARTESIAN_POINT('Ctrl Pts',(3.29037472529985,4.14057671278022,26.35146749773));
#44227=CARTESIAN_POINT('Ctrl Pts',(0.909207831064193,5.21001751122215,26.4308393877834));
#44228=CARTESIAN_POINT('Ctrl Pts',(-1.69344007832135,5.01030957610855,26.5102112778369));
#44229=CARTESIAN_POINT('Ctrl Pts',(-3.88356973299385,3.59010131838702,26.5895831678902));
#44230=CARTESIAN_POINT('Ctrl Pts',(-5.12767039684481,1.29535232606086,26.6689550579437));
#44231=CARTESIAN_POINT('Ctrl Pts',(-5.12268190193029,-1.31494162567991,
26.748326947997));
#44232=CARTESIAN_POINT('Ctrl Pts',(-3.86981943456965,-3.604918707979,26.8276988380504));
#44233=CARTESIAN_POINT('Ctrl Pts',(-1.67427751864785,-5.01674557236666,
26.9070707281038));
#44234=CARTESIAN_POINT('Ctrl Pts',(0.929114694866165,-5.20650431970375,
26.9864426181573));
#44235=CARTESIAN_POINT('Ctrl Pts',(3.30617662527125,-4.12797013916282,27.0658145082107));
#44236=CARTESIAN_POINT('Ctrl Pts',(4.77079146294434,-2.18584915384965,27.1397792503706));
#44237=CARTESIAN_POINT('Ctrl Pts',(5.07297753645236,-0.6708757466937,27.1872866958461));
#44238=CARTESIAN_POINT('Ctrl Pts',(5.07366942975965,0.000128322057781714,
27.2083368446371));
#44239=CARTESIAN_POINT('Origin',(0.,0.,-2.20833684463713));
#44240=CARTESIAN_POINT('',(5.07323119136609,7.27167192501876E-5,25.2083368446371));
#44241=CARTESIAN_POINT('',(5.07340205215522,0.00012010210694157,25.2916631553629));
#44242=CARTESIAN_POINT('',(5.0736,-1.85409460923845E-12,-2.20833684463713));
#44243=CARTESIAN_POINT('Ctrl Pts',(5.07340205215522,0.000120102106941772,
25.2916631553629));
#44244=CARTESIAN_POINT('Ctrl Pts',(5.07363086957761,0.260879072720769,25.2998422169487));
#44245=CARTESIAN_POINT('Ctrl Pts',(4.98999058102238,1.36498517337352,25.334478575219));
#44246=CARTESIAN_POINT('Ctrl Pts',(4.20105773883081,3.21279554629917,25.3955722301737));
#44247=CARTESIAN_POINT('Ctrl Pts',(2.15272056265901,4.83081106300121,25.4749441202272));
#44248=CARTESIAN_POINT('Ctrl Pts',(-0.420014577610356,5.27205169757513,
25.5543160102805));
#44249=CARTESIAN_POINT('Ctrl Pts',(-2.89043509646038,4.42903220810823,25.6336879003339));
#44250=CARTESIAN_POINT('Ctrl Pts',(-4.65675202368223,2.50711027624266,25.7130597903873));
#44251=CARTESIAN_POINT('Ctrl Pts',(-5.28869446548081,-0.0255381695211706,
25.7924316804408));
#44252=CARTESIAN_POINT('Ctrl Pts',(-4.63232264181493,-2.55196557371741,
25.8718035704942));
#44253=CARTESIAN_POINT('Ctrl Pts',(-2.84752727607513,-4.45673981283608,
25.9511754605475));
#44254=CARTESIAN_POINT('Ctrl Pts',(-0.369080568778156,-5.27586209837409,
26.030547350601));
#44255=CARTESIAN_POINT('Ctrl Pts',(2.19927334812716,-4.80979605467087,26.1099192406543));
#44256=CARTESIAN_POINT('Ctrl Pts',(4.23188914543768,-3.17207433835284,26.1892911307078));
#44257=CARTESIAN_POINT('Ctrl Pts',(4.99647384522203,-1.33229055500106,26.2498724356106));
#44258=CARTESIAN_POINT('Ctrl Pts',(5.0736751134574,-0.244543947095586,26.283996443829));
#44259=CARTESIAN_POINT('Ctrl Pts',(5.07344758812249,-0.000125648970980205,
26.2916631553629));
#44260=CARTESIAN_POINT('Ctrl Pts',(5.07323119136609,7.2716719250257E-5,
25.2083368446371));
#44261=CARTESIAN_POINT('Ctrl Pts',(5.07340324942578,0.339366856221997,25.2189782420855));
#44262=CARTESIAN_POINT('Ctrl Pts',(4.95650365046512,1.52211798561692,25.2560769362184));
#44263=CARTESIAN_POINT('Ctrl Pts',(4.04746852150308,3.40425320955296,25.3196329270358));
#44264=CARTESIAN_POINT('Ctrl Pts',(1.92626575763449,4.92548896844514,25.3990048170892));
#44265=CARTESIAN_POINT('Ctrl Pts',(-0.664171081076968,5.24688651700902,
25.4783767071426));
#44266=CARTESIAN_POINT('Ctrl Pts',(-3.09281731455583,4.2901541238158,25.5577485971959));
#44267=CARTESIAN_POINT('Ctrl Pts',(-4.76806009604388,2.2883496821561,25.6371204872494));
#44268=CARTESIAN_POINT('Ctrl Pts',(-5.28181399205765,-0.2708916769007,25.7164923773028));
#44269=CARTESIAN_POINT('Ctrl Pts',(-4.50892969070311,-2.76414442307307,
25.7958642673562));
#44270=CARTESIAN_POINT('Ctrl Pts',(-2.63768009703987,-4.58405770611471,
25.8752361574096));
#44271=CARTESIAN_POINT('Ctrl Pts',(-0.123897470143628,-5.28730467858643,
25.9546080474629));
#44272=CARTESIAN_POINT('Ctrl Pts',(2.42006630623721,-4.70257593460492,26.0339799375165));
#44273=CARTESIAN_POINT('Ctrl Pts',(4.37450728714461,-2.97231010192892,26.1133518275698));
#44274=CARTESIAN_POINT('Ctrl Pts',(5.02533394688967,-1.17517261458846,26.17147079661));
#44275=CARTESIAN_POINT('Ctrl Pts',(5.07386036677103,-0.166021846101412,
26.2031324689658));
#44276=CARTESIAN_POINT('Ctrl Pts',(5.07368988190431,-0.000126739092140768,
26.2083368446371));
#44277=CARTESIAN_POINT('Origin',(0.,0.,-2.20833684463713));
#44278=CARTESIAN_POINT('',(5.07403460521456,1.01146903839872E-6,24.2083368446371));
#44279=CARTESIAN_POINT('',(5.07393893245752,-7.63518475177419E-5,24.2916631553629));
#44280=CARTESIAN_POINT('',(5.0736,-1.85409460923845E-12,-2.20833684463713));
#44281=CARTESIAN_POINT('Ctrl Pts',(5.07393893245752,-7.63518475176573E-5,
24.2916631553629));
#44282=CARTESIAN_POINT('Ctrl Pts',(5.0733825372435,0.765632623134578,24.3156879900684));
#44283=CARTESIAN_POINT('Ctrl Pts',(4.70398212533016,2.37509554318665,24.3661701214584));
#44284=CARTESIAN_POINT('Ctrl Pts',(3.0696404085172,4.30676782630642,24.4431095495329));
#44285=CARTESIAN_POINT('Ctrl Pts',(0.635870902865647,5.25039137038364,24.5224814395863));
#44286=CARTESIAN_POINT('Ctrl Pts',(-1.95279534724764,4.9150311981795,24.6018533296397));
#44287=CARTESIAN_POINT('Ctrl Pts',(-4.06576497321052,3.38238030533593,24.6812252196931));
#44288=CARTESIAN_POINT('Ctrl Pts',(-5.18832325111748,1.02578905688434,24.7605971097465));
#44289=CARTESIAN_POINT('Ctrl Pts',(-5.04701746921096,-1.58068213527875,
24.8399689997999));
#44290=CARTESIAN_POINT('Ctrl Pts',(-3.67626940318832,-3.80210265806849,
24.9193408898533));
#44291=CARTESIAN_POINT('Ctrl Pts',(-1.40999024783327,-5.09733938916421,
24.9987127799067));
#44292=CARTESIAN_POINT('Ctrl Pts',(1.19975941093347,-5.1508755278289,25.0780846699601));
#44293=CARTESIAN_POINT('Ctrl Pts',(3.51725033281924,-3.94966978918403,25.1574565600135));
#44294=CARTESIAN_POINT('Ctrl Pts',(4.82742597758186,-2.00925929492118,25.2286493884811));
#44295=CARTESIAN_POINT('Ctrl Pts',(5.07289070026022,-0.582613469337955,
25.2733849202643));
#44296=CARTESIAN_POINT('Ctrl Pts',(5.07340205215522,0.000120102106941772,
25.2916631553629));
#44297=CARTESIAN_POINT('Ctrl Pts',(5.07403455984306,1.01136344364921E-6,
24.2083368446371));
#44298=CARTESIAN_POINT('Ctrl Pts',(5.07403457120051,0.000953086505682821,
24.2083667185208));
#44299=CARTESIAN_POINT('Ctrl Pts',(5.07380195086792,0.845094303182403,24.2348538890889));
#44300=CARTESIAN_POINT('Ctrl Pts',(4.64316632240633,2.53218242822061,24.2877983563415));
#44301=CARTESIAN_POINT('Ctrl Pts',(2.86651231988729,4.4445526734691,24.3671702463949));
#44302=CARTESIAN_POINT('Ctrl Pts',(0.391582261162602,5.27423972531146,24.4465421364484));
#44303=CARTESIAN_POINT('Ctrl Pts',(-2.1787363696294,4.81913365439931,24.5259140265017));
#44304=CARTESIAN_POINT('Ctrl Pts',(-4.21831964333045,3.19009729224708,24.6052859165552));
#44305=CARTESIAN_POINT('Ctrl Pts',(-5.23032958900859,0.783960290863936,
24.6846578066085));
#44306=CARTESIAN_POINT('Ctrl Pts',(-4.9682428239423,-1.81314770210696,24.764029696662));
#44307=CARTESIAN_POINT('Ctrl Pts',(-3.49590310398264,-3.96857692817898,
24.8434015867153));
#44308=CARTESIAN_POINT('Ctrl Pts',(-1.17196912594307,-5.15726959884261,
24.9227734767688));
#44309=CARTESIAN_POINT('Ctrl Pts',(1.43745393706658,-5.08966281065081,25.0021453668222));
#44310=CARTESIAN_POINT('Ctrl Pts',(3.69671640275713,-3.78222542756197,25.0815172568756));
#44311=CARTESIAN_POINT('Ctrl Pts',(4.87329911188321,-1.85225894830422,25.1502477494805));
#44312=CARTESIAN_POINT('Ctrl Pts',(5.07297546809779,-0.504207096881882,
25.192520945401));
#44313=CARTESIAN_POINT('Ctrl Pts',(5.07323119136609,7.2716719250257E-5,
25.2083368446371));
#44314=CARTESIAN_POINT('Origin',(0.,0.,-2.20833684463713));
#44315=CARTESIAN_POINT('',(5.07323420419449,-7.41988534934401E-5,23.2083368446371));
#44316=CARTESIAN_POINT('',(5.07316553675605,-5.48786176412603E-6,23.2916631553629));
#44317=CARTESIAN_POINT('',(5.0736,-1.85409460923845E-12,-2.20833684463713));
#44318=CARTESIAN_POINT('Ctrl Pts',(5.07316569050492,-5.48591970746248E-6,
23.2916631553629));
#44319=CARTESIAN_POINT('Ctrl Pts',(5.07314958741115,0.42768514602335,23.3050764665037));
#44320=CARTESIAN_POINT('Ctrl Pts',(4.91412543793041,1.69899265595715,23.344947074329));
#44321=CARTESIAN_POINT('Ctrl Pts',(3.86415592530766,3.6109888303426,23.4112749788386));
#44322=CARTESIAN_POINT('Ctrl Pts',(1.66640053022393,5.01936755177924,23.4906468688921));
#44323=CARTESIAN_POINT('Ctrl Pts',(-0.937286345425383,5.20503944789203,
23.5700187589454));
#44324=CARTESIAN_POINT('Ctrl Pts',(-3.31265234202061,4.12277525560054,23.6493906489989));
#44325=CARTESIAN_POINT('Ctrl Pts',(-4.88106356050821,2.03621213668325,23.7287625390522));
#44326=CARTESIAN_POINT('Ctrl Pts',(-5.26045849971908,-0.546367751667005,
23.8081344291057));
#44327=CARTESIAN_POINT('Ctrl Pts',(-4.35841739221935,-2.99585366506712,
23.887506319159));
#44328=CARTESIAN_POINT('Ctrl Pts',(-2.3946754551717,-4.71555625687105,23.9668782092125));
#44329=CARTESIAN_POINT('Ctrl Pts',(0.152404122233421,-5.28655978220554,
24.0462500992659));
#44330=CARTESIAN_POINT('Ctrl Pts',(2.66235839280233,-4.56976904619763,24.1256219893193));
#44331=CARTESIAN_POINT('Ctrl Pts',(4.52376805191542,-2.73979268554746,24.2049938793727));
#44332=CARTESIAN_POINT('Ctrl Pts',(5.05332835032277,-0.998334355631039,
24.2603409347206));
#44333=CARTESIAN_POINT('Ctrl Pts',(5.07399526625627,-0.0776027111923523,
24.289230693384));
#44334=CARTESIAN_POINT('Ctrl Pts',(5.07393893245752,-7.63518475176573E-5,
24.2916631553629));
#44335=CARTESIAN_POINT('Ctrl Pts',(5.07323420419449,-7.41988534933707E-5,
23.2083368446371));
#44336=CARTESIAN_POINT('Ctrl Pts',(5.07297208311489,0.506109773689648,23.2242124916405));
#44337=CARTESIAN_POINT('Ctrl Pts',(4.87223466883649,1.85606959653113,23.2665454353283));
#44338=CARTESIAN_POINT('Ctrl Pts',(3.69245444696201,3.78638634033052,23.3353356757007));
#44339=CARTESIAN_POINT('Ctrl Pts',(1.43172095156667,5.09127847004479,23.4147075657541));
#44340=CARTESIAN_POINT('Ctrl Pts',(-1.17777659548102,5.1559464348325,23.4940794558075));
#44341=CARTESIAN_POINT('Ctrl Pts',(-3.50037037246962,3.96463726004727,23.5734513458609));
#44342=CARTESIAN_POINT('Ctrl Pts',(-4.97028167379665,1.80755122457705,23.6528232359143));
#44343=CARTESIAN_POINT('Ctrl Pts',(-5.22944336137752,-0.789850288405212,
23.7321951259677));
#44344=CARTESIAN_POINT('Ctrl Pts',(-4.21472422106041,-3.19484601935549,
23.8115670160211));
#44345=CARTESIAN_POINT('Ctrl Pts',(-2.17330758975551,-4.82158433170509,
23.8909389060745));
#44346=CARTESIAN_POINT('Ctrl Pts',(0.397521959947206,-5.27379537322471,
23.9703107961279));
#44347=CARTESIAN_POINT('Ctrl Pts',(2.87151604007067,-4.4413215351868,24.0496826861813));
#44348=CARTESIAN_POINT('Ctrl Pts',(4.64534728528402,-2.52767212981305,24.129024702351));
#44349=CARTESIAN_POINT('Ctrl Pts',(5.07402451266825,-0.842236060605585,
24.1819094218363));
#44350=CARTESIAN_POINT('Ctrl Pts',(5.07403455984306,1.01136344364921E-6,
24.2083368446371));
#44351=CARTESIAN_POINT('Origin',(0.,0.,-2.20833684463713));
#44352=CARTESIAN_POINT('',(5.07368445537635,0.000127432987209741,22.2083368446371));
#44353=CARTESIAN_POINT('',(5.0739114897015,8.59482686052055E-5,22.2916631553629));
#44354=CARTESIAN_POINT('',(5.0736,-1.85409460923845E-12,-2.20833684463713));
#44355=CARTESIAN_POINT('Ctrl Pts',(5.0739114897015,8.59482686050433E-5,
22.2916631553629));
#44356=CARTESIAN_POINT('Ctrl Pts',(5.07398263122595,0.0893847065795861,
22.2944649429389));
#44357=CARTESIAN_POINT('Ctrl Pts',(5.04987059102411,1.02189374093949,22.3237240271994));
#44358=CARTESIAN_POINT('Ctrl Pts',(4.50458503707303,2.77121862106756,22.3794404081444));
#44359=CARTESIAN_POINT('Ctrl Pts',(2.63048120009391,4.58819259887664,22.4588122981978));
#44360=CARTESIAN_POINT('Ctrl Pts',(0.115597647321455,5.28749259670008,22.5381841882512));
#44361=CARTESIAN_POINT('Ctrl Pts',(-2.42744506809483,4.69877132337436,22.6175560783046));
#44362=CARTESIAN_POINT('Ctrl Pts',(-4.37916762715256,2.96543963879382,22.696927968358));
#44363=CARTESIAN_POINT('Ctrl Pts',(-5.26413459813381,0.509733484286287,
22.7762998584114));
#44364=CARTESIAN_POINT('Ctrl Pts',(-4.86677005798463,-2.07014265165558,
22.8556717484648));
#44365=CARTESIAN_POINT('Ctrl Pts',(-3.28387109087741,-4.14573660239302,
22.9350436385182));
#44366=CARTESIAN_POINT('Ctrl Pts',(-0.901028401772815,-5.21143830245831,
23.0144155285717));
#44367=CARTESIAN_POINT('Ctrl Pts',(1.70130281532621,-5.00764516247504,23.093787418625));
#44368=CARTESIAN_POINT('Ctrl Pts',(3.88920043041414,-3.58400074773866,23.1731593086785));
#44369=CARTESIAN_POINT('Ctrl Pts',(4.92006185002291,-1.67542824897262,23.239117887591));
#44370=CARTESIAN_POINT('Ctrl Pts',(5.07318135021192,-0.415919972782139,
23.2786191698192));
#44371=CARTESIAN_POINT('Ctrl Pts',(5.07316569050492,-5.48591970746248E-6,
23.2916631553629));
#44372=CARTESIAN_POINT('Ctrl Pts',(5.07368445537635,0.000127432987209863,
22.2083368446371));
#44373=CARTESIAN_POINT('Ctrl Pts',(5.07385799503573,0.167927931732477,22.2136009680757));
#44374=CARTESIAN_POINT('Ctrl Pts',(5.02468445773871,1.17898674996513,22.2453223881989));
#44375=CARTESIAN_POINT('Ctrl Pts',(4.37115162329097,2.97723307464397,22.3035011050064));
#44376=CARTESIAN_POINT('Ctrl Pts',(2.4147715124657,4.70529942618521,22.3828729950599));
#44377=CARTESIAN_POINT('Ctrl Pts',(-0.129853572474074,5.28716128664959,
22.4622448851132));
#44378=CARTESIAN_POINT('Ctrl Pts',(-2.64284027062663,4.58108446095525,22.5416167751666));
#44379=CARTESIAN_POINT('Ctrl Pts',(-4.51204028846786,2.7590644882843,22.62098866522));
#44380=CARTESIAN_POINT('Ctrl Pts',(-5.28211549991429,0.264943102456049,
22.7003605552734));
#44381=CARTESIAN_POINT('Ctrl Pts',(-4.76548000969985,-2.2937181486802,22.7797324453269));
#44382=CARTESIAN_POINT('Ctrl Pts',(-3.08798363825926,-4.29363457062517,
22.8591043353802));
#44383=CARTESIAN_POINT('Ctrl Pts',(-0.658261551986295,-5.24763120247219,
22.9384762254337));
#44384=CARTESIAN_POINT('Ctrl Pts',(1.93181173129385,-4.92331644248731,23.017848115487));
#44385=CARTESIAN_POINT('Ctrl Pts',(4.05129987868926,-3.39969271923279,23.0972200055405));
#44386=CARTESIAN_POINT('Ctrl Pts',(4.95736217363157,-1.51830523331034,23.1607162485905));
#44387=CARTESIAN_POINT('Ctrl Pts',(5.07340891666056,-0.3374627456306,23.197755194956));
#44388=CARTESIAN_POINT('Ctrl Pts',(5.07323420419449,-7.41988534933707E-5,
23.2083368446371));
#44389=CARTESIAN_POINT('Origin',(0.,0.,-2.20833684463713));
#44390=CARTESIAN_POINT('',(5.0647135783285,-0.000493560823505712,21.2083368446371));
#44391=CARTESIAN_POINT('',(5.07311795825563,-0.000541267147824199,21.2916631553629));
#44392=CARTESIAN_POINT('',(5.0736,-1.85409460923845E-12,-2.20833684463713));
#44393=CARTESIAN_POINT('Ctrl Pts',(5.07311795825563,-0.000541267147824084,
21.2916631553629));
#44394=CARTESIAN_POINT('Ctrl Pts',(5.07265472641037,0.594063927299599,21.3103107160587));
#44395=CARTESIAN_POINT('Ctrl Pts',(4.82066183061084,2.03342224951305,21.3554155734389));
#44396=CARTESIAN_POINT('Ctrl Pts',(3.48937383888172,3.97367066688458,21.4269777275036));
#44397=CARTESIAN_POINT('Ctrl Pts',(1.16402860508423,5.15930893371516,21.5063496175569));
#44398=CARTESIAN_POINT('Ctrl Pts',(-1.44552439996815,5.08729102078623,21.5857215076104));
#44399=CARTESIAN_POINT('Ctrl Pts',(-3.70260503654192,3.77647571272897,21.6650933976637));
#44400=CARTESIAN_POINT('Ctrl Pts',(-5.057922432142,1.54547807796832,21.7444652877172));
#44401=CARTESIAN_POINT('Ctrl Pts',(-5.18104412158608,-1.06186685398839,
21.8238371777705));
#44402=CARTESIAN_POINT('Ctrl Pts',(-4.04212630117128,-3.41061102326193,
21.903209067824));
#44403=CARTESIAN_POINT('Ctrl Pts',(-1.91852825506946,-4.92850206746972,
21.9825809578774));
#44404=CARTESIAN_POINT('Ctrl Pts',(0.672404619068471,-5.245839892308,22.0619528479308));
#44405=CARTESIAN_POINT('Ctrl Pts',(3.09954884704109,-4.28529268150223,22.1413247379842));
#44406=CARTESIAN_POINT('Ctrl Pts',(4.71262161876037,-2.35161833566565,22.2178948404616));
#44407=CARTESIAN_POINT('Ctrl Pts',(5.07331084138903,-0.753863997357442,
22.2680076462545));
#44408=CARTESIAN_POINT('Ctrl Pts',(5.0739114897015,8.59482686050433E-5,
22.2916631553629));
#44409=CARTESIAN_POINT('Ctrl Pts',(5.0647135783285,-0.000493560823505643,
21.2083368446371));
#44410=CARTESIAN_POINT('Ctrl Pts',(5.06741194864459,0.674127865172368,21.2294467411954));
#44411=CARTESIAN_POINT('Ctrl Pts',(4.7845254230904,2.19368980981962,21.2770139344383));
#44412=CARTESIAN_POINT('Ctrl Pts',(3.29092685490723,4.12830747359771,21.3510384243656));
#44413=CARTESIAN_POINT('Ctrl Pts',(0.929079443196039,5.20946188754723,21.430410314419));
#44414=CARTESIAN_POINT('Ctrl Pts',(-1.68303999757346,5.01382783115869,21.5097822044724));
#44415=CARTESIAN_POINT('Ctrl Pts',(-3.8722246926078,3.60110493868854,21.5891540945258));
#44416=CARTESIAN_POINT('Ctrl Pts',(-5.12503498129818,1.30888173016128,21.6685259845792));
#44417=CARTESIAN_POINT('Ctrl Pts',(-5.12574462250326,-1.300972874894,21.7478978746326));
#44418=CARTESIAN_POINT('Ctrl Pts',(-3.87976959979778,-3.59455409188016,
21.827269764686));
#44419=CARTESIAN_POINT('Ctrl Pts',(-1.68766624540451,-5.01217052435348,
21.9066416547394));
#44420=CARTESIAN_POINT('Ctrl Pts',(0.915005995631755,-5.2090130440819,21.9860135447928));
#44421=CARTESIAN_POINT('Ctrl Pts',(3.29507231119182,-4.13685632854986,22.0653854348462));
#44422=CARTESIAN_POINT('Ctrl Pts',(4.76770779675958,-2.19496036885575,22.139493201461));
#44423=CARTESIAN_POINT('Ctrl Pts',(5.07298579089609,-0.675431391209716,
22.1871436713913));
#44424=CARTESIAN_POINT('Ctrl Pts',(5.07368445537635,0.000127432987209863,
22.2083368446371));
#44425=CARTESIAN_POINT('Origin',(0.,0.,-2.20833684463713));
#44426=CARTESIAN_POINT('',(5.07022284182504,-0.00437131830465176,20.2083368446371));
#44427=CARTESIAN_POINT('',(5.07763086250027,0.00422747191343611,20.2916631553629));
#44428=CARTESIAN_POINT('',(5.0736,-1.85409460923845E-12,-2.20833684463713));
#44429=CARTESIAN_POINT('Ctrl Pts',(5.07763086250027,0.00422747191343598,
20.2916631553629));
#44430=CARTESIAN_POINT('Ctrl Pts',(5.07981016603818,0.259793667372929,20.2996991924939));
#44431=CARTESIAN_POINT('Ctrl Pts',(4.94610737387947,2.19579442888697,20.3606498229938));
#44432=CARTESIAN_POINT('Ctrl Pts',(2.45559119020176,5.46873373673919,20.4745150468627));
#44433=CARTESIAN_POINT('Ctrl Pts',(-3.26379011618977,5.03400372054189,20.6332588269695));
#44434=CARTESIAN_POINT('Ctrl Pts',(-5.99600976813329,-0.0197068834827358,
20.7920026070763));
#44435=CARTESIAN_POINT('Ctrl Pts',(-3.70230252414087,-4.19446206534972,
20.9242890904987));
#44436=CARTESIAN_POINT('Ctrl Pts',(-0.376480053418488,-5.26605971579228,
21.0301182772365));
#44437=CARTESIAN_POINT('Ctrl Pts',(2.18257651229242,-4.8205851862161,21.10949016729));
#44438=CARTESIAN_POINT('Ctrl Pts',(4.22530652207796,-3.18086119603153,21.1888620573433));
#44439=CARTESIAN_POINT('Ctrl Pts',(4.99434160286696,-1.34186431057878,21.249586386701));
#44440=CARTESIAN_POINT('Ctrl Pts',(5.07331196316984,-0.249566309185764,
21.2838534193742));
#44441=CARTESIAN_POINT('Ctrl Pts',(5.07311795825563,-0.000541267147824084,
21.2916631553629));
#44442=CARTESIAN_POINT('Ctrl Pts',(5.07022284182504,-0.00437131830465176,
20.2083368446371));
#44443=CARTESIAN_POINT('Ctrl Pts',(5.06064558604025,1.17531423721709,20.2452925143152));
#44444=CARTESIAN_POINT('Ctrl Pts',(4.06283412548092,4.05874270439873,20.3351627773622));
#44445=CARTESIAN_POINT('Ctrl Pts',(-0.73672307947618,5.95134306184733,20.4779476337782));
#44446=CARTESIAN_POINT('Ctrl Pts',(-5.3995463563661,2.60828838171381,20.6366914138849));
#44447=CARTESIAN_POINT('Ctrl Pts',(-5.1196790448508,-3.11863163173554,20.7954351939918));
#44448=CARTESIAN_POINT('Ctrl Pts',(-0.158509478954971,-5.99736559883163,
20.9541789740985));
#44449=CARTESIAN_POINT('Ctrl Pts',(4.27441519030586,-3.72585141387614,21.091812857647));
#44450=CARTESIAN_POINT('Ctrl Pts',(5.06064814629056,-1.01689503187705,21.1765321478265));
#44451=CARTESIAN_POINT('Ctrl Pts',(5.0647135783285,-0.000493560823505643,
21.2083368446371));
#44452=CARTESIAN_POINT('Origin',(0.,0.,-2.20833684463713));
#44453=CARTESIAN_POINT('',(5.08190747034449,-0.0016131106486481,19.2083368446371));
#44454=CARTESIAN_POINT('',(5.0654395261759,0.00158764291868628,19.2916631553629));
#44455=CARTESIAN_POINT('',(5.0736,-1.85409460923845E-12,-2.20833684463713));
#44456=CARTESIAN_POINT('Ctrl Pts',(5.0654395261759,0.00158764291868674,
19.2916631553629));
#44457=CARTESIAN_POINT('Ctrl Pts',(5.06734596007678,0.765537039397172,19.3155449656136));
#44458=CARTESIAN_POINT('Ctrl Pts',(4.5467586954857,3.21970245674355,19.3923413692333));
#44459=CARTESIAN_POINT('Ctrl Pts',(0.736723079475925,5.95134306184737,19.5220523662219));
#44460=CARTESIAN_POINT('Ctrl Pts',(-4.59927593805429,3.84720861430001,19.6807961463287));
#44461=CARTESIAN_POINT('Ctrl Pts',(-5.72720375155086,-1.77677009197966,
19.8395399264355));
#44462=CARTESIAN_POINT('Ctrl Pts',(-1.61419617037545,-5.77483540889735,
19.9982837065423));
#44463=CARTESIAN_POINT('Ctrl Pts',(3.69280075007907,-4.55444079317796,20.1489914495181));
#44464=CARTESIAN_POINT('Ctrl Pts',(5.0654601874783,-1.42302350869954,20.246784599125));
#44465=CARTESIAN_POINT('Ctrl Pts',(5.07763086250027,0.00422747191343598,
20.2916631553629));
#44466=CARTESIAN_POINT('Ctrl Pts',(5.08190747034449,-0.00161311064864815,
19.2083368446371));
#44467=CARTESIAN_POINT('Ctrl Pts',(5.08137262398886,1.67206424053112,19.2611382874349));
#44468=CARTESIAN_POINT('Ctrl Pts',(3.25971341308398,5.0343135906333,19.3668543236016));
#44469=CARTESIAN_POINT('Ctrl Pts',(-2.45559119020206,5.46873373673905,19.5254849531373));
#44470=CARTESIAN_POINT('Ctrl Pts',(-5.92771323046149,0.905806267444168,
19.6842287332441));
#44471=CARTESIAN_POINT('Ctrl Pts',(-3.97578039972873,-4.48936692070992,
19.8429725133509));
#44472=CARTESIAN_POINT('Ctrl Pts',(1.61419617037569,-5.77483540889728,20.0017162934577));
#44473=CARTESIAN_POINT('Ctrl Pts',(4.76969253787625,-2.70752266133374,20.1235044038864));
#44474=CARTESIAN_POINT('Ctrl Pts',(5.0743586806711,-0.513806323102652,20.1923779209462));
#44475=CARTESIAN_POINT('Ctrl Pts',(5.07022284182504,-0.00437131830465176,
20.2083368446371));
#44476=CARTESIAN_POINT('Origin',(0.,0.,-2.20833684463713));
#44477=CARTESIAN_POINT('',(5.07322996641872,-7.44046081432859E-5,18.2083368446371));
#44478=CARTESIAN_POINT('',(5.0733324096026,-5.65345686568016E-5,18.2916631553629));
#44479=CARTESIAN_POINT('',(5.0736,-1.85409460923845E-12,-2.20833684463713));
#44480=CARTESIAN_POINT('Ctrl Pts',(5.0733324096026,-5.65345686565077E-5,
18.2916631553629));
#44481=CARTESIAN_POINT('Ctrl Pts',(5.07342932055268,0.423040487316443,18.3049334420489));
#44482=CARTESIAN_POINT('Ctrl Pts',(4.9168904884294,1.68971643561363,18.3446610254193));
#44483=CARTESIAN_POINT('Ctrl Pts',(3.87222469260764,3.60110493868871,18.4108459054742));
#44484=CARTESIAN_POINT('Ctrl Pts',(1.68303999757325,5.01382783115876,18.4902177955276));
#44485=CARTESIAN_POINT('Ctrl Pts',(-0.929079443196312,5.2094618875472,18.569589685581));
#44486=CARTESIAN_POINT('Ctrl Pts',(-3.29092685490746,4.12830747359753,18.6489615756344));
#44487=CARTESIAN_POINT('Ctrl Pts',(-5.42625155540715,1.36247937795741,18.7547907623723));
#44488=CARTESIAN_POINT('Ctrl Pts',(-4.95432466322409,-3.37745298000962,
18.8870772457946));
#44489=CARTESIAN_POINT('Ctrl Pts',(0.158509478955228,-5.99736559883162,
19.0458210259014));
#44490=CARTESIAN_POINT('Ctrl Pts',(4.3733083201864,-3.5517155504766,19.1806829957575));
#44491=CARTESIAN_POINT('Ctrl Pts',(5.06312190111345,-0.927134966817506,
19.2626303722447));
#44492=CARTESIAN_POINT('Ctrl Pts',(5.0654395261759,0.00158764291868674,
19.2916631553629));
#44493=CARTESIAN_POINT('Ctrl Pts',(5.07322996641872,-7.44046081432165E-5,
18.2083368446371));
#44494=CARTESIAN_POINT('Ctrl Pts',(5.07298661447134,0.501546775803683,18.2240694671857));
#44495=CARTESIAN_POINT('Ctrl Pts',(4.87479289587003,1.8469289142109,18.2662593864187));
#44496=CARTESIAN_POINT('Ctrl Pts',(3.70260503654169,3.77647571272922,18.3349066023362));
#44497=CARTESIAN_POINT('Ctrl Pts',(1.44552439996779,5.08729102078633,18.4142784923897));
#44498=CARTESIAN_POINT('Ctrl Pts',(-1.16402860508455,5.15930893371508,18.4936503824431));
#44499=CARTESIAN_POINT('Ctrl Pts',(-3.48937383888192,3.97367066688439,18.5730222724965));
#44500=CARTESIAN_POINT('Ctrl Pts',(-4.96594823061187,1.82167865277138,18.6523941625499));
#44501=CARTESIAN_POINT('Ctrl Pts',(-5.23050112077116,-0.77713504302674,
18.7317660526033));
#44502=CARTESIAN_POINT('Ctrl Pts',(-4.22530652207786,-3.18086119603167,
18.8111379426567));
#44503=CARTESIAN_POINT('Ctrl Pts',(-2.18257651229225,-4.82058518621618,
18.8905098327101));
#44504=CARTESIAN_POINT('Ctrl Pts',(0.37648005341871,-5.26605971579227,18.9698817227635));
#44505=CARTESIAN_POINT('Ctrl Pts',(3.70230252414111,-4.19446206534953,19.0757109095013));
#44506=CARTESIAN_POINT('Ctrl Pts',(5.08048878136776,-1.68603810060634,19.1551959501259));
#44507=CARTESIAN_POINT('Ctrl Pts',(5.08190861649065,-0.00519970863047212,
19.2082236940659));
#44508=CARTESIAN_POINT('Ctrl Pts',(5.08190747034449,-0.00161311064864815,
19.2083368446371));
#44509=CARTESIAN_POINT('Origin',(0.,0.,-2.20833684463713));
#44510=CARTESIAN_POINT('',(5.07369825422177,0.000126003717071388,17.2083368446371));
#44511=CARTESIAN_POINT('',(5.07392231800261,8.23068815517256E-5,17.2916631553629));
#44512=CARTESIAN_POINT('',(5.0736,-1.85409460923845E-12,-2.20833684463713));
#44513=CARTESIAN_POINT('Ctrl Pts',(5.07392231800261,8.23068815519051E-5,
17.2916631553629));
#44514=CARTESIAN_POINT('Ctrl Pts',(5.07398762507078,0.0848220371273371,
17.2943219184842));
#44515=CARTESIAN_POINT('Ctrl Pts',(5.05121938853888,1.01276996498335,17.3234379782898));
#44516=CARTESIAN_POINT('Ctrl Pts',(4.51204028846775,2.7590644882845,17.3790113347799));
#44517=CARTESIAN_POINT('Ctrl Pts',(2.64284027062647,4.58108446095533,17.4583832248334));
#44518=CARTESIAN_POINT('Ctrl Pts',(0.129853572473924,5.28716128664959,17.5377551148867));
#44519=CARTESIAN_POINT('Ctrl Pts',(-2.41477151246584,4.70529942618515,17.6171270049402));
#44520=CARTESIAN_POINT('Ctrl Pts',(-4.37115162329109,2.9772330746438,17.6964988949936));
#44521=CARTESIAN_POINT('Ctrl Pts',(-5.2627514922539,0.523926824466488,17.775870785047));
#44522=CARTESIAN_POINT('Ctrl Pts',(-4.87231403886184,-2.05702097999283,
17.8552426751004));
#44523=CARTESIAN_POINT('Ctrl Pts',(-3.29507231119166,-4.13685632854999,
17.9346145651538));
#44524=CARTESIAN_POINT('Ctrl Pts',(-0.915005995631555,-5.20901304408194,
18.0139864552072));
#44525=CARTESIAN_POINT('Ctrl Pts',(1.68766624540468,-5.01217052435341,18.0933583452606));
#44526=CARTESIAN_POINT('Ctrl Pts',(3.8797695997979,-3.59455409188004,18.172730235314));
#44527=CARTESIAN_POINT('Ctrl Pts',(4.9174284825737,-1.68443961943593,18.2388318386815));
#44528=CARTESIAN_POINT('Ctrl Pts',(5.07323610680991,-0.420498442869185,
18.2784761453644));
#44529=CARTESIAN_POINT('Ctrl Pts',(5.0733324096026,-5.65345686565077E-5,
18.2916631553629));
#44530=CARTESIAN_POINT('Ctrl Pts',(5.07369825422177,0.000126003717071926,
17.2083368446371));
#44531=CARTESIAN_POINT('Ctrl Pts',(5.07386566986272,0.163365799600409,17.2134579436209));
#44532=CARTESIAN_POINT('Ctrl Pts',(5.02624395147431,1.16985927909857,17.2450363392892));
#44533=CARTESIAN_POINT('Ctrl Pts',(4.37916762715237,2.96543963879408,17.303072031642));
#44534=CARTESIAN_POINT('Ctrl Pts',(2.42744506809458,4.69877132337447,17.3824439216954));
#44535=CARTESIAN_POINT('Ctrl Pts',(-0.115597647321682,5.28749259670007,
17.4618158117488));
#44536=CARTESIAN_POINT('Ctrl Pts',(-2.63048120009413,4.58819259887652,17.5411877018022));
#44537=CARTESIAN_POINT('Ctrl Pts',(-4.5045850370732,2.7712186210673,17.6205595918556));
#44538=CARTESIAN_POINT('Ctrl Pts',(-5.28138253005218,0.27918271172893,17.699931481909));
#44539=CARTESIAN_POINT('Ctrl Pts',(-4.77164579536179,-2.28086298099153,
17.7793033719624));
#44540=CARTESIAN_POINT('Ctrl Pts',(-3.09954884704088,-4.28529268150238,
17.8586752620158));
#44541=CARTESIAN_POINT('Ctrl Pts',(-0.672404619068171,-5.24583989230806,
17.9380471520692));
#44542=CARTESIAN_POINT('Ctrl Pts',(1.91852825506979,-4.9285020674696,18.0174190421226));
#44543=CARTESIAN_POINT('Ctrl Pts',(4.04212630117149,-3.41061102326166,18.096790932176));
#44544=CARTESIAN_POINT('Ctrl Pts',(4.95529462550652,-1.52742091164643,18.1604301996809));
#44545=CARTESIAN_POINT('Ctrl Pts',(5.07339585550224,-0.342021443822988,
18.1976121705012));
#44546=CARTESIAN_POINT('Ctrl Pts',(5.07322996641872,-7.44046081432165E-5,
18.2083368446371));
#44547=CARTESIAN_POINT('Origin',(0.,0.,-2.20833684463713));
#44548=CARTESIAN_POINT('',(5.07366101292862,-0.000128884195875409,16.2083368446371));
#44549=CARTESIAN_POINT('',(5.07342183474754,-0.000122761774360241,16.2916631553629));
#44550=CARTESIAN_POINT('',(5.0736,-1.85409460923845E-12,-2.20833684463713));
#44551=CARTESIAN_POINT('Ctrl Pts',(5.07342183474754,-0.000122761774360089,
16.2916631553629));
#44552=CARTESIAN_POINT('Ctrl Pts',(5.07288953552851,0.589818979702204,16.3101676916039));
#44553=CARTESIAN_POINT('Ctrl Pts',(4.82300217163475,2.02368301235074,16.3551295245292));
#44554=CARTESIAN_POINT('Ctrl Pts',(3.50037037246945,3.9646372600474,16.4265486541391));
#44555=CARTESIAN_POINT('Ctrl Pts',(1.17777659548083,5.15594643483254,16.5059205441925));
#44556=CARTESIAN_POINT('Ctrl Pts',(-1.43172095156687,5.09127847004474,16.5852924342459));
#44557=CARTESIAN_POINT('Ctrl Pts',(-3.69245444696213,3.78638634033038,16.6646643242993));
#44558=CARTESIAN_POINT('Ctrl Pts',(-5.05371420635461,1.5591388772047,16.7440362143527));
#44559=CARTESIAN_POINT('Ctrl Pts',(-5.18390038229795,-1.04791136166686,
16.8234081044061));
#44560=CARTESIAN_POINT('Ctrl Pts',(-4.05129987868913,-3.39969271923294,
16.9027799944595));
#44561=CARTESIAN_POINT('Ctrl Pts',(-1.93181173129365,-4.9233164424874,16.9821518845129));
#44562=CARTESIAN_POINT('Ctrl Pts',(0.658261551986501,-5.24763120247215,
17.0615237745663));
#44563=CARTESIAN_POINT('Ctrl Pts',(3.08798363825942,-4.29363457062506,17.1408956646198));
#44564=CARTESIAN_POINT('Ctrl Pts',(4.70928800664519,-2.36071043051411,17.2176087915519));
#44565=CARTESIAN_POINT('Ctrl Pts',(5.0733377557896,-0.758421261304332,17.2678646217997));
#44566=CARTESIAN_POINT('Ctrl Pts',(5.07392231800261,8.23068815519051E-5,
17.2916631553629));
#44567=CARTESIAN_POINT('Ctrl Pts',(5.07366101292862,-0.000128884195875374,
16.2083368446371));
#44568=CARTESIAN_POINT('Ctrl Pts',(5.07297133880781,0.668223813333716,16.2293037167406));
#44569=CARTESIAN_POINT('Ctrl Pts',(4.77257120255655,2.18054683036438,16.2767278855287));
#44570=CARTESIAN_POINT('Ctrl Pts',(3.31265234202039,4.12277525560071,16.3506093510011));
#44571=CARTESIAN_POINT('Ctrl Pts',(0.937286345425132,5.20503944789207,16.4299812410546));
#44572=CARTESIAN_POINT('Ctrl Pts',(-1.66640053022416,5.01936755177917,16.509353131108));
#44573=CARTESIAN_POINT('Ctrl Pts',(-3.86415592530783,3.6109888303424,16.5887250211614));
#44574=CARTESIAN_POINT('Ctrl Pts',(-5.12061148999576,1.32298122241861,16.6680969112148));
#44575=CARTESIAN_POINT('Ctrl Pts',(-5.1296974302943,-1.28730168253218,16.7474688012682));
#44576=CARTESIAN_POINT('Ctrl Pts',(-3.88920043041393,-3.58400074773889,
16.8268406913216));
#44577=CARTESIAN_POINT('Ctrl Pts',(-1.70130281532588,-5.00764516247516,
16.906212581375));
#44578=CARTESIAN_POINT('Ctrl Pts',(0.90102840177319,-5.21143830245825,16.9855844714284));
#44579=CARTESIAN_POINT('Ctrl Pts',(3.28387109087768,-4.1457366023928,17.0649563614818));
#44580=CARTESIAN_POINT('Ctrl Pts',(4.76464092528408,-2.20406061763576,17.1392071525514));
#44581=CARTESIAN_POINT('Ctrl Pts',(5.07300074510805,-0.679985153784537,
17.1870006469365));
#44582=CARTESIAN_POINT('Ctrl Pts',(5.07369825422177,0.000126003717071926,
17.2083368446371));
#44583=CARTESIAN_POINT('Origin',(0.,0.,-2.20833684463713));
#44584=CARTESIAN_POINT('',(5.07324617544329,7.96922658102828E-5,15.2083368446371));
#44585=CARTESIAN_POINT('',(5.07342714732068,0.00012340910666319,15.2916631553629));
#44586=CARTESIAN_POINT('',(5.0736,-1.85409460923845E-12,-2.20833684463713));
#44587=CARTESIAN_POINT('Ctrl Pts',(5.07342714732068,0.000123409106663336,
15.2916631553629));
#44588=CARTESIAN_POINT('Ctrl Pts',(5.07365576358557,0.251759202071401,15.2995561680391));
#44589=CARTESIAN_POINT('Ctrl Pts',(4.99363067660841,1.34673145111339,15.3339064773998));
#44590=CARTESIAN_POINT('Ctrl Pts',(4.21831964333036,3.19009729224721,15.3947140834449));
#44591=CARTESIAN_POINT('Ctrl Pts',(2.17873636962922,4.81913365439941,15.4740859734983));
#44592=CARTESIAN_POINT('Ctrl Pts',(-0.391582261162836,5.27423972531144,
15.5534578635517));
#44593=CARTESIAN_POINT('Ctrl Pts',(-2.86651231988745,4.44455267346898,15.6328297536051));
#44594=CARTESIAN_POINT('Ctrl Pts',(-4.64316632240643,2.53218242822043,15.7122016436585));
#44595=CARTESIAN_POINT('Ctrl Pts',(-5.28875528625864,0.00297814834715876,
15.7915735337119));
#44596=CARTESIAN_POINT('Ctrl Pts',(-4.64601516884489,-2.52695160186966,
15.8709454237653));
#44597=CARTESIAN_POINT('Ctrl Pts',(-2.87151604007055,-4.44132153518687,
15.9503173138187));
#44598=CARTESIAN_POINT('Ctrl Pts',(-0.397521959947054,-5.27379537322474,
16.0296892038721));
#44599=CARTESIAN_POINT('Ctrl Pts',(2.1733075897557,-4.82158433170501,16.1090610939255));
#44600=CARTESIAN_POINT('Ctrl Pts',(4.21472422106055,-3.1948460193553,16.1884329839789));
#44601=CARTESIAN_POINT('Ctrl Pts',(4.99287463290549,-1.35054413899492,16.2493003377914));
#44602=CARTESIAN_POINT('Ctrl Pts',(5.07365060287866,-0.253664125066255,
16.2837103949194));
#44603=CARTESIAN_POINT('Ctrl Pts',(5.07342183474754,-0.000122761774360089,
16.2916631553629));
#44604=CARTESIAN_POINT('Ctrl Pts',(5.07324617544329,7.96922658102828E-5,
15.2083368446371));
#44605=CARTESIAN_POINT('Ctrl Pts',(5.07343036424897,0.330250553788653,15.2186921931759));
#44606=CARTESIAN_POINT('Ctrl Pts',(4.96059306642381,1.5038639780885,15.2555048383992));
#44607=CARTESIAN_POINT('Ctrl Pts',(4.06576497321036,3.38238030533612,15.3187747803069));
#44608=CARTESIAN_POINT('Ctrl Pts',(1.95279534724736,4.91503119817963,15.3981466703603));
#44609=CARTESIAN_POINT('Ctrl Pts',(-0.635870902865948,5.2503913703836,15.4775185604137));
#44610=CARTESIAN_POINT('Ctrl Pts',(-3.06964040851742,4.30676782630626,15.5568904504671));
#44611=CARTESIAN_POINT('Ctrl Pts',(-4.75565230518791,2.31402517260967,15.6362623405205));
#44612=CARTESIAN_POINT('Ctrl Pts',(-5.28319782677237,-0.24240889112691,
15.7156342305739));
#44613=CARTESIAN_POINT('Ctrl Pts',(-4.52376805191524,-2.73979268554778,
15.7950061206273));
#44614=CARTESIAN_POINT('Ctrl Pts',(-2.66235839280204,-4.56976904619777,
15.8743780106807));
#44615=CARTESIAN_POINT('Ctrl Pts',(-0.15240412223312,-5.28655978220556,
15.9537499007341));
#44616=CARTESIAN_POINT('Ctrl Pts',(2.39467545517194,-4.71555625687092,16.0331217907875));
#44617=CARTESIAN_POINT('Ctrl Pts',(4.35841739221953,-2.99585366506689,16.112493680841));
#44618=CARTESIAN_POINT('Ctrl Pts',(5.02217539318898,-1.19342375387563,16.1708986987908));
#44619=CARTESIAN_POINT('Ctrl Pts',(5.0738416122916,-0.175144979162809,16.2028464200562));
#44620=CARTESIAN_POINT('Ctrl Pts',(5.07366101292862,-0.000128884195875374,
16.2083368446371));
#44621=CARTESIAN_POINT('Origin',(0.,0.,-2.20833684463713));
#44622=CARTESIAN_POINT('',(5.07403332299931,-8.66482790312043E-6,14.2083368446371));
#44623=CARTESIAN_POINT('',(5.07391786048903,-8.38031740753252E-5,14.2916631553629));
#44624=CARTESIAN_POINT('',(5.0736,-1.85409460923845E-12,-2.20833684463713));
#44625=CARTESIAN_POINT('Ctrl Pts',(5.07391786048903,-8.38031740754523E-5,
14.2916631553629));
#44626=CARTESIAN_POINT('Ctrl Pts',(5.07332646114364,0.756517455027875,14.3154019411588));
#44627=CARTESIAN_POINT('Ctrl Pts',(4.7106825315255,2.35691208085668,14.3655980236392));
#44628=CARTESIAN_POINT('Ctrl Pts',(3.09281731455568,4.29015412381589,14.442251402804));
#44629=CARTESIAN_POINT('Ctrl Pts',(0.664171081076821,5.24688651700904,14.5216232928574));
#44630=CARTESIAN_POINT('Ctrl Pts',(-1.92626575763464,4.9254889684451,14.6009951829108));
#44631=CARTESIAN_POINT('Ctrl Pts',(-4.04746852150321,3.4042532095528,14.6803670729642));
#44632=CARTESIAN_POINT('Ctrl Pts',(-5.1827169124532,1.05374890400015,14.7597389630177));
#44633=CARTESIAN_POINT('Ctrl Pts',(-5.05546693527891,-1.55344630213332,
14.839110853071));
#44634=CARTESIAN_POINT('Ctrl Pts',(-3.69671640275692,-3.78222542756219,
14.9184827431245));
#44635=CARTESIAN_POINT('Ctrl Pts',(-1.43745393706629,-5.08966281065088,
14.9978546331779));
#44636=CARTESIAN_POINT('Ctrl Pts',(1.17196912594334,-5.15726959884254,15.0772265232312));
#44637=CARTESIAN_POINT('Ctrl Pts',(3.49590310398282,-3.96857692817882,15.1565984132847));
#44638=CARTESIAN_POINT('Ctrl Pts',(4.82182831793198,-2.02749096887971,15.2280772906619));
#44639=CARTESIAN_POINT('Ctrl Pts',(5.07288944423512,-0.591721367900843,
15.2730988713546));
#44640=CARTESIAN_POINT('Ctrl Pts',(5.07342714732068,0.000123409106663336,
15.2916631553629));
#44641=CARTESIAN_POINT('Ctrl Pts',(5.07403332299931,-8.66482790325162E-6,
14.2083368446371));
#44642=CARTESIAN_POINT('Ctrl Pts',(5.07395003551347,0.835016825572543,14.2345379662956));
#44643=CARTESIAN_POINT('Ctrl Pts',(4.65105118571099,2.51331333377907,14.2871963846386));
#44644=CARTESIAN_POINT('Ctrl Pts',(2.89043509646017,4.42903220810837,14.3663120996661));
#44645=CARTESIAN_POINT('Ctrl Pts',(0.420014577610126,5.27205169757513,14.4456839897195));
#44646=CARTESIAN_POINT('Ctrl Pts',(-2.15272056265924,4.83081106300113,14.5250558797729));
#44647=CARTESIAN_POINT('Ctrl Pts',(-4.201057738831,3.21279554629894,14.6044277698263));
#44648=CARTESIAN_POINT('Ctrl Pts',(-5.22602654870706,0.81215014592063,14.6837996598797));
#44649=CARTESIAN_POINT('Ctrl Pts',(-4.97794685893165,-1.78633323234006,
14.7631715499331));
#44650=CARTESIAN_POINT('Ctrl Pts',(-3.51725033281897,-3.94966978918425,
14.8425434399865));
#44651=CARTESIAN_POINT('Ctrl Pts',(-1.19975941093315,-5.15087552782897,
14.9219153300399));
#44652=CARTESIAN_POINT('Ctrl Pts',(1.40999024783357,-5.09733938916413,15.0012872200933));
#44653=CARTESIAN_POINT('Ctrl Pts',(3.67626940318851,-3.8021026580683,15.0806591101467));
#44654=CARTESIAN_POINT('Ctrl Pts',(4.86818118380815,-1.87050241988135,15.1496756516613));
#44655=CARTESIAN_POINT('Ctrl Pts',(5.07295977285751,-0.513316266501481,
15.1922348964914));
#44656=CARTESIAN_POINT('Ctrl Pts',(5.07324617544329,7.96922658102828E-5,
15.2083368446371));
#44657=CARTESIAN_POINT('Origin',(0.,0.,-2.20833684463713));
#44658=CARTESIAN_POINT('',(5.07322036085286,-6.69861637152269E-5,13.2083368446371));
#44659=CARTESIAN_POINT('',(5.07316540514723,3.01288341894208E-6,13.2916631553629));
#44660=CARTESIAN_POINT('',(5.0736,-1.85409460923845E-12,-2.20833684463713));
#44661=CARTESIAN_POINT('Ctrl Pts',(5.07316545149283,3.01256212205392E-6,
13.2916631553629));
#44662=CARTESIAN_POINT('Ctrl Pts',(5.07317410528241,0.418572877762161,13.3047904175941));
#44663=CARTESIAN_POINT('Ctrl Pts',(4.91873112752187,1.68074170142874,13.3443749765097));
#44664=CARTESIAN_POINT('Ctrl Pts',(3.8835697329937,3.59010131838716,13.4104168321098));
#44665=CARTESIAN_POINT('Ctrl Pts',(1.69344007832116,5.01030957610862,13.4897887221632));
#44666=CARTESIAN_POINT('Ctrl Pts',(-0.909207831064397,5.21001751122212,
13.5691606122166));
#44667=CARTESIAN_POINT('Ctrl Pts',(-3.29037472530003,4.14057671278008,13.64853250227));
#44668=CARTESIAN_POINT('Ctrl Pts',(-4.87001361957351,2.06250059211591,13.7279043923234));
#44669=CARTESIAN_POINT('Ctrl Pts',(-5.26332797571119,-0.517996107520081,
13.8072762823768));
#44670=CARTESIAN_POINT('Ctrl Pts',(-4.37450728714447,-2.97231010192914,
13.8866481724302));
#44671=CARTESIAN_POINT('Ctrl Pts',(-2.420066306237,-4.70257593460501,13.9660200624836));
#44672=CARTESIAN_POINT('Ctrl Pts',(0.123897470143854,-5.28730467858643,
14.045391952537));
#44673=CARTESIAN_POINT('Ctrl Pts',(2.63768009704007,-4.58405770611459,14.1247638425904));
#44674=CARTESIAN_POINT('Ctrl Pts',(4.50892969070322,-2.76414442307289,14.2041357326438));
#44675=CARTESIAN_POINT('Ctrl Pts',(5.05065740926092,-1.01658127603429,14.2597688369013));
#44676=CARTESIAN_POINT('Ctrl Pts',(5.07398558617533,-0.0867280307438605,
14.2889446444744));
#44677=CARTESIAN_POINT('Ctrl Pts',(5.07391786048903,-8.38031740754523E-5,
14.2916631553629));
#44678=CARTESIAN_POINT('Ctrl Pts',(5.07322036085286,-6.69861637153657E-5,
13.2083368446371));
#44679=CARTESIAN_POINT('Ctrl Pts',(5.07298878663719,0.497000397927876,13.2239264427309));
#44680=CARTESIAN_POINT('Ctrl Pts',(4.87730902789417,1.83782529464356,13.2659733375091));
#44681=CARTESIAN_POINT('Ctrl Pts',(3.71281646953824,3.76642207019282,13.3344775289718));
#44682=CARTESIAN_POINT('Ctrl Pts',(1.45915164597774,5.08348481077208,13.4138494190252));
#44683=CARTESIAN_POINT('Ctrl Pts',(-1.14995928876559,5.16222190355004,13.4932213090786));
#44684=CARTESIAN_POINT('Ctrl Pts',(-3.47894268615732,3.98345316700755,13.572593199132));
#44685=CARTESIAN_POINT('Ctrl Pts',(-4.96046334571011,1.83432405620607,13.6519650891854));
#44686=CARTESIAN_POINT('Ctrl Pts',(-5.23362611404733,-0.761642334479749,
13.7313369792388));
#44687=CARTESIAN_POINT('Ctrl Pts',(-4.23188914543755,-3.17207433835303,
13.8107088692922));
#44688=CARTESIAN_POINT('Ctrl Pts',(-2.19927334812693,-4.80979605467098,
13.8900807593456));
#44689=CARTESIAN_POINT('Ctrl Pts',(0.369080568778457,-5.27586209837409,
13.9694526493991));
#44690=CARTESIAN_POINT('Ctrl Pts',(2.84752727607539,-4.45673981283591,14.0488245394524));
#44691=CARTESIAN_POINT('Ctrl Pts',(4.63232264181505,-2.55196557371717,14.1281964295059));
#44692=CARTESIAN_POINT('Ctrl Pts',(5.07202231626624,-0.859526521495883,
14.1813671979007));
#44693=CARTESIAN_POINT('Ctrl Pts',(5.07403413732223,-0.00817292128436273,
14.2080806696111));
#44694=CARTESIAN_POINT('Ctrl Pts',(5.07403332299931,-8.66482790325162E-6,
14.2083368446371));
#44695=CARTESIAN_POINT('Origin',(0.,0.,-2.20833684463713));
#44696=CARTESIAN_POINT('',(5.07371259150425,0.000124614973235349,12.2083368446371));
#44697=CARTESIAN_POINT('',(5.07393295843892,7.85666071205126E-5,12.2916631553629));
#44698=CARTESIAN_POINT('',(5.0736,-1.85409460923845E-12,-2.20833684463713));
#44699=CARTESIAN_POINT('Ctrl Pts',(5.07393295843892,7.85666071204203E-5,
12.2916631553629));
#44700=CARTESIAN_POINT('Ctrl Pts',(5.07399255467328,0.080259357669063,12.2941788940293));
#44701=CARTESIAN_POINT('Ctrl Pts',(5.0525559141232,1.00364648464526,12.3231519293802));
#44702=CARTESIAN_POINT('Ctrl Pts',(4.51946174941847,2.74689039512926,12.3785822614155));
#44703=CARTESIAN_POINT('Ctrl Pts',(2.6551818185972,4.57394259446934,12.4579541514689));
#44704=CARTESIAN_POINT('Ctrl Pts',(0.144105473910954,5.28679250204684,12.5373260415223));
#44705=CARTESIAN_POINT('Ctrl Pts',(-2.40207464524796,4.7117914582425,12.6166979315757));
#44706=CARTESIAN_POINT('Ctrl Pts',(-4.36311469772651,2.98900844458373,12.6960698216291));
#44707=CARTESIAN_POINT('Ctrl Pts',(-5.26130966742946,0.538109589882336,
12.7754417116825));
#44708=CARTESIAN_POINT('Ctrl Pts',(-4.87786124785798,-2.043871569829,12.854813601736));
#44709=CARTESIAN_POINT('Ctrl Pts',(-3.30617662527107,-4.12797013916298,
12.9341854917893));
#44710=CARTESIAN_POINT('Ctrl Pts',(-0.929114694865931,-5.20650431970379,
13.0135573818428));
#44711=CARTESIAN_POINT('Ctrl Pts',(1.67427751864803,-5.01674557236658,13.0929292718962));
#44712=CARTESIAN_POINT('Ctrl Pts',(3.86981943456978,-3.60491870797887,13.1723011619496));
#44713=CARTESIAN_POINT('Ctrl Pts',(4.91547184132152,-1.69367935817457,13.2385457897718));
#44714=CARTESIAN_POINT('Ctrl Pts',(5.07315666403118,-0.425032354751582,
13.2783331209096));
#44715=CARTESIAN_POINT('Ctrl Pts',(5.07316545149283,3.01256212205392E-6,
13.2916631553629));
#44716=CARTESIAN_POINT('Ctrl Pts',(5.07371259150425,0.000124614973235296,
12.2083368446371));
#44717=CARTESIAN_POINT('Ctrl Pts',(5.07387461653381,0.158804080659856,12.2133149191661));
#44718=CARTESIAN_POINT('Ctrl Pts',(5.02779682862049,1.1607339041827,12.2447502903796));
#44719=CARTESIAN_POINT('Ctrl Pts',(4.38714636147788,2.95362288559007,12.3026429582776));
#44720=CARTESIAN_POINT('Ctrl Pts',(2.44010389315499,4.69220996311119,12.382014848331));
#44721=CARTESIAN_POINT('Ctrl Pts',(-0.101342482462103,5.28778507964898,
12.4613867383844));
#44722=CARTESIAN_POINT('Ctrl Pts',(-2.61810205366918,4.59526745509803,12.5407586284378));
#44723=CARTESIAN_POINT('Ctrl Pts',(-4.49709775967304,2.78335284993721,12.6201305184912));
#44724=CARTESIAN_POINT('Ctrl Pts',(-5.28061040557763,0.293419651378745,
12.6995024085446));
#44725=CARTESIAN_POINT('Ctrl Pts',(-4.7777780451164,-2.26798992478223,12.778874298598));
#44726=CARTESIAN_POINT('Ctrl Pts',(-3.11108952829712,-4.27692217537683,
12.8582461886514));
#44727=CARTESIAN_POINT('Ctrl Pts',(-0.686546488664521,-5.24400565085626,
12.9376180787048));
#44728=CARTESIAN_POINT('Ctrl Pts',(1.90523775596186,-4.93366095719673,13.0169899687582));
#44729=CARTESIAN_POINT('Ctrl Pts',(4.03291030040817,-3.42148737483739,13.0963618588116));
#44730=CARTESIAN_POINT('Ctrl Pts',(4.95323103438167,-1.53655914035534,13.1601441507712));
#44731=CARTESIAN_POINT('Ctrl Pts',(5.07338179405736,-0.346578710011678,
13.1974691460464));
#44732=CARTESIAN_POINT('Ctrl Pts',(5.07322036085286,-6.69861637153657E-5,
13.2083368446371));
#44733=CARTESIAN_POINT('Origin',(0.,0.,-2.20833684463713));
#44734=CARTESIAN_POINT('',(5.0736465461671,-0.000129729951178492,11.2083368446371));
#44735=CARTESIAN_POINT('',(5.07340926806867,-0.000121118768615341,11.2916631553629));
#44736=CARTESIAN_POINT('',(5.0736,-1.85409460923845E-12,-2.20833684463713));
#44737=CARTESIAN_POINT('Ctrl Pts',(5.07340926806867,-0.000121118768615022,
11.2916631553629));
#44738=CARTESIAN_POINT('Ctrl Pts',(5.07289012258619,0.585265031435054,11.310024667149));
#44739=CARTESIAN_POINT('Ctrl Pts',(4.82580215794652,2.01456720880964,11.3548434756196));
#44740=CARTESIAN_POINT('Ctrl Pts',(3.51104609249152,3.95518604919035,11.4261195807747));
#44741=CARTESIAN_POINT('Ctrl Pts',(1.19167245960881,5.152752477688,11.5054914708281));
#44742=CARTESIAN_POINT('Ctrl Pts',(-1.41798994671238,5.09511980804502,11.5848633608815));
#44743=CARTESIAN_POINT('Ctrl Pts',(-3.68223314068194,3.79632723101863,11.6642352509349));
#44744=CARTESIAN_POINT('Ctrl Pts',(-5.04949249206616,1.57275774354392,11.7436071409883));
#44745=CARTESIAN_POINT('Ctrl Pts',(-5.18670664924514,-1.03393204901786,
11.8229790310417));
#44746=CARTESIAN_POINT('Ctrl Pts',(-4.06045054724843,-3.38875828300867,
11.9023509210951));
#44747=CARTESIAN_POINT('Ctrl Pts',(-1.94507767959685,-4.91809050014781,
11.9817228111485));
#44748=CARTESIAN_POINT('Ctrl Pts',(0.644111805448097,-5.24938675745961,
12.0610947012019));
#44749=CARTESIAN_POINT('Ctrl Pts',(3.0763970804032,-4.30194401997477,12.1404665912553));
#44750=CARTESIAN_POINT('Ctrl Pts',(4.70593891054333,-2.36980219715329,12.2173227426423));
#44751=CARTESIAN_POINT('Ctrl Pts',(5.07336579829568,-0.762978855367823,
12.2677215973449));
#44752=CARTESIAN_POINT('Ctrl Pts',(5.07393295843892,7.85666071204203E-5,
12.2916631553629));
#44753=CARTESIAN_POINT('Ctrl Pts',(5.0736465461671,-0.000129729951178388,
11.2083368446371));
#44754=CARTESIAN_POINT('Ctrl Pts',(5.07296127147132,0.663669285094766,11.2291606922858));
#44755=CARTESIAN_POINT('Ctrl Pts',(4.77561643393883,2.17143981582611,11.276441836619));
#44756=CARTESIAN_POINT('Ctrl Pts',(3.32375507563458,4.11382954733217,11.3501802776367));
#44757=CARTESIAN_POINT('Ctrl Pts',(0.951315435152466,5.20249366075065,11.4295521676901));
#44758=CARTESIAN_POINT('Ctrl Pts',(-1.6528625396318,5.02384183393465,11.5089240577436));
#44759=CARTESIAN_POINT('Ctrl Pts',(-3.85440685831092,3.62139325645746,11.5882959477969));
#44760=CARTESIAN_POINT('Ctrl Pts',(-5.11702619789041,1.33678129752526,11.6676678378503));
#44761=CARTESIAN_POINT('Ctrl Pts',(-5.13314928200913,-1.27346762656892,
11.7470397279037));
#44762=CARTESIAN_POINT('Ctrl Pts',(-3.89884856306365,-3.57350265560368,
11.8264116179572));
#44763=CARTESIAN_POINT('Ctrl Pts',(-1.71479696411077,-5.00304034754732,
11.9057835080105));
#44764=CARTESIAN_POINT('Ctrl Pts',(0.886975379660772,-5.21384848487043,
11.985155398064));
#44765=CARTESIAN_POINT('Ctrl Pts',(3.27268248423369,-4.15457467193696,12.0645272881174));
#44766=CARTESIAN_POINT('Ctrl Pts',(4.76154396611873,-2.21316538967253,12.1389211036417));
#44767=CARTESIAN_POINT('Ctrl Pts',(5.0730134915642,-0.684540002865494,12.1868576224816));
#44768=CARTESIAN_POINT('Ctrl Pts',(5.07371259150425,0.000124614973235296,
12.2083368446371));
#44769=CARTESIAN_POINT('Origin',(0.,0.,-2.20833684463713));
#44770=CARTESIAN_POINT('',(5.07325419654647,8.30592867887003E-5,10.2083368446371));
#44771=CARTESIAN_POINT('',(5.07344000894767,0.000124864012350097,10.2916631553629));
#44772=CARTESIAN_POINT('',(5.0736,-1.85409460923845E-12,-2.20833684463713));
#44773=CARTESIAN_POINT('Ctrl Pts',(5.07344000894767,0.000124864012350061,
10.2916631553629));
#44774=CARTESIAN_POINT('Ctrl Pts',(5.07366802985413,0.247199120889535,10.2994131435843));
#44775=CARTESIAN_POINT('Ctrl Pts',(4.99543134296861,1.33760465491503,10.3336204284901));
#44776=CARTESIAN_POINT('Ctrl Pts',(4.22690463795744,3.1787133448809,10.3942850100804));
#44777=CARTESIAN_POINT('Ctrl Pts',(2.1917205673539,4.81324238969408,10.4736569001339));
#44778=CARTESIAN_POINT('Ctrl Pts',(-0.377361782165876,5.27527624230907,
10.5530287901872));
#44779=CARTESIAN_POINT('Ctrl Pts',(-2.85451963682615,4.45226447892349,10.6324006802407));
#44780=CARTESIAN_POINT('Ctrl Pts',(-4.63632282632763,2.54469094339242,10.711772570294));
#44781=CARTESIAN_POINT('Ctrl Pts',(-5.28872803766221,0.0172363266288179,
10.7911444603475));
#44782=CARTESIAN_POINT('Ctrl Pts',(-4.65281080542322,-2.5144170211496,10.8705163504009));
#44783=CARTESIAN_POINT('Ctrl Pts',(-2.88347915980519,-4.43356394814365,
10.9498882404543));
#44784=CARTESIAN_POINT('Ctrl Pts',(-0.411738373331464,-5.27270451089727,
11.0292601305077));
#44785=CARTESIAN_POINT('Ctrl Pts',(2.16030096951836,-4.82742592572977,11.1086320205611));
#44786=CARTESIAN_POINT('Ctrl Pts',(4.20609577793862,-3.20619707038057,11.1880039106145));
#44787=CARTESIAN_POINT('Ctrl Pts',(4.99105565025759,-1.3596709971465,11.2490142888818));
#44788=CARTESIAN_POINT('Ctrl Pts',(5.07363816480692,-0.25822406855438,11.2835673704646));
#44789=CARTESIAN_POINT('Ctrl Pts',(5.07340926806867,-0.000121118768615022,
11.2916631553629));
#44790=CARTESIAN_POINT('Ctrl Pts',(5.07325419654647,8.30592867889779E-5,
10.2083368446371));
#44791=CARTESIAN_POINT('Ctrl Pts',(5.07344390313192,0.32569224224827,10.2185491687211));
#44792=CARTESIAN_POINT('Ctrl Pts',(4.96261803044706,1.49473693663548,10.2552187894896));
#44793=CARTESIAN_POINT('Ctrl Pts',(4.07486890650351,3.37140693807807,10.3183457069425));
#44794=CARTESIAN_POINT('Ctrl Pts',(1.96603890048266,4.90974870936374,10.3977175969959));
#44795=CARTESIAN_POINT('Ctrl Pts',(-0.621713829942471,5.25208656259283,
10.4770894870493));
#44796=CARTESIAN_POINT('Ctrl Pts',(-3.05801844753381,4.31502775447074,10.5564613771027));
#44797=CARTESIAN_POINT('Ctrl Pts',(-4.74939654011498,2.32683773651149,10.6358332671561));
#44798=CARTESIAN_POINT('Ctrl Pts',(-5.28383214813503,-0.228164803694007,
10.7152051572095));
#44799=CARTESIAN_POINT('Ctrl Pts',(-4.53113794043347,-2.72758690275384,
10.7945770472629));
#44800=CARTESIAN_POINT('Ctrl Pts',(-2.67466855994604,-4.56257486971405,
10.8739489373163));
#44801=CARTESIAN_POINT('Ctrl Pts',(-0.166655838534166,-5.2861296975001,
10.9533208273697));
#44802=CARTESIAN_POINT('Ctrl Pts',(2.38195387625819,-4.72199503162473,11.0326927174231));
#44803=CARTESIAN_POINT('Ctrl Pts',(4.3503248991595,-3.00759282800428,11.1120646074765));
#44804=CARTESIAN_POINT('Ctrl Pts',(5.02057706818124,-1.20254945990408,11.1706126498812));
#44805=CARTESIAN_POINT('Ctrl Pts',(5.07383193265951,-0.17970643375256,11.2027033956014));
#44806=CARTESIAN_POINT('Ctrl Pts',(5.0736465461671,-0.000129729951178388,
11.2083368446371));
#44807=CARTESIAN_POINT('Origin',(0.,0.,-2.20833684463713));
#44808=CARTESIAN_POINT('',(5.07403156349013,-1.34850231131101E-5,9.20833684463708));
#44809=CARTESIAN_POINT('',(5.07390676572803,-8.73588085612467E-5,9.29166315536294));
#44810=CARTESIAN_POINT('',(5.0736,-1.85409460923845E-12,-2.20833684463713));
#44811=CARTESIAN_POINT('Ctrl Pts',(5.07390676572803,-8.73588085611478E-5,
9.29166315536294));
#44812=CARTESIAN_POINT('Ctrl Pts',(5.07329990983557,0.75196019632477,9.31525891670402));
#44813=CARTESIAN_POINT('Ctrl Pts',(4.71401054212216,2.34781906214645,9.36531197472956));
#44814=CARTESIAN_POINT('Ctrl Pts',(3.10437209115777,4.28180047024037,9.44182232943961));
#44815=CARTESIAN_POINT('Ctrl Pts',(0.67831398067512,5.24507688131743,9.52119421949299));
#44816=CARTESIAN_POINT('Ctrl Pts',(-1.91297991407746,4.93066417388633,9.6005661095464));
#44817=CARTESIAN_POINT('Ctrl Pts',(-4.03827613607002,3.41515258753654,9.6799379995998));
#44818=CARTESIAN_POINT('Ctrl Pts',(-5.1798572298885,1.06771739017486,9.75930988965322));
#44819=CARTESIAN_POINT('Ctrl Pts',(-5.05963656792565,-1.53981140008104,
9.8386817797066));
#44820=CARTESIAN_POINT('Ctrl Pts',(-3.70689963733171,-3.77224554159189,
9.91805366976003));
#44821=CARTESIAN_POINT('Ctrl Pts',(-1.45117016016697,-5.08576901889487,
9.99742555981341));
#44822=CARTESIAN_POINT('Ctrl Pts',(1.1580611559038,-5.16041042035386,10.0767974498668));
#44823=CARTESIAN_POINT('Ctrl Pts',(3.48519133772131,-3.97798726578937,10.1561693399202));
#44824=CARTESIAN_POINT('Ctrl Pts',(4.81900834166099,-2.03660616436304,10.2277912417523));
#44825=CARTESIAN_POINT('Ctrl Pts',(5.07288960070042,-0.596275311661321,
10.2729558468998));
#44826=CARTESIAN_POINT('Ctrl Pts',(5.07344000894767,0.000124864012350061,
10.2916631553629));
#44827=CARTESIAN_POINT('Ctrl Pts',(5.07403156349013,-1.34850231132098E-5,
9.20833684463708));
#44828=CARTESIAN_POINT('Ctrl Pts',(5.07390455498411,0.830454679150979,9.2343949418408));
#44829=CARTESIAN_POINT('Ctrl Pts',(4.65463656321598,2.50423700786744,9.28691033572898));
#44830=CARTESIAN_POINT('Ctrl Pts',(2.90236501609723,4.42122366100663,9.36588302630163));
#44831=CARTESIAN_POINT('Ctrl Pts',(0.434226208411351,5.27090020273944,9.44525491635504));
#44832=CARTESIAN_POINT('Ctrl Pts',(-2.13968914250016,4.83659712202464,9.52462680640844));
#44833=CARTESIAN_POINT('Ctrl Pts',(-4.1923809544202,3.22410968801074,9.60399869646184));
#44834=CARTESIAN_POINT('Ctrl Pts',(-5.22381804552131,0.826236270443201,
9.68337058651526));
#44835=CARTESIAN_POINT('Ctrl Pts',(-4.98274462345855,-1.77290647376134,
9.76274247656865));
#44836=CARTESIAN_POINT('Ctrl Pts',(-3.52788564023945,-3.94017312521954,
9.84211436662205));
#44837=CARTESIAN_POINT('Ctrl Pts',(-1.21364152390043,-5.14762232479954,
9.92148625667546));
#44838=CARTESIAN_POINT('Ctrl Pts',(1.39624298131078,-5.10112212012714,10.0008581467289));
#44839=CARTESIAN_POINT('Ctrl Pts',(3.66600578680612,-3.81199985813406,10.0802300367823));
#44840=CARTESIAN_POINT('Ctrl Pts',(4.86560152926764,-1.87962374426628,10.1493896027517));
#44841=CARTESIAN_POINT('Ctrl Pts',(5.07295242603298,-0.517870759272535,
10.1920918720366));
#44842=CARTESIAN_POINT('Ctrl Pts',(5.07325419654647,8.30592867889779E-5,
10.2083368446371));
#44843=CARTESIAN_POINT('Origin',(0.,0.,-2.20833684463713));
#44844=CARTESIAN_POINT('',(5.07321399251666,-6.32753131005193E-5,8.20833684463707));
#44845=CARTESIAN_POINT('',(5.07316567838514,7.26391603613751E-6,8.29166315536292));
#44846=CARTESIAN_POINT('',(5.0736,-1.85409460923845E-12,-2.20833684463713));
#44847=CARTESIAN_POINT('Ctrl Pts',(5.07316594763625,7.25941288019782E-6,
8.29166315536292));
#44848=CARTESIAN_POINT('Ctrl Pts',(5.07318657601694,0.414016596607197,8.30464739313926));
#44849=CARTESIAN_POINT('Ctrl Pts',(4.92101378278626,1.67161602862595,8.34408892760008));
#44850=CARTESIAN_POINT('Ctrl Pts',(3.89323433265495,3.57961838445758,8.40998775874535));
#44851=CARTESIAN_POINT('Ctrl Pts',(1.70694143925982,5.00572594837628,8.48935964879875));
#44852=CARTESIAN_POINT('Ctrl Pts',(-0.895158610488236,5.21244975125697,
8.56873153885215));
#44853=CARTESIAN_POINT('Ctrl Pts',(-3.27920000412133,4.14943233229326,8.64810342890557));
#44854=CARTESIAN_POINT('Ctrl Pts',(-4.86443553513654,2.0756223817956,8.72747531895896));
#44855=CARTESIAN_POINT('Ctrl Pts',(-5.26470533703792,-0.503804586595236,
8.80684720901237));
#44856=CARTESIAN_POINT('Ctrl Pts',(-4.38250457206448,-2.96050587284403,
8.88621909906576));
#44857=CARTESIAN_POINT('Ctrl Pts',(-2.43273539384546,-4.69603448143659,
8.96559098911917));
#44858=CARTESIAN_POINT('Ctrl Pts',(0.109642741545844,-5.28761948484726,
9.04496287917257));
#44859=CARTESIAN_POINT('Ctrl Pts',(2.62531214778668,-4.59115208569632,9.12433476922599));
#44860=CARTESIAN_POINT('Ctrl Pts',(4.50146132585655,-2.77629020081255,9.20370665927937));
#44861=CARTESIAN_POINT('Ctrl Pts',(5.04930321710503,-1.02570491769659,9.25948278799171));
#44862=CARTESIAN_POINT('Ctrl Pts',(5.07398036113186,-0.0912906316256552,
9.28880162001956));
#44863=CARTESIAN_POINT('Ctrl Pts',(5.07390676572803,-8.73588085611478E-5,
9.29166315536294));
#44864=CARTESIAN_POINT('Ctrl Pts',(5.07321399251666,-6.32753131006233E-5,
8.20833684463707));
#44865=CARTESIAN_POINT('Ctrl Pts',(5.07299759473682,0.492445607247212,8.22378341827604));
#44866=CARTESIAN_POINT('Ctrl Pts',(4.87982559067105,1.82870276667211,8.26568728859948));
#44867=CARTESIAN_POINT('Ctrl Pts',(3.72295704063487,3.75639883677136,8.33404845560738));
#44868=CARTESIAN_POINT('Ctrl Pts',(1.47285113468463,5.07953254565499,8.41342034566079));
#44869=CARTESIAN_POINT('Ctrl Pts',(-1.1360380475741,5.16530336977162,8.49279223571419));
#44870=CARTESIAN_POINT('Ctrl Pts',(-3.46819087602133,3.99281772621695,8.57216412576759));
#44871=CARTESIAN_POINT('Ctrl Pts',(-4.95550008378004,1.84769052250801,8.651536015821));
#44872=CARTESIAN_POINT('Ctrl Pts',(-5.23566043994335,-0.74753000269027,
8.7309079058744));
#44873=CARTESIAN_POINT('Ctrl Pts',(-4.24042550187429,-3.16065387386283,
8.81027979592781));
#44874=CARTESIAN_POINT('Ctrl Pts',(-2.21223229757129,-4.8038494573511,8.88965168598121));
#44875=CARTESIAN_POINT('Ctrl Pts',(0.354855797726969,-5.27683794616905,
8.96902357603462));
#44876=CARTESIAN_POINT('Ctrl Pts',(2.83550180615889,-4.46440039138287,9.04839546608801));
#44877=CARTESIAN_POINT('Ctrl Pts',(4.6254258508873,-2.56444478303851,9.12776735614143));
#44878=CARTESIAN_POINT('Ctrl Pts',(5.0708816691802,-0.868647987514843,9.18108114899111));
#44879=CARTESIAN_POINT('Ctrl Pts',(5.07403350920893,-0.0127359204844534,
9.20793764515633));
#44880=CARTESIAN_POINT('Ctrl Pts',(5.07403156349013,-1.34850231132098E-5,
9.20833684463708));
#44881=CARTESIAN_POINT('Origin',(0.,0.,-2.20833684463713));
#44882=CARTESIAN_POINT('',(5.0737268532953,0.000123079057421927,7.20833684463709));
#44883=CARTESIAN_POINT('',(5.07394313380083,7.47405269748897E-5,7.29166315536293));
#44884=CARTESIAN_POINT('',(5.0736,-1.85409460923845E-12,-2.20833684463713));
#44885=CARTESIAN_POINT('Ctrl Pts',(5.07394313380082,7.47405269749084E-5,
7.29166315536293));
#44886=CARTESIAN_POINT('Ctrl Pts',(5.07399715749136,0.0756966636928046,
7.29403586957452));
#44887=CARTESIAN_POINT('Ctrl Pts',(5.05387993962774,0.994523136339973,7.32286588047058));
#44888=CARTESIAN_POINT('Ctrl Pts',(4.52685078861501,2.73469619609302,7.37815318805109));
#44889=CARTESIAN_POINT('Ctrl Pts',(2.66750326347436,4.56676775046241,7.45752507810451));
#44890=CARTESIAN_POINT('Ctrl Pts',(0.158357847769689,5.28638478918814,7.5368969681579));
#44891=CARTESIAN_POINT('Ctrl Pts',(-2.38936318913255,4.71825019448189,7.61626885821132));
#44892=CARTESIAN_POINT('Ctrl Pts',(-4.3550406419278,3.0007602960695,7.69564074826471));
#44893=CARTESIAN_POINT('Ctrl Pts',(-5.25983983406839,0.552291831604834,
7.77501263831812));
#44894=CARTESIAN_POINT('Ctrl Pts',(-4.88335368508791,-2.03071370056153,
7.85438452837152));
#44895=CARTESIAN_POINT('Ctrl Pts',(-3.31729338754006,-4.11904187017964,
7.93375641842492));
#44896=CARTESIAN_POINT('Ctrl Pts',(-0.943147763491834,-5.20398055756651,
8.01312830847834));
#44897=CARTESIAN_POINT('Ctrl Pts',(1.66074656812082,-5.02124109994579,8.09250019853171));
#44898=CARTESIAN_POINT('Ctrl Pts',(3.86008671173945,-3.61533842470695,8.17187208858515));
#44899=CARTESIAN_POINT('Ctrl Pts',(4.91315662948087,-1.70280471015196,8.23825974086219));
#44900=CARTESIAN_POINT('Ctrl Pts',(5.07314454265331,-0.429588399925582,
8.27819009645479));
#44901=CARTESIAN_POINT('Ctrl Pts',(5.07316594763625,7.25941288019782E-6,
8.29166315536292));
#44902=CARTESIAN_POINT('Ctrl Pts',(5.0737268532953,0.000123079057421736,
7.20833684463709));
#44903=CARTESIAN_POINT('Ctrl Pts',(5.07388334783635,0.154242294956097,7.2131718947113));
#44904=CARTESIAN_POINT('Ctrl Pts',(5.02933704432274,1.15160862859258,7.24446424146999));
#44905=CARTESIAN_POINT('Ctrl Pts',(4.39509322077433,2.9417846501764,7.30221388491313));
#44906=CARTESIAN_POINT('Ctrl Pts',(2.45274496186498,4.68561452739722,7.38158577496654));
#44907=CARTESIAN_POINT('Ctrl Pts',(-0.0870865406957981,5.28803907717593,
7.46095766501995));
#44908=CARTESIAN_POINT('Ctrl Pts',(-2.60570395470586,4.60230901263053,7.54032955507335));
#44909=CARTESIAN_POINT('Ctrl Pts',(-4.48957765297745,2.79546665964655,7.61970144512676));
#44910=CARTESIAN_POINT('Ctrl Pts',(-5.27980017249532,0.307654816033177,
7.69907333518014));
#44911=CARTESIAN_POINT('Ctrl Pts',(-4.78387505663278,-2.25510105978351,
7.77844522523357));
#44912=CARTESIAN_POINT('Ctrl Pts',(-3.12260856590233,-4.26851930901846,
7.85781711528695));
#44913=CARTESIAN_POINT('Ctrl Pts',(-0.70068154029489,-5.24213570278374,
7.93718900534038));
#44914=CARTESIAN_POINT('Ctrl Pts',(1.8919299575961,-4.93877944262147,8.01656089539376));
#44915=CARTESIAN_POINT('Ctrl Pts',(4.02367150553262,-3.43234744203947,8.09593278544719));
#44916=CARTESIAN_POINT('Ctrl Pts',(4.95114565728143,-1.54568603506211,8.15985810186161));
#44917=CARTESIAN_POINT('Ctrl Pts',(5.07336824653293,-0.351136531432447,
8.19732612159157));
#44918=CARTESIAN_POINT('Ctrl Pts',(5.07321399251666,-6.32753131006233E-5,
8.20833684463707));
#44919=CARTESIAN_POINT('Origin',(0.,0.,-2.20833684463713));
#44920=CARTESIAN_POINT('',(5.07363207848188,-0.00013042437206158,6.20833684463708));
#44921=CARTESIAN_POINT('',(5.07339692231655,-0.000119345805453296,6.29166315536293));
#44922=CARTESIAN_POINT('',(5.0736,-1.85409460923845E-12,-2.20833684463713));
#44923=CARTESIAN_POINT('Ctrl Pts',(5.07339692231655,-0.000119345805453183,
6.29166315536293));
#44924=CARTESIAN_POINT('Ctrl Pts',(5.07289122007049,0.580711075066297,6.30988164269423));
#44925=CARTESIAN_POINT('Ctrl Pts',(4.82858806615863,2.00545098816607,6.35455742671001));
#44926=CARTESIAN_POINT('Ctrl Pts',(3.52169629398765,3.94570609146495,6.42569050741027));
#44927=CARTESIAN_POINT('Ctrl Pts',(1.20555966211655,5.14952106980711,6.50506239746365));
#44928=CARTESIAN_POINT('Ctrl Pts',(-1.40424863498509,5.09892411381582,6.58443428751707));
#44929=CARTESIAN_POINT('Ctrl Pts',(-3.67198507285601,3.80624052997609,6.66380617757046));
#44930=CARTESIAN_POINT('Ctrl Pts',(-5.04523407478029,1.58636517800468,6.74317806762388));
#44931=CARTESIAN_POINT('Ctrl Pts',(-5.1894752235243,-1.01994521996889,6.82254995767727));
#44932=CARTESIAN_POINT('Ctrl Pts',(-4.06957169452636,-3.37779921996849,
6.90192184773068));
#44933=CARTESIAN_POINT('Ctrl Pts',(-1.95832950858598,-4.91282880661553,
6.98129373778407));
#44934=CARTESIAN_POINT('Ctrl Pts',(0.629957410957137,-5.25110417033315,
7.06066562783749));
#44935=CARTESIAN_POINT('Ctrl Pts',(3.06478809957816,-4.31022218127953,7.14003751789089));
#44936=CARTESIAN_POINT('Ctrl Pts',(4.70257511155161,-2.37889312808664,7.2170366937327));
#44937=CARTESIAN_POINT('Ctrl Pts',(5.07339475843234,-0.767536645770191,
7.26757857289005));
#44938=CARTESIAN_POINT('Ctrl Pts',(5.07394313380082,7.47405269749084E-5,
7.29166315536293));
#44939=CARTESIAN_POINT('Ctrl Pts',(5.07363207848188,-0.000130424372061667,
6.20833684463708));
#44940=CARTESIAN_POINT('Ctrl Pts',(5.07295192244443,0.659114832324929,6.22901766783102));
#44941=CARTESIAN_POINT('Ctrl Pts',(4.77864726944019,2.16233220285461,6.27615578770943));
#44942=CARTESIAN_POINT('Ctrl Pts',(3.33483365177601,4.10485393921541,6.34975120427228));
#44943=CARTESIAN_POINT('Ctrl Pts',(0.96533761058682,5.19991006123149,6.42912309432572));
#44944=CARTESIAN_POINT('Ctrl Pts',(-1.63931253580277,5.02827960213728,6.50849498437909));
#44945=CARTESIAN_POINT('Ctrl Pts',(-3.84462977702757,3.63177136187054,6.58786687443252));
#44946=CARTESIAN_POINT('Ctrl Pts',(-5.11340371451209,1.35057165664169,6.6672387644859));
#44947=CARTESIAN_POINT('Ctrl Pts',(-5.13656382546863,-1.25962431470543,
6.74661065453933));
#44948=CARTESIAN_POINT('Ctrl Pts',(-3.90846835813217,-3.56297859112141,
6.82598254459271));
#44949=CARTESIAN_POINT('Ctrl Pts',(-1.72827865000271,-4.99839916925957,
6.90535443464612));
#44950=CARTESIAN_POINT('Ctrl Pts',(0.872915911787522,-5.21622077353501,
6.98472632469953));
#44951=CARTESIAN_POINT('Ctrl Pts',(3.26147008963291,-4.16338254328616,7.06409821475292));
#44952=CARTESIAN_POINT('Ctrl Pts',(4.7584325270959,-2.22226951355623,7.13863505473211));
#44953=CARTESIAN_POINT('Ctrl Pts',(5.07302701285767,-0.689094952273734,
7.18671459802684));
#44954=CARTESIAN_POINT('Ctrl Pts',(5.0737268532953,0.000123079057421736,
7.20833684463709));
#44955=CARTESIAN_POINT('Origin',(0.,0.,-2.20833684463713));
#44956=CARTESIAN_POINT('',(5.07326256235615,8.6340948239616E-5,5.20833684463708));
#44957=CARTESIAN_POINT('',(5.07345306532775,0.000126183674940957,5.29166315536293));
#44958=CARTESIAN_POINT('',(5.0736,-1.85409460923845E-12,-2.20833684463713));
#44959=CARTESIAN_POINT('Ctrl Pts',(5.07345306532775,0.000126183674940827,
5.29166315536293));
#44960=CARTESIAN_POINT('Ctrl Pts',(5.07368016839978,0.24263894378533,5.29927011912949));
#44961=CARTESIAN_POINT('Ctrl Pts',(4.99721910617995,1.32847790639321,5.33333437958052));
#44962=CARTESIAN_POINT('Ctrl Pts',(4.23545891089922,3.1673062942182,5.39385593671601));
#44963=CARTESIAN_POINT('Ctrl Pts',(2.20468883537238,4.80731614172549,5.47322782676942));
#44964=CARTESIAN_POINT('Ctrl Pts',(-0.363138560455233,5.27627441792221,
5.55259971682281));
#44965=CARTESIAN_POINT('Ctrl Pts',(-2.84250620674952,4.45994392474844,5.63197160687622));
#44966=CARTESIAN_POINT('Ctrl Pts',(-4.62944563286038,2.55718096342436,5.71134349692963));
#44967=CARTESIAN_POINT('Ctrl Pts',(-5.28866234991055,0.0314943796341776,
5.79071538698302));
#44968=CARTESIAN_POINT('Ctrl Pts',(-4.65957262477808,-2.50186416532327,
5.87008727703643));
#44969=CARTESIAN_POINT('Ctrl Pts',(-2.89542132203872,-4.42577413739037,
5.94945916708984));
#44970=CARTESIAN_POINT('Ctrl Pts',(-0.425951794157121,-5.27157532587407,
6.02883105714324));
#44971=CARTESIAN_POINT('Ctrl Pts',(2.14727864795285,-4.8332324334089,6.10820294719664));
#44972=CARTESIAN_POINT('Ctrl Pts',(4.19743676434218,-3.21752481834385,6.18757483725004));
#44973=CARTESIAN_POINT('Ctrl Pts',(4.98922373212554,-1.36879789494917,6.24872823997214));
#44974=CARTESIAN_POINT('Ctrl Pts',(5.0736256122357,-0.262783913782733,6.28342434600977));
#44975=CARTESIAN_POINT('Ctrl Pts',(5.07339692231655,-0.000119345805453183,
6.29166315536293));
#44976=CARTESIAN_POINT('Ctrl Pts',(5.07326256235615,8.63409482398936E-5,
5.20833684463708));
#44977=CARTESIAN_POINT('Ctrl Pts',(5.07345742030602,0.321133824030879,5.21840614426627));
#44978=CARTESIAN_POINT('Ctrl Pts',(4.96462985132702,1.48560987617541,5.25493274057992));
#44979=CARTESIAN_POINT('Ctrl Pts',(4.08394322312664,3.36040906700182,5.31791663357805));
#44980=CARTESIAN_POINT('Ctrl Pts',(1.979268164295,4.90443053586431,5.39728852363145));
#44981=CARTESIAN_POINT('Ctrl Pts',(-0.607552238323124,5.25374358196311,
5.47666041368485));
#44982=CARTESIAN_POINT('Ctrl Pts',(-3.04637426047979,4.32325632045987,5.55603230373826));
#44983=CARTESIAN_POINT('Ctrl Pts',(-4.74310625581864,2.33963338865815,5.63540419379165));
#44984=CARTESIAN_POINT('Ctrl Pts',(-5.28442806592769,-0.213919057930008,
5.71477608384507));
#44985=CARTESIAN_POINT('Ctrl Pts',(-4.53847489605989,-2.71536129550824,
5.79414797389846));
#44986=CARTESIAN_POINT('Ctrl Pts',(-2.68695928725567,-4.55534753185094,
5.87351986395187));
#44987=CARTESIAN_POINT('Ctrl Pts',(-0.180906343559476,-5.28566119252549,
5.95289175400528));
#44988=CARTESIAN_POINT('Ctrl Pts',(2.36921498499841,-4.72839948631341,6.03226364405867));
#44989=CARTESIAN_POINT('Ctrl Pts',(4.3422007873791,-3.01931013137013,6.1116355341121));
#44990=CARTESIAN_POINT('Ctrl Pts',(5.01896602830084,-1.21167525394927,6.17032660097155));
#44991=CARTESIAN_POINT('Ctrl Pts',(5.07382205657331,-0.184267811620037,
6.20256037114655));
#44992=CARTESIAN_POINT('Ctrl Pts',(5.07363207848188,-0.000130424372061667,
6.20833684463708));
#44993=CARTESIAN_POINT('Origin',(0.,0.,-2.20833684463713));
#44994=CARTESIAN_POINT('',(5.07402907570203,-1.82827833135855E-5,4.20833684463708));
#44995=CARTESIAN_POINT('',(5.07389532565035,-9.07960786141478E-5,4.29166315536292));
#44996=CARTESIAN_POINT('',(5.0736,-1.85409460923845E-12,-2.20833684463713));
#44997=CARTESIAN_POINT('Ctrl Pts',(5.07389532565035,-9.07960786142303E-5,
4.29166315536292));
#44998=CARTESIAN_POINT('Ctrl Pts',(5.07327433146367,0.747403143972462,4.3151158922492));
#44999=CARTESIAN_POINT('Ctrl Pts',(4.7173237838915,2.33872520323751,4.36502592581995));
#45000=CARTESIAN_POINT('Ctrl Pts',(3.11590430478523,4.27341569598967,4.44139325607517));
#45001=CARTESIAN_POINT('Ctrl Pts',(0.692451950200399,5.24322912373411,4.52076514612856));
#45002=CARTESIAN_POINT('Ctrl Pts',(-1.89968016673685,4.93580354262775,4.60013703618198));
#45003=CARTESIAN_POINT('Ctrl Pts',(-4.02905439992773,3.42602714375309,4.67950892623537));
#45004=CARTESIAN_POINT('Ctrl Pts',(-5.17695989945686,1.08167811604265,4.75888081628878));
#45005=CARTESIAN_POINT('Ctrl Pts',(-5.06376942648468,-1.5261653064819,4.83825270634218));
#45006=CARTESIAN_POINT('Ctrl Pts',(-3.71705592968434,-3.76223823845706,
4.91762459639559));
#45007=CARTESIAN_POINT('Ctrl Pts',(-1.46487583597662,-5.08183826311717,
4.996996486449));
#45008=CARTESIAN_POINT('Ctrl Pts',(1.14414476892732,-5.16351373534013,5.07636837650239));
#45009=CARTESIAN_POINT('Ctrl Pts',(3.47445424064207,-3.98736869087803,5.15574026655581));
#45010=CARTESIAN_POINT('Ctrl Pts',(4.81617424358115,-2.04572091909076,5.22750519284264));
#45011=CARTESIAN_POINT('Ctrl Pts',(5.07289029565433,-0.600829257314202,
5.27281282244502));
#45012=CARTESIAN_POINT('Ctrl Pts',(5.07345306532775,0.000126183674940827,
5.29166315536293));
#45013=CARTESIAN_POINT('Ctrl Pts',(5.07402907570203,-1.82827833134858E-5,
4.20833684463708));
#45014=CARTESIAN_POINT('Ctrl Pts',(5.07386028856637,0.825892891192897,4.23425191738599));
#45015=CARTESIAN_POINT('Ctrl Pts',(4.65820682968666,2.49515959185088,4.28662428681936));
#45016=CARTESIAN_POINT('Ctrl Pts',(2.91427384097298,4.41338297988409,4.36545395293721));
#45017=CARTESIAN_POINT('Ctrl Pts',(0.44843468320075,5.26971039832481,4.44482584299061));
#45018=CARTESIAN_POINT('Ctrl Pts',(-2.12664217080585,4.84234802803972,4.52419773304401));
#45019=CARTESIAN_POINT('Ctrl Pts',(-4.18367369924674,3.23540039647972,4.60356962309741));
#45020=CARTESIAN_POINT('Ctrl Pts',(-5.22157157495578,0.840316389774564,
4.68294151315082));
#45021=CARTESIAN_POINT('Ctrl Pts',(-4.98750617275825,-1.75946682947089,
4.76231340320422));
#45022=CARTESIAN_POINT('Ctrl Pts',(-3.53849530653447,-3.93064782357102,
4.84168529325762));
#45023=CARTESIAN_POINT('Ctrl Pts',(-1.22751481596538,-5.14433170819062,
4.92105718331103));
#45024=CARTESIAN_POINT('Ctrl Pts',(1.3824855667149,-5.10486777548008,5.00042907336443));
#45025=CARTESIAN_POINT('Ctrl Pts',(3.65571552542333,-3.82186935209575,5.07980096341784));
#45026=CARTESIAN_POINT('Ctrl Pts',(4.86300805809873,-1.88874478353847,5.14910355384205));
#45027=CARTESIAN_POINT('Ctrl Pts',(5.07294542694196,-0.522425194224716,
5.1919488475818));
#45028=CARTESIAN_POINT('Ctrl Pts',(5.07326256235615,8.63409482398936E-5,
5.20833684463708));
#45029=CARTESIAN_POINT('Origin',(0.,0.,-2.20833684463713));
#45030=CARTESIAN_POINT('',(5.0732079990561,-5.95000919163813E-5,3.20833684463708));
#45031=CARTESIAN_POINT('',(5.07316685382493,1.14989646604178E-5,3.29166315536292));
#45032=CARTESIAN_POINT('',(5.0736,-1.85409460923845E-12,-2.20833684463713));
#45033=CARTESIAN_POINT('Ctrl Pts',(5.07316685382493,1.14989646600797E-5,
3.29166315536292));
#45034=CARTESIAN_POINT('Ctrl Pts',(5.07319917633903,0.409460216043812,3.30450436868445));
#45035=CARTESIAN_POINT('Ctrl Pts',(4.923282999623,1.66249023374937,3.34380287869045));
#45036=CARTESIAN_POINT('Ctrl Pts',(3.90287063578958,3.56910943340232,3.40955868538091));
#45037=CARTESIAN_POINT('Ctrl Pts',(1.7204303939291,5.00110593838552,3.48893057543432));
#45038=CARTESIAN_POINT('Ctrl Pts',(-0.881102883784432,5.21484410653825,
3.56830246548772));
#45039=CARTESIAN_POINT('Ctrl Pts',(-3.26800144929621,4.15825779319991,3.64767435554113));
#45040=CARTESIAN_POINT('Ctrl Pts',(-4.85882209535798,2.08872908558557,3.72704624559453));
#45041=CARTESIAN_POINT('Ctrl Pts',(-5.2660444338108,-0.489609403954008,
3.80641813564793));
#45042=CARTESIAN_POINT('Ctrl Pts',(-4.39047000437897,-2.94868012642242,
3.88579002570134));
#45043=CARTESIAN_POINT('Ctrl Pts',(-2.44538680002092,-4.68945889688708,
3.96516191575474));
#45044=CARTESIAN_POINT('Ctrl Pts',(0.0953872160503347,-5.28789586001125,
4.04453380580815));
#45045=CARTESIAN_POINT('Ctrl Pts',(2.61292511742776,-4.59821309619564,4.12390569586154));
#45046=CARTESIAN_POINT('Ctrl Pts',(4.49396024381142,-2.78841580011883,4.20327758591496));
#45047=CARTESIAN_POINT('Ctrl Pts',(5.04793652990732,-1.03482867897542,4.25919673908208));
#45048=CARTESIAN_POINT('Ctrl Pts',(5.07397488200138,-0.0958531905725829,
4.28865859556473));
#45049=CARTESIAN_POINT('Ctrl Pts',(5.07389532565035,-9.07960786142303E-5,
4.29166315536292));
#45050=CARTESIAN_POINT('Ctrl Pts',(5.0732079990561,-5.95000919163813E-5,
3.20833684463708));
#45051=CARTESIAN_POINT('Ctrl Pts',(5.07300669336618,0.487890744857983,3.22364039382123));
#45052=CARTESIAN_POINT('Ctrl Pts',(4.88232843229471,1.81957999791209,3.26540123968986));
#45053=CARTESIAN_POINT('Ctrl Pts',(3.73307055280206,3.74634830136122,3.33361938224296));
#45054=CARTESIAN_POINT('Ctrl Pts',(1.48653991852054,5.07554336184363,3.41299127229636));
#45055=CARTESIAN_POINT('Ctrl Pts',(-1.12210854951228,5.16834729390561,3.49236316234976));
#45056=CARTESIAN_POINT('Ctrl Pts',(-3.45741385862906,4.00215326511488,3.57173505240317));
#45057=CARTESIAN_POINT('Ctrl Pts',(-4.95050080463958,1.86104355955814,3.65110694245657));
#45058=CARTESIAN_POINT('Ctrl Pts',(-5.23765671238755,-0.733412237756895,
3.73047883250997));
#45059=CARTESIAN_POINT('Ctrl Pts',(-4.24893103835441,-3.14921043733482,
3.80985072256337));
#45060=CARTESIAN_POINT('Ctrl Pts',(-2.22517516822744,-4.79786794503704,
3.88922261261678));
#45061=CARTESIAN_POINT('Ctrl Pts',(0.340628447538026,-5.2777754412288,3.96859450267018));
#45062=CARTESIAN_POINT('Ctrl Pts',(2.82345572745151,-4.472028522095,4.04796639272359));
#45063=CARTESIAN_POINT('Ctrl Pts',(4.61849544177105,-2.57690535364612,4.12733828277699));
#45064=CARTESIAN_POINT('Ctrl Pts',(5.06972869559084,-0.877769583505955,
4.18079510008149));
#45065=CARTESIAN_POINT('Ctrl Pts',(5.07403260725396,-0.0172989136932101,
4.20779462070152));
#45066=CARTESIAN_POINT('Ctrl Pts',(5.07402907570203,-1.82827833134858E-5,
4.20833684463708));
#45067=CARTESIAN_POINT('Origin',(0.,0.,-2.20833684463713));
#45068=CARTESIAN_POINT('',(5.07374102492394,0.00012139426775859,2.20833684463708));
#45069=CARTESIAN_POINT('',(5.07395289332891,7.08096438841769E-5,2.29166315536292));
#45070=CARTESIAN_POINT('',(5.0736,-1.85409460923845E-12,-2.20833684463713));
#45071=CARTESIAN_POINT('Ctrl Pts',(5.07395289332891,7.08096438841854E-5,
2.29166315536292));
#45072=CARTESIAN_POINT('Ctrl Pts',(5.07400149993288,0.0711339346777274,
2.2938928451197));
#45073=CARTESIAN_POINT('Ctrl Pts',(5.05519150559033,0.985399910949532,2.32257983156095));
#45074=CARTESIAN_POINT('Ctrl Pts',(4.53420692607935,2.72248212093367,2.37772411468667));
#45075=CARTESIAN_POINT('Ctrl Pts',(2.67980532059554,4.5595597146017,2.45709600474007));
#45076=CARTESIAN_POINT('Ctrl Pts',(0.172609070663326,5.28593865420646,2.53646789479348));
#45077=CARTESIAN_POINT('Ctrl Pts',(-2.37663436681889,4.72467463787357,2.61583978484688));
#45078=CARTESIAN_POINT('Ctrl Pts',(-4.34693493313492,3.01249033764445,2.69521167490029));
#45079=CARTESIAN_POINT('Ctrl Pts',(-5.25833177151656,0.56647005919948,2.77458356495369));
#45080=CARTESIAN_POINT('Ctrl Pts',(-4.88881062947673,-2.01754107180632,
2.85395545500709));
#45081=CARTESIAN_POINT('Ctrl Pts',(-3.32838603929513,-4.11008366347149,
2.93332734506049));
#45082=CARTESIAN_POINT('Ctrl Pts',(-0.957173977198773,-5.20141897223089,
3.0126992351139));
#45083=CARTESIAN_POINT('Ctrl Pts',(1.64720354707453,-5.02570013250045,3.0920711251673));
#45084=CARTESIAN_POINT('Ctrl Pts',(3.85032593330369,-3.62573186469146,3.1714430152207));
#45085=CARTESIAN_POINT('Ctrl Pts',(4.91082792455161,-1.71192991859137,3.23797369195258));
#45086=CARTESIAN_POINT('Ctrl Pts',(5.07313258089171,-0.434144349474542,
3.27804707199999));
#45087=CARTESIAN_POINT('Ctrl Pts',(5.07316685382493,1.14989646600797E-5,
3.29166315536292));
#45088=CARTESIAN_POINT('Ctrl Pts',(5.07374102492394,0.000121394267758555,
2.20833684463708));
#45089=CARTESIAN_POINT('Ctrl Pts',(5.07389186228029,0.149680441629337,2.21302887025649));
#45090=CARTESIAN_POINT('Ctrl Pts',(5.03086461164817,1.14248345247706,2.24417819256036));
#45091=CARTESIAN_POINT('Ctrl Pts',(4.40300813596794,2.92992503348825,2.3017848115487));
#45092=CARTESIAN_POINT('Ctrl Pts',(2.46536820371062,4.67898503603904,2.38115670160211));
#45093=CARTESIAN_POINT('Ctrl Pts',(-0.0728299659737919,5.28825464055465,
2.46052859165552));
#45094=CARTESIAN_POINT('Ctrl Pts',(-2.59328691715172,4.60931711999155,2.53990048170891));
#45095=CARTESIAN_POINT('Ctrl Pts',(-4.4820249154556,2.80756015154502,2.61927237176233));
#45096=CARTESIAN_POINT('Ctrl Pts',(-5.27895156514789,0.321887744613165,
2.69864426181572));
#45097=CARTESIAN_POINT('Ctrl Pts',(-4.7899372983315,-2.2421958044211,2.77801615186913));
#45098=CARTESIAN_POINT('Ctrl Pts',(-3.13410490798781,-4.26008541851404,
2.85738804192253));
#45099=CARTESIAN_POINT('Ctrl Pts',(-0.714811499281904,-5.2402276541964,
2.93675993197593));
#45100=CARTESIAN_POINT('Ctrl Pts',(1.8786084084407,-4.94386203236353,3.01613182202934));
#45101=CARTESIAN_POINT('Ctrl Pts',(4.01440346609632,-3.44318256249998,3.09550371208274));
#45102=CARTESIAN_POINT('Ctrl Pts',(4.9490470546202,-1.55481288423713,3.15957205295199));
#45103=CARTESIAN_POINT('Ctrl Pts',(5.07335471749433,-0.355694245953322,
3.19718309713677));
#45104=CARTESIAN_POINT('Ctrl Pts',(5.0732079990561,-5.95000919163813E-5,
3.20833684463708));
#45105=CARTESIAN_POINT('Origin',(0.,0.,-2.20833684463713));
#45106=CARTESIAN_POINT('',(5.07361762168166,-0.000130982038957922,1.20833684463708));
#45107=CARTESIAN_POINT('',(5.07338480805012,-0.000117445791330803,1.29166315536292));
#45108=CARTESIAN_POINT('',(5.0736,-1.85409460923845E-12,-2.20833684463713));
#45109=CARTESIAN_POINT('Ctrl Pts',(5.07338480805012,-0.000117445791331001,
1.29166315536292));
#45110=CARTESIAN_POINT('Ctrl Pts',(5.07289281667254,0.576157106237108,1.30973861823942));
#45111=CARTESIAN_POINT('Ctrl Pts',(4.83135991405541,1.99633436079896,1.35427137780039));
#45112=CARTESIAN_POINT('Ctrl Pts',(3.53232089954478,3.93619745533352,1.42526143404583));
#45113=CARTESIAN_POINT('Ctrl Pts',(1.21943810235538,5.14625223481536,1.50463332409923));
#45114=CARTESIAN_POINT('Ctrl Pts',(-1.39049711694202,5.10269135980955,1.58400521415263));
#45115=CARTESIAN_POINT('Ctrl Pts',(-3.66171031660135,3.81612616476449,1.66337710420604));
#45116=CARTESIAN_POINT('Ctrl Pts',(-5.04093898807,1.59996108251987,1.74274899425944));
#45117=CARTESIAN_POINT('Ctrl Pts',(-5.19220608004013,-1.00595097780601,
1.82212088431284));
#45118=CARTESIAN_POINT('Ctrl Pts',(-4.07866326363067,-3.3668156066614,1.90149277436625));
#45119=CARTESIAN_POINT('Ctrl Pts',(-1.97156710418735,-4.90753140600723,
1.98086466441965));
#45120=CARTESIAN_POINT('Ctrl Pts',(0.61579843785608,-5.25278341751101,2.06023655447306));
#45121=CARTESIAN_POINT('Ctrl Pts',(3.0531568434793,-4.31846901533485,2.13960844452646));
#45122=CARTESIAN_POINT('Ctrl Pts',(4.69919647653223,-2.38798317189229,2.21675064482308));
#45123=CARTESIAN_POINT('Ctrl Pts',(5.07342473837308,-0.772094669942323,
2.26743554843524));
#45124=CARTESIAN_POINT('Ctrl Pts',(5.07395289332891,7.08096438841854E-5,
2.29166315536292));
#45125=CARTESIAN_POINT('Ctrl Pts',(5.07361762168166,-0.000130982038957766,
1.20833684463708));
#45126=CARTESIAN_POINT('Ctrl Pts',(5.07294327622754,0.654560436527497,1.2288746433762));
#45127=CARTESIAN_POINT('Ctrl Pts',(4.78166373276894,2.15322402421039,1.2758697387998));
#45128=CARTESIAN_POINT('Ctrl Pts',(3.34588798700519,4.09584848370755,1.34932213090786));
#45129=CARTESIAN_POINT('Ctrl Pts',(0.979352771366438,5.19728867487042,1.42869402096127));
#45130=CARTESIAN_POINT('Ctrl Pts',(-1.6257506180571,5.03268082057239,1.50806591101467));
#45131=CARTESIAN_POINT('Ctrl Pts',(-3.83482475204895,3.64212307300266,1.58743780106807));
#45132=CARTESIAN_POINT('Ctrl Pts',(-5.10974406648874,1.36435219862418,1.66680969112148));
#45133=CARTESIAN_POINT('Ctrl Pts',(-5.13994103560183,-1.2457718471981,1.74618158117488));
#45134=CARTESIAN_POINT('Ctrl Pts',(-3.91805974601548,-3.55242863073578,
1.82555347122828));
#45135=CARTESIAN_POINT('Ctrl Pts',(-1.74174777450957,-4.99372166181597,
1.90492536128169));
#45136=CARTESIAN_POINT('Ctrl Pts',(0.858850099431454,-5.21855515011689,
1.98429725133509));
#45137=CARTESIAN_POINT('Ctrl Pts',(3.25023399025869,-4.17216015459491,2.0636691413885));
#45138=CARTESIAN_POINT('Ctrl Pts',(4.75530658628425,-2.2313729735679,2.13834900582249));
#45139=CARTESIAN_POINT('Ctrl Pts',(5.0730413237258,-0.693650010686127,2.18657157357202));
#45140=CARTESIAN_POINT('Ctrl Pts',(5.07374102492394,0.000121394267758555,
2.20833684463708));
#45141=CARTESIAN_POINT('Origin',(0.,0.,-2.20833684463713));
#45142=CARTESIAN_POINT('',(5.07327550687406,0.000108476183186546,0.208336844637077));
#45143=CARTESIAN_POINT('',(5.07346622253939,0.000127574377019038,0.291663155362924));
#45144=CARTESIAN_POINT('',(5.0736,-1.85409460923845E-12,-2.20833684463713));
#45145=CARTESIAN_POINT('',(1.3130361863565,-4.90075024188322,0.));
#45146=CARTESIAN_POINT('Ctrl Pts',(1.3130361863565,-4.90075024188322,0.));
#45147=CARTESIAN_POINT('Ctrl Pts',(2.12771778283771,-4.68247622999897,0.0264572966844678));
#45148=CARTESIAN_POINT('Ctrl Pts',(3.64531650851188,-3.8320815322798,0.0793718900534037));
#45149=CARTESIAN_POINT('Ctrl Pts',(4.86042636846397,-1.89775322538081,0.148817504932429));
#45150=CARTESIAN_POINT('Ctrl Pts',(5.07294944175775,-0.526932428119567,
0.191805823126987));
#45151=CARTESIAN_POINT('Ctrl Pts',(5.07327550687406,0.000108476183186372,
0.208336844637077));
#45152=CARTESIAN_POINT('',(-1.31317395760259,-4.90115117757553,2.08166817117217E-16));
#45153=CARTESIAN_POINT('Origin',(0.,0.,0.));
#45154=CARTESIAN_POINT('Ctrl Pts',(-1.31317395760259,-4.90115117757553,
2.32154790183459E-16));
#45155=CARTESIAN_POINT('Ctrl Pts',(-0.533836595431888,-5.10962665469163,
0.025313101045988));
#45156=CARTESIAN_POINT('Ctrl Pts',(1.16384881260007,-5.14969078544564,0.0770834987764434));
#45157=CARTESIAN_POINT('Ctrl Pts',(3.46369715057722,-3.99673439595713,0.155311193191368));
#45158=CARTESIAN_POINT('Ctrl Pts',(4.8133239766203,-2.05483010796368,0.22721914393302));
#45159=CARTESIAN_POINT('Ctrl Pts',(5.0728909576883,-0.605381739016801,0.272669797990206));
#45160=CARTESIAN_POINT('Ctrl Pts',(5.07346622253938,0.000127574377019116,
0.291663155362924));
#45161=CARTESIAN_POINT('Origin',(4.45462538595717E-16,-1.65775395963113E-16,
40.));
#45162=CARTESIAN_POINT('Ctrl Pts',(3.43378788736169,2.9358415841302,40.));
#45163=CARTESIAN_POINT('Ctrl Pts',(3.52814292550769,2.83820823955091,40.));
#45164=CARTESIAN_POINT('Ctrl Pts',(3.61787392647867,2.73637499985595,40.));
#45165=CARTESIAN_POINT('Ctrl Pts',(3.7028436241849,2.63075402506017,40.));
#45166=CARTESIAN_POINT('Ctrl Pts',(3.78889648523297,2.52378663182211,40.));
#45167=CARTESIAN_POINT('Ctrl Pts',(3.87006637156126,2.41293377092847,40.));
#45168=CARTESIAN_POINT('Ctrl Pts',(3.94617716449749,2.2985820569619,40.));
#45169=CARTESIAN_POINT('Ctrl Pts',(3.98452054291682,2.24097352507873,40.));
#45170=CARTESIAN_POINT('Ctrl Pts',(4.02157936104048,2.18247639180456,40.));
#45171=CARTESIAN_POINT('Ctrl Pts',(4.0573273224032,2.12313686354418,40.));
#45172=CARTESIAN_POINT('Ctrl Pts',(4.07057108419318,2.10115299237913,40.));
#45173=CARTESIAN_POINT('Ctrl Pts',(4.08363549665298,2.07905229886435,40.));
#45174=CARTESIAN_POINT('Ctrl Pts',(4.09651028112638,2.05685278711327,40.));
#45175=CARTESIAN_POINT('Ctrl Pts',(4.16636767341313,1.93640028523473,40.));
#45176=CARTESIAN_POINT('Ctrl Pts',(4.23070798356748,1.81293936852798,40.));
#45177=CARTESIAN_POINT('Ctrl Pts',(4.28936081037521,1.68687424953695,40.));
#45178=CARTESIAN_POINT('Ctrl Pts',(4.34350578332916,1.57049806053275,40.));
#45179=CARTESIAN_POINT('Ctrl Pts',(4.39280381894615,1.45190174917925,40.));
#45180=CARTESIAN_POINT('Ctrl Pts',(4.4370895395389,1.33137973638483,40.));
#45181=CARTESIAN_POINT('Ctrl Pts',(4.45048806014006,1.29491613932226,40.));
#45182=CARTESIAN_POINT('Ctrl Pts',(4.46342755329992,1.25827614359673,40.));
#45183=CARTESIAN_POINT('Ctrl Pts',(4.47590283035858,1.22146759434429,40.));
#45184=CARTESIAN_POINT('Ctrl Pts',(4.48543045669819,1.19335614625929,40.));
#45185=CARTESIAN_POINT('Ctrl Pts',(4.49468731429383,1.16514638329788,40.));
#45186=CARTESIAN_POINT('Ctrl Pts',(4.50367097326761,1.13684175481395,40.));
#45187=CARTESIAN_POINT('Ctrl Pts',(4.50984234488601,1.11739774192287,40.));
#45188=CARTESIAN_POINT('Ctrl Pts',(4.51588427541961,1.09791040265649,40.));
#45189=CARTESIAN_POINT('Ctrl Pts',(4.52179265714445,1.0783924896528,40.));
#45190=CARTESIAN_POINT('Ctrl Pts',(4.53324480098953,1.04056115821829,40.));
#45191=CARTESIAN_POINT('Ctrl Pts',(4.54419899621228,1.00260320591424,40.));
#45192=CARTESIAN_POINT('Ctrl Pts',(4.5546518960517,0.964527761093808,40.));
#45193=CARTESIAN_POINT('Ctrl Pts',(4.59117593379611,0.831486307992675,40.));
#45194=CARTESIAN_POINT('Ctrl Pts',(4.62158314424656,0.697012525339414,40.));
#45195=CARTESIAN_POINT('Ctrl Pts',(4.64596931935994,0.561539349137144,40.));
#45196=CARTESIAN_POINT('Ctrl Pts',(4.67073918176772,0.42393466456182,40.));
#45197=CARTESIAN_POINT('Ctrl Pts',(4.68929722659476,0.28529820513645,40.));
#45198=CARTESIAN_POINT('Ctrl Pts',(4.70169535323682,0.146060437529888,40.));
#45199=CARTESIAN_POINT('Ctrl Pts',(4.71417778478848,0.00587587951314419,
40.));
#45200=CARTESIAN_POINT('Ctrl Pts',(4.7204163646451,-0.134918963378981,40.));
#45201=CARTESIAN_POINT('Ctrl Pts',(4.72041312729179,-0.275897046739804,
40.));
#45202=CARTESIAN_POINT('Ctrl Pts',(4.72041101510801,-0.367877004659711,
40.));
#45203=CARTESIAN_POINT('Ctrl Pts',(4.71775084452937,-0.459935190334389,
40.));
#45204=CARTESIAN_POINT('Ctrl Pts',(4.71242122767243,-0.55195336772424,40.));
#45205=CARTESIAN_POINT('Ctrl Pts',(4.71074982773409,-0.580810822236322,
40.));
#45206=CARTESIAN_POINT('Ctrl Pts',(4.70881582061262,-0.609664336690085,
40.));
#45207=CARTESIAN_POINT('Ctrl Pts',(4.70661866095158,-0.638510242454293,
40.));
#45208=CARTESIAN_POINT('Ctrl Pts',(4.70521659891363,-0.65691752988966,40.));
#45209=CARTESIAN_POINT('Ctrl Pts',(4.70370712995809,-0.675324500804579,
40.));
#45210=CARTESIAN_POINT('Ctrl Pts',(4.70209092940465,-0.693720810758238,
40.));
#45211=CARTESIAN_POINT('Ctrl Pts',(4.68953110086222,-0.836682337618008,
40.));
#45212=CARTESIAN_POINT('Ctrl Pts',(4.67055276432277,-0.978761795279802,
40.));
#45213=CARTESIAN_POINT('Ctrl Pts',(4.64522498551854,-1.11951304986637,40.));
#45214=CARTESIAN_POINT('Ctrl Pts',(4.63006091029742,-1.20378268237205,40.));
#45215=CARTESIAN_POINT('Ctrl Pts',(4.61261985737539,-1.28757653832611,40.));
#45216=CARTESIAN_POINT('Ctrl Pts',(4.59290787692688,-1.37080047994428,40.));
#45217=CARTESIAN_POINT('Ctrl Pts',(4.56017758990635,-1.5089876856012,40.));
#45218=CARTESIAN_POINT('Ctrl Pts',(4.52118921321033,-1.64560413309505,40.));
#45219=CARTESIAN_POINT('Ctrl Pts',(4.47619425969956,-1.78030079004358,40.));
#45220=CARTESIAN_POINT('Ctrl Pts',(4.43085717885509,-1.91602163758472,40.));
#45221=CARTESIAN_POINT('Ctrl Pts',(4.3794215892058,-2.04979410792511,40.));
#45222=CARTESIAN_POINT('Ctrl Pts',(4.32209322112883,-2.18124988516394,40.));
#45223=CARTESIAN_POINT('Ctrl Pts',(4.29589299313303,-2.24132784395735,40.));
#45224=CARTESIAN_POINT('Ctrl Pts',(4.26846127047772,-2.30092169976294,40.));
#45225=CARTESIAN_POINT('Ctrl Pts',(4.23981435864377,-2.35999488119432,40.));
#45226=CARTESIAN_POINT('Ctrl Pts',(4.22808815540088,-2.38417564230685,40.));
#45227=CARTESIAN_POINT('Ctrl Pts',(4.21615831686625,-2.40826914901153,40.));
#45228=CARTESIAN_POINT('Ctrl Pts',(4.20402586547368,-2.43227283763382,40.));
#45229=CARTESIAN_POINT('Ctrl Pts',(4.19226175293326,-2.45554777896271,40.));
#45230=CARTESIAN_POINT('Ctrl Pts',(4.18030467857245,-2.47874278381504,40.));
#45231=CARTESIAN_POINT('Ctrl Pts',(4.16817016036066,-2.50182817485463,40.));
#45232=CARTESIAN_POINT('Ctrl Pts',(4.10062993280007,-2.63032050861895,40.));
#45233=CARTESIAN_POINT('Ctrl Pts',(4.02752679248241,-2.75556160907446,40.));
#45234=CARTESIAN_POINT('Ctrl Pts',(3.94914189359867,-2.87720021634157,40.));
#45235=CARTESIAN_POINT('Ctrl Pts',(3.87013649228652,-2.99980172656921,40.));
#45236=CARTESIAN_POINT('Ctrl Pts',(3.78576510402317,-3.11874421706065,40.));
#45237=CARTESIAN_POINT('Ctrl Pts',(3.69626453833047,-3.23365468399741,40.));
#45238=CARTESIAN_POINT('Ctrl Pts',(3.6256051940776,-3.3243747613366,40.));
#45239=CARTESIAN_POINT('Ctrl Pts',(3.55174784325694,-3.41258159925288,40.));
#45240=CARTESIAN_POINT('Ctrl Pts',(3.4747885470066,-3.49808125449705,40.));
#45241=CARTESIAN_POINT('Ctrl Pts',(3.37754842452615,-3.60611234824477,40.));
#45242=CARTESIAN_POINT('Ctrl Pts',(3.27535698426899,-3.70982288325437,40.));
#45243=CARTESIAN_POINT('Ctrl Pts',(3.16857103825032,-3.80899091582305,40.));
#45244=CARTESIAN_POINT('Ctrl Pts',(3.13709749914945,-3.83821919039451,40.));
#45245=CARTESIAN_POINT('Ctrl Pts',(3.10522459675968,-3.86705262006651,40.));
#45246=CARTESIAN_POINT('Ctrl Pts',(3.07296088810501,-3.89548488187744,40.));
#45247=CARTESIAN_POINT('Ctrl Pts',(3.05413623645007,-3.91207402945752,40.));
#45248=CARTESIAN_POINT('Ctrl Pts',(3.03517853882814,-3.92852660249152,40.));
#45249=CARTESIAN_POINT('Ctrl Pts',(3.01608945850777,-3.94484129509693,40.));
#45250=CARTESIAN_POINT('Ctrl Pts',(3.00324987792049,-3.95581478396849,40.));
#45251=CARTESIAN_POINT('Ctrl Pts',(2.99035184084321,-3.96672500977969,40.));
#45252=CARTESIAN_POINT('Ctrl Pts',(2.97740348730282,-3.97756535219416,40.));
#45253=CARTESIAN_POINT('Ctrl Pts',(2.86172546572695,-4.07441082060052,40.));
#45254=CARTESIAN_POINT('Ctrl Pts',(2.74187291014631,-4.16582105105552,40.));
#45255=CARTESIAN_POINT('Ctrl Pts',(2.61830752500134,-4.25161650299712,40.));
#45256=CARTESIAN_POINT('Ctrl Pts',(2.49666368456262,-4.33607776416752,40.));
#45257=CARTESIAN_POINT('Ctrl Pts',(2.37142082394795,-4.41509790443455,40.));
#45258=CARTESIAN_POINT('Ctrl Pts',(2.24297630552737,-4.4884725438774,40.));
#45259=CARTESIAN_POINT('Ctrl Pts',(2.11148832986889,-4.56358577505025,40.));
#45260=CARTESIAN_POINT('Ctrl Pts',(1.97664462468232,-4.63278348201276,40.));
#45261=CARTESIAN_POINT('Ctrl Pts',(1.83883549494666,-4.69580305762063,40.));
#45262=CARTESIAN_POINT('Ctrl Pts',(1.701026365211,-4.7588226332285,40.));
#45263=CARTESIAN_POINT('Ctrl Pts',(1.56025109502399,-4.81566463443687,40.));
#45264=CARTESIAN_POINT('Ctrl Pts',(1.41687422066896,-4.86601447289837,40.));
#45265=CARTESIAN_POINT('Ctrl Pts',(1.38245545626202,-4.8781013539643,40.));
#45266=CARTESIAN_POINT('Ctrl Pts',(1.34788667776073,-4.88981384734562,40.));
#45267=CARTESIAN_POINT('Ctrl Pts',(1.31317395760249,-4.90115117757556,40.));
#45268=CARTESIAN_POINT('Ctrl Pts',(-1.31303618635638,-4.90075024188325,
40.));
#45269=CARTESIAN_POINT('Ctrl Pts',(-1.45437915259461,-4.85452838596849,
40.));
#45270=CARTESIAN_POINT('Ctrl Pts',(-1.59345673045457,-4.80203124199391,
40.));
#45271=CARTESIAN_POINT('Ctrl Pts',(-1.72991111250498,-4.74351762389719,
40.));
#45272=CARTESIAN_POINT('Ctrl Pts',(-1.86679415923463,-4.68482018816886,
40.));
#45273=CARTESIAN_POINT('Ctrl Pts',(-2.001038164382,-4.62006797676633,40.));
#45274=CARTESIAN_POINT('Ctrl Pts',(-2.1322557155067,-4.54947707893507,40.));
#45275=CARTESIAN_POINT('Ctrl Pts',(-2.19315308373731,-4.5167162183481,40.));
#45276=CARTESIAN_POINT('Ctrl Pts',(-2.25339817251141,-4.48269720490963,
40.));
#45277=CARTESIAN_POINT('Ctrl Pts',(-2.31294973629581,-4.44743875160342,
40.));
#45278=CARTESIAN_POINT('Ctrl Pts',(-2.33562884151057,-4.43401122558351,
40.));
#45279=CARTESIAN_POINT('Ctrl Pts',(-2.35820900730168,-4.42040290103079,
40.));
#45280=CARTESIAN_POINT('Ctrl Pts',(-2.38068262652232,-4.40661797963936,
40.));
#45281=CARTESIAN_POINT('Ctrl Pts',(-2.50650561756839,-4.32944037759069,
40.));
#45282=CARTESIAN_POINT('Ctrl Pts',(-2.62877991395688,-4.24686153480494,
40.));
#45283=CARTESIAN_POINT('Ctrl Pts',(-2.74713717330506,-4.15910670751388,
40.));
#45284=CARTESIAN_POINT('Ctrl Pts',(-2.86467013316358,-4.07196304898213,
40.));
#45285=CARTESIAN_POINT('Ctrl Pts',(-2.97834099898066,-3.97971476207056,
40.));
#45286=CARTESIAN_POINT('Ctrl Pts',(-3.08775357309594,-3.88254556003572,
40.));
#45287=CARTESIAN_POINT('Ctrl Pts',(-3.14513584653695,-3.8315844180802,40.));
#45288=CARTESIAN_POINT('Ctrl Pts',(-3.2013462077245,-3.77926917964798,40.));
#45289=CARTESIAN_POINT('Ctrl Pts',(-3.25632275100474,-3.72562292402786,
40.));
#45290=CARTESIAN_POINT('Ctrl Pts',(-3.27574922848208,-3.70666651617886,
40.));
#45291=CARTESIAN_POINT('Ctrl Pts',(-3.29502416873062,-3.6875411953518,40.));
#45292=CARTESIAN_POINT('Ctrl Pts',(-3.31412620910246,-3.66826697432299,
40.));
#45293=CARTESIAN_POINT('Ctrl Pts',(-3.34404060290358,-3.63808294021764,
40.));
#45294=CARTESIAN_POINT('Ctrl Pts',(-3.37353997543889,-3.60752519082335,
40.));
#45295=CARTESIAN_POINT('Ctrl Pts',(-3.40261591802411,-3.57659932769541,
40.));
#45296=CARTESIAN_POINT('Ctrl Pts',(-3.50164274205642,-3.47127204562902,
40.));
#45297=CARTESIAN_POINT('Ctrl Pts',(-3.59576101414824,-3.36167756876611,
40.));
#45298=CARTESIAN_POINT('Ctrl Pts',(-3.68480291336662,-3.24822038520781,
40.));
#45299=CARTESIAN_POINT('Ctrl Pts',(-3.77450749603108,-3.13391881043548,
40.));
#45300=CARTESIAN_POINT('Ctrl Pts',(-3.85906025603562,-3.01569612122462,
40.));
#45301=CARTESIAN_POINT('Ctrl Pts',(-3.93824649098464,-2.893935566612,40.));
#45302=CARTESIAN_POINT('Ctrl Pts',(-4.01670520549023,-2.7732936823433,40.));
#45303=CARTESIAN_POINT('Ctrl Pts',(-4.08989581732523,-2.64917791019356,
40.));
#45304=CARTESIAN_POINT('Ctrl Pts',(-4.15756259897637,-2.52194215997081,
40.));
#45305=CARTESIAN_POINT('Ctrl Pts',(-4.20177691057784,-2.43880474793609,
40.));
#45306=CARTESIAN_POINT('Ctrl Pts',(-4.24363187369716,-2.35433490941293,
40.));
#45307=CARTESIAN_POINT('Ctrl Pts',(-4.2830443332661,-2.26862918510464,40.));
#45308=CARTESIAN_POINT('Ctrl Pts',(-4.30136127527663,-2.22879744663171,
40.));
#45309=CARTESIAN_POINT('Ctrl Pts',(-4.31915051766851,-2.18869875186795,
40.));
#45310=CARTESIAN_POINT('Ctrl Pts',(-4.33640298127534,-2.14834275431588,
40.));
#45311=CARTESIAN_POINT('Ctrl Pts',(-4.3436590160159,-2.13136984384344,40.));
#45312=CARTESIAN_POINT('Ctrl Pts',(-4.35081962128211,-2.11435240712678,
40.));
#45313=CARTESIAN_POINT('Ctrl Pts',(-4.35787943356684,-2.09730289812436,
40.));
#45314=CARTESIAN_POINT('Ctrl Pts',(-4.41262610226673,-1.96508920982698,
40.));
#45315=CARTESIAN_POINT('Ctrl Pts',(-4.46139597719794,-1.83076168016892,
40.));
#45316=CARTESIAN_POINT('Ctrl Pts',(-4.50399603348697,-1.69468832090704,
40.));
#45317=CARTESIAN_POINT('Ctrl Pts',(-4.527154798591,-1.62071445235899,40.));
#45318=CARTESIAN_POINT('Ctrl Pts',(-4.54848933959424,-1.54622425456777,
40.));
#45319=CARTESIAN_POINT('Ctrl Pts',(-4.56796247846724,-1.47127487515815,
40.));
#45320=CARTESIAN_POINT('Ctrl Pts',(-4.60386684913915,-1.33308398988268,
40.));
#45321=CARTESIAN_POINT('Ctrl Pts',(-4.633446346586,-1.19333212031901,40.));
#45322=CARTESIAN_POINT('Ctrl Pts',(-4.65669710227076,-1.05245525970538,
40.));
#45323=CARTESIAN_POINT('Ctrl Pts',(-4.67988218362711,-0.911976321350021,
40.));
#45324=CARTESIAN_POINT('Ctrl Pts',(-4.6967741641367,-0.770377936579903,
40.));
#45325=CARTESIAN_POINT('Ctrl Pts',(-4.70731777033656,-0.628096038990404,
40.));
#45326=CARTESIAN_POINT('Ctrl Pts',(-4.71196239382317,-0.565418637090442,
40.));
#45327=CARTESIAN_POINT('Ctrl Pts',(-4.71537442348699,-0.502608716141042,
40.));
#45328=CARTESIAN_POINT('Ctrl Pts',(-4.71754599609844,-0.439704378705418,
40.));
#45329=CARTESIAN_POINT('Ctrl Pts',(-4.71847271903558,-0.412859827415833,
40.));
#45330=CARTESIAN_POINT('Ctrl Pts',(-4.71917350957111,-0.385998089715844,
40.));
#45331=CARTESIAN_POINT('Ctrl Pts',(-4.71964765055488,-0.359122168611144,
40.));
#45332=CARTESIAN_POINT('Ctrl Pts',(-4.72007766112019,-0.334747709487924,
40.));
#45333=CARTESIAN_POINT('Ctrl Pts',(-4.72032117948226,-0.310357499793734,
40.));
#45334=CARTESIAN_POINT('Ctrl Pts',(-4.72037779701569,-0.28598141917232,
40.));
#45335=CARTESIAN_POINT('Ctrl Pts',(-4.72070503729545,-0.145091575346323,
40.));
#45336=CARTESIAN_POINT('Ctrl Pts',(-4.71479792201471,-0.00450394063596596,
40.));
#45337=CARTESIAN_POINT('Ctrl Pts',(-4.7026779767235,0.135364936808135,40.));
#45338=CARTESIAN_POINT('Ctrl Pts',(-4.6906385436001,0.274304672555548,40.));
#45339=CARTESIAN_POINT('Ctrl Pts',(-4.67246842821977,0.412535934949348,
40.));
#45340=CARTESIAN_POINT('Ctrl Pts',(-4.64813815685378,0.549644620304502,
40.));
#45341=CARTESIAN_POINT('Ctrl Pts',(-4.62922788638654,0.656209906177027,
40.));
#45342=CARTESIAN_POINT('Ctrl Pts',(-4.60659531784607,0.762097046731738,
40.));
#45343=CARTESIAN_POINT('Ctrl Pts',(-4.58020591978812,0.867104757427845,
40.));
#45344=CARTESIAN_POINT('Ctrl Pts',(-4.54608550784896,1.00287543085781,40.));
#45345=CARTESIAN_POINT('Ctrl Pts',(-4.5056856677851,1.13717725960422,40.));
#45346=CARTESIAN_POINT('Ctrl Pts',(-4.45916773762384,1.26960241773677,40.));
#45347=CARTESIAN_POINT('Ctrl Pts',(-4.44595800567878,1.30720729043101,40.));
#45348=CARTESIAN_POINT('Ctrl Pts',(-4.43225465907289,1.34466063579127,40.));
#45349=CARTESIAN_POINT('Ctrl Pts',(-4.41806080497834,1.381952618119,40.));
#45350=CARTESIAN_POINT('Ctrl Pts',(-4.41034395548629,1.40222735202608,40.));
#45351=CARTESIAN_POINT('Ctrl Pts',(-4.40248211604979,1.42245438558641,40.));
#45352=CARTESIAN_POINT('Ctrl Pts',(-4.39447575604619,1.44263210700853,40.));
#45353=CARTESIAN_POINT('Ctrl Pts',(-4.38774337392406,1.45959913458491,40.));
#45354=CARTESIAN_POINT('Ctrl Pts',(-4.38091020364865,1.47652766568619,40.));
#45355=CARTESIAN_POINT('Ctrl Pts',(-4.37398035764513,1.49340802308437,40.));
#45356=CARTESIAN_POINT('Ctrl Pts',(-4.32139777601335,1.62149352028206,40.));
#45357=CARTESIAN_POINT('Ctrl Pts',(-4.26319329324451,1.74695839038908,40.));
#45358=CARTESIAN_POINT('Ctrl Pts',(-4.19959993118347,1.86944841739778,40.));
#45359=CARTESIAN_POINT('Ctrl Pts',(-4.13606105752427,1.99183349185173,40.));
#45360=CARTESIAN_POINT('Ctrl Pts',(-4.06714208355231,2.1112494937512,40.));
#45361=CARTESIAN_POINT('Ctrl Pts',(-3.99303011697524,2.22731770598438,40.));
#45362=CARTESIAN_POINT('Ctrl Pts',(-3.9202059518248,2.34136906700981,40.));
#45363=CARTESIAN_POINT('Ctrl Pts',(-3.84236718991447,2.45218850722107,40.));
#45364=CARTESIAN_POINT('Ctrl Pts',(-3.75965485123955,2.55938335127685,40.));
#45365=CARTESIAN_POINT('Ctrl Pts',(-3.67819754057762,2.66495168429094,40.));
#45366=CARTESIAN_POINT('Ctrl Pts',(-3.59201299654429,2.76700506575445,40.));
#45367=CARTESIAN_POINT('Ctrl Pts',(-3.50120707213067,2.86512829543056,40.));
#45368=CARTESIAN_POINT('Ctrl Pts',(-3.47910751146495,2.88900867857677,40.));
#45369=CARTESIAN_POINT('Ctrl Pts',(-3.45673410716774,2.91265607078183,40.));
#45370=CARTESIAN_POINT('Ctrl Pts',(-3.43409108914464,2.93606647242288,40.));
#45371=CARTESIAN_POINT('Origin',(0.,0.,-2.20833684463713));
#45372=CARTESIAN_POINT('Ctrl Pts',(5.07346622253938,0.000127574377019116,
0.291663155362924));
#45373=CARTESIAN_POINT('Ctrl Pts',(5.07369228799229,0.238078384188188,0.299127094674674));
#45374=CARTESIAN_POINT('Ctrl Pts',(4.99899491470862,1.31934885093053,0.333048330670892));
#45375=CARTESIAN_POINT('Ctrl Pts',(4.24398161873799,3.15587819282154,0.393426863351577));
#45376=CARTESIAN_POINT('Ctrl Pts',(2.21764149317933,4.80135391043019,0.472798753404982));
#45377=CARTESIAN_POINT('Ctrl Pts',(-0.348912918530393,5.27723479734493,
0.552170643458385));
#45378=CARTESIAN_POINT('Ctrl Pts',(-2.83047200092439,4.46759066254957,0.631542533511789));
#45379=CARTESIAN_POINT('Ctrl Pts',(-4.62253485344812,2.56965255248809,0.710914423565193));
#45380=CARTESIAN_POINT('Ctrl Pts',(-5.28855819093304,0.045752121671659,
0.790286313618596));
#45381=CARTESIAN_POINT('Ctrl Pts',(-4.66630059499956,-2.48929308216644,
0.869658203672));
#45382=CARTESIAN_POINT('Ctrl Pts',(-2.90734243084918,-4.4179521825598,0.949030093725403));
#45383=CARTESIAN_POINT('Ctrl Pts',(-0.440162123945536,-5.27040781417518,
1.02840198377881));
#45384=CARTESIAN_POINT('Ctrl Pts',(2.1342407222512,-4.83900381899044,1.10777387383221));
#45385=CARTESIAN_POINT('Ctrl Pts',(4.18874724188064,-3.228829177505,1.18714576388562));
#45386=CARTESIAN_POINT('Ctrl Pts',(4.9873788651986,-1.37792482956251,1.24844219106252));
#45387=CARTESIAN_POINT('Ctrl Pts',(5.07361295102991,-0.267343660459586,
1.28328132155495));
#45388=CARTESIAN_POINT('Ctrl Pts',(5.07338480805012,-0.000117445791331001,
1.29166315536292));
#45389=CARTESIAN_POINT('Ctrl Pts',(5.07327550687406,0.000108476183186372,
0.208336844637077));
#45390=CARTESIAN_POINT('Ctrl Pts',(5.07347129707779,0.316577306682802,0.218263119811455));
#45391=CARTESIAN_POINT('Ctrl Pts',(4.96661393653962,1.47641857544861,0.254646691670301));
#45392=CARTESIAN_POINT('Ctrl Pts',(4.09299916691648,3.34943642687043,0.317487560213614));
#45393=CARTESIAN_POINT('Ctrl Pts',(1.99247705733062,4.89905044646781,0.396859450267019));
#45394=CARTESIAN_POINT('Ctrl Pts',(-0.593383061700938,5.2553763257097,0.476231340320422));
#45395=CARTESIAN_POINT('Ctrl Pts',(-3.03470961035893,4.33144609848054,0.555603230373826));
#45396=CARTESIAN_POINT('Ctrl Pts',(-4.73678060915323,2.35241593705463,0.634975120427228));
#45397=CARTESIAN_POINT('Ctrl Pts',(-5.28498604656423,-0.199673823356779,
0.714347010480634));
#45398=CARTESIAN_POINT('Ctrl Pts',(-4.5457786161601,-2.703114858517,0.793718900534037));
#45399=CARTESIAN_POINT('Ctrl Pts',(-2.69923061743508,-4.5480876646044,0.87309079058744));
#45400=CARTESIAN_POINT('Ctrl Pts',(-0.195155463808127,-5.28515396379925,
0.952462680640845));
#45401=CARTESIAN_POINT('Ctrl Pts',(2.35645883694709,-4.73476973691702,1.03183457069425));
#45402=CARTESIAN_POINT('Ctrl Pts',(4.33404513553918,-3.03100540392648,1.11120646074765));
#45403=CARTESIAN_POINT('Ctrl Pts',(5.01734225874463,-1.22080114526538,1.17004055206193));
#45404=CARTESIAN_POINT('Ctrl Pts',(5.0738119846015,-0.188829126190742,1.20241734669174));
#45405=CARTESIAN_POINT('Ctrl Pts',(5.07361762168166,-0.000130982038957766,
1.20833684463708));
#45406=CARTESIAN_POINT('Ctrl Pts',(-3.43378788736187,2.93584158412999,-1.38777878078145E-15));
#45407=CARTESIAN_POINT('Ctrl Pts',(-3.92183073605352,2.36502208507736,0.0264572966844665));
#45408=CARTESIAN_POINT('Ctrl Pts',(-4.60729903172261,0.975909964327098,
0.0793718900534022));
#45409=CARTESIAN_POINT('Ctrl Pts',(-4.51258247789853,-1.34695556252418,
0.158743780106806));
#45410=CARTESIAN_POINT('Ctrl Pts',(-3.3188765366808,-3.34104229843846,0.23811567016021));
#45411=CARTESIAN_POINT('Ctrl Pts',(-1.31656588610641,-4.52159485055713,
0.317487560213613));
#45412=CARTESIAN_POINT('Ctrl Pts',(1.00638734295355,-4.60052063353559,0.396859450267017));
#45413=CARTESIAN_POINT('Ctrl Pts',(3.08422378627015,-3.55886290155616,0.476231340320421));
#45414=CARTESIAN_POINT('Ctrl Pts',(4.41073058968579,-1.65022475069956,0.555603230373823));
#45415=CARTESIAN_POINT('Ctrl Pts',(4.66280353786907,0.660378394082181,0.634975120427229));
#45416=CARTESIAN_POINT('Ctrl Pts',(3.77902238214553,2.81012864743368,0.71434701048063));
#45417=CARTESIAN_POINT('Ctrl Pts',(1.9746826426622,4.27533046137772,0.793718900534036));
#45418=CARTESIAN_POINT('Ctrl Pts',(-0.310686955552407,4.69907511544172,
0.873090790587439));
#45419=CARTESIAN_POINT('Ctrl Pts',(-2.52037308462949,3.97813341921581,0.952462680640842));
#45420=CARTESIAN_POINT('Ctrl Pts',(-4.11610234038262,2.28812831500376,1.03183457069425));
#45421=CARTESIAN_POINT('Ctrl Pts',(-4.70915794841686,0.0407396420060994,
1.11120646074765));
#45422=CARTESIAN_POINT('Ctrl Pts',(-4.15507322474362,-2.21657281259016,
1.19057835080105));
#45423=CARTESIAN_POINT('Ctrl Pts',(-2.58882179654858,-3.93393319787912,
1.26995024085446));
#45424=CARTESIAN_POINT('Ctrl Pts',(-0.391939142907391,-4.69299607822649,
1.34932213090786));
#45425=CARTESIAN_POINT('Ctrl Pts',(1.90041903637464,-4.30885554699701,1.42869402096126));
#45426=CARTESIAN_POINT('Ctrl Pts',(3.72983933538439,-2.87508731801348,1.50806591101467));
#45427=CARTESIAN_POINT('Ctrl Pts',(4.65067903319439,-0.740954194967835,
1.58743780106807));
#45428=CARTESIAN_POINT('Ctrl Pts',(4.43862360995218,1.57367373662795,1.66680969112148));
#45429=CARTESIAN_POINT('Ctrl Pts',(3.1453293014661,3.50495822568453,1.74618158117488));
#45430=CARTESIAN_POINT('Ctrl Pts',(1.08583973646247,4.58244265094549,1.82555347122828));
#45431=CARTESIAN_POINT('Ctrl Pts',(-1.2381579844814,4.54365418850119,1.90492536128169));
#45432=CARTESIAN_POINT('Ctrl Pts',(-3.26054316123182,3.39804162347539,1.98429725133509));
#45433=CARTESIAN_POINT('Ctrl Pts',(-4.48866724088482,1.42467364012815,2.0636691413885));
#45434=CARTESIAN_POINT('Ctrl Pts',(-4.62336191621359,-0.895741688344198,
2.1430410314419));
#45435=CARTESIAN_POINT('Ctrl Pts',(-3.63181586235956,-2.99795632430514,
2.2224129214953));
#45436=CARTESIAN_POINT('Ctrl Pts',(-1.75556750333933,-4.36987543548745,
2.30178481154871));
#45437=CARTESIAN_POINT('Ctrl Pts',(0.548333213620371,-4.67730256316232,
2.38115670160211));
#45438=CARTESIAN_POINT('Ctrl Pts',(2.71866117345249,-3.84534913947276,2.46052859165552));
#45439=CARTESIAN_POINT('Ctrl Pts',(4.22672928908848,-2.07667717694978,2.53990048170891));
#45440=CARTESIAN_POINT('Ctrl Pts',(4.7051755056078,0.19786874923449,2.61927237176232));
#45441=CARTESIAN_POINT('Ctrl Pts',(4.03745138369107,2.42421428607854,2.69864426181572));
#45442=CARTESIAN_POINT('Ctrl Pts',(2.38621304145389,4.06002658874208,2.77801615186912));
#45443=CARTESIAN_POINT('Ctrl Pts',(0.153698484111727,4.70682540110399,2.85738804192253));
#45444=CARTESIAN_POINT('Ctrl Pts',(-2.11625668375435,4.20705196413855,2.93675993197593));
#45445=CARTESIAN_POINT('Ctrl Pts',(-3.87069640771252,2.68244998086038,3.01613182202934));
#45446=CARTESIAN_POINT('Ctrl Pts',(-4.68224305439313,0.504409119747013,
3.09550371208274));
#45447=CARTESIAN_POINT('Ctrl Pts',(-4.35320565699276,-1.79650468644612,
3.17487560213615));
#45448=CARTESIAN_POINT('Ctrl Pts',(-2.96373699720624,-3.65979392751662,
3.25424749218954));
#45449=CARTESIAN_POINT('Ctrl Pts',(-0.852308565020845,-4.63156546866054,
3.33361938224295));
#45450=CARTESIAN_POINT('Ctrl Pts',(1.46674034705061,-4.47509791343502,3.41299127229636));
#45451=CARTESIAN_POINT('Ctrl Pts',(3.42849455715522,-3.22850641195795,3.49236316234976));
#45452=CARTESIAN_POINT('Ctrl Pts',(4.55507508198081,-1.19545789470566,3.57173505240317));
#45453=CARTESIAN_POINT('Ctrl Pts',(4.57204939932356,1.12880151959577,3.65110694245656));
#45454=CARTESIAN_POINT('Ctrl Pts',(3.47528260305076,3.17808738228345,3.73047883250997));
#45455=CARTESIAN_POINT('Ctrl Pts',(1.53194465708238,4.45319819322398,3.80985072256337));
#45456=CARTESIAN_POINT('Ctrl Pts',(-0.784571616449287,4.64351978128216,
3.88922261261678));
#45457=CARTESIAN_POINT('Ctrl Pts',(-2.90996798083373,3.70269022887672,3.96859450267018));
#45458=CARTESIAN_POINT('Ctrl Pts',(-4.32650258619195,1.85989353248269,4.04796639272359));
#45459=CARTESIAN_POINT('Ctrl Pts',(-4.68911073810485,-0.4359691116196,4.12733828277699));
#45460=CARTESIAN_POINT('Ctrl Pts',(-3.90946189338598,-2.62563064513263,
4.2067101728304));
#45461=CARTESIAN_POINT('Ctrl Pts',(-2.17747678488539,-4.17569436522619,
4.28608206288379));
#45462=CARTESIAN_POINT('Ctrl Pts',(0.0849368486501527,-4.70856818069336,
4.3654539529372));
#45463=CARTESIAN_POINT('Ctrl Pts',(2.32666005385904,-4.09444520958252,4.4448258429906));
#45464=CARTESIAN_POINT('Ctrl Pts',(4.00161401992256,-2.48292444831813,4.52419773304401));
#45465=CARTESIAN_POINT('Ctrl Pts',(4.70178366815532,-0.266568787303479,
4.60356962309741));
#45466=CARTESIAN_POINT('Ctrl Pts',(4.25660922204708,2.0147224402583,4.68294151315081));
#45467=CARTESIAN_POINT('Ctrl Pts',(2.77453419129287,3.80523174088563,4.76231340320422));
#45468=CARTESIAN_POINT('Ctrl Pts',(0.616588772866969,4.6687950121708,4.84168529325762));
#45469=CARTESIAN_POINT('Ctrl Pts',(-1.69155630583321,4.39505015269366,4.92105718331103));
#45470=CARTESIAN_POINT('Ctrl Pts',(-3.5876420126288,3.05068080429882,5.00042907336443));
#45471=CARTESIAN_POINT('Ctrl Pts',(-4.60978606625892,0.96317236454425,5.07980096341783));
#45472=CARTESIAN_POINT('Ctrl Pts',(-4.50899643773674,-1.35896273126747,
5.15917285347124));
#45473=CARTESIAN_POINT('Ctrl Pts',(-3.30982525747623,-3.3500575137554,5.23854474352463));
#45474=CARTESIAN_POINT('Ctrl Pts',(-1.30438797066844,-4.52508570111905,
5.31791663357805));
#45475=CARTESIAN_POINT('Ctrl Pts',(1.01879533858038,-4.5978130277974,5.39728852363144));
#45476=CARTESIAN_POINT('Ctrl Pts',(3.09380235841625,-3.55052327799082,5.47666041368486));
#45477=CARTESIAN_POINT('Ctrl Pts',(4.41516597175728,-1.63833391661564,5.55603230373825));
#45478=CARTESIAN_POINT('Ctrl Pts',(4.66100492718236,0.672949960456484,5.63540419379167));
#45479=CARTESIAN_POINT('Ctrl Pts',(3.77143339930522,2.82030471671088,5.71477608384506));
#45480=CARTESIAN_POINT('Ctrl Pts',(1.96314904328358,4.28063948661312,5.79414797389847));
#45481=CARTESIAN_POINT('Ctrl Pts',(-0.323354074325263,4.69821995261119,
5.87351986395187));
#45482=CARTESIAN_POINT('Ctrl Pts',(-2.53108885516056,3.97132443748664,5.95289175400528));
#45483=CARTESIAN_POINT('Ctrl Pts',(-4.1222559933489,2.2770230797679,6.03226364405868));
#45484=CARTESIAN_POINT('Ctrl Pts',(-4.70925069601632,0.0280439399227974,
6.11163553411208));
#45485=CARTESIAN_POINT('Ctrl Pts',(-4.14908235288379,-2.22776664161329,
6.19100742416549));
#45486=CARTESIAN_POINT('Ctrl Pts',(-2.57820673242676,-3.94089820033021,
6.27037931421889));
#45487=CARTESIAN_POINT('Ctrl Pts',(-0.37928565871439,-4.6940356804769,6.34975120427229));
#45488=CARTESIAN_POINT('Ctrl Pts',(1.91202856192625,-4.30371645893114,6.42912309432569));
#45489=CARTESIAN_POINT('Ctrl Pts',(3.73757685708508,-2.86502143410457,6.5084949843791));
#45490=CARTESIAN_POINT('Ctrl Pts',(4.65265970284404,-0.728413529547492,
6.58786687443251));
#45491=CARTESIAN_POINT('Ctrl Pts',(4.43436494347775,1.58563429849135,6.6672387644859));
#45492=CARTESIAN_POINT('Ctrl Pts',(3.13586869918061,3.51342512115968,6.74661065453932));
#45493=CARTESIAN_POINT('Ctrl Pts',(1.07348178089069,4.58535336114812,6.8259825445927));
#45494=CARTESIAN_POINT('Ctrl Pts',(-1.25040292311256,4.54029967186839,6.90535443464612));
#45495=CARTESIAN_POINT('Ctrl Pts',(-3.26969224276554,3.38923903230437,6.98472632469952));
#45496=CARTESIAN_POINT('Ctrl Pts',(-4.49249176942184,1.41256726642436,7.06409821475293));
#45497=CARTESIAN_POINT('Ctrl Pts',(-4.62093024500886,-0.908202758892002,
7.14347010480633));
#45498=CARTESIAN_POINT('Ctrl Pts',(-3.62372034116731,-3.00773660241498,
7.22284199485974));
#45499=CARTESIAN_POINT('Ctrl Pts',(-1.74378018318635,-4.37459246710173,
7.30221388491313));
#45500=CARTESIAN_POINT('Ctrl Pts',(0.560940967626854,-4.67580728979868,
7.38158577496654));
#45501=CARTESIAN_POINT('Ctrl Pts',(2.72901814034792,-3.83800580642455,7.46095766501994));
#45502=CARTESIAN_POINT('Ctrl Pts',(4.23231253465944,-2.06527460388716,7.54032955507336));
#45503=CARTESIAN_POINT('Ctrl Pts',(4.70462496359279,0.210552920749357,7.61970144512673));
#45504=CARTESIAN_POINT('Ctrl Pts',(4.03090116490568,2.4350902199423,7.69907333518017));
#45505=CARTESIAN_POINT('Ctrl Pts',(2.37525876469593,4.06644493153808,7.77844522523354));
#45506=CARTESIAN_POINT('Ctrl Pts',(0.141008586952364,4.70722265873438,7.85781711528697));
#45507=CARTESIAN_POINT('Ctrl Pts',(-2.1275909704556,4.2013313655236,7.93718900534037));
#45508=CARTESIAN_POINT('Ctrl Pts',(-3.87791407680332,2.67200505116051,8.01656089539376));
#45509=CARTESIAN_POINT('Ctrl Pts',(-4.68358589765895,0.491784220717585,
8.09593278544718));
#45510=CARTESIAN_POINT('Ctrl Pts',(-4.3483465607864,-1.80823415734624,8.17530467550056));
#45511=CARTESIAN_POINT('Ctrl Pts',(-2.95385962660815,-3.66777069713892,
8.25467656555399));
#45512=CARTESIAN_POINT('Ctrl Pts',(-0.839819025645543,-4.63384641358131,
8.33404845560737));
#45513=CARTESIAN_POINT('Ctrl Pts',(1.47879963105641,-4.47112740052035,8.41342034566079));
#45514=CARTESIAN_POINT('Ctrl Pts',(3.43718597090052,-3.21925164936531,8.49279223571418));
#45515=CARTESIAN_POINT('Ctrl Pts',(4.55828141631537,-1.1831733221175,8.57216412576761));
#45516=CARTESIAN_POINT('Ctrl Pts',(4.56898959830056,1.1411234074884,8.65153601582098));
#45517=CARTESIAN_POINT('Ctrl Pts',(3.46670202742665,3.18744500086393,8.73090790587441));
#45518=CARTESIAN_POINT('Ctrl Pts',(1.51993351608642,4.45731204731885,8.8102797959278));
#45519=CARTESIAN_POINT('Ctrl Pts',(-0.797087435456723,4.64138774513978,
8.88965168598121));
#45520=CARTESIAN_POINT('Ctrl Pts',(-2.91993965204571,3.69483166178214,8.96902357603462));
#45521=CARTESIAN_POINT('Ctrl Pts',(-4.33150103257314,1.84822276398555,9.04839546608801));
#45522=CARTESIAN_POINT('Ctrl Pts',(-4.68791834918067,-0.448609108146216,
9.12776735614143));
#45523=CARTESIAN_POINT('Ctrl Pts',(-3.90236913245906,-2.63616079451299,
9.20713924619481));
#45524=CARTESIAN_POINT('Ctrl Pts',(-2.16621143281798,-4.18154954637933,
9.28651113624823));
#45525=CARTESIAN_POINT('Ctrl Pts',(0.0976305770298679,-4.70832208445062,
9.36588302630162));
#45526=CARTESIAN_POINT('Ctrl Pts',(2.33768999441487,-4.08815778444389,9.44525491635505));
#45527=CARTESIAN_POINT('Ctrl Pts',(4.00829330354943,-2.47212729713041,9.52462680640842));
#45528=CARTESIAN_POINT('Ctrl Pts',(4.70248523614611,-0.253892072196923,
9.60399869646185));
#45529=CARTESIAN_POINT('Ctrl Pts',(4.25116217399211,2.02619069954319,9.68337058651524));
#45530=CARTESIAN_POINT('Ctrl Pts',(2.76426541604147,3.81269790177162,9.76274247656865));
#45531=CARTESIAN_POINT('Ctrl Pts',(0.603999721340871,4.67044033439211,9.84211436662206));
#45532=CARTESIAN_POINT('Ctrl Pts',(-1.70339896854767,4.39047383939904,9.92148625667545));
#45533=CARTESIAN_POINT('Ctrl Pts',(-3.59585344010767,3.04099763527736,10.0008581467289));
#45534=CARTESIAN_POINT('Ctrl Pts',(-4.61236597294403,0.95074113833618,10.0802300367823));
#45535=CARTESIAN_POINT('Ctrl Pts',(-4.5053163640701,-1.37111379547384,10.1596019268357));
#45536=CARTESIAN_POINT('Ctrl Pts',(-3.30078166125737,-3.35896844361534,
10.2389738168891));
#45537=CARTESIAN_POINT('Ctrl Pts',(-1.29218385191862,-4.5285858138427,10.3183457069425));
#45538=CARTESIAN_POINT('Ctrl Pts',(1.03118708354706,-4.59504970367267,10.3977175969959));
#45539=CARTESIAN_POINT('Ctrl Pts',(3.1033631279546,-3.54216965665798,10.4770894870493));
#45540=CARTESIAN_POINT('Ctrl Pts',(4.41956678357015,-1.62642492174092,10.5564613771027));
#45541=CARTESIAN_POINT('Ctrl Pts',(4.65917375325315,0.68551332408169,10.6358332671561));
#45542=CARTESIAN_POINT('Ctrl Pts',(3.76381630954987,2.83046204151602,10.7152051572095));
#45543=CARTESIAN_POINT('Ctrl Pts',(1.95160154390631,4.28591647075852,10.7945770472629));
#45544=CARTESIAN_POINT('Ctrl Pts',(-0.336019038036085,4.69733113443942,
10.8739489373163));
#45545=CARTESIAN_POINT('Ctrl Pts',(-2.54178612607839,3.96448633113698,10.9533208273697));
#45546=CARTESIAN_POINT('Ctrl Pts',(-4.12837973995617,2.26590143281123,11.0326927174231));
#45547=CARTESIAN_POINT('Ctrl Pts',(-4.70930918719419,0.0153479609404256,
11.1120646074765));
#45548=CARTESIAN_POINT('Ctrl Pts',(-4.14306134031078,-2.23894424024334,
11.1914364975299));
#45549=CARTESIAN_POINT('Ctrl Pts',(-2.5675729214384,-3.94783458032284,11.2708083875833));
#45550=CARTESIAN_POINT('Ctrl Pts',(-0.366629422129896,-4.69504115501934,
11.3501802776367));
#45551=CARTESIAN_POINT('Ctrl Pts',(1.92362419288899,-4.29854609665044,11.4295521676901));
#45552=CARTESIAN_POINT('Ctrl Pts',(3.74528721239005,-2.85493472380791,11.5089240577435));
#45553=CARTESIAN_POINT('Ctrl Pts',(4.65460655700554,-0.715867571536574,
11.5882959477969));
#45554=CARTESIAN_POINT('Ctrl Pts',(4.43007404713131,1.59758333661508,11.6676678378504));
#45555=CARTESIAN_POINT('Ctrl Pts',(3.12638530517848,3.52186648015801,11.7470397279037));
#45556=CARTESIAN_POINT('Ctrl Pts',(1.06111602302068,4.5882307446537,11.8264116179572));
#45557=CARTESIAN_POINT('Ctrl Pts',(-1.26263877360451,4.53691215562823,11.9057835080105));
#45558=CARTESIAN_POINT('Ctrl Pts',(-3.27881755978316,3.38041180777642,11.985155398064));
#45559=CARTESIAN_POINT('Ctrl Pts',(-4.49628364593817,1.40045062596491,12.0645272881173));
#45560=CARTESIAN_POINT('Ctrl Pts',(-4.6184649882977,-0.920657228486762,
12.1438991781708));
#45561=CARTESIAN_POINT('Ctrl Pts',(-3.61559848230676,-3.01749501991928,
12.2232710682242));
#45562=CARTESIAN_POINT('Ctrl Pts',(-1.7319801890174,-4.37927770361138,12.3026429582776));
#45563=CARTESIAN_POINT('Ctrl Pts',(0.573544644643477,-4.67427803207056,
12.382014848331));
#45564=CARTESIAN_POINT('Ctrl Pts',(2.73935527238874,-3.83063457825627,12.4613867383844));
#45565=CARTESIAN_POINT('Ctrl Pts',(4.23786501924016,-2.05385702014458,12.5407586284378));
#45566=CARTESIAN_POINT('Ctrl Pts',(4.7040402277598,0.22323556193892,12.6201305184912));
#45567=CARTESIAN_POINT('Ctrl Pts',(4.02432164901358,2.44594845525766,12.6995024085446));
#45568=CARTESIAN_POINT('Ctrl Pts',(2.3642872242525,4.0728337188907,12.778874298598));
#45569=CARTESIAN_POINT('Ctrl Pts',(0.12831766492455,4.70758570366646,12.8582461886514));
#45570=CARTESIAN_POINT('Ctrl Pts',(-2.13890979355269,4.19558023109331,12.9376180787048));
#45571=CARTESIAN_POINT('Ctrl Pts',(-3.88510356071705,2.66154070098513,13.0169899687582));
#45572=CARTESIAN_POINT('Ctrl Pts',(-4.68489470002156,0.479155747337376,
13.0963618588116));
#45573=CARTESIAN_POINT('Ctrl Pts',(-4.34345586023936,-1.81995048576848,
13.175733748865));
#45574=CARTESIAN_POINT('Ctrl Pts',(-2.94396078697933,-3.67572080893321,
13.2551056389184));
#45575=CARTESIAN_POINT('Ctrl Pts',(-0.827323382357809,-4.63609367911183,
13.3344775289718));
#45576=CARTESIAN_POINT('Ctrl Pts',(1.49084816695683,-4.4671243908781,13.4138494190252));
#45577=CARTESIAN_POINT('Ctrl Pts',(3.44585240273723,-3.2099734888386,13.4932213090786));
#45578=CARTESIAN_POINT('Ctrl Pts',(4.56145462047577,-1.17088015007382,13.572593199132));
#45579=CARTESIAN_POINT('Ctrl Pts',(4.56589658927495,1.15343700154968,13.6519650891854));
#45580=CARTESIAN_POINT('Ctrl Pts',(3.45809625536746,3.19677945268519,13.7313369792388));
#45581=CARTESIAN_POINT('Ctrl Pts',(1.50791132801865,4.4613935050979,13.8107088692922));
#45582=CARTESIAN_POINT('Ctrl Pts',(-0.809597461130395,4.63922197479575,
13.8900807593457));
#45583=CARTESIAN_POINT('Ctrl Pts',(-2.92989010076163,3.68694624017703,13.969452649399));
#45584=CARTESIAN_POINT('Ctrl Pts',(-4.33646799704908,1.83653856236827,14.0488245394525));
#45585=CARTESIAN_POINT('Ctrl Pts',(-4.68669188786449,-0.461245844124263,
14.1281964295058));
#45586=CARTESIAN_POINT('Ctrl Pts',(-3.8952480086126,-2.64667178393849,14.2075683195593));
#45587=CARTESIAN_POINT('Ctrl Pts',(-2.15493033644793,-4.1873743354939,14.2869402096127));
#45588=CARTESIAN_POINT('Ctrl Pts',(0.110323595818042,-4.70804176751889,
14.3663120996661));
#45589=CARTESIAN_POINT('Ctrl Pts',(2.34870294433987,-4.08184064604999,14.4456839897195));
#45590=CARTESIAN_POINT('Ctrl Pts',(4.01494345438633,-2.46131217820434,14.5250558797729));
#45591=CARTESIAN_POINT('Ctrl Pts',(4.70315262587088,-0.241213511770193,
14.6044277698263));
#45592=CARTESIAN_POINT('Ctrl Pts',(4.24568422794502,2.03764423221413,14.6837996598797));
#45593=CARTESIAN_POINT('Ctrl Pts',(2.7539765497544,3.82013635148006,14.7631715499331));
#45594=CARTESIAN_POINT('Ctrl Pts',(0.591406279867313,4.67205171125386,14.8425434399865));
#45595=CARTESIAN_POINT('Ctrl Pts',(-1.71522925073988,4.38586561557727,14.9219153300399));
#45596=CARTESIAN_POINT('Ctrl Pts',(-3.60403873246238,3.0312923638949,15.0012872200933));
#45597=CARTESIAN_POINT('Ctrl Pts',(-4.61491235636145,0.938303002019602,
15.0806591101467));
#45598=CARTESIAN_POINT('Ctrl Pts',(-4.50160354518612,-1.38325489424921,
15.1600310002001));
#45599=CARTESIAN_POINT('Ctrl Pts',(-3.29171407453388,-3.36785496006171,
15.2394028902535));
#45600=CARTESIAN_POINT('Ctrl Pts',(-1.27997034141067,-4.53205301222367,
15.3187747803069));
#45601=CARTESIAN_POINT('Ctrl Pts',(1.04357133371383,-4.59225298213712,15.3981466703603));
#45602=CARTESIAN_POINT('Ctrl Pts',(3.11290134185163,-3.53379029038156,15.4775185604137));
#45603=CARTESIAN_POINT('Ctrl Pts',(4.42393547340459,-1.6145041058012,15.5568904504671));
#45604=CARTESIAN_POINT('Ctrl Pts',(4.65730871585136,0.69807170530811,15.6362623405205));
#45605=CARTESIAN_POINT('Ctrl Pts',(3.75617186389461,2.84059879415993,15.7156342305739));
#45606=CARTESIAN_POINT('Ctrl Pts',(1.94003986003872,4.2911623043131,15.7950061206273));
#45607=CARTESIAN_POINT('Ctrl Pts',(-0.348681559517582,4.69640817546235,
15.8743780106807));
#45608=CARTESIAN_POINT('Ctrl Pts',(-2.55246492296822,3.95761941039193,15.9537499007341));
#45609=CARTESIAN_POINT('Ctrl Pts',(-4.13447348097045,2.25476331699244,16.0331217907876));
#45610=CARTESIAN_POINT('Ctrl Pts',(-4.70933345050753,0.00265187040668795,
16.1124936808409));
#45611=CARTESIAN_POINT('Ctrl Pts',(-4.13701021543854,-2.25010556593871,
16.1918655708943));
#45612=CARTESIAN_POINT('Ctrl Pts',(-2.55692044899651,-3.95474226694862,
16.2712374609477));
#45613=CARTESIAN_POINT('Ctrl Pts',(-0.353970520843347,-4.69601250539775,
16.3506093510012));
#45614=CARTESIAN_POINT('Ctrl Pts',(1.93520584271894,-4.29334449198998,16.4299812410546));
#45615=CARTESIAN_POINT('Ctrl Pts',(3.75297034643966,-2.8448272634702,16.509353131108));
#45616=CARTESIAN_POINT('Ctrl Pts',(4.65651958094123,-0.703316410525392,
16.5887250211614));
#45617=CARTESIAN_POINT('Ctrl Pts',(4.42575095234045,1.60952076333056,16.6680969112148));
#45618=CARTESIAN_POINT('Ctrl Pts',(3.11687918839165,3.53028224171774,16.7474688012682));
#45619=CARTESIAN_POINT('Ctrl Pts',(1.04874255247428,4.59107478042509,16.8268406913216));
#45620=CARTESIAN_POINT('Ctrl Pts',(-1.27486544641699,4.53349166431028,16.906212581375));
#45621=CARTESIAN_POINT('Ctrl Pts',(-3.28791904717816,3.37156001439364,16.9855844714284));
#45622=CARTESIAN_POINT('Ctrl Pts',(-4.50004284053898,1.38832380607291,17.0649563614818));
#45623=CARTESIAN_POINT('Ctrl Pts',(-4.61596616842608,-0.933105005158158,
17.1443282515352));
#45624=CARTESIAN_POINT('Ctrl Pts',(-3.60745033643721,-3.02723150865552,
17.2237001415886));
#45625=CARTESIAN_POINT('Ctrl Pts',(-1.72016762240852,-4.3839311057331,17.303072031642));
#45626=CARTESIAN_POINT('Ctrl Pts',(0.586144182924747,-4.67271481097615,
17.3824439216954));
#45627=CARTESIAN_POINT('Ctrl Pts',(2.74967243806105,-3.82323548987727,17.4618158117488));
#45628=CARTESIAN_POINT('Ctrl Pts',(4.24338680893684,-2.04242454395285,17.5411877018022));
#45629=CARTESIAN_POINT('Ctrl Pts',(4.70342110133588,0.235916647177909,17.6205595918556));
#45630=CARTESIAN_POINT('Ctrl Pts',(4.01771326340766,2.45678878743836,17.699931481909));
#45631=CARTESIAN_POINT('Ctrl Pts',(2.35329778315649,4.07919314165109,17.7793033719624));
#45632=CARTESIAN_POINT('Ctrl Pts',(0.115627163561191,4.70791408521782,17.8586752620158));
#45633=CARTESIAN_POINT('Ctrl Pts',(-2.15021562607272,4.18979944864554,17.9380471520692));
#45634=CARTESIAN_POINT('Ctrl Pts',(-3.89225998228542,2.6510554089743,18.0174190421226));
#45635=CARTESIAN_POINT('Ctrl Pts',(-4.68617856238767,0.466526807638264,
18.096790932176));
#45636=CARTESIAN_POINT('Ctrl Pts',(-4.33851638857381,-1.83165928184378,
18.1761628222294));
#45637=CARTESIAN_POINT('Ctrl Pts',(-2.93407303174987,-3.68363345125881,
18.2555347122828));
#45638=CARTESIAN_POINT('Ctrl Pts',(-0.814760394348088,-4.63832755437977,
18.3349066023362));
#45639=CARTESIAN_POINT('Ctrl Pts',(1.50277006074129,-4.46305057284721,18.4142784923896));
#45640=CARTESIAN_POINT('Ctrl Pts',(3.45471245456617,-3.20074439226408,18.493650382443));
#45641=CARTESIAN_POINT('Ctrl Pts',(4.56418179760217,-1.15844177813615,18.5730222724965));
#45642=CARTESIAN_POINT('Ctrl Pts',(4.56354990278295,1.16548416044567,18.6523941625499));
#45643=CARTESIAN_POINT('Ctrl Pts',(3.44799414715945,3.20657754587687,18.7317660526033));
#45644=CARTESIAN_POINT('Ctrl Pts',(1.49865065220682,4.46452630956668,18.8111379426567));
#45645=CARTESIAN_POINT('Ctrl Pts',(-0.827291992766502,4.63872722375952,
18.8905098327101));
#45646=CARTESIAN_POINT('Ctrl Pts',(-2.93038174053102,3.67602118591242,18.9698817227635));
#45647=CARTESIAN_POINT('Ctrl Pts',(-4.8317659974063,1.21320979378885,19.0757109095013));
#45648=CARTESIAN_POINT('Ctrl Pts',(-4.41154214902252,-3.00742829557681,
19.2079973929237));
#45649=CARTESIAN_POINT('Ctrl Pts',(0.14114360583215,-5.34031031892966,19.3667411730305));
#45650=CARTESIAN_POINT('Ctrl Pts',(4.55878074835922,-2.77696271962162,19.5254849531373));
#45651=CARTESIAN_POINT('Ctrl Pts',(4.80798654830346,2.32253130646654,19.6842287332441));
#45652=CARTESIAN_POINT('Ctrl Pts',(0.656009676029318,5.29932988758691,19.8429725133509));
#45653=CARTESIAN_POINT('Ctrl Pts',(-4.09539160933947,3.42571876325565,20.0017162934577));
#45654=CARTESIAN_POINT('Ctrl Pts',(-5.09974667860472,-1.58211192901314,
20.1604600735645));
#45655=CARTESIAN_POINT('Ctrl Pts',(-1.43734916996091,-5.14215993940121,
20.3192038536714));
#45656=CARTESIAN_POINT('Ctrl Pts',(3.54020456892056,-3.99752392897281,20.4779476337781));
#45657=CARTESIAN_POINT('Ctrl Pts',(5.27828887711237,0.806568563691912,20.636691413885));
#45658=CARTESIAN_POINT('Ctrl Pts',(2.1865632094635,4.86959394496087,20.7954351939918));
#45659=CARTESIAN_POINT('Ctrl Pts',(-2.90621803008048,4.48249178265495,20.9541789740986));
#45660=CARTESIAN_POINT('Ctrl Pts',(-5.339103029404,-0.0175478502156508,
21.1129227542054));
#45661=CARTESIAN_POINT('Ctrl Pts',(-3.29668819545046,-3.73492805813105,
21.2452092376277));
#45662=CARTESIAN_POINT('Ctrl Pts',(-0.335233909123966,-4.68912434583344,
21.3510384243656));
#45663=CARTESIAN_POINT('Ctrl Pts',(1.9434592869775,-4.29245481019942,21.430410314419));
#45664=CARTESIAN_POINT('Ctrl Pts',(3.76239327895729,-2.83237457985877,21.5097822044724));
#45665=CARTESIAN_POINT('Ctrl Pts',(4.65746145505442,-0.691994213306775,
21.5891540945258));
#45666=CARTESIAN_POINT('Ctrl Pts',(4.42189226956134,1.62210042840564,21.6685259845792));
#45667=CARTESIAN_POINT('Ctrl Pts',(3.10708740551244,3.53832597274477,21.7478978746326));
#45668=CARTESIAN_POINT('Ctrl Pts',(1.03650075501011,4.59406889295405,21.827269764686));
#45669=CARTESIAN_POINT('Ctrl Pts',(-1.28715662605568,4.52994106929143,21.9066416547395));
#45670=CARTESIAN_POINT('Ctrl Pts',(-3.29695756540469,3.36273516855513,21.9860135447928));
#45671=CARTESIAN_POINT('Ctrl Pts',(-4.5037900244027,1.37615964733944,22.0653854348462));
#45672=CARTESIAN_POINT('Ctrl Pts',(-4.61342283197247,-0.945531571193242,
22.1447573248996));
#45673=CARTESIAN_POINT('Ctrl Pts',(-3.59928179145312,-3.03695363259649,
22.224129214953));
#45674=CARTESIAN_POINT('Ctrl Pts',(-1.70833944819064,-4.388548607559,22.3035011050065));
#45675=CARTESIAN_POINT('Ctrl Pts',(0.598737773532913,-4.67111975194625,
22.3828729950598));
#45676=CARTESIAN_POINT('Ctrl Pts',(2.75997059360609,-3.81580751573965,22.4622448851133));
#45677=CARTESIAN_POINT('Ctrl Pts',(4.24887708766878,-2.03097775393672,22.5416167751666));
#45678=CARTESIAN_POINT('Ctrl Pts',(4.7027684336848,0.248596203073706,22.6209886652201));
#45679=CARTESIAN_POINT('Ctrl Pts',(4.01107478934813,2.46761134605171,22.7003605552734));
#45680=CARTESIAN_POINT('Ctrl Pts',(2.34229273922348,4.08552253105782,22.7797324453269));
#45681=CARTESIAN_POINT('Ctrl Pts',(0.10293307930986,4.70820909782832,22.8591043353802));
#45682=CARTESIAN_POINT('Ctrl Pts',(-2.16150070095897,4.18398654725925,22.9384762254337));
#45683=CARTESIAN_POINT('Ctrl Pts',(-3.89939777427635,2.64055403030605,23.017848115487));
#45684=CARTESIAN_POINT('Ctrl Pts',(-4.6874101388992,0.453888451717589,23.0972200055405));
#45685=CARTESIAN_POINT('Ctrl Pts',(-4.33357979136315,-1.84334337837373,
23.1765918955938));
#45686=CARTESIAN_POINT('Ctrl Pts',(-2.92409898707257,-3.69154082613157,
23.2559637856473));
#45687=CARTESIAN_POINT('Ctrl Pts',(-0.802314148160901,-4.64048710795707,
23.3353356757007));
#45688=CARTESIAN_POINT('Ctrl Pts',(1.51491264465863,-4.45902099747155,23.4147075657541));
#45689=CARTESIAN_POINT('Ctrl Pts',(3.46311006868958,-3.19134724418486,23.4940794558075));
#45690=CARTESIAN_POINT('Ctrl Pts',(4.56770154637975,-1.14626836492011,23.5734513458609));
#45691=CARTESIAN_POINT('Ctrl Pts',(4.55961103731633,1.17803895017003,23.6528232359143));
#45692=CARTESIAN_POINT('Ctrl Pts',(3.44080937235073,3.21537858488653,23.7321951259677));
#45693=CARTESIAN_POINT('Ctrl Pts',(1.48383416024502,4.46945911326291,23.8115670160211));
#45694=CARTESIAN_POINT('Ctrl Pts',(-0.834599768812189,4.6347892947245,23.8909389060745));
#45695=CARTESIAN_POINT('Ctrl Pts',(-2.94972704158065,3.67109506287238,23.9703107961279));
#45696=CARTESIAN_POINT('Ctrl Pts',(-4.34630733610966,1.81313019956259,24.0496826861813));
#45697=CARTESIAN_POINT('Ctrl Pts',(-4.68413678396127,-0.486509167079313,
24.1290545762347));
#45698=CARTESIAN_POINT('Ctrl Pts',(-3.8809208793951,-2.66763597748286,24.2084264662881));
#45699=CARTESIAN_POINT('Ctrl Pts',(-2.13232123888401,-4.19893256848769,
24.2877983563416));
#45700=CARTESIAN_POINT('Ctrl Pts',(0.13570713560786,-4.70737847998643,24.3671702463949));
#45701=CARTESIAN_POINT('Ctrl Pts',(2.37067755224746,-4.06911741336709,24.4465421364484));
#45702=CARTESIAN_POINT('Ctrl Pts',(4.02815616456577,-2.43962835168955,24.5259140265017));
#45703=CARTESIAN_POINT('Ctrl Pts',(4.70438485136804,-0.215851223566548,
24.6052859165551));
#45704=CARTESIAN_POINT('Ctrl Pts',(4.23463580135646,2.06050678483885,24.6846578066085));
#45705=CARTESIAN_POINT('Ctrl Pts',(2.73333884334173,3.83492990131186,24.7640296966619));
#45706=CARTESIAN_POINT('Ctrl Pts',(0.566206593231879,4.6751725822987,24.8434015867153));
#45707=CARTESIAN_POINT('Ctrl Pts',(-1.73885232971224,4.3765535705565,24.9227734767688));
#45708=CARTESIAN_POINT('Ctrl Pts',(-3.62033067402275,3.0118157963638,25.0021453668221));
#45709=CARTESIAN_POINT('Ctrl Pts',(-4.61990447960738,0.913406360718075,
25.0815172568756));
#45710=CARTESIAN_POINT('Ctrl Pts',(-4.49407977994478,-1.40750684260792,
25.1608891469289));
#45711=CARTESIAN_POINT('Ctrl Pts',(-3.27350719336448,-3.38555449453819,
25.2402610369824));
#45712=CARTESIAN_POINT('Ctrl Pts',(-1.25551550026584,-4.53888856539668,
25.3196329270357));
#45713=CARTESIAN_POINT('Ctrl Pts',(1.06831698966113,-4.58655942838399,25.3990048170892));
#45714=CARTESIAN_POINT('Ctrl Pts',(3.1319098255862,-3.51695456679402,25.4783767071426));
#45715=CARTESIAN_POINT('Ctrl Pts',(4.43257636036326,-1.59062735737991,25.557748597196));
#45716=CARTESIAN_POINT('Ctrl Pts',(4.65347710509718,0.723173155497971,25.6371204872493));
#45717=CARTESIAN_POINT('Ctrl Pts',(3.74080112732632,2.86081028841317,25.7164923773028));
#45718=CARTESIAN_POINT('Ctrl Pts',(1.91687427506164,4.30156036736711,25.7958642673562));
#45719=CARTESIAN_POINT('Ctrl Pts',(-0.373998907678805,4.69445986217281,
25.8752361574096));
#45720=CARTESIAN_POINT('Ctrl Pts',(-2.57376678434128,3.9437993255639,25.954608047463));
#45721=CARTESIAN_POINT('Ctrl Pts',(-4.14657076927436,2.23243800269932,26.0339799375164));
#45722=CARTESIAN_POINT('Ctrl Pts',(-4.70927929309089,-0.0227402762051125,
26.1133518275698));
#45723=CARTESIAN_POINT('Ctrl Pts',(-4.1248178049234,-2.27237907416072,26.1927237176232));
#45724=CARTESIAN_POINT('Ctrl Pts',(-2.53555982960589,-3.96847135947655,
26.2720956076766));
#45725=CARTESIAN_POINT('Ctrl Pts',(-0.328645092162861,-4.69785280568621,
26.35146749773));
#45726=CARTESIAN_POINT('Ctrl Pts',(1.95832686228742,-4.28284770695154,26.4308393877834));
#45727=CARTESIAN_POINT('Ctrl Pts',(3.76825472776749,-2.8245503867261,26.5102112778369));
#45728=CARTESIAN_POINT('Ctrl Pts',(4.66024408245379,-0.67819884433039,26.5895831678902));
#45729=CARTESIAN_POINT('Ctrl Pts',(4.41700829392964,1.63336043537654,26.6689550579436));
#45730=CARTESIAN_POINT('Ctrl Pts',(3.09779906188623,3.54703672840772,26.748326947997));
#45731=CARTESIAN_POINT('Ctrl Pts',(1.0239728352293,4.59666272563139,26.8276988380504));
#45732=CARTESIAN_POINT('Ctrl Pts',(-1.29929090756406,4.52655185743165,26.9070707281039));
#45733=CARTESIAN_POINT('Ctrl Pts',(-3.30605026120649,3.35378297611415,26.9864426181572));
#45734=CARTESIAN_POINT('Ctrl Pts',(-4.50746308903716,1.36403998528792,27.0658145082107));
#45735=CARTESIAN_POINT('Ctrl Pts',(-4.61086788547865,-0.957980126703151,
27.1451863982641));
#45736=CARTESIAN_POINT('Ctrl Pts',(-3.59107547100053,-3.04663840028233,
27.2245582883174));
#45737=CARTESIAN_POINT('Ctrl Pts',(-1.69650502049742,-4.39314230317249,
27.3039301783709));
#45738=CARTESIAN_POINT('Ctrl Pts',(0.611330297848721,-4.66948646506538,
27.3833020684242));
#45739=CARTESIAN_POINT('Ctrl Pts',(2.77024690879558,-3.80835405980132,27.4626739584777));
#45740=CARTESIAN_POINT('Ctrl Pts',(4.25433750459734,-2.01951503521836,27.542045848531));
#45741=CARTESIAN_POINT('Ctrl Pts',(4.70208090109553,0.261273381823074,27.6214177385845));
#45742=CARTESIAN_POINT('Ctrl Pts',(4.00440779796637,2.47841618137125,27.7007896286379));
#45743=CARTESIAN_POINT('Ctrl Pts',(2.33126981885889,4.09182228501852,27.7801615186913));
#45744=CARTESIAN_POINT('Ctrl Pts',(0.0902396720556605,4.70846953713028,
27.8595334087446));
#45745=CARTESIAN_POINT('Ctrl Pts',(-2.17277265911822,4.17814403201768,27.9389052987981));
#45746=CARTESIAN_POINT('Ctrl Pts',(-3.90650237988159,2.63003188887054,28.0182771888515));
#45747=CARTESIAN_POINT('Ctrl Pts',(-4.68861676780222,0.441249799071397,
28.0976490789049));
#45748=CARTESIAN_POINT('Ctrl Pts',(-4.32859448916339,-1.85501976509172,
28.1770209689583));
#45749=CARTESIAN_POINT('Ctrl Pts',(-2.91413617414575,-3.69941062049508,
28.2563928590117));
#45750=CARTESIAN_POINT('Ctrl Pts',(-0.78980073743719,-4.64263323725236,
28.3357647490651));
#45751=CARTESIAN_POINT('Ctrl Pts',(1.52692841071678,-4.4549206737093,28.4151366391185));
#45752=CARTESIAN_POINT('Ctrl Pts',(3.47170117781886,-3.18199929485031,28.494508529172));
#45753=CARTESIAN_POINT('Ctrl Pts',(4.57077522248444,-1.13394993100173,28.5738804192253));
#45754=CARTESIAN_POINT('Ctrl Pts',(4.55641854019218,1.19032712608322,28.6532523092787));
#45755=CARTESIAN_POINT('Ctrl Pts',(3.43212838697049,3.22464312999871,28.7326241993321));
#45756=CARTESIAN_POINT('Ctrl Pts',(1.47177935557015,4.47344320507303,28.8119960893855));
#45757=CARTESIAN_POINT('Ctrl Pts',(-0.84709186911874,4.63252241719017,28.891367979439));
#45758=CARTESIAN_POINT('Ctrl Pts',(-2.95961338949639,3.66312942239424,28.9707398694923));
#45759=CARTESIAN_POINT('Ctrl Pts',(-4.35117963918583,1.80140620850249,29.0501117595457));
#45760=CARTESIAN_POINT('Ctrl Pts',(-4.68280815994235,-0.499135570435458,
29.1294836495992));
#45761=CARTESIAN_POINT('Ctrl Pts',(-3.87371497815696,-2.67808902923317,
29.2088555396525));
#45762=CARTESIAN_POINT('Ctrl Pts',(-2.12099340201518,-4.2046659283592,29.288227429706));
#45763=CARTESIAN_POINT('Ctrl Pts',(0.148397472118242,-4.70699551420707,
29.3675993197594));
#45764=CARTESIAN_POINT('Ctrl Pts',(2.38163905051584,-4.06271141155196,29.4469712098127));
#45765=CARTESIAN_POINT('Ctrl Pts',(4.03471862787643,-2.428759801702,29.5263430998662));
#45766=CARTESIAN_POINT('Ctrl Pts',(4.70494967818454,-0.203167680126035,
29.6057149899196));
#45767=CARTESIAN_POINT('Ctrl Pts',(4.22906540111636,2.07191563862461,29.685086879973));
#45768=CARTESIAN_POINT('Ctrl Pts',(2.72299015321369,3.84228489391376,29.7644587700264));
#45769=CARTESIAN_POINT('Ctrl Pts',(0.553600531224683,4.67668205379885,29.8438306600798));
#45770=CARTESIAN_POINT('Ctrl Pts',(-1.75064495479666,4.37184981703873,29.9232025501332));
#45771=CARTESIAN_POINT('Ctrl Pts',(-3.62843720481647,3.00204464177339,30.0025744401866));
#45772=CARTESIAN_POINT('Ctrl Pts',(-4.62235018315249,0.900948036685143,
30.08194633024));
#45773=CARTESIAN_POINT('Ctrl Pts',(-4.49026888827113,-1.41961751592495,
30.1613182202934));
#45774=CARTESIAN_POINT('Ctrl Pts',(-3.26436803124854,-3.39436738392576,
30.2406901103467));
#45775=CARTESIAN_POINT('Ctrl Pts',(-1.24327434736992,-4.54225687050705,
30.3200620004003));
#45776=CARTESIAN_POINT('Ctrl Pts',(1.08067821558697,-4.58366263754788,30.3994338904535));
#45777=CARTESIAN_POINT('Ctrl Pts',(3.14137995726753,-3.50849833184719,30.4788057805071));
#45778=CARTESIAN_POINT('Ctrl Pts',(4.4368484946843,-1.57867159843783,30.5581776705604));
#45779=CARTESIAN_POINT('Ctrl Pts',(4.65151055959353,0.735716042020659,30.6375495606138));
#45780=CARTESIAN_POINT('Ctrl Pts',(3.73307494812974,2.87088488312276,30.7169214506672));
#45781=CARTESIAN_POINT('Ctrl Pts',(1.90527054232277,4.30671252129204,30.7962933407206));
#45782=CARTESIAN_POINT('Ctrl Pts',(-0.386653550349159,4.69343452202104,
30.875665230774));
#45783=CARTESIAN_POINT('Ctrl Pts',(-2.58438969399916,3.93684626192686,30.9550371208274));
#45784=CARTESIAN_POINT('Ctrl Pts',(-4.15257422864054,2.2212509664887,31.0344090108808));
#45785=CARTESIAN_POINT('Ctrl Pts',(-4.70920087275226,-0.0354361477304668,
31.1137809009342));
#45786=CARTESIAN_POINT('Ctrl Pts',(-4.11867660790086,-2.28349109479913,
31.1931527909877));
#45787=CARTESIAN_POINT('Ctrl Pts',(-2.52485183790083,-3.97529266559651,
31.272524681041));
#45788=CARTESIAN_POINT('Ctrl Pts',(-0.315978748852904,-4.69872174221564,
31.3518965710945));
#45789=CARTESIAN_POINT('Ctrl Pts',(1.9698660640085,-4.27755260287519,31.4312684611479));
#45790=CARTESIAN_POINT('Ctrl Pts',(3.77585586390199,-2.81438111767642,31.5106403512012));
#45791=CARTESIAN_POINT('Ctrl Pts',(4.66205553306415,-0.665632621738598,
31.5900122412547));
#45792=CARTESIAN_POINT('Ctrl Pts',(4.41258879365675,1.64526250750188,31.669384131308));
#45793=CARTESIAN_POINT('Ctrl Pts',(3.08822519121424,3.55537533164171,31.7487560213615));
#45794=CARTESIAN_POINT('Ctrl Pts',(1.01157676786242,4.59940659468345,31.8281279114149));
#45795=CARTESIAN_POINT('Ctrl Pts',(-1.31148951705349,4.52303259187412,31.9074998014683));
#45796=CARTESIAN_POINT('Ctrl Pts',(-3.31507985854797,3.34485786124704,31.9868716915217));
#45797=CARTESIAN_POINT('Ctrl Pts',(-4.51112408430495,1.35188315933753,32.066243581575));
#45798=CARTESIAN_POINT('Ctrl Pts',(-4.60826846832906,-0.970407287843986,
32.1456154716285));
#45799=CARTESIAN_POINT('Ctrl Pts',(-3.58284885369746,-3.05630866766684,
32.2249873616819));
#45800=CARTESIAN_POINT('Ctrl Pts',(-1.68465518880656,-4.39770002107054,
32.3043592517353));
#45801=CARTESIAN_POINT('Ctrl Pts',(0.623916751156621,-4.66782138348531,
32.3837311417887));
#45802=CARTESIAN_POINT('Ctrl Pts',(2.7805039515543,-3.80087178893047,32.4631030318421));
#45803=CARTESIAN_POINT('Ctrl Pts',(4.25976654389448,-2.00803823967918,32.5424749218955));
#45804=CARTESIAN_POINT('Ctrl Pts',(4.7013594349753,0.273948980040725,32.6218468119489));
#45805=CARTESIAN_POINT('Ctrl Pts',(3.99771157397872,2.4892028345985,32.7012187020023));
#45806=CARTESIAN_POINT('Ctrl Pts',(2.32023002234538,4.09809238840509,32.7805905920557));
#45807=CARTESIAN_POINT('Ctrl Pts',(0.0775455730107522,4.70869570736983,
32.8599624821091));
#45808=CARTESIAN_POINT('Ctrl Pts',(-2.18402880626508,4.17227117454043,32.9393343721625));
#45809=CARTESIAN_POINT('Ctrl Pts',(-3.91357860260051,2.61949061875855,33.018706262216));
#45810=CARTESIAN_POINT('Ctrl Pts',(-4.68978931390171,0.42860794639128,33.0980781522693));
#45811=CARTESIAN_POINT('Ctrl Pts',(-4.32357772900909,-1.86668267300931,
33.1774500423228));
#45812=CARTESIAN_POINT('Ctrl Pts',(-2.90415217940683,-3.70725352509686,
33.2568219323761));
#45813=CARTESIAN_POINT('Ctrl Pts',(-0.777281587132916,-4.64474562433732,
33.3361938224295));
#45814=CARTESIAN_POINT('Ctrl Pts',(1.53893307928302,-4.45078797045929,33.4155657124829));
#45815=CARTESIAN_POINT('Ctrl Pts',(3.4802670539562,-3.17262821862943,33.4949376025364));
#45816=CARTESIAN_POINT('Ctrl Pts',(4.57381567772608,-1.12162325523486,33.5743094925897));
#45817=CARTESIAN_POINT('Ctrl Pts',(4.55319292637118,1.20260665046394,33.6536813826432));
#45818=CARTESIAN_POINT('Ctrl Pts',(3.42342245647383,3.23388423803441,33.7330532726965));
#45819=CARTESIAN_POINT('Ctrl Pts',(1.45971385379651,4.47739478330101,33.81242516275));
#45820=CARTESIAN_POINT('Ctrl Pts',(-0.859577812643769,4.63022186990074,
33.8917970528033));
#45821=CARTESIAN_POINT('Ctrl Pts',(-2.96947822656726,3.65513715781495,33.9711689428568));
#45822=CARTESIAN_POINT('Ctrl Pts',(-4.35602031732756,1.78966912459429,34.0505408329101));
#45823=CARTESIAN_POINT('Ctrl Pts',(-4.6814455006743,-0.511758346012144,
34.1299127229636));
#45824=CARTESIAN_POINT('Ctrl Pts',(-3.86648092226059,-2.68852261628789,
34.209284613017));
#45825=CARTESIAN_POINT('Ctrl Pts',(-2.1096501494946,-4.21036872817975,34.2886565030704));
#45826=CARTESIAN_POINT('Ctrl Pts',(0.161086730056863,-4.70657833738016,
34.3680283931238));
#45827=CARTESIAN_POINT('Ctrl Pts',(2.39258323872595,-4.05627588142921,34.4474002831772));
#45828=CARTESIAN_POINT('Ctrl Pts',(4.04125176633455,-2.41787359917646,34.5267721732306));
#45829=CARTESIAN_POINT('Ctrl Pts',(4.7054803088231,-0.190482660036747,34.606144063284));
#45830=CARTESIAN_POINT('Ctrl Pts',(4.22346426348634,2.08330943346165,34.6855159533374));
#45831=CARTESIAN_POINT('Ctrl Pts',(2.71262167204393,3.84961196029602,34.7648878433908));
#45832=CARTESIAN_POINT('Ctrl Pts',(0.540990445577805,4.67815753457386,34.8442597334442));
#45833=CARTESIAN_POINT('Ctrl Pts',(-1.76242485596904,4.36711428835555,34.9236316234976));
#45834=CARTESIAN_POINT('Ctrl Pts',(-3.63651736366306,2.99225166793732,35.0030035135511));
#45835=CARTESIAN_POINT('Ctrl Pts',(-4.62476229086341,0.888483164446288,
35.0823754036044));
#45836=CARTESIAN_POINT('Ctrl Pts',(-4.48642536074711,-1.43171787127975,
35.1617472936579));
#45837=CARTESIAN_POINT('Ctrl Pts',(-3.25520514328689,-3.40315560261577,
35.2411191837112));
#45838=CARTESIAN_POINT('Ctrl Pts',(-1.2310241581964,-4.54559216191174,35.3204910737646));
#45839=CARTESIAN_POINT('Ctrl Pts',(1.09303158700498,-4.58073253206361,35.399862963818));
#45840=CARTESIAN_POINT('Ctrl Pts',(3.15082725699632,-3.50001659668431,35.4792348538714));
#45841=CARTESIAN_POINT('Ctrl Pts',(4.44108838142123,-1.56670436550804,35.5586067439248));
#45842=CARTESIAN_POINT('Ctrl Pts',(4.64951020631433,0.748253581264717,35.6379786339782));
#45843=CARTESIAN_POINT('Ctrl Pts',(3.72532163646553,2.8809386118726,35.7173505240316));
#45844=CARTESIAN_POINT('Ctrl Pts',(1.89365296183327,4.31183337347777,35.7967224140851));
#45845=CARTESIAN_POINT('Ctrl Pts',(-0.399305382771815,4.69237506938502,
35.8760943041384));
#45846=CARTESIAN_POINT('Ctrl Pts',(-2.59499381998119,3.92986458478612,35.9554661941919));
#45847=CARTESIAN_POINT('Ctrl Pts',(-4.1585475065645,2.210047785941,36.0348380842453));
#45848=CARTESIAN_POINT('Ctrl Pts',(-4.70908822533747,-0.0481317617014899,
36.1142099742986));
#45849=CARTESIAN_POINT('Ctrl Pts',(-4.11250547580826,-2.29458651873135,
36.1935818643521));
#45850=CARTESIAN_POINT('Ctrl Pts',(-2.51412549524861,-3.98208507877941,
36.2729537544055));
#45851=CARTESIAN_POINT('Ctrl Pts',(-0.303310108968769,-4.6995565278326,
36.3523256444589));
#45852=CARTESIAN_POINT('Ctrl Pts',(1.98139094849032,-4.27222640899768,36.4316975345123));
#45853=CARTESIAN_POINT('Ctrl Pts',(3.7834295566316,-2.80419139334371,36.5110694245656));
#45854=CARTESIAN_POINT('Ctrl Pts',(4.66383309925673,-0.653061561243602,
36.5904413146191));
#45855=CARTESIAN_POINT('Ctrl Pts',(4.4081372221224,1.65715262164824,36.6698132046725));
#45856=CARTESIAN_POINT('Ctrl Pts',(3.07862887492527,3.56368809395169,36.7491850947259));
#45857=CARTESIAN_POINT('Ctrl Pts',(0.999173348225765,4.60211703465827,36.8285569847793));
#45858=CARTESIAN_POINT('Ctrl Pts',(-1.3236785944688,4.51948045233538,36.9079288748327));
#45859=CARTESIAN_POINT('Ctrl Pts',(-3.32408536146365,3.33590843552393,36.9873007648862));
#45860=CARTESIAN_POINT('Ctrl Pts',(-4.51475229214413,1.33971650772689,37.0666726549395));
#45861=CARTESIAN_POINT('Ctrl Pts',(-4.60563555769299,-0.982827395940232,
37.146044544993));
#45862=CARTESIAN_POINT('Ctrl Pts',(-3.57459619578919,-3.06595672140786,
37.2254164350463));
#45863=CARTESIAN_POINT('Ctrl Pts',(-1.67279311282567,-4.40222577592056,
37.3047883250997));
#45864=CARTESIAN_POINT('Ctrl Pts',(0.636498669757439,-4.6661223755806,37.3841602151531));
#45865=CARTESIAN_POINT('Ctrl Pts',(2.79074078525356,-3.79336189283575,37.4635321052066));
#45866=CARTESIAN_POINT('Ctrl Pts',(4.26516462266191,-1.9965468494605,37.5429039952599));
#45867=CARTESIAN_POINT('Ctrl Pts',(4.70060379877145,0.286622587162363,37.6222758853134));
#45868=CARTESIAN_POINT('Ctrl Pts',(3.99098629411051,2.49997139597979,37.7016477753667));
#45869=CARTESIAN_POINT('Ctrl Pts',(2.3091733621022,4.10433270633122,37.7810196654202));
#45870=CARTESIAN_POINT('Ctrl Pts',(0.0648509103550771,4.70888765420329,
37.8603915554735));
#45871=CARTESIAN_POINT('Ctrl Pts',(-2.19526907961097,4.16636799246395,37.9397634455269));
#45872=CARTESIAN_POINT('Ctrl Pts',(-3.92062638092667,2.60893030984724,38.0191353355804));
#45873=CARTESIAN_POINT('Ctrl Pts',(-4.69092777401319,0.415962978544177,
38.0985072256337));
#45874=CARTESIAN_POINT('Ctrl Pts',(-4.31852954453265,-1.87833201365752,
38.1778791156872));
#45875=CARTESIAN_POINT('Ctrl Pts',(-2.89414707692572,-3.71506948486711,
38.2572510057405));
#45876=CARTESIAN_POINT('Ctrl Pts',(-0.764756787430149,-4.64682425288566,
38.336622895794));
#45877=CARTESIAN_POINT('Ctrl Pts',(1.55092656265596,-4.44662291817819,38.4159947858474));
#45878=CARTESIAN_POINT('Ctrl Pts',(3.48880763512333,-3.16323408359078,38.4953666759007));
#45879=CARTESIAN_POINT('Ctrl Pts',(4.57682288978048,-1.10928842689192,38.5747385659542));
#45880=CARTESIAN_POINT('Ctrl Pts',(4.5499342195639,1.21487743324952,38.6541104560075));
#45881=CARTESIAN_POINT('Ctrl Pts',(3.41469164371823,3.24310184347568,38.733482346061));
#45882=CARTESIAN_POINT('Ctrl Pts',(1.44763774336306,4.48131381605587,38.8128542361143));
#45883=CARTESIAN_POINT('Ctrl Pts',(-0.872057510020701,4.62788767559439,
38.8922261261678));
#45884=CARTESIAN_POINT('Ctrl Pts',(-2.9793214784951,3.6471183158447,38.9715980162212));
#45885=CARTESIAN_POINT('Ctrl Pts',(-4.36082934025308,1.77791905463904,39.0509699062746));
#45886=CARTESIAN_POINT('Ctrl Pts',(-4.68004880681061,-0.524377442655287,
39.130341796328));
#45887=CARTESIAN_POINT('Ctrl Pts',(-3.85921878174905,-2.6989365861694,39.2097136863814));
#45888=CARTESIAN_POINT('Ctrl Pts',(-2.09829153079023,-4.21604107122303,
39.2890855764348));
#45889=CARTESIAN_POINT('Ctrl Pts',(0.173774754931348,-4.70612667927191,
39.3684574664882));
#45890=CARTESIAN_POINT('Ctrl Pts',(2.40351015490339,-4.04981138575493,39.4478293565416));
#45891=CARTESIAN_POINT('Ctrl Pts',(4.04775531046155,-2.40696884895629,39.527201246595));
#45892=CARTESIAN_POINT('Ctrl Pts',(4.70597715859854,-0.177798095133498,
39.6065731366484));
#45893=CARTESIAN_POINT('Ctrl Pts',(4.21783163769349,2.0946915601602,39.6859450267019));
#45894=CARTESIAN_POINT('Ctrl Pts',(2.70223496968604,3.85690448821556,39.7653169167552));
#45895=CARTESIAN_POINT('Ctrl Pts',(0.528373605920714,4.67961139929736,39.8446888068086));
#45896=CARTESIAN_POINT('Ctrl Pts',(-1.77418661813221,4.36232362711485,39.9240606968621));
#45897=CARTESIAN_POINT('Ctrl Pts',(-3.6445811625546,2.98248116081159,40.0034325869154));
#45898=CARTESIAN_POINT('Ctrl Pts',(-4.62712170766669,0.875927969712799,
40.0828044769689));
#45899=CARTESIAN_POINT('Ctrl Pts',(-4.48258575488106,-1.44364637546354,
40.1621763670223));
#45900=CARTESIAN_POINT('Ctrl Pts',(-3.24594541476057,-3.41224896374515,
40.2415482570757));
#45901=CARTESIAN_POINT('Ctrl Pts',(-1.89461073269764,-4.16947670058303,
40.2944628504446));
#45902=CARTESIAN_POINT('Ctrl Pts',(-1.16918346556913,-4.36383719750631,
40.3209201471291));
#45903=CARTESIAN_POINT('Ctrl Pts',(-3.57461543774205,3.05624720968391,-0.106973382376353));
#45904=CARTESIAN_POINT('Ctrl Pts',(-4.08267404777841,2.46201708819397,-0.0805160856918847));
#45905=CARTESIAN_POINT('Ctrl Pts',(-4.79625497710715,1.01593427979912,-0.027601492322949));
#45906=CARTESIAN_POINT('Ctrl Pts',(-4.69765387924802,-1.40219731261579,
0.051770397730455));
#45907=CARTESIAN_POINT('Ctrl Pts',(-3.45499130789169,-3.47806613859392,
0.131142287783858));
#45908=CARTESIAN_POINT('Ctrl Pts',(-1.37056128557091,-4.70703587006775,
0.210514177837262));
#45909=CARTESIAN_POINT('Ctrl Pts',(1.04766160592227,-4.78919858119765,0.289886067890666));
#45910=CARTESIAN_POINT('Ctrl Pts',(3.21071490770584,-3.70482006635648,0.36925795794407));
#45911=CARTESIAN_POINT('Ctrl Pts',(4.59162481050196,-1.71790426872487,0.448629847997472));
#45912=CARTESIAN_POINT('Ctrl Pts',(4.85403585089543,0.687462033087635,0.528001738050878));
#45913=CARTESIAN_POINT('Ctrl Pts',(3.93400879434301,2.92537849589629,0.607373628104279));
#45914=CARTESIAN_POINT('Ctrl Pts',(2.05566892616791,4.45067161106188,0.686745518157684));
#45915=CARTESIAN_POINT('Ctrl Pts',(-0.323428943211738,4.89179500940945,
0.766117408211087));
#45916=CARTESIAN_POINT('Ctrl Pts',(-2.62373939006112,4.1412858336604,0.845489298264492));
#45917=CARTESIAN_POINT('Ctrl Pts',(-4.28491317807112,2.38196972749854,0.924861188317894));
#45918=CARTESIAN_POINT('Ctrl Pts',(-4.90229136258891,0.042410468561284,
1.0042330783713));
#45919=CARTESIAN_POINT('Ctrl Pts',(-4.32548234816227,-2.30747956911558,
1.0836049684247));
#45920=CARTESIAN_POINT('Ctrl Pts',(-2.69499534131545,-4.09527285943935,
1.16297685847811));
#45921=CARTESIAN_POINT('Ctrl Pts',(-0.408013469920106,-4.88546665687605,
1.24234874853151));
#45922=CARTESIAN_POINT('Ctrl Pts',(1.97835959833349,-4.48557163766149,1.32172063858491));
#45923=CARTESIAN_POINT('Ctrl Pts',(3.8828086375498,-2.99300127117732,1.40109252863832));
#45924=CARTESIAN_POINT('Ctrl Pts',(4.84141409235741,-0.771342433159628,
1.48046441869172));
#45925=CARTESIAN_POINT('Ctrl Pts',(4.62066178777609,1.63821372124453,1.55983630874512));
#45926=CARTESIAN_POINT('Ctrl Pts',(3.27432650082566,3.64870463556752,1.63920819879853));
#45927=CARTESIAN_POINT('Ctrl Pts',(1.13037252509344,4.77037917890212,1.71858008885193));
#45928=CARTESIAN_POINT('Ctrl Pts',(-1.2889376953016,4.72999991227064,1.79795197890533));
#45929=CARTESIAN_POINT('Ctrl Pts',(-3.394265546355,3.53740313723842,1.87732386895874));
#45930=CARTESIAN_POINT('Ctrl Pts',(-4.67275782327988,1.48310278759205,1.95669575901214));
#45931=CARTESIAN_POINT('Ctrl Pts',(-4.81297663748911,-0.9324781181648,2.03606764906555));
#45932=CARTESIAN_POINT('Ctrl Pts',(-3.78076499611659,-3.12090941842389,
2.11543953911895));
#45933=CARTESIAN_POINT('Ctrl Pts',(-1.82756737028867,-4.54909409232738,
2.19481142917235));
#45934=CARTESIAN_POINT('Ctrl Pts',(0.57082162169894,-4.86912951461188,2.27418331922576));
#45935=CARTESIAN_POINT('Ctrl Pts',(2.8301597301281,-4.00305576476012,2.35355520927916));
#45936=CARTESIAN_POINT('Ctrl Pts',(4.40007719275289,-2.16184649123289,2.43292709933256));
#45937=CARTESIAN_POINT('Ctrl Pts',(4.89814559062742,0.205983802396055,2.51229898938597));
#45938=CARTESIAN_POINT('Ctrl Pts',(4.20303656448716,2.52363689769692,2.59167087943937));
#45939=CARTESIAN_POINT('Ctrl Pts',(2.48407713450111,4.22653763069529,2.67104276949277));
#45940=CARTESIAN_POINT('Ctrl Pts',(0.160002012962259,4.89986315213815,2.75041465954618));
#45941=CARTESIAN_POINT('Ctrl Pts',(-2.20304924477586,4.37959285538356,2.82978654959959));
#45942=CARTESIAN_POINT('Ctrl Pts',(-4.02944258285332,2.79246343312173,2.90915843965298));
#45943=CARTESIAN_POINT('Ctrl Pts',(-4.8742726267676,0.525096099564501,2.9885303297064));
#45944=CARTESIAN_POINT('Ctrl Pts',(-4.53174064782075,-1.87018348156618,
3.06790221975979));
#45945=CARTESIAN_POINT('Ctrl Pts',(-3.08528667790254,-3.80989050616825,
3.1472741098132));
#45946=CARTESIAN_POINT('Ctrl Pts',(-0.887263702413488,-4.82151663651732,
3.2266459998666));
#45947=CARTESIAN_POINT('Ctrl Pts',(1.52689474705858,-4.65863198645683,3.30601788992001));
#45948=CARTESIAN_POINT('Ctrl Pts',(3.56910501587138,-3.36091489620245,3.38538977997341));
#45949=CARTESIAN_POINT('Ctrl Pts',(4.74188920289787,-1.24448637649211,3.46476167002681));
#45950=CARTESIAN_POINT('Ctrl Pts',(4.75955967609216,1.17509626990786,3.54413356008022));
#45951=CARTESIAN_POINT('Ctrl Pts',(3.61781194729703,3.30842806598974,3.62350545013362));
#45952=CARTESIAN_POINT('Ctrl Pts',(1.59477323603129,4.63583410827783,3.70287734018703));
#45953=CARTESIAN_POINT('Ctrl Pts',(-0.816748705561003,4.83396122303419,
3.78224923024042));
#45954=CARTESIAN_POINT('Ctrl Pts',(-3.02931247032122,3.85454608365112,3.86162112029383));
#45955=CARTESIAN_POINT('Ctrl Pts',(-4.50394242258063,1.93617205018365,3.94099301034724));
#45956=CARTESIAN_POINT('Ctrl Pts',(-4.88142197000684,-0.453849209064403,
4.02036490040064));
#45957=CARTESIAN_POINT('Ctrl Pts',(-4.06979793038364,-2.73331380556256,
4.09973679045404));
#45958=CARTESIAN_POINT('Ctrl Pts',(-2.2667801232639,-4.34694920911316,4.17910868050745));
#45959=CARTESIAN_POINT('Ctrl Pts',(0.0884203044502142,-4.90167740713265,
4.25848057056085));
#45960=CARTESIAN_POINT('Ctrl Pts',(2.42208174171528,-4.26236783845356,4.33785246061425));
#45961=CARTESIAN_POINT('Ctrl Pts',(4.16572942788551,-2.58475489891836,4.41722435066765));
#45962=CARTESIAN_POINT('Ctrl Pts',(4.89461464610853,-0.277501387264568,
4.49659624072106));
#45963=CARTESIAN_POINT('Ctrl Pts',(4.43118257058524,2.09735084808797,4.57596813077446));
#45964=CARTESIAN_POINT('Ctrl Pts',(2.88832422912366,3.96129305925364,4.65534002082787));
#45965=CARTESIAN_POINT('Ctrl Pts',(0.641876498644775,4.86027304935857,4.73471191088126));
#45966=CARTESIAN_POINT('Ctrl Pts',(-1.76093092613442,4.57530128267169,4.81408380093468));
#45967=CARTESIAN_POINT('Ctrl Pts',(-3.73477947506178,3.17579625078358,4.89345569098808));
#45968=CARTESIAN_POINT('Ctrl Pts',(-4.79884401065823,1.00267428171038,4.97282758104148));
#45969=CARTESIAN_POINT('Ctrl Pts',(-4.6939207673194,-1.41469692300561,5.05219947109488));
#45970=CARTESIAN_POINT('Ctrl Pts',(-3.44556881487893,-3.48745108865595,
5.13157136114829));
#45971=CARTESIAN_POINT('Ctrl Pts',(-1.35788392577118,-4.71066988845176,
5.21094325120169));
#45972=CARTESIAN_POINT('Ctrl Pts',(1.06057848202937,-4.78637993031164,5.2903151412551));
#45973=CARTESIAN_POINT('Ctrl Pts',(3.22068631915819,-3.69613841561989,5.3696870313085));
#45974=CARTESIAN_POINT('Ctrl Pts',(4.59624209780833,-1.70552576414673,5.44905892136191));
#45975=CARTESIAN_POINT('Ctrl Pts',(4.85216347504167,0.700549188355308,5.52843081141531));
#45976=CARTESIAN_POINT('Ctrl Pts',(3.92610856983656,2.93597190921332,5.60780270146871));
#45977=CARTESIAN_POINT('Ctrl Pts',(2.04366230731317,4.45619837165057,5.68717459152211));
#45978=CARTESIAN_POINT('Ctrl Pts',(-0.336615569701915,4.89090477438153,
5.76654648157553));
#45979=CARTESIAN_POINT('Ctrl Pts',(-2.63489463902355,4.13419759990724,5.84591837162891));
#45980=CARTESIAN_POINT('Ctrl Pts',(-4.29131920651939,2.37040904098672,5.92529026168234));
#45981=CARTESIAN_POINT('Ctrl Pts',(-4.90238791398106,0.0291940864932555,
6.00466215173572));
#45982=CARTESIAN_POINT('Ctrl Pts',(-4.31924577684855,-2.31913248284995,
6.08403404178914));
#45983=CARTESIAN_POINT('Ctrl Pts',(-2.68394492896408,-4.1025235126836,6.16340593184253));
#45984=CARTESIAN_POINT('Ctrl Pts',(-0.394841037195299,-4.88654889560929,
6.24277782189594));
#45985=CARTESIAN_POINT('Ctrl Pts',(1.99044525726845,-4.48022178375707,6.32214971194934));
#45986=CARTESIAN_POINT('Ctrl Pts',(3.89086349283745,-2.98252256218433,6.40152160200274));
#45987=CARTESIAN_POINT('Ctrl Pts',(4.84347599383151,-0.758287446165202,
6.48089349205615));
#45988=CARTESIAN_POINT('Ctrl Pts',(4.61622846358046,1.65066481329898,6.56026538210956));
#45989=CARTESIAN_POINT('Ctrl Pts',(3.26447789744962,3.65751877792811,6.63963727216296));
#45990=CARTESIAN_POINT('Ctrl Pts',(1.11750774129931,4.77340926403445,6.71900916221636));
#45991=CARTESIAN_POINT('Ctrl Pts',(-1.30168482707007,4.7265078191842,6.79838105226977));
#45992=CARTESIAN_POINT('Ctrl Pts',(-3.4037898527957,3.52823953152828,6.87775294232317));
#45993=CARTESIAN_POINT('Ctrl Pts',(-4.67673920454132,1.4704999036178,6.95712483237657));
#45994=CARTESIAN_POINT('Ctrl Pts',(-4.81044523784733,-0.945450245917632,
7.03649672242998));
#45995=CARTESIAN_POINT('Ctrl Pts',(-3.77233745895366,-3.13109080826615,
7.11586861248337));
#45996=CARTESIAN_POINT('Ctrl Pts',(-1.81529662498623,-4.554004580273,7.19524050253679));
#45997=CARTESIAN_POINT('Ctrl Pts',(0.583946448736947,-4.8675729166435,7.27461239259018));
#45998=CARTESIAN_POINT('Ctrl Pts',(2.84094146009133,-3.99541126470955,7.3539842826436));
#45999=CARTESIAN_POINT('Ctrl Pts',(4.40588942008474,-2.14997627238517,7.433356172697));
#46000=CARTESIAN_POINT('Ctrl Pts',(4.8975724696163,0.219188181000477,7.51272806275039));
#46001=CARTESIAN_POINT('Ctrl Pts',(4.19621770614212,2.53495887865921,7.59209995280381));
#46002=CARTESIAN_POINT('Ctrl Pts',(2.47267359762208,4.23321920451286,7.6714718428572));
#46003=CARTESIAN_POINT('Ctrl Pts',(0.14679167389147,4.90027670221897,7.75084373291062));
#46004=CARTESIAN_POINT('Ctrl Pts',(-2.21484837668125,4.37363764184302,7.83021562296401));
#46005=CARTESIAN_POINT('Ctrl Pts',(-4.03695626517815,2.78159013279685,7.90958751301742));
#46006=CARTESIAN_POINT('Ctrl Pts',(-4.87567054312876,0.511953424346666,
7.98895940307082));
#46007=CARTESIAN_POINT('Ctrl Pts',(-4.52668226888691,-1.88239400508467,
8.06833129312423));
#46008=CARTESIAN_POINT('Ctrl Pts',(-3.07500421358545,-3.81819442148583,
8.14770318317762));
#46009=CARTESIAN_POINT('Ctrl Pts',(-0.874261938260974,-4.82389112824304,
8.22707507323104));
#46010=CARTESIAN_POINT('Ctrl Pts',(1.53944861007788,-4.65449863366217,8.30644696328443));
#46011=CARTESIAN_POINT('Ctrl Pts',(3.5781528845135,-3.35128057447919,8.38581885333784));
#46012=CARTESIAN_POINT('Ctrl Pts',(4.74522703638871,-1.23169798528678,8.46519074339124));
#46013=CARTESIAN_POINT('Ctrl Pts',(4.75637438558149,1.18792350680425,8.54456263344465));
#46014=CARTESIAN_POINT('Ctrl Pts',(3.60887946250276,3.31816946206181,8.62393452349805));
#46015=CARTESIAN_POINT('Ctrl Pts',(1.58226949047756,4.64011668100466,8.70330641355145));
#46016=CARTESIAN_POINT('Ctrl Pts',(-0.829777827133893,4.83174174717884,
8.78267830360486));
#46017=CARTESIAN_POINT('Ctrl Pts',(-3.03969310273758,3.84636521861918,8.86205019365827));
#46018=CARTESIAN_POINT('Ctrl Pts',(-4.50914586676094,1.9240226365889,8.94142208371166));
#46019=CARTESIAN_POINT('Ctrl Pts',(-4.88018067846642,-0.467007600962554,
9.02079397376508));
#46020=CARTESIAN_POINT('Ctrl Pts',(-4.0624142789942,-2.74427582062334,9.10016586381847));
#46021=CARTESIAN_POINT('Ctrl Pts',(-2.25505275316047,-4.35304452473175,
9.17953775387187));
#46022=CARTESIAN_POINT('Ctrl Pts',(0.101634631868527,-4.90142121791617,
9.25890964392528));
#46023=CARTESIAN_POINT('Ctrl Pts',(2.4335640455388,-4.25582255152803,9.33828153397868));
#46024=CARTESIAN_POINT('Ctrl Pts',(4.17268264431847,-2.57351493169112,9.41765342403209));
#46025=CARTESIAN_POINT('Ctrl Pts',(4.89534498701854,-0.264304770872935,
9.49702531408549));
#46026=CARTESIAN_POINT('Ctrl Pts',(4.42551212654324,2.10928944710123,9.57639720413889));
#46027=CARTESIAN_POINT('Ctrl Pts',(2.8776343077469,3.96906542459454,9.65576909419229));
#46028=CARTESIAN_POINT('Ctrl Pts',(0.628771141118955,4.86198585003388,9.73514098424571));
#46029=CARTESIAN_POINT('Ctrl Pts',(-1.77325928372426,4.57053728422814,9.81451287429909));
#46030=CARTESIAN_POINT('Ctrl Pts',(-3.74332767209512,3.16571595269709,9.89388476435253));
#46031=CARTESIAN_POINT('Ctrl Pts',(-4.80152972525885,0.989733222282404,
9.97325665440589));
#46032=CARTESIAN_POINT('Ctrl Pts',(-4.69008976535528,-1.42734633034291,
10.0526285444593));
#46033=CARTESIAN_POINT('Ctrl Pts',(-3.43615431994881,-3.49672747627419,
10.1320004345127));
#46034=CARTESIAN_POINT('Ctrl Pts',(-1.34517928800141,-4.71431354886008,
10.2113723245661));
#46035=CARTESIAN_POINT('Ctrl Pts',(1.07347844099931,-4.78350327589974,10.2907442146195));
#46036=CARTESIAN_POINT('Ctrl Pts',(3.23063919787684,-3.68744219303511,10.3701161046729));
#46037=CARTESIAN_POINT('Ctrl Pts',(4.60082339705013,-1.69312835396196,10.4494879947263));
#46038=CARTESIAN_POINT('Ctrl Pts',(4.85025720045185,0.713627804460256,10.5288598847798));
#46039=CARTESIAN_POINT('Ctrl Pts',(3.91817908568572,2.94654580930431,10.6082317748331));
#46040=CARTESIAN_POINT('Ctrl Pts',(2.03164121838884,4.46169177707037,10.6876036648866));
#46041=CARTESIAN_POINT('Ctrl Pts',(-0.349799952746016,4.8899795037293,10.7669755549399));
#46042=CARTESIAN_POINT('Ctrl Pts',(-2.64603062966098,4.12707904706582,10.8463474449934));
#46043=CARTESIAN_POINT('Ctrl Pts',(-4.29769410207999,2.35883126967163,10.9257193350467));
#46044=CARTESIAN_POINT('Ctrl Pts',(-4.90244880401686,0.0159774161698882,
11.0050912251002));
#46045=CARTESIAN_POINT('Ctrl Pts',(-4.31297782868159,-2.33076850054543,
11.0844631151536));
#46046=CARTESIAN_POINT('Ctrl Pts',(-2.672875000894,-4.10974436959645,11.163835005207));
#46047=CARTESIAN_POINT('Ctrl Pts',(-0.381665739197088,-4.88759560697865,
11.2432068952604));
#46048=CARTESIAN_POINT('Ctrl Pts',(2.00251645176545,-4.47483937301022,11.3225787853138));
#46049=CARTESIAN_POINT('Ctrl Pts',(3.89889006757291,-2.97202217266546,11.4019506753672));
#46050=CARTESIAN_POINT('Ctrl Pts',(4.84550269296641,-0.745226949518873,
11.4813225654206));
#46051=CARTESIAN_POINT('Ctrl Pts',(4.61176158769154,1.66310390899864,11.560694455474));
#46052=CARTESIAN_POINT('Ctrl Pts',(3.25460556761616,3.66630633650213,11.6400663455274));
#46053=CARTESIAN_POINT('Ctrl Pts',(1.10463483521672,4.77640465566513,11.7194382355808));
#46054=CARTESIAN_POINT('Ctrl Pts',(-1.3144224979738,4.72298137310049,11.7988101256342));
#46055=CARTESIAN_POINT('Ctrl Pts',(-3.41328942008276,3.51905028219049,11.8781820156876));
#46056=CARTESIAN_POINT('Ctrl Pts',(-4.6806865946475,1.45788633182458,11.957553905741));
#46057=CARTESIAN_POINT('Ctrl Pts',(-4.80787887528018,-0.95841550199713,
12.0369257957944));
#46058=CARTESIAN_POINT('Ctrl Pts',(-3.76388250395398,-3.14124944094907,
12.1162976858478));
#46059=CARTESIAN_POINT('Ctrl Pts',(-1.80301268587722,-4.55888196912352,
12.1956695759012));
#46060=CARTESIAN_POINT('Ctrl Pts',(0.59706703157835,-4.86598094053357,12.2750414659546));
#46061=CARTESIAN_POINT('Ctrl Pts',(2.8517025417269,-3.98773772549578,12.354413356008));
#46062=CARTESIAN_POINT('Ctrl Pts',(4.41166962484727,-2.13809042723494,12.4337852460614));
#46063=CARTESIAN_POINT('Ctrl Pts',(4.89696375241996,0.232390966517433,12.5131571361148));
#46064=CARTESIAN_POINT('Ctrl Pts',(4.18936834914853,2.54626243521486,12.5925290261683));
#46065=CARTESIAN_POINT('Ctrl Pts',(2.46125208903407,4.23987001075024,12.6719009162216));
#46066=CARTESIAN_POINT('Ctrl Pts',(0.133580267920011,4.90065463645993,12.751272806275));
#46067=CARTESIAN_POINT('Ctrl Pts',(-2.22663141078444,4.36765064014303,12.8306446963284));
#46068=CARTESIAN_POINT('Ctrl Pts',(-4.04444060638688,2.770696615518,12.9100165863818));
#46069=CARTESIAN_POINT('Ctrl Pts',(-4.87703302249085,0.498807028185692,
12.9893884764353));
#46070=CARTESIAN_POINT('Ctrl Pts',(-4.52159098944558,-1.89459084712199,
13.0687603664886));
#46071=CARTESIAN_POINT('Ctrl Pts',(-3.06469939974324,-3.82647058567648,
13.1481322565421));
#46072=CARTESIAN_POINT('Ctrl Pts',(-0.861253819860521,-4.82623055930914,
13.2275041465954));
#46073=CARTESIAN_POINT('Ctrl Pts',(1.55199128418723,-4.65033145137426,13.3068760366489));
#46074=CARTESIAN_POINT('Ctrl Pts',(3.58717474668141,-3.34162189521869,13.3862479267023));
#46075=CARTESIAN_POINT('Ctrl Pts',(4.74853038096063,-1.21890064194246,13.4656198167557));
#46076=CARTESIAN_POINT('Ctrl Pts',(4.75315452513156,1.20074210972015,13.5449917068091));
#46077=CARTESIAN_POINT('Ctrl Pts',(3.59992074790953,3.32788674125251,13.6243635968625));
#46078=CARTESIAN_POINT('Ctrl Pts',(1.56975424478615,4.64436552876813,13.7037354869159));
#46079=CARTESIAN_POINT('Ctrl Pts',(-0.842800917775063,4.82948715360455,
13.7831073769693));
#46080=CARTESIAN_POINT('Ctrl Pts',(-3.05005164227443,3.83815639771137,13.8624792670227));
#46081=CARTESIAN_POINT('Ctrl Pts',(-4.51431653789056,1.91185923895083,13.9418511570761));
#46082=CARTESIAN_POINT('Ctrl Pts',(-4.87890391714672,-0.480162598589543,
14.0212230471295));
#46083=CARTESIAN_POINT('Ctrl Pts',(-4.05500110145656,-2.75521788993537,
14.1005949371829));
#46084=CARTESIAN_POINT('Ctrl Pts',(-2.24330899304429,-4.35910820186428,
14.1799668272363));
#46085=CARTESIAN_POINT('Ctrl Pts',(0.114848220593315,-4.90112940454139,
14.2593387172897));
#46086=CARTESIAN_POINT('Ctrl Pts',(2.4450286619066,-4.2492463327382,14.3387106073431));
#46087=CARTESIAN_POINT('Ctrl Pts',(4.17960553315863,-2.56225625982719,14.4180824973965));
#46088=CARTESIAN_POINT('Ctrl Pts',(4.89603974793314,-0.2511062334803,14.4974543874499));
#46089=CARTESIAN_POINT('Ctrl Pts',(4.41980951731128,2.12121271552818,14.5768262775033));
#46090=CARTESIAN_POINT('Ctrl Pts',(2.86692347135483,3.97680894225867,14.6561981675567));
#46091=CARTESIAN_POINT('Ctrl Pts',(0.615661213603817,4.86366331317225,14.7355700576101));
#46092=CARTESIAN_POINT('Ctrl Pts',(-1.78557475303814,4.56574006653321,14.8149419476636));
#46093=CARTESIAN_POINT('Ctrl Pts',(-3.75184866214265,3.15561264578087,14.8943138377169));
#46094=CARTESIAN_POINT('Ctrl Pts',(-4.80418054172537,0.976784969346447,
14.9736857277704));
#46095=CARTESIAN_POINT('Ctrl Pts',(-4.68622467521704,-1.43998536354391,
15.0530576178237));
#46096=CARTESIAN_POINT('Ctrl Pts',(-3.42671485060823,-3.50597844922854,
15.1324295078772));
#46097=CARTESIAN_POINT('Ctrl Pts',(-1.33246487329588,-4.71792294503274,
15.2118013979305));
#46098=CARTESIAN_POINT('Ctrl Pts',(1.08637059779033,-4.78059185437226,15.291173287984));
#46099=CARTESIAN_POINT('Ctrl Pts',(3.24056859589536,-3.67871916964732,15.3705451780373));
#46100=CARTESIAN_POINT('Ctrl Pts',(4.60537125691718,-1.68071863790306,15.4499170680908));
#46101=CARTESIAN_POINT('Ctrl Pts',(4.84831567357043,0.726701233826767,15.5292889581442));
#46102=CARTESIAN_POINT('Ctrl Pts',(3.91022112370653,2.95709829352236,15.6086608481976));
#46103=CARTESIAN_POINT('Ctrl Pts',(2.01960536323555,4.46715275434186,15.688032738251));
#46104=CARTESIAN_POINT('Ctrl Pts',(-0.362981793399331,4.88901869207872,
15.7674046283044));
#46105=CARTESIAN_POINT('Ctrl Pts',(-2.65714738860797,4.11993049808428,15.8467765183578));
#46106=CARTESIAN_POINT('Ctrl Pts',(-4.3040377614491,2.34723635406844,15.9261484084112));
#46107=CARTESIAN_POINT('Ctrl Pts',(-4.90247406242457,0.00276062972017743,
16.0055202984646));
#46108=CARTESIAN_POINT('Ctrl Pts',(-4.30667853324066,-2.34238757791569,
16.084892188518));
#46109=CARTESIAN_POINT('Ctrl Pts',(-2.66178564602119,-4.11693535636137,
16.1642640785714));
#46110=CARTESIAN_POINT('Ctrl Pts',(-0.368487667211246,-4.88860679467341,
16.2436359686248));
#46111=CARTESIAN_POINT('Ctrl Pts',(2.01457309173119,-4.46942443856166,16.3230078586782));
#46112=CARTESIAN_POINT('Ctrl Pts',(3.90688830464663,-2.96150018209857,16.4023797487316));
#46113=CARTESIAN_POINT('Ctrl Pts',(4.84749417442,-0.732161036485258,16.481751638785));
#46114=CARTESIAN_POINT('Ctrl Pts',(4.60726119282582,1.67553091707946,16.5611235288384));
#46115=CARTESIAN_POINT('Ctrl Pts',(3.24470958308425,3.67506724782763,16.6404954188918));
#46116=CARTESIAN_POINT('Ctrl Pts',(1.09175390014313,4.77936533189424,16.7198673089452));
#46117=CARTESIAN_POINT('Ctrl Pts',(-1.32715061480029,4.7194205995551,16.7992391989986));
#46118=CARTESIAN_POINT('Ctrl Pts',(-3.42276418043948,3.50983545637255,16.878611089052));
#46119=CARTESIAN_POINT('Ctrl Pts',(-4.68459996247752,1.44526216311684,16.9579829791054));
#46120=CARTESIAN_POINT('Ctrl Pts',(-4.80527757305004,-0.971373790661056,
17.0373548691589));
#46121=CARTESIAN_POINT('Ctrl Pts',(-3.75540018385452,-3.15138524551466,
17.1167267592122));
#46122=CARTESIAN_POINT('Ctrl Pts',(-1.79071565870356,-4.56372621798453,
17.1960986492656));
#46123=CARTESIAN_POINT('Ctrl Pts',(0.610183305945333,-4.86435360814148,
17.275470539319));
#46124=CARTESIAN_POINT('Ctrl Pts',(2.86244283812717,-3.98003518345987,17.3548424293725));
#46125=CARTESIAN_POINT('Ctrl Pts',(4.41741787585788,-2.1261890788619,17.4342143194258));
#46126=CARTESIAN_POINT('Ctrl Pts',(4.89631923419534,0.245592132270697,17.5135862094793));
#46127=CARTESIAN_POINT('Ctrl Pts',(4.1824889384277,2.55754735438707,17.5929580995327));
#46128=CARTESIAN_POINT('Ctrl Pts',(2.44981194564648,4.24649024808584,17.6723299895861));
#46129=CARTESIAN_POINT('Ctrl Pts',(0.120369299865439,4.90099648569508,17.7517018796395));
#46130=CARTESIAN_POINT('Ctrl Pts',(-2.2384009215371,4.36163277449207,17.8310737696929));
#46131=CARTESIAN_POINT('Ctrl Pts',(-4.0518905292873,2.75978129753081,17.9104456597463));
#46132=CARTESIAN_POINT('Ctrl Pts',(-4.87836953900975,0.485660146581001,
17.9898175497997));
#46133=CARTESIAN_POINT('Ctrl Pts',(-4.51644893866981,-1.90677984789346,
18.0691894398531));
#46134=CARTESIAN_POINT('Ctrl Pts',(-3.05440612489714,-3.83470774368921,
18.1485613299065));
#46135=CARTESIAN_POINT('Ctrl Pts',(-0.848175594775907,-4.82855605094715,
18.2279332199599));
#46136=CARTESIAN_POINT('Ctrl Pts',(1.56440212229575,-4.64609055668262,18.3073051100133));
#46137=CARTESIAN_POINT('Ctrl Pts',(3.59639816964341,-3.33201429213606,18.3866770000667));
#46138=CARTESIAN_POINT('Ctrl Pts',(4.75136940590255,-1.20595214372204,18.4660488901201));
#46139=CARTESIAN_POINT('Ctrl Pts',(4.75071159562135,1.21328335035095,18.5454207801735));
#46140=CARTESIAN_POINT('Ctrl Pts',(3.58940432897552,3.33808667681415,18.6247926702269));
#46141=CARTESIAN_POINT('Ctrl Pts',(1.56011376732896,4.64762681676405,18.7041645602803));
#46142=CARTESIAN_POINT('Ctrl Pts',(-0.861221142909775,4.82897211168874,
18.7835364503337));
#46143=CARTESIAN_POINT('Ctrl Pts',(-3.05056344532316,3.82678328180746,18.8629083403871));
#46144=CARTESIAN_POINT('Ctrl Pts',(-5.02992785007326,1.26296632184503,18.968737527125));
#46145=CARTESIAN_POINT('Ctrl Pts',(-4.59246965375637,-3.13076985705441,
19.1010240105473));
#46146=CARTESIAN_POINT('Ctrl Pts',(0.146932230206506,-5.55932874556365,
19.2597677906541));
#46147=CARTESIAN_POINT('Ctrl Pts',(4.74574684718979,-2.89085235699285,19.418511570761));
#46148=CARTESIAN_POINT('Ctrl Pts',(5.00517315099097,2.41778366488237,19.5772553508677));
#46149=CARTESIAN_POINT('Ctrl Pts',(0.682914143844855,5.5166676123404,19.7359991309746));
#46150=CARTESIAN_POINT('Ctrl Pts',(-4.26335305224441,3.56621538027044,19.8947429110814));
#46151=CARTESIAN_POINT('Ctrl Pts',(-5.30889903625343,-1.64699798333531,
20.0534866911882));
#46152=CARTESIAN_POINT('Ctrl Pts',(-1.49629817009909,-5.35305176256659,
20.212230471295));
#46153=CARTESIAN_POINT('Ctrl Pts',(3.68539651252336,-4.16147159288513,20.3709742514018));
#46154=CARTESIAN_POINT('Ctrl Pts',(5.49476366156206,0.839647798276105,20.5297180315086));
#46155=CARTESIAN_POINT('Ctrl Pts',(2.27623920304293,5.06930720888698,20.6884618116154));
#46156=CARTESIAN_POINT('Ctrl Pts',(-3.02540872545025,4.66632909528393,20.8472055917223));
#46157=CARTESIAN_POINT('Ctrl Pts',(-5.55807194231375,-0.0182675279713449,
21.005949371829));
#46158=CARTESIAN_POINT('Ctrl Pts',(-3.4318929716806,-3.88810606053727,21.1382358552514));
#46159=CARTESIAN_POINT('Ctrl Pts',(-0.348982623888803,-4.88143613581972,
21.2440650419892));
#46160=CARTESIAN_POINT('Ctrl Pts',(2.02316502874914,-4.46849826887164,21.3234369320426));
#46161=CARTESIAN_POINT('Ctrl Pts',(3.91669769333085,-2.94853678524969,21.4028088220961));
#46162=CARTESIAN_POINT('Ctrl Pts',(4.84847467696001,-0.720374489880037,
21.4821807121494));
#46163=CARTESIAN_POINT('Ctrl Pts',(4.60324425657816,1.68862650319429,21.5615526022029));
#46164=CARTESIAN_POINT('Ctrl Pts',(3.23451621663553,3.68344087079137,21.6409244922562));
#46165=CARTESIAN_POINT('Ctrl Pts',(1.07901003836815,4.78248223987442,21.7202963823097));
#46166=CARTESIAN_POINT('Ctrl Pts',(-1.33994588402651,4.71572438645636,21.7996682723631));
#46167=CARTESIAN_POINT('Ctrl Pts',(-3.4321733891171,3.50064868327975,21.8790401624164));
#46168=CARTESIAN_POINT('Ctrl Pts',(-4.68850082698247,1.43259912421573,21.9584120524699));
#46169=CARTESIAN_POINT('Ctrl Pts',(-4.80262992851033,-0.984309998791622,
22.0377839425233));
#46170=CARTESIAN_POINT('Ctrl Pts',(-3.74689662802585,-3.16150609615164,
22.1171558325767));
#46171=CARTESIAN_POINT('Ctrl Pts',(-1.77840238381691,-4.56853309419591,
22.1965277226301));
#46172=CARTESIAN_POINT('Ctrl Pts',(0.62329338871143,-4.86269313206684,22.2758996126835));
#46173=CARTESIAN_POINT('Ctrl Pts',(2.87316334475109,-3.97230257099384,22.3552715027369));
#46174=CARTESIAN_POINT('Ctrl Pts',(4.4231333235665,-2.11427282962158,22.4346433927903));
#46175=CARTESIAN_POINT('Ctrl Pts',(4.89563979914059,0.258791705958885,22.5140152828437));
#46176=CARTESIAN_POINT('Ctrl Pts',(4.17557820525643,2.56881377105699,22.5933871728971));
#46177=CARTESIAN_POINT('Ctrl Pts',(2.43835555951363,4.25307922033076,22.6727590629505));
#46178=CARTESIAN_POINT('Ctrl Pts',(0.107154601980389,4.90130359745224,22.7521309530039));
#46179=CARTESIAN_POINT('Ctrl Pts',(-2.25014882333759,4.35558147263095,22.8315028430573));
#46180=CARTESIAN_POINT('Ctrl Pts',(-4.05932105856842,2.74884923313531,22.9108747331107));
#46181=CARTESIAN_POINT('Ctrl Pts',(-4.87965162531074,0.472503462573818,
22.9902466231641));
#46182=CARTESIAN_POINT('Ctrl Pts',(-4.51130988023697,-1.91894313613435,
23.0696185132175));
#46183=CARTESIAN_POINT('Ctrl Pts',(-3.04402302167418,-3.84293941821872,
23.1489904032709));
#46184=CARTESIAN_POINT('Ctrl Pts',(-0.835218899364871,-4.83080417279082,
23.2283622933243));
#46185=CARTESIAN_POINT('Ctrl Pts',(1.57704270154782,-4.64189571913938,23.3077341833777));
#46186=CARTESIAN_POINT('Ctrl Pts',(3.60514018926443,-3.32223174536946,23.3871060734312));
#46187=CARTESIAN_POINT('Ctrl Pts',(4.75503350768461,-1.19327947079072,23.4664779634845));
#46188=CARTESIAN_POINT('Ctrl Pts',(4.74661118820946,1.22635304091963,23.545849853538));
#46189=CARTESIAN_POINT('Ctrl Pts',(3.58192489000304,3.34724866670522,23.6252217435913));
#46190=CARTESIAN_POINT('Ctrl Pts',(1.54468961690465,4.65276192610169,23.7045936336447));
#46191=CARTESIAN_POINT('Ctrl Pts',(-0.868828627683255,4.82487267911367,
23.7839655236982));
#46192=CARTESIAN_POINT('Ctrl Pts',(-3.0707021417273,3.8216551271151,23.8633374137516));
#46193=CARTESIAN_POINT('Ctrl Pts',(-4.52455941090918,1.88749084526948,23.9427093038049));
#46194=CARTESIAN_POINT('Ctrl Pts',(-4.8762440225472,-0.506462028608541,
24.0220811938584));
#46195=CARTESIAN_POINT('Ctrl Pts',(-4.04008638366986,-2.77704187334428,
24.1014530839117));
#46196=CARTESIAN_POINT('Ctrl Pts',(-2.21977264431323,-4.37114046461548,
24.1808249739652));
#46197=CARTESIAN_POINT('Ctrl Pts',(0.141272797816377,-4.90043891405946,
24.2601968640185));
#46198=CARTESIAN_POINT('Ctrl Pts',(2.46790449909909,-4.23600129097727,24.339568754072));
#46199=CARTESIAN_POINT('Ctrl Pts',(4.19336012701565,-2.53968312964219,24.4189406441254));
#46200=CARTESIAN_POINT('Ctrl Pts',(4.89732250983615,-0.224703779419903,
24.4983125341788));
#46201=CARTESIAN_POINT('Ctrl Pts',(4.40830796930024,2.14501291409586,24.5776844242322));
#46202=CARTESIAN_POINT('Ctrl Pts',(2.84543936506689,3.99220920964338,24.6570563142856));
#46203=CARTESIAN_POINT('Ctrl Pts',(0.589428029776467,4.86691217832701,24.736428204339));
#46204=CARTESIAN_POINT('Ctrl Pts',(-1.8101666688907,4.5560461130975,24.8158000943924));
#46205=CARTESIAN_POINT('Ctrl Pts',(-3.76880877375201,3.13533729935451,24.8951719844458));
#46206=CARTESIAN_POINT('Ctrl Pts',(-4.80937740344408,0.950867259440163,
24.9745438744992));
#46207=CARTESIAN_POINT('Ctrl Pts',(-4.67839234303351,-1.46523194016486,
25.0539157645526));
#46208=CARTESIAN_POINT('Ctrl Pts',(-3.40776126330575,-3.52440388238162,
25.133287654606));
#46209=CARTESIAN_POINT('Ctrl Pts',(-1.30700708278832,-4.72503883998586,
25.2126595446594));
#46210=CARTESIAN_POINT('Ctrl Pts',(1.11213113008524,-4.77466479486562,25.2920314347128));
#46211=CARTESIAN_POINT('Ctrl Pts',(3.26035666133054,-3.66119297425736,25.3714033247662));
#46212=CARTESIAN_POINT('Ctrl Pts',(4.61436652655277,-1.65586264903317,25.4507752148196));
#46213=CARTESIAN_POINT('Ctrl Pts',(4.84432691963378,0.752832152305638,25.530147104873));
#46214=CARTESIAN_POINT('Ctrl Pts',(3.89421999782782,2.97813870770851,25.6095189949265));
#46215=CARTESIAN_POINT('Ctrl Pts',(1.99548970426076,4.47797726591181,25.6888908849798));
#46216=CARTESIAN_POINT('Ctrl Pts',(-0.389337464322654,4.88699047397359,
25.7682627750333));
#46217=CARTESIAN_POINT('Ctrl Pts',(-2.67932288838098,4.10554361974534,25.8476346650867));
#46218=CARTESIAN_POINT('Ctrl Pts',(-4.31663118741032,2.32399542721376,25.92700655514));
#46219=CARTESIAN_POINT('Ctrl Pts',(-4.90241768388754,-0.0236729073104641,
26.0063784451935));
#46220=CARTESIAN_POINT('Ctrl Pts',(-4.29398608388724,-2.36557457401295,
26.0857503352468));
#46221=CARTESIAN_POINT('Ctrl Pts',(-2.63954897842897,-4.13122751059639,
26.1651222253003));
#46222=CARTESIAN_POINT('Ctrl Pts',(-0.342123584367958,-4.89052256991551,
26.2444941153537));
#46223=CARTESIAN_POINT('Ctrl Pts',(2.03864235756733,-4.45849715619131,26.323866005407));
#46224=CARTESIAN_POINT('Ctrl Pts',(3.92279953365755,-2.94039170393502,26.4032378954605));
#46225=CARTESIAN_POINT('Ctrl Pts',(4.85137142631832,-0.706013341046749,
26.4826097855139));
#46226=CARTESIAN_POINT('Ctrl Pts',(4.59815997785643,1.70034830898648,26.5619816755673));
#46227=CARTESIAN_POINT('Ctrl Pts',(3.22484693664317,3.69250887460774,26.6413535656207));
#46228=CARTESIAN_POINT('Ctrl Pts',(1.06596831974129,4.78518245160429,26.7207254556741));
#46229=CARTESIAN_POINT('Ctrl Pts',(-1.3525778203687,4.71219617521178,26.8000973457275));
#46230=CARTESIAN_POINT('Ctrl Pts',(-3.44163899731715,3.49132934080697,26.8794692357809));
#46231=CARTESIAN_POINT('Ctrl Pts',(-4.69232453245783,1.419982406908,26.9588411258343));
#46232=CARTESIAN_POINT('Ctrl Pts',(-4.79997019777595,-0.997269098236029,
27.0382130158877));
#46233=CARTESIAN_POINT('Ctrl Pts',(-3.73835374746968,-3.17158805846741,
27.1175849059411));
#46234=CARTESIAN_POINT('Ctrl Pts',(-1.7660825989855,-4.57331518784726,27.1969567959945));
#46235=CARTESIAN_POINT('Ctrl Pts',(0.636402361454069,-4.860992860329,27.2763286860479));
#46236=CARTESIAN_POINT('Ctrl Pts',(2.88386111529617,-3.96454343165977,27.3557005761013));
#46237=CARTESIAN_POINT('Ctrl Pts',(4.42881768477039,-2.10233999840624,27.4350724661547));
#46238=CARTESIAN_POINT('Ctrl Pts',(4.89492406925623,0.271988805008393,27.5144443562081));
#46239=CARTESIAN_POINT('Ctrl Pts',(4.16863778520187,2.58006173756,27.5938162462615));
#46240=CARTESIAN_POINT('Ctrl Pts',(2.42688056379555,4.25963734171175,27.673188136315));
#46241=CARTESIAN_POINT('Ctrl Pts',(0.0939406088576867,4.90157471796985,
27.7525600263683));
#46242=CARTESIAN_POINT('Ctrl Pts',(-2.2618830704639,4.34949934238213,27.8319319164218));
#46243=CARTESIAN_POINT('Ctrl Pts',(-4.06671704041374,2.73789555444364,27.9113038064751));
#46244=CARTESIAN_POINT('Ctrl Pts',(-4.88090774084432,0.45934646967172,27.9906756965286));
#46245=CARTESIAN_POINT('Ctrl Pts',(-4.50612011931125,-1.93109839836612,
28.0700475865819));
#46246=CARTESIAN_POINT('Ctrl Pts',(-3.03365161084166,-3.85113197097576,
28.1494194766353));
#46247=CARTESIAN_POINT('Ctrl Pts',(-0.822192284844965,-4.83303831979172,
28.2287913666888));
#46248=CARTESIAN_POINT('Ctrl Pts',(1.5895512618482,-4.63762723165528,28.3081632567421));
#46249=CARTESIAN_POINT('Ctrl Pts',(3.61408363956719,-3.31250041510136,28.3875351467956));
#46250=CARTESIAN_POINT('Ctrl Pts',(4.75823324232603,-1.18045582952402,28.4669070368489));
#46251=CARTESIAN_POINT('Ctrl Pts',(4.7432877594249,1.23914518323065,28.5462789269024));
#46252=CARTESIAN_POINT('Ctrl Pts',(3.57288787741725,3.35689317215169,28.6256508169558));
#46253=CARTESIAN_POINT('Ctrl Pts',(1.53214041692396,4.65690941469359,28.7050227070092));
#46254=CARTESIAN_POINT('Ctrl Pts',(-0.881833057796704,4.82251283171032,
28.7843945970626));
#46255=CARTESIAN_POINT('Ctrl Pts',(-3.08099395154251,3.81336279737351,28.863766487116));
#46256=CARTESIAN_POINT('Ctrl Pts',(-4.52963153835698,1.87528602633188,28.9431383771694));
#46257=CARTESIAN_POINT('Ctrl Pts',(-4.87486090859702,-0.519606269848997,
29.0225102672228));
#46258=CARTESIAN_POINT('Ctrl Pts',(-4.03258495182442,-2.78792362882362,
29.1018821572762));
#46259=CARTESIAN_POINT('Ctrl Pts',(-2.20798022676276,-4.37710896278109,
29.1812540473296));
#46260=CARTESIAN_POINT('Ctrl Pts',(0.154483594256982,-4.90004024197141,
29.260625937383));
#46261=CARTESIAN_POINT('Ctrl Pts',(2.47931555365931,-4.22933256427261,29.3399978274364));
#46262=CARTESIAN_POINT('Ctrl Pts',(4.20019173206215,-2.52836883538588,29.4193697174898));
#46263=CARTESIAN_POINT('Ctrl Pts',(4.89791050150138,-0.211500054648609,
29.4987416075432));
#46264=CARTESIAN_POINT('Ctrl Pts',(4.40250911411586,2.15688967125365,29.5781134975966));
#46265=CARTESIAN_POINT('Ctrl Pts',(2.83466625132033,3.9998658474328,29.65748538765));
#46266=CARTESIAN_POINT('Ctrl Pts',(0.576304964130538,4.86848355673019,29.7368572777034));
#46267=CARTESIAN_POINT('Ctrl Pts',(-1.82244293669206,4.55114944781371,29.8162291677568));
#46268=CARTESIAN_POINT('Ctrl Pts',(-3.77724777204552,3.12516540720823,29.8956010578102));
#46269=CARTESIAN_POINT('Ctrl Pts',(-4.81192341092482,0.937897990843109,
29.9749729478637));
#46270=CARTESIAN_POINT('Ctrl Pts',(-4.67442515791461,-1.47783930008941,
30.0543448379171));
#46271=CARTESIAN_POINT('Ctrl Pts',(-3.39824728310101,-3.5335782086619,30.1337167279704));
#46272=CARTESIAN_POINT('Ctrl Pts',(-1.29426389201682,-4.7285452870471,30.2130886180239));
#46273=CARTESIAN_POINT('Ctrl Pts',(1.12499931835819,-4.77164919996508,30.2924605080772));
#46274=CARTESIAN_POINT('Ctrl Pts',(3.27021518492489,-3.65238992963792,30.3718323981307));
#46275=CARTESIAN_POINT('Ctrl Pts',(4.61881387094242,-1.64341655687892,30.451204288184));
#46276=CARTESIAN_POINT('Ctrl Pts',(4.84227972156944,0.765889451494932,30.5305761782375));
#46277=CARTESIAN_POINT('Ctrl Pts',(3.88617695022651,2.98862648475217,30.6099480682908));
#46278=CARTESIAN_POINT('Ctrl Pts',(1.98341007571514,4.48334072153628,30.6893199583443));
#46279=CARTESIAN_POINT('Ctrl Pts',(-0.40251110303664,4.8859230822605,30.7686918483976));
#46280=CARTESIAN_POINT('Ctrl Pts',(-2.69038146803192,4.09830539495341,30.8480637384511));
#46281=CARTESIAN_POINT('Ctrl Pts',(-4.322880862473,2.3123495848808,30.9274356285044));
#46282=CARTESIAN_POINT('Ctrl Pts',(-4.90233604735018,-0.0368894657697565,
31.0068075185579));
#46283=CARTESIAN_POINT('Ctrl Pts',(-4.28759302222965,-2.3771423242123,31.0861794086113));
#46284=CARTESIAN_POINT('Ctrl Pts',(-2.62840182732014,-4.13832857419201,
31.1655512986647));
#46285=CARTESIAN_POINT('Ctrl Pts',(-0.328937765144189,-4.89142714353344,
31.2449231887181));
#46286=CARTESIAN_POINT('Ctrl Pts',(2.05065480852948,-4.45298488770047,31.3242950787715));
#46287=CARTESIAN_POINT('Ctrl Pts',(3.93071240989281,-2.9298053697385,31.4036669688249));
#46288=CARTESIAN_POINT('Ctrl Pts',(4.85325716869055,-0.692931748722414,
31.4830388588783));
#46289=CARTESIAN_POINT('Ctrl Pts',(4.59355922369783,1.712738512504,31.5624107489317));
#46290=CARTESIAN_POINT('Ctrl Pts',(3.21488041948321,3.70118946316684,31.6417826389851));
#46291=CARTESIAN_POINT('Ctrl Pts',(1.05306386109957,4.78803885304619,31.7211545290385));
#46292=CARTESIAN_POINT('Ctrl Pts',(-1.36527672293062,4.70853257646772,31.8005264190919));
#46293=CARTESIAN_POINT('Ctrl Pts',(-3.45103891924366,3.48203818642175,31.8798983091454));
#46294=CARTESIAN_POINT('Ctrl Pts',(-4.69613567357401,1.40732700152429,31.9592701991987));
#46295=CARTESIAN_POINT('Ctrl Pts',(-4.79726417254176,-1.010205925879,32.0386420892522));
#46296=CARTESIAN_POINT('Ctrl Pts',(-3.72978973764247,-3.1816549257911,32.1180139793055));
#46297=CARTESIAN_POINT('Ctrl Pts',(-1.75374677840301,-4.57805982825421,
32.197385869359));
#46298=CARTESIAN_POINT('Ctrl Pts',(0.649505014202782,-4.85925948991811,
32.2767577594123));
#46299=CARTESIAN_POINT('Ctrl Pts',(2.89453882300369,-3.95675429562642,32.3561296494657));
#46300=CARTESIAN_POINT('Ctrl Pts',(4.43446938147393,-2.09039251304725,32.4355015395192));
#46301=CARTESIAN_POINT('Ctrl Pts',(4.89417301414864,0.285184258704931,32.5148734295725));
#46302=CARTESIAN_POINT('Ctrl Pts',(4.16166693364494,2.59129077628124,32.594245319626));
#46303=CARTESIAN_POINT('Ctrl Pts',(2.41538799979881,4.26616459648027,32.6736172096793));
#46304=CARTESIAN_POINT('Ctrl Pts',(0.0807258955723594,4.90181016397187,
32.7529890997328));
#46305=CARTESIAN_POINT('Ctrl Pts',(-2.2736008581318,4.34338562549266,32.8323609897862));
#46306=CARTESIAN_POINT('Ctrl Pts',(-4.07408347532516,2.72692196256443,32.9117328798396));
#46307=CARTESIAN_POINT('Ctrl Pts',(-4.88212837576012,0.446186145494932,
32.991104769893));
#46308=CARTESIAN_POINT('Ctrl Pts',(-4.5008976102678,-1.94323962900084,33.0704766599464));
#46309=CARTESIAN_POINT('Ctrl Pts',(-3.02325814948215,-3.85929653115999,
33.1498485499998));
#46310=CARTESIAN_POINT('Ctrl Pts',(-0.809159695351077,-4.83523734073656,
33.2292204400532));
#46311=CARTESIAN_POINT('Ctrl Pts',(1.60204826952296,-4.63332503672604,33.3085923301066));
#46312=CARTESIAN_POINT('Ctrl Pts',(3.6230008220149,-3.30274500946005,33.3879642201599));
#46313=CARTESIAN_POINT('Ctrl Pts',(4.76139839364027,-1.16762360839165,33.4673361102135));
#46314=CARTESIAN_POINT('Ctrl Pts',(4.73992985575147,1.25192831918992,33.5467080002668));
#46315=CARTESIAN_POINT('Ctrl Pts',(3.56382489665835,3.36651327931318,33.6260798903203));
#46316=CARTESIAN_POINT('Ctrl Pts',(1.51958008113186,4.66102305624645,33.7054517803736));
#46317=CARTESIAN_POINT('Ctrl Pts',(-0.894831078624851,4.82011793367764,
33.784823670427));
#46318=CARTESIAN_POINT('Ctrl Pts',(-3.09126336830355,3.80504275161507,33.8641955604804));
#46319=CARTESIAN_POINT('Ctrl Pts',(-4.53467074385896,1.86306757757831,33.9435674505338));
#46320=CARTESIAN_POINT('Ctrl Pts',(-4.87344236353374,-0.532746734526401,
34.0229393405872));
#46321=CARTESIAN_POINT('Ctrl Pts',(-4.02505421063338,-2.79878512131536,
34.1023112306406));
#46322=CARTESIAN_POINT('Ctrl Pts',(-2.19617176132914,-4.38304564755766,
34.181683120694));
#46323=CARTESIAN_POINT('Ctrl Pts',(0.167693267891119,-4.89960595576193,
34.2610550107475));
#46324=CARTESIAN_POINT('Ctrl Pts',(2.4907085882359,-4.22263309823643,34.3404269008008));
#46325=CARTESIAN_POINT('Ctrl Pts',(4.20699280957637,-2.51703616462034,34.4197987908543));
#46326=CARTESIAN_POINT('Ctrl Pts',(4.89846289452463,-0.198294792667773,
34.4991706809077));
#46327=CARTESIAN_POINT('Ctrl Pts',(4.39667826093041,2.16875075186054,34.578542570961));
#46328=CARTESIAN_POINT('Ctrl Pts',(2.82387253485585,4.00749341368399,34.6579144610145));
#46329=CARTESIAN_POINT('Ctrl Pts',(0.563177709826186,4.87001955037029,34.7372863510678));
#46330=CARTESIAN_POINT('Ctrl Pts',(-1.83470595874441,4.54621970419178,34.8166582411213));
#46331=CARTESIAN_POINT('Ctrl Pts',(-3.78565931681763,3.11497080095877,34.8960301311746));
#46332=CARTESIAN_POINT('Ctrl Pts',(-4.81443444472882,0.924921905483118,
34.9754020212281));
#46333=CARTESIAN_POINT('Ctrl Pts',(-4.67042399847396,-1.49043591888832,
35.0547739112815));
#46334=CARTESIAN_POINT('Ctrl Pts',(-3.38870860399896,-3.5427268524425,35.1341458013349));
#46335=CARTESIAN_POINT('Ctrl Pts',(-1.28151129436916,-4.73201736643453,
35.2135176913883));
#46336=CARTESIAN_POINT('Ctrl Pts',(1.13785932999185,-4.76859892410594,35.2928895814417));
#46337=CARTESIAN_POINT('Ctrl Pts',(3.28004994017574,-3.64356033897983,35.3722614714951));
#46338=CARTESIAN_POINT('Ctrl Pts',(4.62322764520025,-1.63095852016229,35.4516333615485));
#46339=CARTESIAN_POINT('Ctrl Pts',(4.84019732919482,0.77894118410138,35.5310052516019));
#46340=CARTESIAN_POINT('Ctrl Pts',(3.87810565739256,2.99909254007502,35.6103771416553));
#46341=CARTESIAN_POINT('Ctrl Pts',(1.97131603149074,4.48867159166511,35.6897490317087));
#46342=CARTESIAN_POINT('Ctrl Pts',(-0.415681816248198,4.88482017903162,
35.7691209217621));
#46343=CARTESIAN_POINT('Ctrl Pts',(-2.70142049364518,4.09103738315207,35.8484928118155));
#46344=CARTESIAN_POINT('Ctrl Pts',(-4.32909911828301,2.30068693609431,35.9278647018689));
#46345=CARTESIAN_POINT('Ctrl Pts',(-4.90221878000546,-0.0501057561118174,
36.0072365919223));
#46346=CARTESIAN_POINT('Ctrl Pts',(-4.28116879779583,-2.38869279703632,
36.0866084819757));
#46347=CARTESIAN_POINT('Ctrl Pts',(-2.61723557264952,-4.14539955988464,
36.1659803720291));
#46348=CARTESIAN_POINT('Ctrl Pts',(-0.315749555158452,-4.89229616563135,
36.2453522620825));
#46349=CARTESIAN_POINT('Ctrl Pts',(2.06265235506943,-4.44744025434409,36.3247241521359));
#46350=CARTESIAN_POINT('Ctrl Pts',(3.93859671720591,-2.9191977413407,36.4040960421893));
#46351=CARTESIAN_POINT('Ctrl Pts',(4.85510763696701,-0.679845120081316,
36.4834679322428));
#46352=CARTESIAN_POINT('Ctrl Pts',(4.58892508296144,1.72511626761826,36.5628398222961));
#46353=CARTESIAN_POINT('Ctrl Pts',(3.20489053615983,3.70984315100612,36.6422117123496));
#46354=CARTESIAN_POINT('Ctrl Pts',(1.04015174865454,4.7908604544074,36.721583602403));
#46355=CARTESIAN_POINT('Ctrl Pts',(-1.37796570248609,4.70483475550478,36.8009554924563));
#46356=CARTESIAN_POINT('Ctrl Pts',(-3.46041375857649,3.47272172413633,36.8803273825098));
#46357=CARTESIAN_POINT('Ctrl Pts',(-4.69991268257361,1.39466136750738,36.9596992725631));
#46358=CARTESIAN_POINT('Ctrl Pts',(-4.79452328017606,-1.02313541121578,
37.0390711626166));
#46359=CARTESIAN_POINT('Ctrl Pts',(-3.72119861922486,-3.19169866843862,
37.11844305267));
#46360=CARTESIAN_POINT('Ctrl Pts',(-1.74139821136397,-4.5827711947349,37.1978149427234));
#46361=CARTESIAN_POINT('Ctrl Pts',(0.66260294626563,-4.85749080178586,37.2771868327768));
#46362=CARTESIAN_POINT('Ctrl Pts',(2.90519549283168,-3.94893640139516,37.3565587228302));
#46363=CARTESIAN_POINT('Ctrl Pts',(4.44008884788513,-2.07842983444732,37.4359306128835));
#46364=CARTESIAN_POINT('Ctrl Pts',(4.8933863875636,0.298377639646022,37.515302502937));
#46365=CARTESIAN_POINT('Ctrl Pts',(4.15466583455884,2.60250098116825,37.5946743929904));
#46366=CARTESIAN_POINT('Ctrl Pts',(2.40387788045201,4.272660844218,37.6740462830438));
#46367=CARTESIAN_POINT('Ctrl Pts',(0.0675105955612736,4.90200998298708,
37.7534181730972));
#46368=CARTESIAN_POINT('Ctrl Pts',(-2.28530212097756,4.33724034032229,37.8327900631506));
#46369=CARTESIAN_POINT('Ctrl Pts',(-4.08142029927378,2.71592855106086,37.9121619532041));
#46370=CARTESIAN_POINT('Ctrl Pts',(-4.883313526743,0.433022578390986,37.9915338432574));
#46371=CARTESIAN_POINT('Ctrl Pts',(-4.49564238811839,-1.95536673594121,
38.0709057333108));
#46372=CARTESIAN_POINT('Ctrl Pts',(-3.01284271470332,-3.86743304144309,
38.1502776233642));
#46373=CARTESIAN_POINT('Ctrl Pts',(-0.796121224763853,-4.8374012186294,
38.2296495134176));
#46374=CARTESIAN_POINT('Ctrl Pts',(1.61453363327388,-4.62898916605744,38.309021403471));
#46375=CARTESIAN_POINT('Ctrl Pts',(3.63189167208741,-3.29296559930574,38.3883932935244));
#46376=CARTESIAN_POINT('Ctrl Pts',(4.76452893838759,-1.15478290032729,38.4677651835778));
#46377=CARTESIAN_POINT('Ctrl Pts',(4.73653750187218,1.26470235504111,38.5471370736312));
#46378=CARTESIAN_POINT('Ctrl Pts',(3.55473601316178,3.37610891998471,38.6265089636846));
#46379=CARTESIAN_POINT('Ctrl Pts',(1.50700870159436,4.66510281756139,38.705880853738));
#46380=CARTESIAN_POINT('Ctrl Pts',(-0.907822597135966,4.81768800868639,
38.7852527437914));
#46381=CARTESIAN_POINT('Ctrl Pts',(-3.10151031466514,3.79669503846564,38.8646246338448));
#46382=CARTESIAN_POINT('Ctrl Pts',(-4.53967699589137,1.85083561019,38.9439965238982));
#46383=CARTESIAN_POINT('Ctrl Pts',(-4.87198838803768,-0.545883369388725,
39.0233684139517));
#46384=CARTESIAN_POINT('Ctrl Pts',(-4.01749423301241,-2.80962619208844,
39.102740304005));
#46385=CARTESIAN_POINT('Ctrl Pts',(-2.18434729950916,-4.38895062645438,
39.1821121940585));
#46386=CARTESIAN_POINT('Ctrl Pts',(0.180901657890313,-4.89913577411435,
39.2614840841118));
#46387=CARTESIAN_POINT('Ctrl Pts',(2.50208364241399,-4.21590347870473,39.3408559741653));
#46388=CARTESIAN_POINT('Ctrl Pts',(4.21376307902776,-2.50568418547649,39.4202278642187));
#46389=CARTESIAN_POINT('Ctrl Pts',(4.89898012125377,-0.185090004541199,
39.4995997542721));
#46390=CARTESIAN_POINT('Ctrl Pts',(4.39081462818005,2.18059968579169,39.5789716443255));
#46391=CARTESIAN_POINT('Ctrl Pts',(2.81305984991034,4.01508502497055,39.6583435343788));
#46392=CARTESIAN_POINT('Ctrl Pts',(0.55004342451412,4.87153304143481,39.7377154244323));
#46393=CARTESIAN_POINT('Ctrl Pts',(-1.84695009786503,4.54123256689917,39.8170873144857));
#46394=CARTESIAN_POINT('Ctrl Pts',(-3.79405383067523,3.10479958283119,39.8964592045391));
#46395=CARTESIAN_POINT('Ctrl Pts',(-4.8168906266497,0.911851793294956,39.9758310945925));
#46396=CARTESIAN_POINT('Ctrl Pts',(-4.66642692152748,-1.50285363850387,
40.0552029846459));
#46397=CARTESIAN_POINT('Ctrl Pts',(-3.37906911267765,-3.55219315325672,
40.1345748746994));
#46398=CARTESIAN_POINT('Ctrl Pts',(-1.9723130827443,-4.34047654372169,40.1874894680682));
#46399=CARTESIAN_POINT('Ctrl Pts',(-1.21713437249821,-4.54280821229862,
40.2139467647527));
#46400=CARTESIAN_POINT('Ctrl Pts',(-3.71544298812222,3.17665283523783,-0.213946764752703));
#46401=CARTESIAN_POINT('Ctrl Pts',(-4.2435173595033,2.55901209131059,-0.187489468068236));
#46402=CARTESIAN_POINT('Ctrl Pts',(-4.98521092249169,1.05595859527115,-0.1345748746993));
#46403=CARTESIAN_POINT('Ctrl Pts',(-4.8827252805975,-1.45743906270739,-0.0552029846458962));
#46404=CARTESIAN_POINT('Ctrl Pts',(-3.59110607910258,-3.61508997874938,
0.0241689054075074));
#46405=CARTESIAN_POINT('Ctrl Pts',(-1.42455668503541,-4.89247688957836,
0.103540795460911));
#46406=CARTESIAN_POINT('Ctrl Pts',(1.08893586889099,-4.9778765288597,0.182912685514315));
#46407=CARTESIAN_POINT('Ctrl Pts',(3.33720602914152,-3.85077723115681,0.262284575567719));
#46408=CARTESIAN_POINT('Ctrl Pts',(4.77251903131815,-1.78558378675016,0.341656465621122));
#46409=CARTESIAN_POINT('Ctrl Pts',(5.04526816392178,0.714545672093079,0.421028355674526));
#46410=CARTESIAN_POINT('Ctrl Pts',(4.0889952065405,3.04062834435892,0.500400245727928));
#46411=CARTESIAN_POINT('Ctrl Pts',(2.13665520967362,4.62601276074604,0.579772135781332));
#46412=CARTESIAN_POINT('Ctrl Pts',(-0.336170930871067,5.08451490337719,
0.659144025834737));
#46413=CARTESIAN_POINT('Ctrl Pts',(-2.72710569549275,4.30443824810499,0.738515915888139));
#46414=CARTESIAN_POINT('Ctrl Pts',(-4.45372401575963,2.47581113999331,0.817887805941545));
#46415=CARTESIAN_POINT('Ctrl Pts',(-5.09542477676098,0.0440812951164733,
0.897259695994947));
#46416=CARTESIAN_POINT('Ctrl Pts',(-4.49589147158092,-2.39838632564101,
0.976631586048351));
#46417=CARTESIAN_POINT('Ctrl Pts',(-2.80116888608231,-4.25661252099957,
1.05600347610176));
#46418=CARTESIAN_POINT('Ctrl Pts',(-0.424087796932823,-5.07793723552562,
1.13537536615516));
#46419=CARTESIAN_POINT('Ctrl Pts',(2.05630016029234,-4.66228772832596,1.21474725620856));
#46420=CARTESIAN_POINT('Ctrl Pts',(4.03577793971522,-3.11091522434116,1.29411914626197));
#46421=CARTESIAN_POINT('Ctrl Pts',(5.03214915152042,-0.801730671351417,
1.37349103631537));
#46422=CARTESIAN_POINT('Ctrl Pts',(4.80269996559999,1.70275370586111,1.45286292636877));
#46423=CARTESIAN_POINT('Ctrl Pts',(3.40332370018522,3.79245104545052,1.53223481642218));
#46424=CARTESIAN_POINT('Ctrl Pts',(1.17490531372441,4.95831570685873,1.61160670647558));
#46425=CARTESIAN_POINT('Ctrl Pts',(-1.33971740612181,4.9163456360401,1.69097859652898));
#46426=CARTESIAN_POINT('Ctrl Pts',(-3.52798793147818,3.67676465100145,1.77035048658239));
#46427=CARTESIAN_POINT('Ctrl Pts',(-4.85684840567494,1.54153193505596,1.84972237663579));
#46428=CARTESIAN_POINT('Ctrl Pts',(-5.00259135876462,-0.969214547985408,
1.9290942666892));
#46429=CARTESIAN_POINT('Ctrl Pts',(-3.92971412987363,-3.24386251254264,
2.0084661567426));
#46430=CARTESIAN_POINT('Ctrl Pts',(-1.89956723723801,-4.72831274916731,
2.087838046796));
#46431=CARTESIAN_POINT('Ctrl Pts',(0.593310029777512,-5.06095646606144,
2.16720993684941));
#46432=CARTESIAN_POINT('Ctrl Pts',(2.94165828680369,-4.16076239004749,2.24658182690281));
#46433=CARTESIAN_POINT('Ctrl Pts',(4.57342509641733,-2.24701580551599,2.32595371695621));
#46434=CARTESIAN_POINT('Ctrl Pts',(5.09111567564703,0.214098855557618,2.40532560700962));
#46435=CARTESIAN_POINT('Ctrl Pts',(4.36862174528326,2.62305950931529,2.48469749706302));
#46436=CARTESIAN_POINT('Ctrl Pts',(2.58194122754832,4.39304867264849,2.56406938711643));
#46437=CARTESIAN_POINT('Ctrl Pts',(0.166305541812792,5.09290090317231,2.64344127716983));
#46438=CARTESIAN_POINT('Ctrl Pts',(-2.28984180579737,4.55213374662856,2.72281316722323));
#46439=CARTESIAN_POINT('Ctrl Pts',(-4.18818875799412,2.90247688538309,2.80218505727664));
#46440=CARTESIAN_POINT('Ctrl Pts',(-5.06630219914209,0.545783079381991,
2.88155694733003));
#46441=CARTESIAN_POINT('Ctrl Pts',(-4.71027563864874,-1.94386227668626,
2.96092883738345));
#46442=CARTESIAN_POINT('Ctrl Pts',(-3.20683635859883,-3.95998708481986,
3.04030072743684));
#46443=CARTESIAN_POINT('Ctrl Pts',(-0.922218839806132,-5.01146780437411,
3.11967261749025));
#46444=CARTESIAN_POINT('Ctrl Pts',(1.58704914706656,-4.84216605947864,3.19904450754365));
#46445=CARTESIAN_POINT('Ctrl Pts',(3.70971547458753,-3.49332338044696,3.27841639759706));
#46446=CARTESIAN_POINT('Ctrl Pts',(4.92870332381492,-1.29351485827855,3.35778828765046));
#46447=CARTESIAN_POINT('Ctrl Pts',(4.94706995286075,1.22139102021994,3.43716017770387));
#46448=CARTESIAN_POINT('Ctrl Pts',(3.76034129154331,3.43876874969603,3.51653206775727));
#46449=CARTESIAN_POINT('Ctrl Pts',(1.65760181498019,4.81847002333168,3.59590395781068));
#46450=CARTESIAN_POINT('Ctrl Pts',(-0.848925794672718,5.02440266478622,
3.67527584786407));
#46451=CARTESIAN_POINT('Ctrl Pts',(-3.14865695980872,4.00640193842551,3.75464773791748));
#46452=CARTESIAN_POINT('Ctrl Pts',(-4.68138225896931,2.01245056788461,3.83401962797088));
#46453=CARTESIAN_POINT('Ctrl Pts',(-5.07373320190881,-0.471729306509208,
3.91339151802429));
#46454=CARTESIAN_POINT('Ctrl Pts',(-4.23013396738131,-2.84099696599249,
3.99276340807769));
#46455=CARTESIAN_POINT('Ctrl Pts',(-2.3560834616424,-4.51820405300012,4.0721352981311));
#46456=CARTESIAN_POINT('Ctrl Pts',(0.0919037602502722,-5.09478663357196,
4.1515071881845));
#46457=CARTESIAN_POINT('Ctrl Pts',(2.51750342957152,-4.43029046732459,4.2308790782379));
#46458=CARTESIAN_POINT('Ctrl Pts',(4.32984483584847,-2.6865853495186,4.3102509682913));
#46459=CARTESIAN_POINT('Ctrl Pts',(5.08744562406172,-0.288433987225658,
4.38962285834471));
#46460=CARTESIAN_POINT('Ctrl Pts',(4.60575591912341,2.17997925591765,4.46899474839811));
#46461=CARTESIAN_POINT('Ctrl Pts',(3.00211426695445,4.11735437762165,4.54836663845152));
#46462=CARTESIAN_POINT('Ctrl Pts',(0.667164224422586,5.05175108654635,4.62773852850492));
#46463=CARTESIAN_POINT('Ctrl Pts',(-1.83030554643563,4.75555241264972,4.70711041855833));
#46464=CARTESIAN_POINT('Ctrl Pts',(-3.88191693749475,3.30091169726834,4.78648230861172));
#46465=CARTESIAN_POINT('Ctrl Pts',(-4.98790195505755,1.04217619887652,4.86585419866514));
#46466=CARTESIAN_POINT('Ctrl Pts',(-4.87884509690204,-1.47043111474375,
4.94522608871853));
#46467=CARTESIAN_POINT('Ctrl Pts',(-3.58131237228163,-3.62484466355651,
5.02459797877194));
#46468=CARTESIAN_POINT('Ctrl Pts',(-1.4113798808739,-4.89625407578446,5.10396986882534));
#46469=CARTESIAN_POINT('Ctrl Pts',(1.10236162547835,-4.97494683282589,5.18334175887874));
#46470=CARTESIAN_POINT('Ctrl Pts',(3.34757027990012,-3.84175355324895,5.26271364893216));
#46471=CARTESIAN_POINT('Ctrl Pts',(4.77731822385938,-1.77271761167783,5.34208553898555));
#46472=CARTESIAN_POINT('Ctrl Pts',(5.04332202290099,0.728148416254135,5.42145742903896));
#46473=CARTESIAN_POINT('Ctrl Pts',(4.0807837403679,3.05163910171577,5.50082931909235));
#46474=CARTESIAN_POINT('Ctrl Pts',(2.12417557134277,4.63175725668802,5.58020120914577));
#46475=CARTESIAN_POINT('Ctrl Pts',(-0.349877065078572,5.08358959615188,
5.65957309919917));
#46476=CARTESIAN_POINT('Ctrl Pts',(-2.73870042288654,4.29707076232783,5.73894498925257));
#46477=CARTESIAN_POINT('Ctrl Pts',(-4.46038241968988,2.46379500220554,5.81831687930597));
#46478=CARTESIAN_POINT('Ctrl Pts',(-5.09552513194581,0.0303442330637155,
5.89768876935938));
#46479=CARTESIAN_POINT('Ctrl Pts',(-4.48940920081331,-2.41049832408661,
5.97706065941278));
#46480=CARTESIAN_POINT('Ctrl Pts',(-2.78968312550141,-4.26414882503699,
6.05643254946618));
#46481=CARTESIAN_POINT('Ctrl Pts',(-0.410396415676208,-5.07906211074168,
6.13580443951959));
#46482=CARTESIAN_POINT('Ctrl Pts',(2.06886195261065,-4.65672710858298,6.21517632957299));
#46483=CARTESIAN_POINT('Ctrl Pts',(4.04415012858982,-3.10002369026409,6.2945482196264));
#46484=CARTESIAN_POINT('Ctrl Pts',(5.03429228481897,-0.788161362782912,
6.37392010967979));
#46485=CARTESIAN_POINT('Ctrl Pts',(4.79809198368318,1.7156953281066,6.45329199973321));
#46486=CARTESIAN_POINT('Ctrl Pts',(3.39308709571864,3.80161243469653,6.5326638897866));
#46487=CARTESIAN_POINT('Ctrl Pts',(1.16153370170793,4.96146516692078,6.61203577984001));
#46488=CARTESIAN_POINT('Ctrl Pts',(-1.35296673102758,4.91271596650001,6.69140766989341));
#46489=CARTESIAN_POINT('Ctrl Pts',(-3.53788746282585,3.66724003075218,6.77077955994682));
#46490=CARTESIAN_POINT('Ctrl Pts',(-4.8609866396608,1.52843254081124,6.85015145000022));
#46491=CARTESIAN_POINT('Ctrl Pts',(-4.99996023068582,-0.982697732943262,
6.92952334005363));
#46492=CARTESIAN_POINT('Ctrl Pts',(-3.92095457674001,-3.25444501411732,
7.00889523010702));
#46493=CARTESIAN_POINT('Ctrl Pts',(-1.8868130667861,-4.73341669344426,7.08826712016043));
#46494=CARTESIAN_POINT('Ctrl Pts',(0.606951929847044,-5.05933854348832,
7.16763901021384));
#46495=CARTESIAN_POINT('Ctrl Pts',(2.95286477983474,-4.15281672299454,7.24701090026724));
#46496=CARTESIAN_POINT('Ctrl Pts',(4.57946630551004,-2.23467794088318,7.32638279032065));
#46497=CARTESIAN_POINT('Ctrl Pts',(5.0905199756398,0.227823441251604,7.40575468037404));
#46498=CARTESIAN_POINT('Ctrl Pts',(4.36153424737857,2.63482753737611,7.48512657042746));
#46499=CARTESIAN_POINT('Ctrl Pts',(2.57008843054822,4.39999347748764,7.56449846048085));
#46500=CARTESIAN_POINT('Ctrl Pts',(0.152574760830579,5.09333074570355,7.64387035053426));
#46501=CARTESIAN_POINT('Ctrl Pts',(-2.3021057829069,4.54594391816246,7.72324224058766));
#46502=CARTESIAN_POINT('Ctrl Pts',(-4.19599845355297,2.89117521443317,7.80261413064106));
#46503=CARTESIAN_POINT('Ctrl Pts',(-5.06775518859857,0.532122627975753,
7.88198602069447));
#46504=CARTESIAN_POINT('Ctrl Pts',(-4.70501797698741,-1.95655385282311,
7.96135791074787));
#46505=CARTESIAN_POINT('Ctrl Pts',(-3.19614880056275,-3.96861814583273,
8.04072980080128));
#46506=CARTESIAN_POINT('Ctrl Pts',(-0.908704850876407,-5.01393584290478,
8.12010169085468));
#46507=CARTESIAN_POINT('Ctrl Pts',(1.60009758909935,-4.83786986680398,8.19947358090808));
#46508=CARTESIAN_POINT('Ctrl Pts',(3.71911979812647,-3.48330949959307,8.27884547096148));
#46509=CARTESIAN_POINT('Ctrl Pts',(4.93217265646204,-1.28022264845606,8.3582173610149));
#46510=CARTESIAN_POINT('Ctrl Pts',(4.94375917286243,1.23472360612009,8.43758925106829));
#46511=CARTESIAN_POINT('Ctrl Pts',(3.75105689757885,3.4488939232597,8.5169611411217));
#46512=CARTESIAN_POINT('Ctrl Pts',(1.64460546486869,4.82292131469047,8.5963330311751));
#46513=CARTESIAN_POINT('Ctrl Pts',(-0.862468218811062,5.02209574921791,
8.67570492122851));
#46514=CARTESIAN_POINT('Ctrl Pts',(-3.15944655342946,3.99789877545622,8.75507681128191));
#46515=CARTESIAN_POINT('Ctrl Pts',(-4.68679070094874,1.99982250919225,8.83444870133531));
#46516=CARTESIAN_POINT('Ctrl Pts',(-5.07244300775217,-0.485406093778898,
8.91382059138872));
#46517=CARTESIAN_POINT('Ctrl Pts',(-4.22245942552934,-2.85239084673368,
8.99319248144211));
#46518=CARTESIAN_POINT('Ctrl Pts',(-2.34389407350296,-4.52453950308418,
9.07256437149552));
#46519=CARTESIAN_POINT('Ctrl Pts',(0.105638686707185,-5.09452035138171,
9.15193626154893));
#46520=CARTESIAN_POINT('Ctrl Pts',(2.52943809666274,-4.42348731861218,9.23130815160232));
#46521=CARTESIAN_POINT('Ctrl Pts',(4.33707198508751,-2.67490256625183,9.31068004165574));
#46522=CARTESIAN_POINT('Ctrl Pts',(5.08820473789098,-0.274717469548947,
9.39005193170913));
#46523=CARTESIAN_POINT('Ctrl Pts',(4.59986207909436,2.19238819465928,9.46942382176255));
#46524=CARTESIAN_POINT('Ctrl Pts',(2.99100319945234,4.12543294741746,9.54879571181595));
#46525=CARTESIAN_POINT('Ctrl Pts',(0.653542560897033,5.05353136567566,9.62816760186935));
#46526=CARTESIAN_POINT('Ctrl Pts',(-1.84311959890086,4.75060072905723,9.70753949192275));
#46527=CARTESIAN_POINT('Ctrl Pts',(-3.89080190408257,3.29043427011681,9.78691138197615));
#46528=CARTESIAN_POINT('Ctrl Pts',(-4.99069347757367,1.02872530622863,9.86628327202957));
#46529=CARTESIAN_POINT('Ctrl Pts',(-4.87486316664046,-1.48357886521197,
9.94565516208295));
#46530=CARTESIAN_POINT('Ctrl Pts',(-3.57152697864026,-3.63448650893304,
10.0250270521364));
#46531=CARTESIAN_POINT('Ctrl Pts',(-1.39817472408419,-4.90004128387748,
10.1043989421898));
#46532=CARTESIAN_POINT('Ctrl Pts',(1.11576979845155,-4.9719568481268,10.1837708322432));
#46533=CARTESIAN_POINT('Ctrl Pts',(3.35791526779908,-3.83271472941224,10.2631427222966));
#46534=CARTESIAN_POINT('Ctrl Pts',(4.7820800105301,-1.75983178618299,10.34251461235));
#46535=CARTESIAN_POINT('Ctrl Pts',(5.04134064765054,0.741742284838825,10.4218865024034));
#46536=CARTESIAN_POINT('Ctrl Pts',(4.07254186182158,3.0626295770926,10.5012583924568));
#46537=CARTESIAN_POINT('Ctrl Pts',(2.11168089287137,4.63746708338223,10.5806302825102));
#46538=CARTESIAN_POINT('Ctrl Pts',(-0.363580867455945,5.08262787301918,
10.6600021725636));
#46539=CARTESIAN_POINT('Ctrl Pts',(-2.75027513324356,4.28967176299466,10.739374062617));
#46540=CARTESIAN_POINT('Ctrl Pts',(-4.46700846420381,2.45176110653202,10.8187459526704));
#46541=CARTESIAN_POINT('Ctrl Pts',(-5.09558842083953,0.0166068713993523,
10.8981178427238));
#46542=CARTESIAN_POINT('Ctrl Pts',(-4.48289431705241,-2.42259276084751,
10.9774897327772));
#46543=CARTESIAN_POINT('Ctrl Pts',(-2.77817708034959,-4.27165415887005,
11.0568616228306));
#46544=CARTESIAN_POINT('Ctrl Pts',(-0.396702056264276,-5.08015005893795,
11.136233512884));
#46545=CARTESIAN_POINT('Ctrl Pts',(2.0814087106419,-4.65113264937,11.2156054029374));
#46546=CARTESIAN_POINT('Ctrl Pts',(4.05249292275577,-3.08910962152302,11.2949772929908));
#46547=CARTESIAN_POINT('Ctrl Pts',(5.03639882892726,-0.774586327501172,
11.3743491830442));
#46548=CARTESIAN_POINT('Ctrl Pts',(4.79344912825178,1.7286244813822,11.4537210730976));
#46549=CARTESIAN_POINT('Ctrl Pts',(3.38282583005384,3.81074619284624,11.533092963151));
#46550=CARTESIAN_POINT('Ctrl Pts',(1.14815364741277,4.96457856667656,11.6124648532044));
#46551=CARTESIAN_POINT('Ctrl Pts',(-1.36620622234309,4.90905059057276,11.6918367432579));
#46552=CARTESIAN_POINT('Ctrl Pts',(-3.54776128038234,3.65768875660455,11.7712086333112));
#46553=CARTESIAN_POINT('Ctrl Pts',(-4.86508954335683,1.51532203768426,11.8505805233647));
#46554=CARTESIAN_POINT('Ctrl Pts',(-4.99729276226266,-0.9961737755075,11.9299524134181));
#46555=CARTESIAN_POINT('Ctrl Pts',(-3.91216652560121,-3.26500386197887,
12.0093243034715));
#46556=CARTESIAN_POINT('Ctrl Pts',(-1.87404518273703,-4.73848623463566,
12.0886961935249));
#46557=CARTESIAN_POINT('Ctrl Pts',(0.620589418513222,-5.05768384899659,
12.1680680835782));
#46558=CARTESIAN_POINT('Ctrl Pts',(2.96404981106505,-4.14484087273527,12.2474399736317));
#46559=CARTESIAN_POINT('Ctrl Pts',(4.58547423045439,-2.2223238343253,12.3268118636851));
#46560=CARTESIAN_POINT('Ctrl Pts',(5.08988727708011,0.241546371095948,12.4061837537385));
#46561=CARTESIAN_POINT('Ctrl Pts',(4.3544150492835,2.64657641517207,12.4855556437919));
#46562=CARTESIAN_POINT('Ctrl Pts',(2.55821695381563,4.40690630260979,12.5649275338453));
#46563=CARTESIAN_POINT('Ctrl Pts',(0.138842870915485,5.09372356925339,12.6442994238987));
#46564=CARTESIAN_POINT('Ctrl Pts',(-2.3143530280162,4.53972104919276,12.7236713139521));
#46565=CARTESIAN_POINT('Ctrl Pts',(-4.20377765205669,2.87985253005087,12.8030432040055));
#46566=CARTESIAN_POINT('Ctrl Pts',(-5.06917134496016,0.518458309034014,
12.8824150940589));
#46567=CARTESIAN_POINT('Ctrl Pts',(-4.69972611865178,-1.9692312084755,12.9617869841123));
#46568=CARTESIAN_POINT('Ctrl Pts',(-3.18543801250715,-3.97722036241972,
13.0411588741657));
#46569=CARTESIAN_POINT('Ctrl Pts',(-0.895184257363228,-5.01636743950647,
13.1205307642191));
#46570=CARTESIAN_POINT('Ctrl Pts',(1.61313440141763,-4.83353851187042,13.1999026542725));
#46571=CARTESIAN_POINT('Ctrl Pts',(3.72849709062559,-3.47327030159879,13.2792745443259));
#46572=CARTESIAN_POINT('Ctrl Pts',(4.93560614144549,-1.26692113381109,13.3586464343793));
#46573=CARTESIAN_POINT('Ctrl Pts',(4.94041246098816,1.24804721789062,13.4380183244327));
#46574=CARTESIAN_POINT('Ctrl Pts',(3.74174524045162,3.45899402981983,13.5173902144861));
#46575=CARTESIAN_POINT('Ctrl Pts',(1.63159716155366,4.82733755243838,13.5967621045395));
#46576=CARTESIAN_POINT('Ctrl Pts',(-0.87600437441973,5.01975233241333,13.6761339945929));
#46577=CARTESIAN_POINT('Ctrl Pts',(-3.17021318378723,3.98936655524573,13.7555058846463));
#46578=CARTESIAN_POINT('Ctrl Pts',(-4.69216507873203,1.98717991553337,13.8348777746998));
#46579=CARTESIAN_POINT('Ctrl Pts',(-5.07111594642896,-0.499079353054812,
13.9142496647532));
#46580=CARTESIAN_POINT('Ctrl Pts',(-4.21475419430051,-2.86376399593225,
13.9936215548066));
#46581=CARTESIAN_POINT('Ctrl Pts',(-2.33168764964064,-4.53084206823465,
14.07299344486));
#46582=CARTESIAN_POINT('Ctrl Pts',(0.119372845368581,-5.09421704156391,
14.1523653349133));
#46583=CARTESIAN_POINT('Ctrl Pts',(2.54135437947334,-4.4166520194264,14.2317372249668));
#46584=CARTESIAN_POINT('Ctrl Pts',(4.34426761193091,-2.66320034145004,14.3111091150202));
#46585=CARTESIAN_POINT('Ctrl Pts',(5.08892686999541,-0.260998955190403,
14.3904810050736));
#46586=CARTESIAN_POINT('Ctrl Pts',(4.59393480667753,2.20478119884224,14.469852895127));
#46587=CARTESIAN_POINT('Ctrl Pts',(2.97987039295526,4.13348153303728,14.5492247851804));
#46588=CARTESIAN_POINT('Ctrl Pts',(0.639916147340316,5.05527491509065,14.6285966752338));
#46589=CARTESIAN_POINT('Ctrl Pts',(-1.85592025533638,4.74561451748915,14.7079685652872));
#46590=CARTESIAN_POINT('Ctrl Pts',(-3.89965859182293,3.27993292766684,14.7873404553406));
#46591=CARTESIAN_POINT('Ctrl Pts',(-4.99344872708928,1.01526693667329,14.866712345394));
#46592=CARTESIAN_POINT('Ctrl Pts',(-4.87084580524798,-1.49671583283861,
14.9460842354474));
#46593=CARTESIAN_POINT('Ctrl Pts',(-3.56171562668257,-3.64410193839537,
15.0254561255008));
#46594=CARTESIAN_POINT('Ctrl Pts',(-1.38495940518108,-4.90379287784181,
15.1048280155542));
#46595=CARTESIAN_POINT('Ctrl Pts',(1.12916986186683,-4.9689307266074,15.1841999056076));
#46596=CARTESIAN_POINT('Ctrl Pts',(3.36823584993909,-3.82364804891307,15.263571795661));
#46597=CARTESIAN_POINT('Ctrl Pts',(4.78680704042976,-1.74693317000493,15.3429436857144));
#46598=CARTESIAN_POINT('Ctrl Pts',(5.0393226312895,0.755330762345426,15.4223155757678));
#46599=CARTESIAN_POINT('Ctrl Pts',(4.06427038351844,3.07359779288479,15.5016874658212));
#46600=CARTESIAN_POINT('Ctrl Pts',(2.09917086643239,4.64314320437064,15.5810593558746));
#46601=CARTESIAN_POINT('Ctrl Pts',(-0.377282027281083,5.08162920869508,
15.660431245928));
#46602=CARTESIAN_POINT('Ctrl Pts',(-2.76182985424771,4.28224158577663,15.7398031359814));
#46603=CARTESIAN_POINT('Ctrl Pts',(-4.47360204192776,2.43970939114443,15.8191750260348));
#46604=CARTESIAN_POINT('Ctrl Pts',(-5.09561467434161,0.00286938903366673,
15.8985469160882));
#46605=CARTESIAN_POINT('Ctrl Pts',(-4.47634685104277,-2.43466958989267,
15.9779188061416));
#46606=CARTESIAN_POINT('Ctrl Pts',(-2.76665084304587,-4.27912844577413,
16.0572906961951));
#46607=CARTESIAN_POINT('Ctrl Pts',(-0.383004813579153,-5.08120108394907,
16.1366625862484));
#46608=CARTESIAN_POINT('Ctrl Pts',(2.09394034074345,-4.64550438513334,16.2160344763019));
#46609=CARTESIAN_POINT('Ctrl Pts',(4.06080626285358,-3.07817310072693,16.2954063663552));
#46610=CARTESIAN_POINT('Ctrl Pts',(5.03846876789878,-0.761005662445124,
16.3747782564087));
#46611=CARTESIAN_POINT('Ctrl Pts',(4.7887714333112,1.74154107082836,16.4541501464621));
#46612=CARTESIAN_POINT('Ctrl Pts',(3.37253997777685,3.81985225393751,16.5335220365155));
#46613=CARTESIAN_POINT('Ctrl Pts',(1.13476524781198,4.96765588336339,16.6128939265689));
#46614=CARTESIAN_POINT('Ctrl Pts',(-1.37943578318358,4.90534953479992,16.6922658166222));
#46615=CARTESIAN_POINT('Ctrl Pts',(-3.5576093137008,3.64811089835147,16.7716377066757));
#46616=CARTESIAN_POINT('Ctrl Pts',(-4.86915708441607,1.50220052016076,16.851009596729));
#46617=CARTESIAN_POINT('Ctrl Pts',(-4.99458897767399,-1.00964257616395,
16.9303814867825));
#46618=CARTESIAN_POINT('Ctrl Pts',(-3.90335003127183,-3.2755389823738,17.0097533768359));
#46619=CARTESIAN_POINT('Ctrl Pts',(-1.8612636949986,-4.74352133023597,17.0891252668893));
#46620=CARTESIAN_POINT('Ctrl Pts',(0.634222428965914,-5.05599240530682,
17.1684971569427));
#46621=CARTESIAN_POINT('Ctrl Pts',(2.9752132381933,-4.13683487704247,17.2478690469961));
#46622=CARTESIAN_POINT('Ctrl Pts',(4.59144894277892,-2.20995361377096,17.3272409370495));
#46623=CARTESIAN_POINT('Ctrl Pts',(5.08921736705481,0.255267617363485,17.4066128271029));
#46624=CARTESIAN_POINT('Ctrl Pts',(4.34726461344772,2.65830592133578,17.4859847171563));
#46625=CARTESIAN_POINT('Ctrl Pts',(2.54632610813648,4.41378735452059,17.5653566072097));
#46626=CARTESIAN_POINT('Ctrl Pts',(0.125111436169681,5.09407888617233,17.6447284972631));
#46627=CARTESIAN_POINT('Ctrl Pts',(-2.32658621700147,4.53346610033861,17.7241003873165));
#46628=CARTESIAN_POINT('Ctrl Pts',(-4.21152107628919,2.8685071860873,17.8034722773699));
#46629=CARTESIAN_POINT('Ctrl Pts',(-5.07056051563183,0.504793485523745,
17.8828441674233));
#46630=CARTESIAN_POINT('Ctrl Pts',(-4.69438148876582,-1.98190041394314,
17.9622160574767));
#46631=CARTESIAN_POINT('Ctrl Pts',(-3.1747392180444,-3.9857820361196,18.0415879475301));
#46632=CARTESIAN_POINT('Ctrl Pts',(-0.881590795203727,-5.01878454751455,
18.1209598375835));
#46633=CARTESIAN_POINT('Ctrl Pts',(1.62603418385021,-4.82913054051801,18.2003317276369));
#46634=CARTESIAN_POINT('Ctrl Pts',(3.73808388472066,-3.46328419200805,18.2797036176903));
#46635=CARTESIAN_POINT('Ctrl Pts',(4.93855701420293,-1.25346250930793,18.3590755077438));
#46636=CARTESIAN_POINT('Ctrl Pts',(4.93787328845974,1.26108254025623,18.4384473977971));
#46637=CARTESIAN_POINT('Ctrl Pts',(3.73081451079157,3.46959580775143,18.5178192878506));
#46638=CARTESIAN_POINT('Ctrl Pts',(1.62157688245111,4.83072732396141,18.597191177904));
#46639=CARTESIAN_POINT('Ctrl Pts',(-0.895150293053049,5.01921699961797,
18.6765630679574));
#46640=CARTESIAN_POINT('Ctrl Pts',(-3.17074515011531,3.97754537770249,18.7559349580108));
#46641=CARTESIAN_POINT('Ctrl Pts',(-5.22808970274021,1.31272284990122,18.8617641447486));
#46642=CARTESIAN_POINT('Ctrl Pts',(-4.77339715849023,-3.25411141853201,
18.994050628171));
#46643=CARTESIAN_POINT('Ctrl Pts',(0.152720854580862,-5.77834717219764,
19.1527944082778));
#46644=CARTESIAN_POINT('Ctrl Pts',(4.93271294602037,-3.00474199436408,19.3115381883846));
#46645=CARTESIAN_POINT('Ctrl Pts',(5.20235975367847,2.51303602329821,19.4702819684914));
#46646=CARTESIAN_POINT('Ctrl Pts',(0.709818611660393,5.73400533709388,19.6290257485982));
#46647=CARTESIAN_POINT('Ctrl Pts',(-4.43131449514935,3.70671199728522,19.787769528705));
#46648=CARTESIAN_POINT('Ctrl Pts',(-5.51805139390214,-1.71188403765749,
19.9465133088118));
#46649=CARTESIAN_POINT('Ctrl Pts',(-1.55524717023727,-5.56394358573197,
20.1052570889187));
#46650=CARTESIAN_POINT('Ctrl Pts',(3.83058845612614,-4.32541925679744,20.2640008690254));
#46651=CARTESIAN_POINT('Ctrl Pts',(5.71123844601177,0.87272703286029,20.4227446491323));
#46652=CARTESIAN_POINT('Ctrl Pts',(2.36591519662234,5.26902047281308,20.581488429239));
#46653=CARTESIAN_POINT('Ctrl Pts',(-3.14459942082001,4.85016640791291,20.7402322093459));
#46654=CARTESIAN_POINT('Ctrl Pts',(-5.77704085522352,-0.0189872057270379,
20.8989759894526));
#46655=CARTESIAN_POINT('Ctrl Pts',(-3.56709774791074,-4.0412840629435,21.031262472875));
#46656=CARTESIAN_POINT('Ctrl Pts',(-0.362731338653644,-5.07374792580599,
21.1370916596129));
#46657=CARTESIAN_POINT('Ctrl Pts',(2.10287077052077,-4.64454172754387,21.2164635496663));
#46658=CARTESIAN_POINT('Ctrl Pts',(4.07100210770441,-3.06469899064061,21.2958354397197));
#46659=CARTESIAN_POINT('Ctrl Pts',(5.03948789886561,-0.748754766453301,
21.3752073297731));
#46660=CARTESIAN_POINT('Ctrl Pts',(4.78459624359497,1.75515257798294,21.4545792198265));
#46661=CARTESIAN_POINT('Ctrl Pts',(3.36194502775863,3.82855576883798,21.5339511098799));
#46662=CARTESIAN_POINT('Ctrl Pts',(1.12151932172619,4.97089558679479,21.6133229999333));
#46663=CARTESIAN_POINT('Ctrl Pts',(-1.39273514199732,4.9015077036213,21.6926948899867));
#46664=CARTESIAN_POINT('Ctrl Pts',(-3.56738921282951,3.63856219800436,21.7720667800401));
#46665=CARTESIAN_POINT('Ctrl Pts',(-4.87321162956223,1.48903860109202,21.8514386700935));
#46666=CARTESIAN_POINT('Ctrl Pts',(-4.99183702504821,-1.02308842639,21.9308105601469));
#46667=CARTESIAN_POINT('Ctrl Pts',(-3.89451146459856,-3.28605855970678,
22.0101824502003));
#46668=CARTESIAN_POINT('Ctrl Pts',(-1.84846531944319,-4.74851758083281,
22.0895543402537));
#46669=CARTESIAN_POINT('Ctrl Pts',(0.647849003889951,-5.05426651218743,
22.1689262303072));
#46670=CARTESIAN_POINT('Ctrl Pts',(2.98635609589609,-4.12879762624803,22.2482981203605));
#46671=CARTESIAN_POINT('Ctrl Pts',(4.59738955946421,-2.19756790530644,22.3276700104139));
#46672=CARTESIAN_POINT('Ctrl Pts',(5.08851116459638,0.268987208844064,22.4070419004674));
#46673=CARTESIAN_POINT('Ctrl Pts',(4.34008162116472,2.67001619606227,22.4864137905207));
#46674=CARTESIAN_POINT('Ctrl Pts',(2.53441837980377,4.4206359096037,22.5657856805742));
#46675=CARTESIAN_POINT('Ctrl Pts',(0.11137612465092,5.09439809707615,22.6451575706275));
#46676=CARTESIAN_POINT('Ctrl Pts',(-2.3387969457162,4.52717639800266,22.724529460681));
#46677=CARTESIAN_POINT('Ctrl Pts',(-4.2192443428605,2.85714443596456,22.8039013507343));
#46678=CARTESIAN_POINT('Ctrl Pts',(-5.07189311172227,0.491118473430054,
22.8832732407878));
#46679=CARTESIAN_POINT('Ctrl Pts',(-4.6890399691108,-1.99454289389497,22.9626451308412));
#46680=CARTESIAN_POINT('Ctrl Pts',(-3.1639470562758,-3.99433801030587,23.0420170208946));
#46681=CARTESIAN_POINT('Ctrl Pts',(-0.868123650568842,-5.02112123762457,
23.121388910948));
#46682=CARTESIAN_POINT('Ctrl Pts',(1.63917275843702,-4.82477044080721,23.2007608010014));
#46683=CARTESIAN_POINT('Ctrl Pts',(3.74717030983928,-3.45311624655406,23.2801326910548));
#46684=CARTESIAN_POINT('Ctrl Pts',(4.94236546898948,-1.24029057666132,23.3595045811082));
#46685=CARTESIAN_POINT('Ctrl Pts',(4.93361133910258,1.27466713166923,23.4388764711616));
#46686=CARTESIAN_POINT('Ctrl Pts',(3.72304040765536,3.47911874852391,23.518248361215));
#46687=CARTESIAN_POINT('Ctrl Pts',(1.60554507356429,4.83606473894047,23.5976202512684));
#46688=CARTESIAN_POINT('Ctrl Pts',(-0.903057486554317,5.01495606350285,
23.6769921413218));
#46689=CARTESIAN_POINT('Ctrl Pts',(-3.19167724187396,3.97221519135782,23.7563640313752));
#46690=CARTESIAN_POINT('Ctrl Pts',(-4.70281148570869,1.96185149097637,23.8357359214286));
#46691=CARTESIAN_POINT('Ctrl Pts',(-5.06835126113314,-0.526414890137771,
23.915107811482));
#46692=CARTESIAN_POINT('Ctrl Pts',(-4.1992518879446,-2.88644776920571,23.9944797015354));
#46693=CARTESIAN_POINT('Ctrl Pts',(-2.30722404974247,-4.54334836074326,
24.0738515915888));
#46694=CARTESIAN_POINT('Ctrl Pts',(0.1468384600249,-5.09349934813251,24.1532234816422));
#46695=CARTESIAN_POINT('Ctrl Pts',(2.56513144595071,-4.40288516858744,24.2325953716957));
#46696=CARTESIAN_POINT('Ctrl Pts',(4.35856408946553,-2.63973790759483,24.311967261749));
#46697=CARTESIAN_POINT('Ctrl Pts',(5.09026016830426,-0.23355633527326,24.3913391518024));
#46698=CARTESIAN_POINT('Ctrl Pts',(4.58198013724401,2.22951904335289,24.4707110418559));
#46699=CARTESIAN_POINT('Ctrl Pts',(2.95753988679205,4.1494885179749,24.5500829319092));
#46700=CARTESIAN_POINT('Ctrl Pts',(0.612649466321058,5.05865177435533,24.6294548219626));
#46701=CARTESIAN_POINT('Ctrl Pts',(-1.88148100806917,4.73553865563851,24.7088267120161));
#46702=CARTESIAN_POINT('Ctrl Pts',(-3.91728687348126,3.25885880234522,24.7881986020694));
#46703=CARTESIAN_POINT('Ctrl Pts',(-4.99885032728078,0.988328158162253,
24.8675704921229));
#46704=CARTESIAN_POINT('Ctrl Pts',(-4.86270490612224,-1.5229570377218,24.9469423821763));
#46705=CARTESIAN_POINT('Ctrl Pts',(-3.54201533324704,-3.66325327022505,
25.0263142722297));
#46706=CARTESIAN_POINT('Ctrl Pts',(-1.3584986653108,-4.91118911457504,25.1056861622831));
#46707=CARTESIAN_POINT('Ctrl Pts',(1.15594527050936,-4.96277016134726,25.1850580523365));
#46708=CARTESIAN_POINT('Ctrl Pts',(3.38880349707489,-3.80543138172069,25.2644299423899));
#46709=CARTESIAN_POINT('Ctrl Pts',(4.79615669274227,-1.72109794068643,25.3438018324433));
#46710=CARTESIAN_POINT('Ctrl Pts',(5.0351767341704,0.782491149113306,25.4231737224967));
#46711=CARTESIAN_POINT('Ctrl Pts',(4.04763886832931,3.09546712700384,25.5025456125501));
#46712=CARTESIAN_POINT('Ctrl Pts',(2.07410513345989,4.65439416445651,25.5819175026035));
#46713=CARTESIAN_POINT('Ctrl Pts',(-0.404676020966502,5.07952108577436,
25.6612893926569));
#46714=CARTESIAN_POINT('Ctrl Pts',(-2.78487899242069,4.26728791392678,25.7406612827102));
#46715=CARTESIAN_POINT('Ctrl Pts',(-4.48669160554627,2.41555285172821,25.8200331727637));
#46716=CARTESIAN_POINT('Ctrl Pts',(-5.09555607468418,-0.0246055384158182,
25.8994050628171));
#46717=CARTESIAN_POINT('Ctrl Pts',(-4.46315436285108,-2.45877007386518,
25.9787769528705));
#46718=CARTESIAN_POINT('Ctrl Pts',(-2.74353812725205,-4.29398366171623,
26.0581488429239));
#46719=CARTESIAN_POINT('Ctrl Pts',(-0.355602076573053,-5.0831923341448,
26.1375207329773));
#46720=CARTESIAN_POINT('Ctrl Pts',(2.11895785284724,-4.63414660543109,26.2168926230307));
#46721=CARTESIAN_POINT('Ctrl Pts',(4.07734433954763,-3.05623302114393,26.2962645130841));
#46722=CARTESIAN_POINT('Ctrl Pts',(5.04249877018284,-0.733827837763115,
26.3756364031375));
#46723=CARTESIAN_POINT('Ctrl Pts',(4.77931166178323,1.76733618259643,26.4550082931909));
#46724=CARTESIAN_POINT('Ctrl Pts',(3.3518948114001,3.83798102080776,26.5343801832444));
#46725=CARTESIAN_POINT('Ctrl Pts',(1.10796380425329,4.97370217757719,26.6137520732977));
#46726=CARTESIAN_POINT('Ctrl Pts',(-1.40586473317334,4.89784049299189,26.6931239633511));
#46727=CARTESIAN_POINT('Ctrl Pts',(-3.57722773342779,3.62887570549981,26.7724958534045));
#46728=CARTESIAN_POINT('Ctrl Pts',(-4.87718597587851,1.47592482852807,26.851867743458));
#46729=CARTESIAN_POINT('Ctrl Pts',(-4.98907251007324,-1.0365580697689,26.9312396335114));
#46730=CARTESIAN_POINT('Ctrl Pts',(-3.88563202393884,-3.29653771665249,
27.0106115235647));
#46731=CARTESIAN_POINT('Ctrl Pts',(-1.83566017747357,-4.75348807252204,
27.0899834136182));
#46732=CARTESIAN_POINT('Ctrl Pts',(0.661474425059423,-5.05249925559262,
27.1693553036715));
#46733=CARTESIAN_POINT('Ctrl Pts',(2.99747532179674,-4.12073280351822,27.248727193725));
#46734=CARTESIAN_POINT('Ctrl Pts',(4.60329786494346,-2.18516496159412,27.3280990837784));
#46735=CARTESIAN_POINT('Ctrl Pts',(5.08776723741692,0.282704228193704,27.4074709738318));
#46736=CARTESIAN_POINT('Ctrl Pts',(4.33286777243738,2.68170729374875,27.4868428638852));
#46737=CARTESIAN_POINT('Ctrl Pts',(2.5224913087322,4.42745239840498,27.5662147539386));
#46738=CARTESIAN_POINT('Ctrl Pts',(0.0976415456597213,5.09467989880942,
27.6455866439919));
#46739=CARTESIAN_POINT('Ctrl Pts',(-2.35099348180958,4.52085465274658,27.7249585340454));
#46740=CARTESIAN_POINT('Ctrl Pts',(-4.22693170094588,2.84575922001675,27.8043304240988));
#46741=CARTESIAN_POINT('Ctrl Pts',(-5.07319871388641,0.477443140272041,
27.8837023141522));
#46742=CARTESIAN_POINT('Ctrl Pts',(-4.68364574945911,-2.00717703164051,
27.9630742042056));
#46743=CARTESIAN_POINT('Ctrl Pts',(-3.15316704753758,-4.00285332145644,
28.042446094259));
#46744=CARTESIAN_POINT('Ctrl Pts',(-0.854583832252744,-5.02344340233109,
28.1218179843124));
#46745=CARTESIAN_POINT('Ctrl Pts',(1.65217411297962,-4.82033378960126,28.2011898743658));
#46746=CARTESIAN_POINT('Ctrl Pts',(3.75646610131553,-3.44300153535241,28.2805617644192));
#46747=CARTESIAN_POINT('Ctrl Pts',(4.94569126216762,-1.22696172804632,28.3599336544726));
#46748=CARTESIAN_POINT('Ctrl Pts',(4.93015697865761,1.28796324037807,28.439305544526));
#46749=CARTESIAN_POINT('Ctrl Pts',(3.71364736786401,3.48914321430466,28.5186774345794));
#46750=CARTESIAN_POINT('Ctrl Pts',(1.59250147827778,4.84037562431415,28.5980493246328));
#46751=CARTESIAN_POINT('Ctrl Pts',(-0.916574246474672,5.01250324623047,
28.6774212146862));
#46752=CARTESIAN_POINT('Ctrl Pts',(-3.20237451358863,3.96359617235279,28.7567931047396));
#46753=CARTESIAN_POINT('Ctrl Pts',(-4.70808343752814,1.94916584416126,28.836164994793));
#46754=CARTESIAN_POINT('Ctrl Pts',(-5.0669136572517,-0.540076969262536,
28.9155368848465));
#46755=CARTESIAN_POINT('Ctrl Pts',(-4.19145492549188,-2.89775822841407,
28.9949087748998));
#46756=CARTESIAN_POINT('Ctrl Pts',(-2.29496705151034,-4.54955199720298,
29.0742806649532));
#46757=CARTESIAN_POINT('Ctrl Pts',(0.160569716395729,-5.09308496973575,
29.1536525550067));
#46758=CARTESIAN_POINT('Ctrl Pts',(2.57699205680278,-4.39595371699326,29.23302444506));
#46759=CARTESIAN_POINT('Ctrl Pts',(4.36566483624787,-2.62797786906977,29.3123963351135));
#46760=CARTESIAN_POINT('Ctrl Pts',(5.09087132481821,-0.219832429171176,
29.3917682251668));
#46761=CARTESIAN_POINT('Ctrl Pts',(4.57595282711536,2.24186370388268,29.4711401152203));
#46762=CARTESIAN_POINT('Ctrl Pts',(2.94634234942697,4.15744680095185,29.5505120052737));
#46763=CARTESIAN_POINT('Ctrl Pts',(0.599009397036387,5.06028505966152,29.6298838953271));
#46764=CARTESIAN_POINT('Ctrl Pts',(-1.89424091858745,4.73044907858869,29.7092557853805));
#46765=CARTESIAN_POINT('Ctrl Pts',(-3.92605833927458,3.24828617264307,29.7886276754339));
#46766=CARTESIAN_POINT('Ctrl Pts',(-5.00149663869715,0.974847945001076,
29.8679995654873));
#46767=CARTESIAN_POINT('Ctrl Pts',(-4.85858142755809,-1.53606108425386,
29.9473714555407));
#46768=CARTESIAN_POINT('Ctrl Pts',(-3.53212653495348,-3.67278903339805,
30.026743345594));
#46769=CARTESIAN_POINT('Ctrl Pts',(-1.34525343666372,-4.91483370358714,
30.1061152356475));
#46770=CARTESIAN_POINT('Ctrl Pts',(1.16932042112941,-4.95963576238229,30.1854871257009));
#46771=CARTESIAN_POINT('Ctrl Pts',(3.39905041258226,-3.79628152742866,30.2648590157543));
#46772=CARTESIAN_POINT('Ctrl Pts',(4.80077924720052,-1.70816151532001,30.3442309058077));
#46773=CARTESIAN_POINT('Ctrl Pts',(5.03304888354535,0.796062860969203,30.4236027958611));
#46774=CARTESIAN_POINT('Ctrl Pts',(4.03927895232327,3.10636808638158,30.5029746859145));
#46775=CARTESIAN_POINT('Ctrl Pts',(2.06154960910751,4.65996892178051,30.5823465759679));
#46776=CARTESIAN_POINT('Ctrl Pts',(-0.418368655724119,5.07841164249995,
30.6617184660213));
#46777=CARTESIAN_POINT('Ctrl Pts',(-2.79637324206467,4.25976452797996,30.7410903560747));
#46778=CARTESIAN_POINT('Ctrl Pts',(-4.49318749630546,2.4034482032729,30.8204622461281));
#46779=CARTESIAN_POINT('Ctrl Pts',(-5.09547122194811,-0.0383427838090456,
30.8998341361815));
#46780=CARTESIAN_POINT('Ctrl Pts',(-4.45650943655845,-2.47079355362547,
30.9792060262349));
#46781=CARTESIAN_POINT('Ctrl Pts',(-2.73195181673944,-4.3013644827875,31.0585779162883));
#46782=CARTESIAN_POINT('Ctrl Pts',(-0.341896781435476,-5.08413254485124,
31.1379498063417));
#46783=CARTESIAN_POINT('Ctrl Pts',(2.13144355305047,-4.62841717252575,31.2173216963952));
#46784=CARTESIAN_POINT('Ctrl Pts',(4.08556895588362,-3.04522962180058,31.2966935864485));
#46785=CARTESIAN_POINT('Ctrl Pts',(5.04445880431697,-0.720230875706232,
31.376065476502));
#46786=CARTESIAN_POINT('Ctrl Pts',(4.77452965373889,1.78021451750611,31.4554373665553));
#46787=CARTESIAN_POINT('Ctrl Pts',(3.34153564775218,3.84700359469197,31.5348092566088));
#46788=CARTESIAN_POINT('Ctrl Pts',(1.09455095433672,4.97667111140894,31.6141811466621));
#46789=CARTESIAN_POINT('Ctrl Pts',(-1.41906392880775,4.89403256106132,31.6935530367156));
#46790=CARTESIAN_POINT('Ctrl Pts',(-3.58699797993935,3.61921851159646,31.772924926769));
#46791=CARTESIAN_POINT('Ctrl Pts',(-4.88114726284307,1.46277084371106,31.8522968168224));
#46792=CARTESIAN_POINT('Ctrl Pts',(-4.98625987675445,-1.05000456391402,
31.9316687068758));
#46793=CARTESIAN_POINT('Ctrl Pts',(-3.87673062158748,-3.30700118391536,
32.0110405969292));
#46794=CARTESIAN_POINT('Ctrl Pts',(-1.82283836799946,-4.75841963543788,
32.0904124869826));
#46795=CARTESIAN_POINT('Ctrl Pts',(0.675093277248947,-5.0506975963509,32.169784377036));
#46796=CARTESIAN_POINT('Ctrl Pts',(3.00857369445308,-4.11263680232238,32.2491562670894));
#46797=CARTESIAN_POINT('Ctrl Pts',(4.60917221905339,-2.17274678641531,32.3285281571428));
#46798=CARTESIAN_POINT('Ctrl Pts',(5.08698659332197,0.296419537369132,32.4079000471962));
#46799=CARTESIAN_POINT('Ctrl Pts',(4.32562229331115,2.69337871796399,32.4872719372496));
#46800=CARTESIAN_POINT('Ctrl Pts',(2.51054597725224,4.43423680455544,32.566643827303));
#46801=CARTESIAN_POINT('Ctrl Pts',(0.0839062181339619,5.09492462057391,
32.6460157173564));
#46802=CARTESIAN_POINT('Ctrl Pts',(-2.3631729099985,4.51450007644488,32.7253876074099));
#46803=CARTESIAN_POINT('Ctrl Pts',(-4.23458834804982,2.8343533063703,32.8047594974632));
#46804=CARTESIAN_POINT('Ctrl Pts',(-5.07446743761851,0.463764344598583,
32.8841313875167));
#46805=CARTESIAN_POINT('Ctrl Pts',(-4.67821749152652,-2.01979658499237,
32.96350327757));
#46806=CARTESIAN_POINT('Ctrl Pts',(-3.14236411955747,-4.01133953722311,
33.0428751676235));
#46807=CARTESIAN_POINT('Ctrl Pts',(-0.841037803569241,-5.02572905713579,
33.1222470576768));
#46808=CARTESIAN_POINT('Ctrl Pts',(1.6651634597629,-4.81586210299279,33.2016189477303));
#46809=CARTESIAN_POINT('Ctrl Pts',(3.76573459007359,-3.43286180029067,33.2809908377836));
#46810=CARTESIAN_POINT('Ctrl Pts',(4.94898110955447,-1.21362396154845,33.3603627278371));
#46811=CARTESIAN_POINT('Ctrl Pts',(4.92666678513176,1.3012499879159,33.4397346178904));
#46812=CARTESIAN_POINT('Ctrl Pts',(3.70422733684289,3.49914232059194,33.5191065079439));
#46813=CARTESIAN_POINT('Ctrl Pts',(1.5794463084672,4.8446513291919,33.5984783979973));
#46814=CARTESIAN_POINT('Ctrl Pts',(-0.930084344605925,5.01001399745455,
33.6778502880506));
#46815=CARTESIAN_POINT('Ctrl Pts',(-3.21304851003985,3.95494834541518,33.7572221781041));
#46816=CARTESIAN_POINT('Ctrl Pts',(-4.71332117039034,1.93646603056234,33.8365940681574));
#46817=CARTESIAN_POINT('Ctrl Pts',(-5.06543922639319,-0.553735123040657,
33.9159659582109));
#46818=CARTESIAN_POINT('Ctrl Pts',(-4.18362749900617,-2.90904762634284,
33.9953378482642));
#46819=CARTESIAN_POINT('Ctrl Pts',(-2.28269337316369,-4.55572256693558,
34.0747097383177));
#46820=CARTESIAN_POINT('Ctrl Pts',(0.174299805725373,-5.0926335741437,34.154081628371));
#46821=CARTESIAN_POINT('Ctrl Pts',(2.58883393774586,-4.38899031504365,34.2334535184245));
#46822=CARTESIAN_POINT('Ctrl Pts',(4.37273385281817,-2.61619873006421,34.3128254084779));
#46823=CARTESIAN_POINT('Ctrl Pts',(5.09144548022617,-0.206106925298799,
34.3921972985313));
#46824=CARTESIAN_POINT('Ctrl Pts',(4.56989225837449,2.25419207025942,34.4715691885847));
#46825=CARTESIAN_POINT('Ctrl Pts',(2.93512339766776,4.16537486707196,34.5509410786381));
#46826=CARTESIAN_POINT('Ctrl Pts',(0.585364974074578,5.06188156616671,34.6303129686915));
#46827=CARTESIAN_POINT('Ctrl Pts',(-1.9069870615198,4.72532512002801,34.7096848587449));
#46828=CARTESIAN_POINT('Ctrl Pts',(-3.93480126997218,3.23768993398022,34.7890567487983));
#46829=CARTESIAN_POINT('Ctrl Pts',(-5.00410659859424,0.961360646519953,
34.8684286388517));
#46830=CARTESIAN_POINT('Ctrl Pts',(-4.85442263620079,-1.54915396649689,
34.9478005289051));
#46831=CARTESIAN_POINT('Ctrl Pts',(-3.52221206471105,-3.68229810226921,
35.0271724189585));
#46832=CARTESIAN_POINT('Ctrl Pts',(-1.33199843054191,-4.91844257095733,
35.1065443090119));
#46833=CARTESIAN_POINT('Ctrl Pts',(1.1826870729787,-4.95646531614826,35.1859161990653));
#46834=CARTESIAN_POINT('Ctrl Pts',(3.40927262335516,-3.78710408127537,35.2652880891187));
#46835=CARTESIAN_POINT('Ctrl Pts',(4.80536690897926,-1.69521267481654,35.3446599791721));
#46836=CARTESIAN_POINT('Ctrl Pts',(5.03088445207529,0.809628786938043,35.4240318692255));
#46837=CARTESIAN_POINT('Ctrl Pts',(4.0308896783196,3.11724646827744,35.503403759279));
#46838=CARTESIAN_POINT('Ctrl Pts',(2.04897910114821,4.66550980985245,35.5827756493324));
#46839=CARTESIAN_POINT('Ctrl Pts',(-0.432058249724576,5.0772652886782,35.6621475393857));
#46840=CARTESIAN_POINT('Ctrl Pts',(-2.80784716730917,4.25221018151802,35.7415194294392));
#46841=CARTESIAN_POINT('Ctrl Pts',(-4.49965073000152,2.39132608624762,35.8208913194925));
#46842=CARTESIAN_POINT('Ctrl Pts',(-5.09534933467344,-0.052079750522149,
35.9002632095459));
#46843=CARTESIAN_POINT('Ctrl Pts',(-4.4498321197834,-2.48279907534128,35.9796350995994));
#46844=CARTESIAN_POINT('Ctrl Pts',(-2.72034565005043,-4.30871404098988,
36.0590069896527));
#46845=CARTESIAN_POINT('Ctrl Pts',(-0.328189001348134,-5.08503580343008,
36.1383788797062));
#46846=CARTESIAN_POINT('Ctrl Pts',(2.14391376164854,-4.62265409969052,36.2177507697596));
#46847=CARTESIAN_POINT('Ctrl Pts',(4.0937638777802,-3.03420408933768,36.2971226598129));
#46848=CARTESIAN_POINT('Ctrl Pts',(5.0463821746773,-0.706628678919033,36.3764945498664));
#46849=CARTESIAN_POINT('Ctrl Pts',(4.76971294380048,1.79307991358828,36.4558664399198));
#46850=CARTESIAN_POINT('Ctrl Pts',(3.33115219739438,3.85599820806056,36.5352383299732));
#46851=CARTESIAN_POINT('Ctrl Pts',(1.08113014908331,4.97960387415652,36.6146102200266));
#46852=CARTESIAN_POINT('Ctrl Pts',(-1.4322528105034,4.89018905867418,36.69398211008));
#46853=CARTESIAN_POINT('Ctrl Pts',(-3.59674215568932,3.60953501274872,36.7733540001334));
#46854=CARTESIAN_POINT('Ctrl Pts',(-4.88507307300309,1.44960622728788,36.8527258901868));
#46855=CARTESIAN_POINT('Ctrl Pts',(-4.98341100265913,-1.06344342649134,
36.9320977802402));
#46856=CARTESIAN_POINT('Ctrl Pts',(-3.86780104266052,-3.31744061546937,
37.0114696702936));
#46857=CARTESIAN_POINT('Ctrl Pts',(-1.81000330990226,-4.76331661354924,
37.090841560347));
#46858=CARTESIAN_POINT('Ctrl Pts',(0.688707222773825,-5.04885922799112,
37.1702134504005));
#46859=CARTESIAN_POINT('Ctrl Pts',(3.0196502004098,-4.10451090995456,37.2495853404537));
#46860=CARTESIAN_POINT('Ctrl Pts',(4.61501307310836,-2.16031281943414,37.3289572305073));
#46861=CARTESIAN_POINT('Ctrl Pts',(5.08616897635574,0.310132692129688,37.4083291205606));
#46862=CARTESIAN_POINT('Ctrl Pts',(4.31834537500717,2.70503056635669,37.4877010106141));
#46863=CARTESIAN_POINT('Ctrl Pts',(2.49858239880182,4.44098898210481,37.5670729006674));
#46864=CARTESIAN_POINT('Ctrl Pts',(0.0701702807674692,5.09513231177087,
37.6464447907209));
#46865=CARTESIAN_POINT('Ctrl Pts',(-2.37533516234416,4.50811268818063,37.7258166807742));
#46866=CARTESIAN_POINT('Ctrl Pts',(-4.2422142176209,2.82292679227449,37.8051885708277));
#46867=CARTESIAN_POINT('Ctrl Pts',(-5.07569927947281,0.450082178237795,
37.884560460881));
#46868=CARTESIAN_POINT('Ctrl Pts',(-4.67275523170413,-2.03240145822491,
37.9639323509345));
#46869=CARTESIAN_POINT('Ctrl Pts',(-3.13153835248091,-4.01979659801907,
38.0433042409878));
#46870=CARTESIAN_POINT('Ctrl Pts',(-0.827485662097561,-5.02797818437316,
38.1226761310413));
#46871=CARTESIAN_POINT('Ctrl Pts',(1.6781407038918,-4.81135541393667,38.2020480210947));
#46872=CARTESIAN_POINT('Ctrl Pts',(3.77497570905148,-3.42269711502072,38.281419911148));
#46873=CARTESIAN_POINT('Ctrl Pts',(4.95223498699472,-1.20027737376265,38.3607918012015));
#46874=CARTESIAN_POINT('Ctrl Pts',(4.92314078418044,1.31452727683269,38.4401636912548));
#46875=CARTESIAN_POINT('Ctrl Pts',(3.69478038260533,3.50911599649374,38.5195355813083));
#46876=CARTESIAN_POINT('Ctrl Pts',(1.56637965982565,4.8488918190669,38.5989074713616));
#46877=CARTESIAN_POINT('Ctrl Pts',(-0.943587684251231,5.00748834177839,
38.6782793614151));
#46878=CARTESIAN_POINT('Ctrl Pts',(-3.22369915083517,3.94627176108658,38.7576512514684));
#46879=CARTESIAN_POINT('Ctrl Pts',(-4.71852465152966,1.92375216574096,38.8370231415219));
#46880=CARTESIAN_POINT('Ctrl Pts',(-5.06392796926474,-0.567389296122155,
38.9163950315753));
#46881=CARTESIAN_POINT('Ctrl Pts',(-4.17576968427578,-2.92031579800749,
38.9957669216287));
#46882=CARTESIAN_POINT('Ctrl Pts',(-2.27040306822808,-4.56186018168572,
39.0751388116821));
#46883=CARTESIAN_POINT('Ctrl Pts',(0.188028560849278,-5.0921448689568,39.1545107017355));
#46884=CARTESIAN_POINT('Ctrl Pts',(2.60065712992459,-4.38199557165452,39.2338825917889));
#46885=CARTESIAN_POINT('Ctrl Pts',(4.37977084759398,-2.60439952199669,39.3132544818424));
#46886=CARTESIAN_POINT('Ctrl Pts',(5.091983083909,-0.192381913948899,39.3926263718957));
#46887=CARTESIAN_POINT('Ctrl Pts',(4.56379761866661,2.26650781142318,39.4719982619492));
#46888=CARTESIAN_POINT('Ctrl Pts',(2.92388473013463,4.17326556172555,39.5513701520025));
#46889=CARTESIAN_POINT('Ctrl Pts',(0.571713243107522,5.06345468357226,39.6307420420559));
#46890=CARTESIAN_POINT('Ctrl Pts',(-1.91971357759784,4.72014150668349,39.7101139321093));
#46891=CARTESIAN_POINT('Ctrl Pts',(-3.94352649879586,3.22711800485078,39.7894858221628));
#46892=CARTESIAN_POINT('Ctrl Pts',(-5.00665954563271,0.947775616877117,
39.8688577122161));
#46893=CARTESIAN_POINT('Ctrl Pts',(-4.85026808817391,-1.56206090154421,
39.9482296022695));
#46894=CARTESIAN_POINT('Ctrl Pts',(-3.51219281059473,-3.69213734276829,
40.027601492323));
#46895=CARTESIAN_POINT('Ctrl Pts',(-2.05001543279097,-4.51147638686035,
40.0805160856919));
#46896=CARTESIAN_POINT('Ctrl Pts',(-1.2650852794273,-4.72177922709094,40.1069733823764));
#46897=CARTESIAN_POINT('Ctrl Pts',(-3.8562705385024,3.29705846079174,-0.320920147129055));
#46898=CARTESIAN_POINT('Ctrl Pts',(-4.40436067122819,2.6560070944272,-0.294462850444587));
#46899=CARTESIAN_POINT('Ctrl Pts',(-5.17416686787623,1.09598291074317,-0.241548257075651));
#46900=CARTESIAN_POINT('Ctrl Pts',(-5.06779668194698,-1.512680812799,-0.162176367022247));
#46901=CARTESIAN_POINT('Ctrl Pts',(-3.72722085031348,-3.75211381890485,
-0.0828044769688437));
#46902=CARTESIAN_POINT('Ctrl Pts',(-1.47855208449991,-5.07791790908896,
-0.00343258691543986));
#46903=CARTESIAN_POINT('Ctrl Pts',(1.1302101318597,-5.16655447652177,0.0759393031379633));
#46904=CARTESIAN_POINT('Ctrl Pts',(3.46369715057722,-3.99673439595713,0.155311193191368));
#46905=CARTESIAN_POINT('Ctrl Pts',(4.95341325213432,-1.85326330477546,0.23468308324477));
#46906=CARTESIAN_POINT('Ctrl Pts',(5.23650047694814,0.741629311098527,0.314054973298175));
#46907=CARTESIAN_POINT('Ctrl Pts',(4.24398161873799,3.15587819282154,0.393426863351577));
#46908=CARTESIAN_POINT('Ctrl Pts',(2.21764149317933,4.80135391043019,0.472798753404982));
#46909=CARTESIAN_POINT('Ctrl Pts',(-0.348912918530393,5.27723479734493,
0.552170643458385));
#46910=CARTESIAN_POINT('Ctrl Pts',(-2.83047200092439,4.46759066254957,0.631542533511789));
#46911=CARTESIAN_POINT('Ctrl Pts',(-4.62253485344812,2.56965255248809,0.710914423565193));
#46912=CARTESIAN_POINT('Ctrl Pts',(-5.28855819093304,0.045752121671659,
0.790286313618596));
#46913=CARTESIAN_POINT('Ctrl Pts',(-4.66630059499956,-2.48929308216644,
0.869658203672));
#46914=CARTESIAN_POINT('Ctrl Pts',(-2.90734243084918,-4.4179521825598,0.949030093725403));
#46915=CARTESIAN_POINT('Ctrl Pts',(-0.440162123945536,-5.27040781417518,
1.02840198377881));
#46916=CARTESIAN_POINT('Ctrl Pts',(2.1342407222512,-4.83900381899044,1.10777387383221));
#46917=CARTESIAN_POINT('Ctrl Pts',(4.18874724188064,-3.228829177505,1.18714576388562));
#46918=CARTESIAN_POINT('Ctrl Pts',(5.22288421068343,-0.832118909543204,
1.26651765393902));
#46919=CARTESIAN_POINT('Ctrl Pts',(4.98473814342391,1.76729369047769,1.34588954399242));
#46920=CARTESIAN_POINT('Ctrl Pts',(3.53232089954478,3.93619745533352,1.42526143404583));
#46921=CARTESIAN_POINT('Ctrl Pts',(1.21943810235538,5.14625223481536,1.50463332409923));
#46922=CARTESIAN_POINT('Ctrl Pts',(-1.39049711694202,5.10269135980955,1.58400521415263));
#46923=CARTESIAN_POINT('Ctrl Pts',(-3.66171031660135,3.81612616476449,1.66337710420604));
#46924=CARTESIAN_POINT('Ctrl Pts',(-5.04093898807,1.59996108251987,1.74274899425944));
#46925=CARTESIAN_POINT('Ctrl Pts',(-5.19220608004013,-1.00595097780601,
1.82212088431284));
#46926=CARTESIAN_POINT('Ctrl Pts',(-4.07866326363067,-3.3668156066614,1.90149277436625));
#46927=CARTESIAN_POINT('Ctrl Pts',(-1.97156710418735,-4.90753140600723,
1.98086466441965));
#46928=CARTESIAN_POINT('Ctrl Pts',(0.61579843785608,-5.25278341751101,2.06023655447306));
#46929=CARTESIAN_POINT('Ctrl Pts',(3.0531568434793,-4.31846901533485,2.13960844452646));
#46930=CARTESIAN_POINT('Ctrl Pts',(4.74677300008174,-2.3321851197991,2.21898033457986));
#46931=CARTESIAN_POINT('Ctrl Pts',(5.28408576066664,0.222213908719184,2.29835222463327));
#46932=CARTESIAN_POINT('Ctrl Pts',(4.53420692607935,2.72248212093367,2.37772411468667));
#46933=CARTESIAN_POINT('Ctrl Pts',(2.67980532059554,4.5595597146017,2.45709600474007));
#46934=CARTESIAN_POINT('Ctrl Pts',(0.172609070663326,5.28593865420646,2.53646789479348));
#46935=CARTESIAN_POINT('Ctrl Pts',(-2.37663436681889,4.72467463787357,2.61583978484688));
#46936=CARTESIAN_POINT('Ctrl Pts',(-4.34693493313492,3.01249033764445,2.69521167490029));
#46937=CARTESIAN_POINT('Ctrl Pts',(-5.25833177151656,0.56647005919948,2.77458356495369));
#46938=CARTESIAN_POINT('Ctrl Pts',(-4.88881062947673,-2.01754107180632,
2.85395545500709));
#46939=CARTESIAN_POINT('Ctrl Pts',(-3.32838603929513,-4.11008366347149,
2.93332734506049));
#46940=CARTESIAN_POINT('Ctrl Pts',(-0.957173977198773,-5.20141897223089,
3.0126992351139));
#46941=CARTESIAN_POINT('Ctrl Pts',(1.64720354707453,-5.02570013250045,3.0920711251673));
#46942=CARTESIAN_POINT('Ctrl Pts',(3.85032593330369,-3.62573186469146,3.1714430152207));
#46943=CARTESIAN_POINT('Ctrl Pts',(5.11551744473197,-1.342543340065,3.25081490527411));
#46944=CARTESIAN_POINT('Ctrl Pts',(5.13458022962935,1.26768577053204,3.33018679532751));
#46945=CARTESIAN_POINT('Ctrl Pts',(3.90287063578958,3.56910943340232,3.40955868538091));
#46946=CARTESIAN_POINT('Ctrl Pts',(1.7204303939291,5.00110593838552,3.48893057543432));
#46947=CARTESIAN_POINT('Ctrl Pts',(-0.881102883784432,5.21484410653825,
3.56830246548772));
#46948=CARTESIAN_POINT('Ctrl Pts',(-3.26800144929621,4.15825779319991,3.64767435554113));
#46949=CARTESIAN_POINT('Ctrl Pts',(-4.85882209535798,2.08872908558557,3.72704624559453));
#46950=CARTESIAN_POINT('Ctrl Pts',(-5.2660444338108,-0.489609403954008,
3.80641813564793));
#46951=CARTESIAN_POINT('Ctrl Pts',(-4.39047000437897,-2.94868012642242,
3.88579002570134));
#46952=CARTESIAN_POINT('Ctrl Pts',(-2.44538680002092,-4.68945889688708,
3.96516191575474));
#46953=CARTESIAN_POINT('Ctrl Pts',(0.0953872160503347,-5.28789586001125,
4.04453380580815));
#46954=CARTESIAN_POINT('Ctrl Pts',(2.61292511742776,-4.59821309619564,4.12390569586154));
#46955=CARTESIAN_POINT('Ctrl Pts',(4.49396024381142,-2.78841580011883,4.20327758591496));
#46956=CARTESIAN_POINT('Ctrl Pts',(5.28027660201492,-0.299366587186749,
4.28264947596836));
#46957=CARTESIAN_POINT('Ctrl Pts',(4.78032926766157,2.26260766374733,4.36202136602176));
#46958=CARTESIAN_POINT('Ctrl Pts',(3.11590430478523,4.27341569598967,4.44139325607517));
#46959=CARTESIAN_POINT('Ctrl Pts',(0.692451950200399,5.24322912373411,4.52076514612856));
#46960=CARTESIAN_POINT('Ctrl Pts',(-1.89968016673685,4.93580354262775,4.60013703618198));
#46961=CARTESIAN_POINT('Ctrl Pts',(-4.02905439992773,3.42602714375309,4.67950892623537));
#46962=CARTESIAN_POINT('Ctrl Pts',(-5.17695989945686,1.08167811604265,4.75888081628878));
#46963=CARTESIAN_POINT('Ctrl Pts',(-5.06376942648468,-1.5261653064819,4.83825270634218));
#46964=CARTESIAN_POINT('Ctrl Pts',(-3.71705592968434,-3.76223823845706,
4.91762459639559));
#46965=CARTESIAN_POINT('Ctrl Pts',(-1.46487583597662,-5.08183826311717,
4.996996486449));
#46966=CARTESIAN_POINT('Ctrl Pts',(1.14414476892732,-5.16351373534013,5.07636837650239));
#46967=CARTESIAN_POINT('Ctrl Pts',(3.47445424064207,-3.98736869087803,5.15574026655581));
#46968=CARTESIAN_POINT('Ctrl Pts',(4.95839434991041,-1.83990945920892,5.2351121566092));
#46969=CARTESIAN_POINT('Ctrl Pts',(5.23448057076031,0.75574764415296,5.31448404666261));
#46970=CARTESIAN_POINT('Ctrl Pts',(4.23545891089922,3.1673062942182,5.39385593671601));
#46971=CARTESIAN_POINT('Ctrl Pts',(2.20468883537238,4.80731614172549,5.47322782676942));
#46972=CARTESIAN_POINT('Ctrl Pts',(-0.363138560455233,5.27627441792221,
5.55259971682281));
#46973=CARTESIAN_POINT('Ctrl Pts',(-2.84250620674952,4.45994392474844,5.63197160687622));
#46974=CARTESIAN_POINT('Ctrl Pts',(-4.62944563286038,2.55718096342436,5.71134349692963));
#46975=CARTESIAN_POINT('Ctrl Pts',(-5.28866234991055,0.0314943796341776,
5.79071538698302));
#46976=CARTESIAN_POINT('Ctrl Pts',(-4.65957262477808,-2.50186416532327,
5.87008727703643));
#46977=CARTESIAN_POINT('Ctrl Pts',(-2.89542132203872,-4.42577413739037,
5.94945916708984));
#46978=CARTESIAN_POINT('Ctrl Pts',(-0.425951794157121,-5.27157532587407,
6.02883105714324));
#46979=CARTESIAN_POINT('Ctrl Pts',(2.14727864795285,-4.8332324334089,6.10820294719664));
#46980=CARTESIAN_POINT('Ctrl Pts',(4.19743676434218,-3.21752481834385,6.18757483725004));
#46981=CARTESIAN_POINT('Ctrl Pts',(5.22510857580644,-0.81803527940062,6.26694672730345));
#46982=CARTESIAN_POINT('Ctrl Pts',(4.97995550378589,1.78072584291422,6.34631861735685));
#46983=CARTESIAN_POINT('Ctrl Pts',(3.52169629398765,3.94570609146495,6.42569050741027));
#46984=CARTESIAN_POINT('Ctrl Pts',(1.20555966211655,5.14952106980711,6.50506239746365));
#46985=CARTESIAN_POINT('Ctrl Pts',(-1.40424863498509,5.09892411381582,6.58443428751707));
#46986=CARTESIAN_POINT('Ctrl Pts',(-3.67198507285601,3.80624052997609,6.66380617757046));
#46987=CARTESIAN_POINT('Ctrl Pts',(-5.04523407478029,1.58636517800468,6.74317806762388));
#46988=CARTESIAN_POINT('Ctrl Pts',(-5.1894752235243,-1.01994521996889,6.82254995767727));
#46989=CARTESIAN_POINT('Ctrl Pts',(-4.06957169452636,-3.37779921996849,
6.90192184773068));
#46990=CARTESIAN_POINT('Ctrl Pts',(-1.95832950858598,-4.91282880661553,
6.98129373778407));
#46991=CARTESIAN_POINT('Ctrl Pts',(0.629957410957137,-5.25110417033315,
7.06066562783749));
#46992=CARTESIAN_POINT('Ctrl Pts',(3.06478809957816,-4.31022218127953,7.14003751789089));
#46993=CARTESIAN_POINT('Ctrl Pts',(4.75304319093534,-2.31937960938119,7.21940940794429));
#46994=CARTESIAN_POINT('Ctrl Pts',(5.28346748166331,0.236458701502723,7.2987812979977));
#46995=CARTESIAN_POINT('Ctrl Pts',(4.52685078861501,2.73469619609302,7.37815318805109));
#46996=CARTESIAN_POINT('Ctrl Pts',(2.66750326347436,4.56676775046241,7.45752507810451));
#46997=CARTESIAN_POINT('Ctrl Pts',(0.158357847769689,5.28638478918814,7.5368969681579));
#46998=CARTESIAN_POINT('Ctrl Pts',(-2.38936318913255,4.71825019448189,7.61626885821132));
#46999=CARTESIAN_POINT('Ctrl Pts',(-4.3550406419278,3.0007602960695,7.69564074826471));
#47000=CARTESIAN_POINT('Ctrl Pts',(-5.25983983406839,0.552291831604834,
7.77501263831812));
#47001=CARTESIAN_POINT('Ctrl Pts',(-4.88335368508791,-2.03071370056153,
7.85438452837152));
#47002=CARTESIAN_POINT('Ctrl Pts',(-3.31729338754006,-4.11904187017964,
7.93375641842492));
#47003=CARTESIAN_POINT('Ctrl Pts',(-0.943147763491834,-5.20398055756651,
8.01312830847834));
#47004=CARTESIAN_POINT('Ctrl Pts',(1.66074656812082,-5.02124109994579,8.09250019853171));
#47005=CARTESIAN_POINT('Ctrl Pts',(3.86008671173945,-3.61533842470695,8.17187208858515));
#47006=CARTESIAN_POINT('Ctrl Pts',(5.11911827653537,-1.32874731162534,8.25124397863853));
#47007=CARTESIAN_POINT('Ctrl Pts',(5.13114396014337,1.28152370543593,8.33061586869195));
#47008=CARTESIAN_POINT('Ctrl Pts',(3.89323433265495,3.57961838445758,8.40998775874535));
#47009=CARTESIAN_POINT('Ctrl Pts',(1.70694143925982,5.00572594837628,8.48935964879875));
#47010=CARTESIAN_POINT('Ctrl Pts',(-0.895158610488236,5.21244975125697,
8.56873153885215));
#47011=CARTESIAN_POINT('Ctrl Pts',(-3.27920000412133,4.14943233229326,8.64810342890557));
#47012=CARTESIAN_POINT('Ctrl Pts',(-4.86443553513654,2.0756223817956,8.72747531895896));
#47013=CARTESIAN_POINT('Ctrl Pts',(-5.26470533703792,-0.503804586595236,
8.80684720901237));
#47014=CARTESIAN_POINT('Ctrl Pts',(-4.38250457206448,-2.96050587284403,
8.88621909906576));
#47015=CARTESIAN_POINT('Ctrl Pts',(-2.43273539384546,-4.69603448143659,
8.96559098911917));
#47016=CARTESIAN_POINT('Ctrl Pts',(0.109642741545844,-5.28761948484726,
9.04496287917257));
#47017=CARTESIAN_POINT('Ctrl Pts',(2.62531214778668,-4.59115208569632,9.12433476922599));
#47018=CARTESIAN_POINT('Ctrl Pts',(4.50146132585655,-2.77629020081255,9.20370665927937));
#47019=CARTESIAN_POINT('Ctrl Pts',(5.28106448876342,-0.285130168224959,
9.28307854933281));
#47020=CARTESIAN_POINT('Ctrl Pts',(4.77421203164548,2.27548694221733,9.36245043938617));
#47021=CARTESIAN_POINT('Ctrl Pts',(3.10437209115777,4.28180047024037,9.44182232943961));
#47022=CARTESIAN_POINT('Ctrl Pts',(0.67831398067512,5.24507688131743,9.52119421949299));
#47023=CARTESIAN_POINT('Ctrl Pts',(-1.91297991407746,4.93066417388633,9.6005661095464));
#47024=CARTESIAN_POINT('Ctrl Pts',(-4.03827613607002,3.41515258753654,9.6799379995998));
#47025=CARTESIAN_POINT('Ctrl Pts',(-5.1798572298885,1.06771739017486,9.75930988965322));
#47026=CARTESIAN_POINT('Ctrl Pts',(-5.05963656792565,-1.53981140008104,
9.8386817797066));
#47027=CARTESIAN_POINT('Ctrl Pts',(-3.70689963733171,-3.77224554159189,
9.91805366976003));
#47028=CARTESIAN_POINT('Ctrl Pts',(-1.45117016016697,-5.08576901889487,
9.99742555981341));
#47029=CARTESIAN_POINT('Ctrl Pts',(1.1580611559038,-5.16041042035386,10.0767974498668));
#47030=CARTESIAN_POINT('Ctrl Pts',(3.48519133772131,-3.97798726578937,10.1561693399202));
#47031=CARTESIAN_POINT('Ctrl Pts',(4.96333662401008,-1.82653521840402,10.2355412299736));
#47032=CARTESIAN_POINT('Ctrl Pts',(5.23242409484924,0.769856765217389,10.314913120027));
#47033=CARTESIAN_POINT('Ctrl Pts',(4.22690463795744,3.1787133448809,10.3942850100804));
#47034=CARTESIAN_POINT('Ctrl Pts',(2.1917205673539,4.81324238969408,10.4736569001339));
#47035=CARTESIAN_POINT('Ctrl Pts',(-0.377361782165876,5.27527624230907,
10.5530287901872));
#47036=CARTESIAN_POINT('Ctrl Pts',(-2.85451963682615,4.45226447892349,10.6324006802407));
#47037=CARTESIAN_POINT('Ctrl Pts',(-4.63632282632763,2.54469094339242,10.711772570294));
#47038=CARTESIAN_POINT('Ctrl Pts',(-5.28872803766221,0.0172363266288179,
10.7911444603475));
#47039=CARTESIAN_POINT('Ctrl Pts',(-4.65281080542322,-2.5144170211496,10.8705163504009));
#47040=CARTESIAN_POINT('Ctrl Pts',(-2.88347915980519,-4.43356394814365,
10.9498882404543));
#47041=CARTESIAN_POINT('Ctrl Pts',(-0.411738373331464,-5.27270451089727,
11.0292601305077));
#47042=CARTESIAN_POINT('Ctrl Pts',(2.16030096951836,-4.82742592572977,11.1086320205611));
#47043=CARTESIAN_POINT('Ctrl Pts',(4.20609577793862,-3.20619707038057,11.1880039106145));
#47044=CARTESIAN_POINT('Ctrl Pts',(5.22729496488813,-0.803945705483474,
11.2673758006679));
#47045=CARTESIAN_POINT('Ctrl Pts',(4.975136668812,1.79414505376576,11.3467476907213));
#47046=CARTESIAN_POINT('Ctrl Pts',(3.51104609249152,3.95518604919035,11.4261195807747));
#47047=CARTESIAN_POINT('Ctrl Pts',(1.19167245960881,5.152752477688,11.5054914708281));
#47048=CARTESIAN_POINT('Ctrl Pts',(-1.41798994671238,5.09511980804502,11.5848633608815));
#47049=CARTESIAN_POINT('Ctrl Pts',(-3.68223314068194,3.79632723101863,11.6642352509349));
#47050=CARTESIAN_POINT('Ctrl Pts',(-5.04949249206616,1.57275774354392,11.7436071409883));
#47051=CARTESIAN_POINT('Ctrl Pts',(-5.18670664924514,-1.03393204901786,
11.8229790310417));
#47052=CARTESIAN_POINT('Ctrl Pts',(-4.06045054724843,-3.38875828300867,
11.9023509210951));
#47053=CARTESIAN_POINT('Ctrl Pts',(-1.94507767959685,-4.91809050014781,
11.9817228111485));
#47054=CARTESIAN_POINT('Ctrl Pts',(0.644111805448097,-5.24938675745961,
12.0610947012019));
#47055=CARTESIAN_POINT('Ctrl Pts',(3.0763970804032,-4.30194401997477,12.1404665912553));
#47056=CARTESIAN_POINT('Ctrl Pts',(4.7592788360615,-2.30655724141565,12.2198384813087));
#47057=CARTESIAN_POINT('Ctrl Pts',(5.28281080174027,0.250701775674464,12.2992103713621));
#47058=CARTESIAN_POINT('Ctrl Pts',(4.51946174941847,2.74689039512926,12.3785822614155));
#47059=CARTESIAN_POINT('Ctrl Pts',(2.6551818185972,4.57394259446934,12.4579541514689));
#47060=CARTESIAN_POINT('Ctrl Pts',(0.144105473910954,5.28679250204684,12.5373260415223));
#47061=CARTESIAN_POINT('Ctrl Pts',(-2.40207464524796,4.7117914582425,12.6166979315757));
#47062=CARTESIAN_POINT('Ctrl Pts',(-4.36311469772651,2.98900844458373,12.6960698216291));
#47063=CARTESIAN_POINT('Ctrl Pts',(-5.26130966742946,0.538109589882336,
12.7754417116825));
#47064=CARTESIAN_POINT('Ctrl Pts',(-4.87786124785798,-2.043871569829,12.854813601736));
#47065=CARTESIAN_POINT('Ctrl Pts',(-3.30617662527107,-4.12797013916298,
12.9341854917893));
#47066=CARTESIAN_POINT('Ctrl Pts',(-0.929114694865931,-5.20650431970379,
13.0135573818428));
#47067=CARTESIAN_POINT('Ctrl Pts',(1.67427751864803,-5.01674557236658,13.0929292718962));
#47068=CARTESIAN_POINT('Ctrl Pts',(3.86981943456978,-3.60491870797887,13.1723011619496));
#47069=CARTESIAN_POINT('Ctrl Pts',(5.12268190193035,-1.31494162567972,13.251673052003));
#47070=CARTESIAN_POINT('Ctrl Pts',(5.12767039684476,1.29535232606109,13.3310449420564));
#47071=CARTESIAN_POINT('Ctrl Pts',(3.8835697329937,3.59010131838716,13.4104168321098));
#47072=CARTESIAN_POINT('Ctrl Pts',(1.69344007832116,5.01030957610862,13.4897887221632));
#47073=CARTESIAN_POINT('Ctrl Pts',(-0.909207831064397,5.21001751122212,
13.5691606122166));
#47074=CARTESIAN_POINT('Ctrl Pts',(-3.29037472530003,4.14057671278008,13.64853250227));
#47075=CARTESIAN_POINT('Ctrl Pts',(-4.87001361957351,2.06250059211591,13.7279043923234));
#47076=CARTESIAN_POINT('Ctrl Pts',(-5.26332797571119,-0.517996107520081,
13.8072762823768));
#47077=CARTESIAN_POINT('Ctrl Pts',(-4.37450728714447,-2.97231010192914,
13.8866481724302));
#47078=CARTESIAN_POINT('Ctrl Pts',(-2.420066306237,-4.70257593460501,13.9660200624836));
#47079=CARTESIAN_POINT('Ctrl Pts',(0.123897470143854,-5.28730467858643,
14.045391952537));
#47080=CARTESIAN_POINT('Ctrl Pts',(2.63768009704007,-4.58405770611459,14.1247638425904));
#47081=CARTESIAN_POINT('Ctrl Pts',(4.50892969070322,-2.76414442307289,14.2041357326438));
#47082=CARTESIAN_POINT('Ctrl Pts',(5.28181399205766,-0.270891676900501,
14.2835076226972));
#47083=CARTESIAN_POINT('Ctrl Pts',(4.7680600960438,2.28834968215629,14.3628795127506));
#47084=CARTESIAN_POINT('Ctrl Pts',(3.09281731455568,4.29015412381589,14.442251402804));
#47085=CARTESIAN_POINT('Ctrl Pts',(0.664171081076821,5.24688651700904,14.5216232928574));
#47086=CARTESIAN_POINT('Ctrl Pts',(-1.92626575763464,4.9254889684451,14.6009951829108));
#47087=CARTESIAN_POINT('Ctrl Pts',(-4.04746852150321,3.4042532095528,14.6803670729642));
#47088=CARTESIAN_POINT('Ctrl Pts',(-5.1827169124532,1.05374890400015,14.7597389630177));
#47089=CARTESIAN_POINT('Ctrl Pts',(-5.05546693527891,-1.55344630213332,
14.839110853071));
#47090=CARTESIAN_POINT('Ctrl Pts',(-3.69671640275692,-3.78222542756219,
14.9184827431245));
#47091=CARTESIAN_POINT('Ctrl Pts',(-1.43745393706629,-5.08966281065088,
14.9978546331779));
#47092=CARTESIAN_POINT('Ctrl Pts',(1.17196912594334,-5.15726959884254,15.0772265232312));
#47093=CARTESIAN_POINT('Ctrl Pts',(3.49590310398282,-3.96857692817882,15.1565984132847));
#47094=CARTESIAN_POINT('Ctrl Pts',(4.96824282394235,-1.81314770210679,15.2359703033381));
#47095=CARTESIAN_POINT('Ctrl Pts',(5.23032958900857,0.783960290864088,15.3153421933915));
#47096=CARTESIAN_POINT('Ctrl Pts',(4.21831964333036,3.19009729224721,15.3947140834449));
#47097=CARTESIAN_POINT('Ctrl Pts',(2.17873636962922,4.81913365439941,15.4740859734983));
#47098=CARTESIAN_POINT('Ctrl Pts',(-0.391582261162836,5.27423972531144,
15.5534578635517));
#47099=CARTESIAN_POINT('Ctrl Pts',(-2.86651231988745,4.44455267346898,15.6328297536051));
#47100=CARTESIAN_POINT('Ctrl Pts',(-4.64316632240643,2.53218242822043,15.7122016436585));
#47101=CARTESIAN_POINT('Ctrl Pts',(-5.28875528625864,0.00297814834715876,
15.7915735337119));
#47102=CARTESIAN_POINT('Ctrl Pts',(-4.64601516884489,-2.52695160186966,
15.8709454237653));
#47103=CARTESIAN_POINT('Ctrl Pts',(-2.87151604007055,-4.44132153518687,
15.9503173138187));
#47104=CARTESIAN_POINT('Ctrl Pts',(-0.397521959947054,-5.27379537322474,
16.0296892038721));
#47105=CARTESIAN_POINT('Ctrl Pts',(2.1733075897557,-4.82158433170501,16.1090610939255));
#47106=CARTESIAN_POINT('Ctrl Pts',(4.21472422106055,-3.1948460193553,16.1884329839789));
#47107=CARTESIAN_POINT('Ctrl Pts',(5.22944336137754,-0.789850288404984,
16.2678048740323));
#47108=CARTESIAN_POINT('Ctrl Pts',(4.97028167379658,1.80755122457726,16.3471767640857));
#47109=CARTESIAN_POINT('Ctrl Pts',(3.50037037246945,3.9646372600474,16.4265486541391));
#47110=CARTESIAN_POINT('Ctrl Pts',(1.17777659548083,5.15594643483254,16.5059205441925));
#47111=CARTESIAN_POINT('Ctrl Pts',(-1.43172095156687,5.09127847004474,16.5852924342459));
#47112=CARTESIAN_POINT('Ctrl Pts',(-3.69245444696213,3.78638634033038,16.6646643242993));
#47113=CARTESIAN_POINT('Ctrl Pts',(-5.05371420635461,1.5591388772047,16.7440362143527));
#47114=CARTESIAN_POINT('Ctrl Pts',(-5.18390038229795,-1.04791136166686,
16.8234081044061));
#47115=CARTESIAN_POINT('Ctrl Pts',(-4.05129987868913,-3.39969271923294,
16.9027799944595));
#47116=CARTESIAN_POINT('Ctrl Pts',(-1.93181173129365,-4.9233164424874,16.9821518845129));
#47117=CARTESIAN_POINT('Ctrl Pts',(0.658261551986501,-5.24763120247215,
17.0615237745663));
#47118=CARTESIAN_POINT('Ctrl Pts',(3.08798363825942,-4.29363457062506,17.1408956646198));
#47119=CARTESIAN_POINT('Ctrl Pts',(4.76548000969996,-2.29371814868002,17.2202675546731));
#47120=CARTESIAN_POINT('Ctrl Pts',(5.28211549991427,0.264943102456271,17.2996394447266));
#47121=CARTESIAN_POINT('Ctrl Pts',(4.51204028846775,2.7590644882845,17.3790113347799));
#47122=CARTESIAN_POINT('Ctrl Pts',(2.64284027062647,4.58108446095533,17.4583832248334));
#47123=CARTESIAN_POINT('Ctrl Pts',(0.129853572473924,5.28716128664959,17.5377551148867));
#47124=CARTESIAN_POINT('Ctrl Pts',(-2.41477151246584,4.70529942618515,17.6171270049402));
#47125=CARTESIAN_POINT('Ctrl Pts',(-4.37115162329109,2.9772330746438,17.6964988949936));
#47126=CARTESIAN_POINT('Ctrl Pts',(-5.2627514922539,0.523926824466488,17.775870785047));
#47127=CARTESIAN_POINT('Ctrl Pts',(-4.87231403886184,-2.05702097999283,
17.8552426751004));
#47128=CARTESIAN_POINT('Ctrl Pts',(-3.29507231119166,-4.13685632854999,
17.9346145651538));
#47129=CARTESIAN_POINT('Ctrl Pts',(-0.915005995631555,-5.20901304408194,
18.0139864552072));
#47130=CARTESIAN_POINT('Ctrl Pts',(1.68766624540468,-5.01217052435341,18.0933583452606));
#47131=CARTESIAN_POINT('Ctrl Pts',(3.8797695997979,-3.59455409188004,18.172730235314));
#47132=CARTESIAN_POINT('Ctrl Pts',(5.12574462250332,-1.30097287489382,18.2521021253674));
#47133=CARTESIAN_POINT('Ctrl Pts',(5.12503498129813,1.3088817301615,18.3314740154208));
#47134=CARTESIAN_POINT('Ctrl Pts',(3.87222469260764,3.60110493868871,18.4108459054742));
#47135=CARTESIAN_POINT('Ctrl Pts',(1.68303999757325,5.01382783115876,18.4902177955276));
#47136=CARTESIAN_POINT('Ctrl Pts',(-0.929079443196312,5.2094618875472,18.569589685581));
#47137=CARTESIAN_POINT('Ctrl Pts',(-3.29092685490746,4.12830747359753,18.6489615756344));
#47138=CARTESIAN_POINT('Ctrl Pts',(-5.42625155540715,1.36247937795741,18.7547907623723));
#47139=CARTESIAN_POINT('Ctrl Pts',(-4.95432466322409,-3.37745298000962,
18.8870772457946));
#47140=CARTESIAN_POINT('Ctrl Pts',(0.158509478955228,-5.99736559883162,
19.0458210259014));
#47141=CARTESIAN_POINT('Ctrl Pts',(5.11967904485094,-3.11863163173532,19.2045648060083));
#47142=CARTESIAN_POINT('Ctrl Pts',(5.39954635636598,2.60828838171404,19.363308586115));
#47143=CARTESIAN_POINT('Ctrl Pts',(0.736723079475925,5.95134306184737,19.5220523662219));
#47144=CARTESIAN_POINT('Ctrl Pts',(-4.59927593805429,3.84720861430001,19.6807961463287));
#47145=CARTESIAN_POINT('Ctrl Pts',(-5.72720375155086,-1.77677009197966,
19.8395399264355));
#47146=CARTESIAN_POINT('Ctrl Pts',(-1.61419617037545,-5.77483540889735,
19.9982837065423));
#47147=CARTESIAN_POINT('Ctrl Pts',(3.97578039972893,-4.48936692070975,20.1570274866491));
#47148=CARTESIAN_POINT('Ctrl Pts',(5.92771323046147,0.905806267444479,20.3157712667559));
#47149=CARTESIAN_POINT('Ctrl Pts',(2.45559119020176,5.46873373673919,20.4745150468627));
#47150=CARTESIAN_POINT('Ctrl Pts',(-3.26379011618977,5.03400372054189,20.6332588269695));
#47151=CARTESIAN_POINT('Ctrl Pts',(-5.99600976813329,-0.0197068834827358,
20.7920026070763));
#47152=CARTESIAN_POINT('Ctrl Pts',(-3.70230252414087,-4.19446206534972,
20.9242890904987));
#47153=CARTESIAN_POINT('Ctrl Pts',(-0.376480053418488,-5.26605971579228,
21.0301182772365));
#47154=CARTESIAN_POINT('Ctrl Pts',(2.18257651229242,-4.8205851862161,21.10949016729));
#47155=CARTESIAN_POINT('Ctrl Pts',(4.22530652207796,-3.18086119603153,21.1888620573433));
#47156=CARTESIAN_POINT('Ctrl Pts',(5.23050112077121,-0.777135043026565,
21.2682339473968));
#47157=CARTESIAN_POINT('Ctrl Pts',(4.96594823061178,1.82167865277159,21.3476058374501));
#47158=CARTESIAN_POINT('Ctrl Pts',(3.48937383888172,3.97367066688458,21.4269777275036));
#47159=CARTESIAN_POINT('Ctrl Pts',(1.16402860508423,5.15930893371516,21.5063496175569));
#47160=CARTESIAN_POINT('Ctrl Pts',(-1.44552439996815,5.08729102078623,21.5857215076104));
#47161=CARTESIAN_POINT('Ctrl Pts',(-3.70260503654192,3.77647571272897,21.6650933976637));
#47162=CARTESIAN_POINT('Ctrl Pts',(-5.057922432142,1.54547807796832,21.7444652877172));
#47163=CARTESIAN_POINT('Ctrl Pts',(-5.18104412158608,-1.06186685398839,
21.8238371777705));
#47164=CARTESIAN_POINT('Ctrl Pts',(-4.04212630117128,-3.41061102326193,
21.903209067824));
#47165=CARTESIAN_POINT('Ctrl Pts',(-1.91852825506946,-4.92850206746972,
21.9825809578774));
#47166=CARTESIAN_POINT('Ctrl Pts',(0.672404619068471,-5.245839892308,22.0619528479308));
#47167=CARTESIAN_POINT('Ctrl Pts',(3.09954884704109,-4.28529268150223,22.1413247379842));
#47168=CARTESIAN_POINT('Ctrl Pts',(4.77164579536192,-2.28086298099128,22.2206966280376));
#47169=CARTESIAN_POINT('Ctrl Pts',(5.28138253005217,0.279182711729235,22.300068518091));
#47170=CARTESIAN_POINT('Ctrl Pts',(4.50458503707303,2.77121862106756,22.3794404081444));
#47171=CARTESIAN_POINT('Ctrl Pts',(2.63048120009391,4.58819259887664,22.4588122981978));
#47172=CARTESIAN_POINT('Ctrl Pts',(0.115597647321455,5.28749259670008,22.5381841882512));
#47173=CARTESIAN_POINT('Ctrl Pts',(-2.42744506809483,4.69877132337436,22.6175560783046));
#47174=CARTESIAN_POINT('Ctrl Pts',(-4.37916762715256,2.96543963879382,22.696927968358));
#47175=CARTESIAN_POINT('Ctrl Pts',(-5.26413459813381,0.509733484286287,
22.7762998584114));
#47176=CARTESIAN_POINT('Ctrl Pts',(-4.86677005798463,-2.07014265165558,
22.8556717484648));
#47177=CARTESIAN_POINT('Ctrl Pts',(-3.28387109087741,-4.14573660239302,
22.9350436385182));
#47178=CARTESIAN_POINT('Ctrl Pts',(-0.901028401772815,-5.21143830245831,
23.0144155285717));
#47179=CARTESIAN_POINT('Ctrl Pts',(1.70130281532621,-5.00764516247504,23.093787418625));
#47180=CARTESIAN_POINT('Ctrl Pts',(3.88920043041414,-3.58400074773866,23.1731593086785));
#47181=CARTESIAN_POINT('Ctrl Pts',(5.12969743029434,-1.28730168253193,23.2525311987318));
#47182=CARTESIAN_POINT('Ctrl Pts',(5.12061148999571,1.32298122241883,23.3319030887853));
#47183=CARTESIAN_POINT('Ctrl Pts',(3.86415592530766,3.6109888303426,23.4112749788386));
#47184=CARTESIAN_POINT('Ctrl Pts',(1.66640053022393,5.01936755177924,23.4906468688921));
#47185=CARTESIAN_POINT('Ctrl Pts',(-0.937286345425383,5.20503944789203,
23.5700187589454));
#47186=CARTESIAN_POINT('Ctrl Pts',(-3.31265234202061,4.12277525560054,23.6493906489989));
#47187=CARTESIAN_POINT('Ctrl Pts',(-4.88106356050821,2.03621213668325,23.7287625390522));
#47188=CARTESIAN_POINT('Ctrl Pts',(-5.26045849971908,-0.546367751667005,
23.8081344291057));
#47189=CARTESIAN_POINT('Ctrl Pts',(-4.35841739221935,-2.99585366506712,
23.887506319159));
#47190=CARTESIAN_POINT('Ctrl Pts',(-2.3946754551717,-4.71555625687105,23.9668782092125));
#47191=CARTESIAN_POINT('Ctrl Pts',(0.152404122233421,-5.28655978220554,
24.0462500992659));
#47192=CARTESIAN_POINT('Ctrl Pts',(2.66235839280233,-4.56976904619763,24.1256219893193));
#47193=CARTESIAN_POINT('Ctrl Pts',(4.52376805191542,-2.73979268554746,24.2049938793727));
#47194=CARTESIAN_POINT('Ctrl Pts',(5.28319782677237,-0.242408891126616,
24.2843657694261));
#47195=CARTESIAN_POINT('Ctrl Pts',(4.75565230518779,2.3140251726099,24.3637376594795));
#47196=CARTESIAN_POINT('Ctrl Pts',(3.0696404085172,4.30676782630642,24.4431095495329));
#47197=CARTESIAN_POINT('Ctrl Pts',(0.635870902865647,5.25039137038364,24.5224814395863));
#47198=CARTESIAN_POINT('Ctrl Pts',(-1.95279534724764,4.9150311981795,24.6018533296397));
#47199=CARTESIAN_POINT('Ctrl Pts',(-4.06576497321052,3.38238030533593,24.6812252196931));
#47200=CARTESIAN_POINT('Ctrl Pts',(-5.18832325111748,1.02578905688434,24.7605971097465));
#47201=CARTESIAN_POINT('Ctrl Pts',(-5.04701746921096,-1.58068213527875,
24.8399689997999));
#47202=CARTESIAN_POINT('Ctrl Pts',(-3.67626940318832,-3.80210265806849,
24.9193408898533));
#47203=CARTESIAN_POINT('Ctrl Pts',(-1.40999024783327,-5.09733938916421,
24.9987127799067));
#47204=CARTESIAN_POINT('Ctrl Pts',(1.19975941093347,-5.1508755278289,25.0780846699601));
#47205=CARTESIAN_POINT('Ctrl Pts',(3.51725033281924,-3.94966978918403,25.1574565600135));
#47206=CARTESIAN_POINT('Ctrl Pts',(4.97794685893178,-1.7863332323397,25.2368284500669));
#47207=CARTESIAN_POINT('Ctrl Pts',(5.226026548707,0.812150145920977,25.3162003401203));
#47208=CARTESIAN_POINT('Ctrl Pts',(4.20105773883081,3.21279554629917,25.3955722301737));
#47209=CARTESIAN_POINT('Ctrl Pts',(2.15272056265901,4.83081106300121,25.4749441202272));
#47210=CARTESIAN_POINT('Ctrl Pts',(-0.420014577610356,5.27205169757513,
25.5543160102805));
#47211=CARTESIAN_POINT('Ctrl Pts',(-2.89043509646038,4.42903220810823,25.6336879003339));
#47212=CARTESIAN_POINT('Ctrl Pts',(-4.65675202368223,2.50711027624266,25.7130597903873));
#47213=CARTESIAN_POINT('Ctrl Pts',(-5.28869446548081,-0.0255381695211706,
25.7924316804408));
#47214=CARTESIAN_POINT('Ctrl Pts',(-4.63232264181493,-2.55196557371741,
25.8718035704942));
#47215=CARTESIAN_POINT('Ctrl Pts',(-2.84752727607513,-4.45673981283608,
25.9511754605475));
#47216=CARTESIAN_POINT('Ctrl Pts',(-0.369080568778156,-5.27586209837409,
26.030547350601));
#47217=CARTESIAN_POINT('Ctrl Pts',(2.19927334812716,-4.80979605467087,26.1099192406543));
#47218=CARTESIAN_POINT('Ctrl Pts',(4.23188914543768,-3.17207433835284,26.1892911307078));
#47219=CARTESIAN_POINT('Ctrl Pts',(5.23362611404738,-0.761642334479479,
26.2686630207611));
#47220=CARTESIAN_POINT('Ctrl Pts',(4.96046334571002,1.83432405620638,26.3480349108146));
#47221=CARTESIAN_POINT('Ctrl Pts',(3.47894268615705,3.98345316700778,26.427406800868));
#47222=CARTESIAN_POINT('Ctrl Pts',(1.14995928876529,5.16222190355009,26.5067786909214));
#47223=CARTESIAN_POINT('Ctrl Pts',(-1.45915164597797,5.08348481077201,26.5861505809748));
#47224=CARTESIAN_POINT('Ctrl Pts',(-3.71281646953845,3.76642207019263,26.6655224710282));
#47225=CARTESIAN_POINT('Ctrl Pts',(-5.06204741929919,1.53186725014815,26.7448943610816));
#47226=CARTESIAN_POINT('Ctrl Pts',(-5.17817482237054,-1.07584704130177,
26.824266251135));
#47227=CARTESIAN_POINT('Ctrl Pts',(-4.032910300408,-3.42148737483758,26.9036381411884));
#47228=CARTESIAN_POINT('Ctrl Pts',(-1.90523775596165,-4.93366095719681,
26.9830100312419));
#47229=CARTESIAN_POINT('Ctrl Pts',(0.686546488664775,-5.24400565085624,
27.0623819212952));
#47230=CARTESIAN_POINT('Ctrl Pts',(3.11108952829732,-4.27692217537667,27.1417538113486));
#47231=CARTESIAN_POINT('Ctrl Pts',(4.77777804511651,-2.267989924782,27.221125701402));
#47232=CARTESIAN_POINT('Ctrl Pts',(5.28061040557762,0.293419651379019,27.3004975914554));
#47233=CARTESIAN_POINT('Ctrl Pts',(4.49709775967288,2.7833528499375,27.3798694815089));
#47234=CARTESIAN_POINT('Ctrl Pts',(2.61810205366886,4.59526745509821,27.4592413715622));
#47235=CARTESIAN_POINT('Ctrl Pts',(0.101342482461748,5.28778507964899,27.5386132616156));
#47236=CARTESIAN_POINT('Ctrl Pts',(-2.44010389315526,4.69220996311103,27.617985151669));
#47237=CARTESIAN_POINT('Ctrl Pts',(-4.38714636147802,2.95362288558985,27.6973570417224));
#47238=CARTESIAN_POINT('Ctrl Pts',(-5.26548968692851,0.495539810872365,
27.7767289317758));
#47239=CARTESIAN_POINT('Ctrl Pts',(-4.86117137960698,-2.08325566491491,
27.8561008218293));
#47240=CARTESIAN_POINT('Ctrl Pts',(-3.27268248423349,-4.15457467193712,
27.9354727118826));
#47241=CARTESIAN_POINT('Ctrl Pts',(-0.886975379660524,-5.21384848487045,
28.0148446019361));
#47242=CARTESIAN_POINT('Ctrl Pts',(1.71479696411104,-5.00304034754724,28.0942164919895));
#47243=CARTESIAN_POINT('Ctrl Pts',(3.89884856306386,-3.57350265560346,28.1735883820429));
#47244=CARTESIAN_POINT('Ctrl Pts',(5.1331492820092,-1.27346762656861,28.2529602720963));
#47245=CARTESIAN_POINT('Ctrl Pts',(5.11702619789033,1.3367812975255,28.3323321621497));
#47246=CARTESIAN_POINT('Ctrl Pts',(3.85440685831077,3.62139325645763,28.4117040522031));
#47247=CARTESIAN_POINT('Ctrl Pts',(1.6528625396316,5.02384183393471,28.4910759422564));
#47248=CARTESIAN_POINT('Ctrl Pts',(-0.951315435152638,5.20249366075061,
28.5704478323099));
#47249=CARTESIAN_POINT('Ctrl Pts',(-3.32375507563475,4.11382954733206,28.6498197223633));
#47250=CARTESIAN_POINT('Ctrl Pts',(-4.8865353366993,2.02304566199065,28.7291916124167));
#47251=CARTESIAN_POINT('Ctrl Pts',(-5.25896640590637,-0.560547668676075,
28.8085635024701));
#47252=CARTESIAN_POINT('Ctrl Pts',(-4.35032489915935,-3.00759282800452,
28.8879353925235));
#47253=CARTESIAN_POINT('Ctrl Pts',(-2.38195387625792,-4.72199503162487,
28.9673072825769));
#47254=CARTESIAN_POINT('Ctrl Pts',(0.166655838534471,-5.28612969750008,
29.0466791726303));
#47255=CARTESIAN_POINT('Ctrl Pts',(2.67466855994625,-4.56257486971391,29.1260510626837));
#47256=CARTESIAN_POINT('Ctrl Pts',(4.53113794043359,-2.72758690275364,29.2054229527372));
#47257=CARTESIAN_POINT('Ctrl Pts',(5.28383214813505,-0.228164803693758,
29.2847948427905));
#47258=CARTESIAN_POINT('Ctrl Pts',(4.74939654011487,2.32683773651173,29.3641667328439));
#47259=CARTESIAN_POINT('Ctrl Pts',(3.05801844753361,4.31502775447088,29.4435386228973));
#47260=CARTESIAN_POINT('Ctrl Pts',(0.621713829942241,5.25208656259286,29.5229105129507));
#47261=CARTESIAN_POINT('Ctrl Pts',(-1.96603890048284,4.90974870936366,29.6022824030042));
#47262=CARTESIAN_POINT('Ctrl Pts',(-4.07486890650364,3.37140693807791,29.6816542930575));
#47263=CARTESIAN_POINT('Ctrl Pts',(-5.19106986646947,1.01179789915904,29.7610261831109));
#47264=CARTESIAN_POINT('Ctrl Pts',(-5.04273769720158,-1.59428286841832,
29.8403980731643));
#47265=CARTESIAN_POINT('Ctrl Pts',(-3.66600578680595,-3.81199985813419,
29.9197699632177));
#47266=CARTESIAN_POINT('Ctrl Pts',(-1.39624298131062,-5.10112212012718,
29.9991418532712));
#47267=CARTESIAN_POINT('Ctrl Pts',(1.21364152390063,-5.1476223247995,30.0785137433246));
#47268=CARTESIAN_POINT('Ctrl Pts',(3.52788564023963,-3.94017312521939,30.157885633378));
#47269=CARTESIAN_POINT('Ctrl Pts',(4.98274462345863,-1.7729064737611,30.2372575234313));
#47270=CARTESIAN_POINT('Ctrl Pts',(5.22381804552127,0.826236270443475,30.3166294134848));
#47271=CARTESIAN_POINT('Ctrl Pts',(4.19238095442003,3.22410968801099,30.3960013035382));
#47272=CARTESIAN_POINT('Ctrl Pts',(2.13968914249988,4.83659712202475,30.4753731935916));
#47273=CARTESIAN_POINT('Ctrl Pts',(-0.434226208411599,5.27090020273941,
30.554745083645));
#47274=CARTESIAN_POINT('Ctrl Pts',(-2.90236501609743,4.4212236610065,30.6341169736984));
#47275=CARTESIAN_POINT('Ctrl Pts',(-4.66349413013793,2.49454682166501,30.7134888637518));
#47276=CARTESIAN_POINT('Ctrl Pts',(-5.28860639654603,-0.0397961018483339,
30.7928607538052));
#47277=CARTESIAN_POINT('Ctrl Pts',(-4.62542585088724,-2.56444478303865,
30.8722326438586));
#47278=CARTESIAN_POINT('Ctrl Pts',(-2.83550180615875,-4.46440039138299,
30.951604533912));
#47279=CARTESIAN_POINT('Ctrl Pts',(-0.354855797726762,-5.27683794616905,
31.0309764239654));
#47280=CARTESIAN_POINT('Ctrl Pts',(2.21223229757146,-4.80384945735102,31.1103483140188));
#47281=CARTESIAN_POINT('Ctrl Pts',(4.24042550187443,-3.16065387386267,31.1897202040722));
#47282=CARTESIAN_POINT('Ctrl Pts',(5.23566043994338,-0.747530002690045,
31.2690920941256));
#47283=CARTESIAN_POINT('Ctrl Pts',(4.95550008377996,1.84769052250822,31.348463984179));
#47284=CARTESIAN_POINT('Ctrl Pts',(3.46819087602115,3.99281772621712,31.4278358742324));
#47285=CARTESIAN_POINT('Ctrl Pts',(1.13603804757386,5.16530336977167,31.5072077642858));
#47286=CARTESIAN_POINT('Ctrl Pts',(-1.47285113468488,5.07953254565492,31.5865796543392));
#47287=CARTESIAN_POINT('Ctrl Pts',(-3.72295704063504,3.75639883677117,31.6659515443926));
#47288=CARTESIAN_POINT('Ctrl Pts',(-5.06615885211213,1.51821468589782,31.745323434446));
#47289=CARTESIAN_POINT('Ctrl Pts',(-5.17525558096714,-1.08980320194903,
31.8246953244994));
#47290=CARTESIAN_POINT('Ctrl Pts',(-4.02367150553249,-3.43234744203962,
31.9040672145529));
#47291=CARTESIAN_POINT('Ctrl Pts',(-1.89192995759591,-4.93877944262154,
31.9834391046062));
#47292=CARTESIAN_POINT('Ctrl Pts',(0.70068154029511,-5.24213570278371,32.0628109946597));
#47293=CARTESIAN_POINT('Ctrl Pts',(3.12260856590247,-4.26851930901834,32.142182884713));
#47294=CARTESIAN_POINT('Ctrl Pts',(4.78387505663285,-2.25510105978337,32.2215547747665));
#47295=CARTESIAN_POINT('Ctrl Pts',(5.27980017249531,0.307654816033343,32.3009266648198));
#47296=CARTESIAN_POINT('Ctrl Pts',(4.48957765297736,2.79546665964672,32.3802985548733));
#47297=CARTESIAN_POINT('Ctrl Pts',(2.60570395470567,4.60230901263064,32.4596704449267));
#47298=CARTESIAN_POINT('Ctrl Pts',(0.0870865406955613,5.28803907717593,
32.5390423349801));
#47299=CARTESIAN_POINT('Ctrl Pts',(-2.45274496186521,4.68561452739711,32.6184142250335));
#47300=CARTESIAN_POINT('Ctrl Pts',(-4.39509322077448,2.94178465017617,32.6977861150869));
#47301=CARTESIAN_POINT('Ctrl Pts',(-5.26680649947691,0.48134254370224,32.7771580051403));
#47302=CARTESIAN_POINT('Ctrl Pts',(-4.85553737278523,-2.09635354098391,
32.8565298951937));
#47303=CARTESIAN_POINT('Ctrl Pts',(-3.26147008963279,-4.16338254328624,
32.9359017852471));
#47304=CARTESIAN_POINT('Ctrl Pts',(-0.8729159117874,-5.21622077353502,33.0152736753005));
#47305=CARTESIAN_POINT('Ctrl Pts',(1.72827865000283,-4.99839916925953,33.0946455653539));
#47306=CARTESIAN_POINT('Ctrl Pts',(3.9084683581323,-3.5629785911213,33.1740174554073));
#47307=CARTESIAN_POINT('Ctrl Pts',(5.13656382546866,-1.25962431470524,33.2533893454607));
#47308=CARTESIAN_POINT('Ctrl Pts',(5.11340371451205,1.35057165664188,33.3327612355141));
#47309=CARTESIAN_POINT('Ctrl Pts',(3.84462977702742,3.63177136187071,33.4121331255675));
#47310=CARTESIAN_POINT('Ctrl Pts',(1.63931253580255,5.02827960213734,33.4915050156209));
#47311=CARTESIAN_POINT('Ctrl Pts',(-0.965337610587002,5.19991006123145,
33.5708769056743));
#47312=CARTESIAN_POINT('Ctrl Pts',(-3.33483365177614,4.1048539392153,33.6502487957277));
#47313=CARTESIAN_POINT('Ctrl Pts',(-4.89197159692173,2.00986448354636,33.7296206857811));
#47314=CARTESIAN_POINT('Ctrl Pts',(-5.25743608925264,-0.574723511554913,
33.8089925758345));
#47315=CARTESIAN_POINT('Ctrl Pts',(-4.34220078737896,-3.01931013137032,
33.888364465888));
#47316=CARTESIAN_POINT('Ctrl Pts',(-2.36921498499824,-4.72839948631349,
33.9677363559413));
#47317=CARTESIAN_POINT('Ctrl Pts',(0.18090634355963,-5.28566119252548,34.0471082459947));
#47318=CARTESIAN_POINT('Ctrl Pts',(2.68695928725581,-4.55534753185087,34.1264801360481));
#47319=CARTESIAN_POINT('Ctrl Pts',(4.53847489605999,-2.71536129550809,34.2058520261016));
#47320=CARTESIAN_POINT('Ctrl Pts',(5.28442806592769,-0.21391905792982,34.2852239161549));
#47321=CARTESIAN_POINT('Ctrl Pts',(4.74310625581857,2.3396333886583,34.3645958062084));
#47322=CARTESIAN_POINT('Ctrl Pts',(3.04637426047967,4.32325632045994,34.4439676962618));
#47323=CARTESIAN_POINT('Ctrl Pts',(0.607552238322964,5.25374358196314,34.5233395863151));
#47324=CARTESIAN_POINT('Ctrl Pts',(-1.97926816429518,4.90443053586424,34.6027114763686));
#47325=CARTESIAN_POINT('Ctrl Pts',(-4.08394322312674,3.36040906700167,34.6820833664219));
#47326=CARTESIAN_POINT('Ctrl Pts',(-5.19377875245966,0.997799387556786,
34.7614552564754));
#47327=CARTESIAN_POINT('Ctrl Pts',(-5.03842127392763,-1.60787201410546,
34.8408271465287));
#47328=CARTESIAN_POINT('Ctrl Pts',(-3.65571552542313,-3.82186935209593,
34.9201990365822));
#47329=CARTESIAN_POINT('Ctrl Pts',(-1.38248556671468,-5.10486777548014,
34.9995709266355));
#47330=CARTESIAN_POINT('Ctrl Pts',(1.22751481596557,-5.14433170819057,35.078942816689));
#47331=CARTESIAN_POINT('Ctrl Pts',(3.53849530653457,-3.93064782357091,35.1583147067423));
#47332=CARTESIAN_POINT('Ctrl Pts',(4.98750617275828,-1.75946682947078,35.2376865967958));
#47333=CARTESIAN_POINT('Ctrl Pts',(5.22157157495577,0.840316389774704,35.3170584868492));
#47334=CARTESIAN_POINT('Ctrl Pts',(4.18367369924664,3.23540039647985,35.3964303769026));
#47335=CARTESIAN_POINT('Ctrl Pts',(2.12664217080567,4.8423480280398,35.4758022669559));
#47336=CARTESIAN_POINT('Ctrl Pts',(-0.448434683200953,5.2697103983248,35.5551741570095));
#47337=CARTESIAN_POINT('Ctrl Pts',(-2.91427384097317,4.41338297988397,35.6345460470627));
#47338=CARTESIAN_POINT('Ctrl Pts',(-4.67020234172003,2.48196523640092,35.7139179371163));
#47339=CARTESIAN_POINT('Ctrl Pts',(-5.28847988934142,-0.0540537449324728,
35.7932898271696));
#47340=CARTESIAN_POINT('Ctrl Pts',(-4.61849544177097,-2.57690535364626,
35.872661717223));
#47341=CARTESIAN_POINT('Ctrl Pts',(-2.82345572745135,-4.47202852209511,
35.9520336072764));
#47342=CARTESIAN_POINT('Ctrl Pts',(-0.340628447537815,-5.27777544122882,
36.0314054973298));
#47343=CARTESIAN_POINT('Ctrl Pts',(2.22517516822766,-4.79786794503694,36.1107773873833));
#47344=CARTESIAN_POINT('Ctrl Pts',(4.2489310383545,-3.14921043733466,36.1901492774366));
#47345=CARTESIAN_POINT('Ctrl Pts',(5.23765671238758,-0.733412237756749,
36.2695211674901));
#47346=CARTESIAN_POINT('Ctrl Pts',(4.95050080463952,1.8610435595583,36.3488930575434));
#47347=CARTESIAN_POINT('Ctrl Pts',(3.45741385862894,4.002153265115,36.4282649475969));
#47348=CARTESIAN_POINT('Ctrl Pts',(1.12210854951209,5.16834729390565,36.5076368376502));
#47349=CARTESIAN_POINT('Ctrl Pts',(-1.4865399185207,5.07554336184357,36.5870087277037));
#47350=CARTESIAN_POINT('Ctrl Pts',(-3.73307055280216,3.74634830136112,36.666380617757));
#47351=CARTESIAN_POINT('Ctrl Pts',(-5.07023346343257,1.50455108706837,36.7457525078105));
#47352=CARTESIAN_POINT('Ctrl Pts',(-5.17229872514219,-1.10375144176689,
36.8251243978638));
#47353=CARTESIAN_POINT('Ctrl Pts',(-4.01440346609619,-3.44318256250012,
36.9044962879173));
#47354=CARTESIAN_POINT('Ctrl Pts',(-1.87860840844056,-4.94386203236358,
36.9838681779707));
#47355=CARTESIAN_POINT('Ctrl Pts',(0.71481149928202,-5.24022765419639,37.0632400680241));
#47356=CARTESIAN_POINT('Ctrl Pts',(3.13410490798792,-4.26008541851396,37.1426119580775));
#47357=CARTESIAN_POINT('Ctrl Pts',(4.78993729833158,-2.24219580442096,37.2219838481309));
#47358=CARTESIAN_POINT('Ctrl Pts',(5.27895156514787,0.321887744613352,37.3013557381843));
#47359=CARTESIAN_POINT('Ctrl Pts',(4.48202491545551,2.80756015154514,37.3807276282377));
#47360=CARTESIAN_POINT('Ctrl Pts',(2.59328691715162,4.6093171199916,37.4600995182911));
#47361=CARTESIAN_POINT('Ctrl Pts',(0.0728299659736646,5.28825464055466,
37.5394714083445));
#47362=CARTESIAN_POINT('Ctrl Pts',(-2.46536820371075,4.67898503603898,37.6188432983979));
#47363=CARTESIAN_POINT('Ctrl Pts',(-4.40300813596802,2.92992503348812,37.6982151884513));
#47364=CARTESIAN_POINT('Ctrl Pts',(-5.26808503220261,0.467141778084607,
37.7775870785047));
#47365=CARTESIAN_POINT('Ctrl Pts',(-4.84986807528987,-2.10943618050861,
37.8569589685581));
#47366=CARTESIAN_POINT('Ctrl Pts',(-3.2502339902585,-4.17216015459505,37.9363308586115));
#47367=CARTESIAN_POINT('Ctrl Pts',(-0.858850099431265,-5.21855515011692,
38.0157027486649));
#47368=CARTESIAN_POINT('Ctrl Pts',(1.74174777450972,-4.99372166181591,38.0950746387183));
#47369=CARTESIAN_POINT('Ctrl Pts',(3.91805974601555,-3.55242863073569,38.1744465287717));
#47370=CARTESIAN_POINT('Ctrl Pts',(5.13994103560184,-1.24577184719802,38.2538184188251));
#47371=CARTESIAN_POINT('Ctrl Pts',(5.10974406648872,1.36435219862427,38.3331903088785));
#47372=CARTESIAN_POINT('Ctrl Pts',(3.83482475204887,3.64212307300276,38.4125621989319));
#47373=CARTESIAN_POINT('Ctrl Pts',(1.62575061805696,5.03268082057242,38.4919340889853));
#47374=CARTESIAN_POINT('Ctrl Pts',(-0.979352771366501,5.19728867487039,
38.5713059790387));
#47375=CARTESIAN_POINT('Ctrl Pts',(-3.3458879870052,4.09584848370752,38.6506778690921));
#47376=CARTESIAN_POINT('Ctrl Pts',(-4.89737230716795,1.99666872129193,38.7300497591456));
#47377=CARTESIAN_POINT('Ctrl Pts',(-5.2558675504918,-0.588895222855594,
38.809421649199));
#47378=CARTESIAN_POINT('Ctrl Pts',(-4.33404513553914,-3.03100540392653,
38.8887935392523));
#47379=CARTESIAN_POINT('Ctrl Pts',(-2.35645883694701,-4.73476973691708,
38.9681654293058));
#47380=CARTESIAN_POINT('Ctrl Pts',(0.195155463808245,-5.28515396379923,
39.0475373193592));
#47381=CARTESIAN_POINT('Ctrl Pts',(2.69923061743519,-4.54808766460433,39.1269092094126));
#47382=CARTESIAN_POINT('Ctrl Pts',(4.5457786161602,-2.70311485851688,39.2062810994659));
#47383=CARTESIAN_POINT('Ctrl Pts',(5.28498604656423,-0.199673823356607,
39.2856529895194));
#47384=CARTESIAN_POINT('Ctrl Pts',(4.73678060915317,2.35241593705468,39.3650248795727));
#47385=CARTESIAN_POINT('Ctrl Pts',(3.03470961035893,4.33144609848054,39.4443967696262));
#47386=CARTESIAN_POINT('Ctrl Pts',(0.593383061700927,5.25537632570972,39.5237686596795));
#47387=CARTESIAN_POINT('Ctrl Pts',(-1.99247705733066,4.8990504464678,39.603140549733));
#47388=CARTESIAN_POINT('Ctrl Pts',(-4.09299916691649,3.34943642687039,39.6825124397864));
#47389=CARTESIAN_POINT('Ctrl Pts',(-5.19642846461573,0.983699440459269,
39.7618843298398));
#47390=CARTESIAN_POINT('Ctrl Pts',(-5.03410925482033,-1.62126816458454,
39.8412562198932));
#47391=CARTESIAN_POINT('Ctrl Pts',(-3.6453165085118,-3.83208153227987,39.9206281099466));
#47392=CARTESIAN_POINT('Ctrl Pts',(-2.12771778283764,-4.68247622999901,
39.9735427033155));
#47393=CARTESIAN_POINT('Ctrl Pts',(-1.31303618635638,-4.90075024188325,
40.));
#47394=CARTESIAN_POINT('Ctrl Pts',(-3.43378788736187,2.93584158412999,-1.38777878078145E-15));
#47395=CARTESIAN_POINT('Ctrl Pts',(-3.5274298169339,2.83894612463338,-1.38777878078145E-15));
#47396=CARTESIAN_POINT('Ctrl Pts',(-3.61644080326455,2.73799316940158,-1.70682494898246E-15));
#47397=CARTESIAN_POINT('Ctrl Pts',(-3.70070760607863,2.63340714286309,-1.68962066560141E-15));
#47398=CARTESIAN_POINT('Ctrl Pts',(-3.78643913867677,2.52700319677679,-1.67211733650556E-15));
#47399=CARTESIAN_POINT('Ctrl Pts',(-3.86726060843671,2.41683829132909,-1.52825423918462E-15));
#47400=CARTESIAN_POINT('Ctrl Pts',(-3.9430233259709,2.30331415642333,-1.42247325030098E-15));
#47401=CARTESIAN_POINT('Ctrl Pts',(-4.01958942326278,2.18858622372678,-1.31557057111923E-15));
#47402=CARTESIAN_POINT('Ctrl Pts',(-4.09098941448581,2.07042685422507,-1.45703061823736E-15));
#47403=CARTESIAN_POINT('Ctrl Pts',(-4.15703260143776,1.94921318851517,-1.40165656858926E-15));
#47404=CARTESIAN_POINT('Ctrl Pts',(-4.22276474819078,1.82857039656885,-1.34654331125317E-15));
#47405=CARTESIAN_POINT('Ctrl Pts',(-4.28319084758819,1.70490133278768,-1.76868280947178E-15));
#47406=CARTESIAN_POINT('Ctrl Pts',(-4.33807945470206,1.57855051046471,-1.88044024795886E-15));
#47407=CARTESIAN_POINT('Ctrl Pts',(-4.35502796120398,1.53953589802935,-1.91494871469599E-15));
#47408=CARTESIAN_POINT('Ctrl Pts',(-4.37144815676901,1.50026543549027,-1.30689270547165E-15));
#47409=CARTESIAN_POINT('Ctrl Pts',(-4.38733228779962,1.46074889051522,-1.32532873564628E-15));
#47410=CARTESIAN_POINT('Ctrl Pts',(-4.39376253093777,1.44475173009898,-1.33279204328941E-15));
#47411=CARTESIAN_POINT('Ctrl Pts',(-4.40010357988131,1.42871748389362,-1.28259685789569E-15));
#47412=CARTESIAN_POINT('Ctrl Pts',(-4.4063520165592,1.41265478977856,-1.29063426612674E-15));
#47413=CARTESIAN_POINT('Ctrl Pts',(-4.45729152748394,1.28170591015729,-1.35615811881152E-15));
#47414=CARTESIAN_POINT('Ctrl Pts',(-4.50214144181921,1.14871482526442,-2.13815754900839E-15));
#47415=CARTESIAN_POINT('Ctrl Pts',(-4.54074327371246,1.0140904790896,-2.05391259555654E-15));
#47416=CARTESIAN_POINT('Ctrl Pts',(-4.54547345988333,0.997593898764086,
-2.0435893985931E-15));
#47417=CARTESIAN_POINT('Ctrl Pts',(-4.55010977859188,0.981072752949281,
-1.00791691148873E-15));
#47418=CARTESIAN_POINT('Ctrl Pts',(-4.55465189605181,0.964527761093366,
-1.01307850997046E-15));
#47419=CARTESIAN_POINT('Ctrl Pts',(-4.59134817932549,0.830858891175244,
-1.05169067743968E-15));
#47420=CARTESIAN_POINT('Ctrl Pts',(-4.62189967399316,0.695635489793831,
-1.41485248297211E-15));
#47421=CARTESIAN_POINT('Ctrl Pts',(-4.64637428491341,0.559286455771474,
-1.36002320516582E-15));
#47422=CARTESIAN_POINT('Ctrl Pts',(-4.67110897469857,0.42148851201501,-1.30461128535625E-15));
#47423=CARTESIAN_POINT('Ctrl Pts',(-4.68963709540601,0.282540149701787,
-1.43104411647104E-15));
#47424=CARTESIAN_POINT('Ctrl Pts',(-4.70197867697062,0.142866308633218,
-1.36002320516582E-15));
#47425=CARTESIAN_POINT('Ctrl Pts',(-4.71314718957453,0.0164684846393732,
-1.29575284087739E-15));
#47426=CARTESIAN_POINT('Ctrl Pts',(-4.71924875509872,-0.110524098082,-1.66579323769632E-15));
#47427=CARTESIAN_POINT('Ctrl Pts',(-4.72026194547141,-0.237801095913712,
-1.67921232474555E-15));
#47428=CARTESIAN_POINT('Ctrl Pts',(-4.72045200129662,-0.261675913030809,
-1.68172949795545E-15));
#47429=CARTESIAN_POINT('Ctrl Pts',(-4.72046291446759,-0.285560737563283,
-9.9370225703457E-16));
#47430=CARTESIAN_POINT('Ctrl Pts',(-4.72029440609211,-0.309453515786201,
-9.71445146547012E-16));
#47431=CARTESIAN_POINT('Ctrl Pts',(-4.72016631155934,-0.327616021086772,
-9.54526022139039E-16));
#47432=CARTESIAN_POINT('Ctrl Pts',(-4.7199344986873,-0.345781850732525,
-1.1165476318937E-15));
#47433=CARTESIAN_POINT('Ctrl Pts',(-4.7195992402228,-0.363937763232007,
-1.12410081243297E-15));
#47434=CARTESIAN_POINT('Ctrl Pts',(-4.7169715342115,-0.506241106673104,
-1.18330151878048E-15));
#47435=CARTESIAN_POINT('Ctrl Pts',(-4.70799214533038,-0.648137600560786,
-1.67849620506959E-15));
#47436=CARTESIAN_POINT('Ctrl Pts',(-4.69273559502703,-0.789185289486343,
-1.60982338570648E-15));
#47437=CARTESIAN_POINT('Ctrl Pts',(-4.67736001919945,-0.931333376259461,
-1.5406148083796E-15));
#47438=CARTESIAN_POINT('Ctrl Pts',(-4.65560906635571,-1.07262015451611,
-1.29947818212301E-15));
#47439=CARTESIAN_POINT('Ctrl Pts',(-4.62750766548139,-1.21260443247969,
-1.38777878078145E-15));
#47440=CARTESIAN_POINT('Ctrl Pts',(-4.61688292082861,-1.26553052023664,
-1.42116399590398E-15));
#47441=CARTESIAN_POINT('Ctrl Pts',(-4.60534985624838,-1.31827046839259,
-1.10373700911438E-15));
#47442=CARTESIAN_POINT('Ctrl Pts',(-4.59290787692679,-1.37080047994465,
-1.0547118733939E-15));
#47443=CARTESIAN_POINT('Ctrl Pts',(-4.56011975477607,-1.50923186540429,
-9.25516823562078E-16));
#47444=CARTESIAN_POINT('Ctrl Pts',(-4.52102317103095,-1.64620611480812,
-1.41788356490645E-15));
#47445=CARTESIAN_POINT('Ctrl Pts',(-4.47583839059365,-1.78136570298785,
-1.36002320516582E-15));
#47446=CARTESIAN_POINT('Ctrl Pts',(-4.44941052359499,-1.86041841908909,
-1.32618159130998E-15));
#47447=CARTESIAN_POINT('Ctrl Pts',(-4.42089896739826,-1.93885019183042,
-1.30868430769761E-15));
#47448=CARTESIAN_POINT('Ctrl Pts',(-4.3903399301827,-2.01658705378289,-1.30451205393456E-15));
#47449=CARTESIAN_POINT('Ctrl Pts',(-4.37718466105246,-2.05005176450371,
-1.30271595280921E-15));
#47450=CARTESIAN_POINT('Ctrl Pts',(-4.36364988420426,-2.08338766611273,
-1.16152748166208E-15));
#47451=CARTESIAN_POINT('Ctrl Pts',(-4.3497381750326,-2.11658871139626,-1.13797860024079E-15));
#47452=CARTESIAN_POINT('Ctrl Pts',(-4.34244585283277,-2.13399223217085,
-1.12563460794976E-15));
#47453=CARTESIAN_POINT('Ctrl Pts',(-4.33504992528714,-2.15135862906508,
-1.92978013206096E-15));
#47454=CARTESIAN_POINT('Ctrl Pts',(-4.32755662758879,-2.16867384922929,
-1.9151347174784E-15));
#47455=CARTESIAN_POINT('Ctrl Pts',(-4.2701680431329,-2.30128515265925,-1.80297053483165E-15));
#47456=CARTESIAN_POINT('Ctrl Pts',(-4.20699158680529,-2.43109046195038,
-1.71043044263751E-15));
#47457=CARTESIAN_POINT('Ctrl Pts',(-4.13831811099888,-2.55774085897211,
-1.72084568816899E-15));
#47458=CARTESIAN_POINT('Ctrl Pts',(-4.0690864175418,-2.68542074352523,-1.73134559482798E-15));
#47459=CARTESIAN_POINT('Ctrl Pts',(-3.99426770892291,-2.80989493979695,
-1.80815084065395E-15));
#47460=CARTESIAN_POINT('Ctrl Pts',(-3.91410750939009,-2.93079631633735,
-1.80411241501588E-15));
#47461=CARTESIAN_POINT('Ctrl Pts',(-3.83416065570548,-3.05137591465264,
-1.8000847376213E-15));
#47462=CARTESIAN_POINT('Ctrl Pts',(-3.74890035710146,-3.16840239753955,
-1.26386791065628E-15));
#47463=CARTESIAN_POINT('Ctrl Pts',(-3.6585229556131,-3.28149127673775,-1.27675647831893E-15));
#47464=CARTESIAN_POINT('Ctrl Pts',(-3.59945026249498,-3.35540870018578,
-1.2851807347119E-15));
#47465=CARTESIAN_POINT('Ctrl Pts',(-3.5381904788592,-3.42764345712454,-1.45186396209174E-15));
#47466=CARTESIAN_POINT('Ctrl Pts',(-3.47478854700661,-3.49808125449704,
-1.41553435639707E-15));
#47467=CARTESIAN_POINT('Ctrl Pts',(-3.4391425896078,-3.5376829298883,-1.39540507371065E-15));
#47468=CARTESIAN_POINT('Ctrl Pts',(-3.40281937333393,-3.57671648450509,
-1.55816047969468E-15));
#47469=CARTESIAN_POINT('Ctrl Pts',(-3.36583573983685,-3.61517046963578,
-1.55431223447522E-15));
#47470=CARTESIAN_POINT('Ctrl Pts',(-3.34056943595204,-3.64144128139824,
-1.55168320849956E-15));
#47471=CARTESIAN_POINT('Ctrl Pts',(-3.31499488246685,-3.66744157776442,
-1.71311115652187E-15));
#47472=CARTESIAN_POINT('Ctrl Pts',(-3.28911728144163,-3.6931675174981,-1.69309011255336E-15));
#47473=CARTESIAN_POINT('Ctrl Pts',(-3.27259035745335,-3.70959758186502,
-1.68030352265613E-15));
#47474=CARTESIAN_POINT('Ctrl Pts',(-3.25594506354961,-3.7259104717157,-1.35072386705874E-15));
#47475=CARTESIAN_POINT('Ctrl Pts',(-3.23918904311522,-3.74209965697934,
-1.36002320516582E-15));
#47476=CARTESIAN_POINT('Ctrl Pts',(-3.13422859724164,-3.84350942251737,
-1.41827466635674E-15));
#47477=CARTESIAN_POINT('Ctrl Pts',(-3.02485537861799,-3.94013896638234,
-1.29586046630586E-15));
#47478=CARTESIAN_POINT('Ctrl Pts',(-2.91147703861897,-4.03180594754837,
-1.33226762955019E-15));
#47479=CARTESIAN_POINT('Ctrl Pts',(-2.80007805253152,-4.12187261071949,
-1.36803919819172E-15));
#47480=CARTESIAN_POINT('Ctrl Pts',(-2.68481190070853,-4.20714879945784,
-1.75330405072015E-15));
#47481=CARTESIAN_POINT('Ctrl Pts',(-2.5660285220091,-4.28743071443088,-1.77635683940025E-15));
#47482=CARTESIAN_POINT('Ctrl Pts',(-2.51557747120272,-4.32152897813987,
-1.78614808650622E-15));
#47483=CARTESIAN_POINT('Ctrl Pts',(-2.46449152304015,-4.35472587736193,
-1.31186991621621E-15));
#47484=CARTESIAN_POINT('Ctrl Pts',(-2.41279587231268,-4.38700384624999,
-1.27675647831893E-15));
#47485=CARTESIAN_POINT('Ctrl Pts',(-2.38543234505614,-4.40408921163422,
-1.2581702432788E-15));
#47486=CARTESIAN_POINT('Ctrl Pts',(-2.35789457340209,-4.42091901104391,
-1.50863034215941E-15));
#47487=CARTESIAN_POINT('Ctrl Pts',(-2.3302097471481,-4.43747675896359,-1.49880108324396E-15));
#47488=CARTESIAN_POINT('Ctrl Pts',(-2.2023530709709,-4.51394531233533,-1.45340667250483E-15));
#47489=CARTESIAN_POINT('Ctrl Pts',(-2.07127177001784,-4.58467311410489,
-7.9672741319199E-16));
#47490=CARTESIAN_POINT('Ctrl Pts',(-1.93736496285559,-4.64944928440847,
-4.9960036108132E-16));
#47491=CARTESIAN_POINT('Ctrl Pts',(-1.80364190208402,-4.71413656910759,
-2.02881025535331E-16));
#47492=CARTESIAN_POINT('Ctrl Pts',(-1.66710043882179,-4.77288900981815,
-3.16087603122754E-17));
#47493=CARTESIAN_POINT('Ctrl Pts',(-1.52810715957136,-4.82545526764581,
-5.55111512312578E-17));
#47494=CARTESIAN_POINT('Ctrl Pts',(-1.49120032503771,-4.83941316683462,
-6.1857944337824E-17));
#47495=CARTESIAN_POINT('Ctrl Pts',(-1.4541204835251,-4.85293465562285,3.75650465851052E-17));
#47496=CARTESIAN_POINT('Ctrl Pts',(-1.41687422066829,-4.86601447289862,
5.55111512312578E-17));
#47497=CARTESIAN_POINT('Ctrl Pts',(-1.38244754401982,-4.87810413251642,
1.27205291019773E-16));
#47498=CARTESIAN_POINT('Ctrl Pts',(-1.3478786871628,-4.88981645711078,2.24269765851654E-16));
#47499=CARTESIAN_POINT('Ctrl Pts',(-1.31317395760259,-4.90115117757553,
2.22044604925031E-16));
#47500=CARTESIAN_POINT('Ctrl Pts',(4.51755838390264,-0.00010457874560596,
1.61258330249198));
#47501=CARTESIAN_POINT('Ctrl Pts',(4.51776153214983,-0.238054206488734,
1.60420146868401));
#47502=CARTESIAN_POINT('Ctrl Pts',(4.49928771368086,-0.475972597056525,
1.59581963487604));
#47503=CARTESIAN_POINT('Ctrl Pts',(4.46186317968569,-0.710871726876144,
1.58743780106807));
#47504=CARTESIAN_POINT('Ctrl Pts',(4.34373246725773,-1.45233190264972,1.5609805043836));
#47505=CARTESIAN_POINT('Ctrl Pts',(4.03678590132105,-2.16370961033161,1.53452320769914));
#47506=CARTESIAN_POINT('Ctrl Pts',(3.57840923518442,-2.75835983566981,1.50806591101467));
#47507=CARTESIAN_POINT('Ctrl Pts',(3.1200325690478,-3.353010061008,1.4816086143302));
#47508=CARTESIAN_POINT('Ctrl Pts',(2.51022580271121,-3.8309328040025,1.45515131764573));
#47509=CARTESIAN_POINT('Ctrl Pts',(1.82326272299592,-4.13391759737134,1.42869402096126));
#47510=CARTESIAN_POINT('Ctrl Pts',(1.13629964328063,-4.43690239074017,1.4022367242768));
#47511=CARTESIAN_POINT('Ctrl Pts',(0.372180250186614,-4.56494923448333,
1.37577942759233));
#47512=CARTESIAN_POINT('Ctrl Pts',(-0.37602655530059,-4.50246217629702,
1.34932213090786));
#47513=CARTESIAN_POINT('Ctrl Pts',(-1.1242333607878,-4.4399751181107,1.32286483422339));
#47514=CARTESIAN_POINT('Ctrl Pts',(-1.85652757866819,-4.18695415799491,
1.29640753753892));
#47515=CARTESIAN_POINT('Ctrl Pts',(-2.48371659230757,-3.77421694705552,
1.26995024085446));
#47516=CARTESIAN_POINT('Ctrl Pts',(-3.11090560594693,-3.36147973611613,
1.24349294416999));
#47517=CARTESIAN_POINT('Ctrl Pts',(-3.63298941534527,-2.78902627435314,
1.21703564748552));
#47518=CARTESIAN_POINT('Ctrl Pts',(-3.98637877398998,-2.12658080103894,
1.19057835080105));
#47519=CARTESIAN_POINT('Ctrl Pts',(-4.3397681326347,-1.46413532772474,1.16412105411659));
#47520=CARTESIAN_POINT('Ctrl Pts',(-4.52446304052578,-0.711697842859317,
1.13766375743212));
#47521=CARTESIAN_POINT('Ctrl Pts',(-4.51796789313228,0.039085678406338,
1.11120646074765));
#47522=CARTESIAN_POINT('Ctrl Pts',(-4.51147274573878,0.789869199671988,
1.08474916406318));
#47523=CARTESIAN_POINT('Ctrl Pts',(-4.3137875430607,1.53899875733787,1.05829186737871));
#47524=CARTESIAN_POINT('Ctrl Pts',(-3.94899006576281,2.19523105353949,1.03183457069425));
#47525=CARTESIAN_POINT('Ctrl Pts',(-3.58419258846491,2.85146334974111,1.00537727400978));
#47526=CARTESIAN_POINT('Ctrl Pts',(-3.0522828365472,3.41479838447846,0.97891997732531));
#47527=CARTESIAN_POINT('Ctrl Pts',(-2.4180469390755,3.81662285121812,0.952462680640842));
#47528=CARTESIAN_POINT('Ctrl Pts',(-1.78381104160379,4.21844731795778,0.926005383956374));
#47529=CARTESIAN_POINT('Ctrl Pts',(-1.0472489985781,4.45876121669975,0.899548087271906));
#47530=CARTESIAN_POINT('Ctrl Pts',(-0.298073044029486,4.50829405706007,
0.873090790587439));
#47531=CARTESIAN_POINT('Ctrl Pts',(0.451102910519128,4.55782689742038,0.846633493902971));
#47532=CARTESIAN_POINT('Ctrl Pts',(1.21289277659066,4.41657867939905,0.820176197218503));
#47533=CARTESIAN_POINT('Ctrl Pts',(1.89451099954032,4.10175426806438,0.793718900534035));
#47534=CARTESIAN_POINT('Ctrl Pts',(2.57612922248998,3.7869298567297,0.767261603849567));
#47535=CARTESIAN_POINT('Ctrl Pts',(3.17757580231775,3.29852925208169,0.740804307165098));
#47536=CARTESIAN_POINT('Ctrl Pts',(3.6255959515189,2.69603724086577,0.71434701048063));
#47537=CARTESIAN_POINT('Ctrl Pts',(4.07361610072004,2.09354522964985,0.687889713796163));
#47538=CARTESIAN_POINT('Ctrl Pts',(4.36820981929455,1.37696181186601,0.661432417111696));
#47539=CARTESIAN_POINT('Ctrl Pts',(4.47349452055126,0.633569578843809,0.634975120427228));
#47540=CARTESIAN_POINT('Ctrl Pts',(4.50319667153093,0.423849191372714,0.627511181115478));
#47541=CARTESIAN_POINT('Ctrl Pts',(4.51783217716753,0.211995155346536,0.620047241803728));
#47542=CARTESIAN_POINT('Ctrl Pts',(4.51763087883895,0.00011359767064345,
0.612583302491977));
#47543=CARTESIAN_POINT('Ctrl Pts',(1.3130361863565,-4.90075024188322,0.));
#47544=CARTESIAN_POINT('Ctrl Pts',(2.12771778283771,-4.68247622999897,0.0264572966844678));
#47545=CARTESIAN_POINT('Ctrl Pts',(3.64531650851188,-3.8320815322798,0.0793718900534037));
#47546=CARTESIAN_POINT('Ctrl Pts',(5.03410925482037,-1.62126816458446,0.158743780106807));
#47547=CARTESIAN_POINT('Ctrl Pts',(5.19642846461569,0.98369944045933,0.238115670160212));
#47548=CARTESIAN_POINT('Ctrl Pts',(4.09299916691648,3.34943642687043,0.317487560213614));
#47549=CARTESIAN_POINT('Ctrl Pts',(1.99247705733062,4.89905044646781,0.396859450267019));
#47550=CARTESIAN_POINT('Ctrl Pts',(-0.593383061700938,5.2553763257097,0.476231340320422));
#47551=CARTESIAN_POINT('Ctrl Pts',(-3.03470961035893,4.33144609848054,0.555603230373826));
#47552=CARTESIAN_POINT('Ctrl Pts',(-4.73678060915323,2.35241593705463,0.634975120427228));
#47553=CARTESIAN_POINT('Ctrl Pts',(-5.28498604656423,-0.199673823356779,
0.714347010480634));
#47554=CARTESIAN_POINT('Ctrl Pts',(-4.5457786161601,-2.703114858517,0.793718900534037));
#47555=CARTESIAN_POINT('Ctrl Pts',(-2.69923061743508,-4.5480876646044,0.87309079058744));
#47556=CARTESIAN_POINT('Ctrl Pts',(-0.195155463808127,-5.28515396379925,
0.952462680640845));
#47557=CARTESIAN_POINT('Ctrl Pts',(2.35645883694709,-4.73476973691702,1.03183457069425));
#47558=CARTESIAN_POINT('Ctrl Pts',(4.33404513553918,-3.03100540392648,1.11120646074765));
#47559=CARTESIAN_POINT('Ctrl Pts',(5.25586755049182,-0.58889522285553,1.19057835080105));
#47560=CARTESIAN_POINT('Ctrl Pts',(4.89737230716791,1.99666872129196,1.26995024085446));
#47561=CARTESIAN_POINT('Ctrl Pts',(3.34588798700519,4.09584848370755,1.34932213090786));
#47562=CARTESIAN_POINT('Ctrl Pts',(0.979352771366438,5.19728867487042,1.42869402096127));
#47563=CARTESIAN_POINT('Ctrl Pts',(-1.6257506180571,5.03268082057239,1.50806591101467));
#47564=CARTESIAN_POINT('Ctrl Pts',(-3.83482475204895,3.64212307300266,1.58743780106807));
#47565=CARTESIAN_POINT('Ctrl Pts',(-5.10974406648874,1.36435219862418,1.66680969112148));
#47566=CARTESIAN_POINT('Ctrl Pts',(-5.13994103560183,-1.2457718471981,1.74618158117488));
#47567=CARTESIAN_POINT('Ctrl Pts',(-3.91805974601548,-3.55242863073578,
1.82555347122828));
#47568=CARTESIAN_POINT('Ctrl Pts',(-1.74174777450957,-4.99372166181597,
1.90492536128169));
#47569=CARTESIAN_POINT('Ctrl Pts',(0.858850099431454,-5.21855515011689,
1.98429725133509));
#47570=CARTESIAN_POINT('Ctrl Pts',(3.25023399025869,-4.17216015459491,2.0636691413885));
#47571=CARTESIAN_POINT('Ctrl Pts',(4.84986807528995,-2.10943618050841,2.1430410314419));
#47572=CARTESIAN_POINT('Ctrl Pts',(5.26808503220259,0.467141778084788,2.22241292149531));
#47573=CARTESIAN_POINT('Ctrl Pts',(4.40300813596794,2.92992503348825,2.3017848115487));
#47574=CARTESIAN_POINT('Ctrl Pts',(2.46536820371062,4.67898503603904,2.38115670160211));
#47575=CARTESIAN_POINT('Ctrl Pts',(-0.0728299659737919,5.28825464055465,
2.46052859165552));
#47576=CARTESIAN_POINT('Ctrl Pts',(-2.59328691715172,4.60931711999155,2.53990048170891));
#47577=CARTESIAN_POINT('Ctrl Pts',(-4.4820249154556,2.80756015154502,2.61927237176233));
#47578=CARTESIAN_POINT('Ctrl Pts',(-5.27895156514789,0.321887744613165,
2.69864426181572));
#47579=CARTESIAN_POINT('Ctrl Pts',(-4.7899372983315,-2.2421958044211,2.77801615186913));
#47580=CARTESIAN_POINT('Ctrl Pts',(-3.13410490798781,-4.26008541851404,
2.85738804192253));
#47581=CARTESIAN_POINT('Ctrl Pts',(-0.714811499281904,-5.2402276541964,
2.93675993197593));
#47582=CARTESIAN_POINT('Ctrl Pts',(1.8786084084407,-4.94386203236353,3.01613182202934));
#47583=CARTESIAN_POINT('Ctrl Pts',(4.01440346609632,-3.44318256249998,3.09550371208274));
#47584=CARTESIAN_POINT('Ctrl Pts',(5.17229872514222,-1.10375144176671,3.17487560213615));
#47585=CARTESIAN_POINT('Ctrl Pts',(5.07023346343252,1.50455108706853,3.25424749218955));
#47586=CARTESIAN_POINT('Ctrl Pts',(3.73307055280206,3.74634830136122,3.33361938224296));
#47587=CARTESIAN_POINT('Ctrl Pts',(1.48653991852054,5.07554336184363,3.41299127229636));
#47588=CARTESIAN_POINT('Ctrl Pts',(-1.12210854951228,5.16834729390561,3.49236316234976));
#47589=CARTESIAN_POINT('Ctrl Pts',(-3.45741385862906,4.00215326511488,3.57173505240317));
#47590=CARTESIAN_POINT('Ctrl Pts',(-4.95050080463958,1.86104355955814,3.65110694245657));
#47591=CARTESIAN_POINT('Ctrl Pts',(-5.23765671238755,-0.733412237756895,
3.73047883250997));
#47592=CARTESIAN_POINT('Ctrl Pts',(-4.24893103835441,-3.14921043733482,
3.80985072256337));
#47593=CARTESIAN_POINT('Ctrl Pts',(-2.22517516822744,-4.79786794503704,
3.88922261261678));
#47594=CARTESIAN_POINT('Ctrl Pts',(0.340628447538026,-5.2777754412288,3.96859450267018));
#47595=CARTESIAN_POINT('Ctrl Pts',(2.82345572745151,-4.472028522095,4.04796639272359));
#47596=CARTESIAN_POINT('Ctrl Pts',(4.61849544177105,-2.57690535364612,4.12733828277699));
#47597=CARTESIAN_POINT('Ctrl Pts',(5.28847988934143,-0.0540537449322821,
4.2067101728304));
#47598=CARTESIAN_POINT('Ctrl Pts',(4.67020234171992,2.48196523640112,4.2860820628838));
#47599=CARTESIAN_POINT('Ctrl Pts',(2.91427384097298,4.41338297988409,4.36545395293721));
#47600=CARTESIAN_POINT('Ctrl Pts',(0.44843468320075,5.26971039832481,4.44482584299061));
#47601=CARTESIAN_POINT('Ctrl Pts',(-2.12664217080585,4.84234802803972,4.52419773304401));
#47602=CARTESIAN_POINT('Ctrl Pts',(-4.18367369924674,3.23540039647972,4.60356962309741));
#47603=CARTESIAN_POINT('Ctrl Pts',(-5.22157157495578,0.840316389774564,
4.68294151315082));
#47604=CARTESIAN_POINT('Ctrl Pts',(-4.98750617275825,-1.75946682947089,
4.76231340320422));
#47605=CARTESIAN_POINT('Ctrl Pts',(-3.53849530653447,-3.93064782357102,
4.84168529325762));
#47606=CARTESIAN_POINT('Ctrl Pts',(-1.22751481596538,-5.14433170819062,
4.92105718331103));
#47607=CARTESIAN_POINT('Ctrl Pts',(1.3824855667149,-5.10486777548008,5.00042907336443));
#47608=CARTESIAN_POINT('Ctrl Pts',(3.65571552542333,-3.82186935209575,5.07980096341784));
#47609=CARTESIAN_POINT('Ctrl Pts',(5.03842127392769,-1.60787201410522,5.15917285347124));
#47610=CARTESIAN_POINT('Ctrl Pts',(5.1937787524596,0.997799387556994,5.23854474352464));
#47611=CARTESIAN_POINT('Ctrl Pts',(4.08394322312664,3.36040906700182,5.31791663357805));
#47612=CARTESIAN_POINT('Ctrl Pts',(1.979268164295,4.90443053586431,5.39728852363145));
#47613=CARTESIAN_POINT('Ctrl Pts',(-0.607552238323124,5.25374358196311,
5.47666041368485));
#47614=CARTESIAN_POINT('Ctrl Pts',(-3.04637426047979,4.32325632045987,5.55603230373826));
#47615=CARTESIAN_POINT('Ctrl Pts',(-4.74310625581864,2.33963338865815,5.63540419379165));
#47616=CARTESIAN_POINT('Ctrl Pts',(-5.28442806592769,-0.213919057930008,
5.71477608384507));
#47617=CARTESIAN_POINT('Ctrl Pts',(-4.53847489605989,-2.71536129550824,
5.79414797389846));
#47618=CARTESIAN_POINT('Ctrl Pts',(-2.68695928725567,-4.55534753185094,
5.87351986395187));
#47619=CARTESIAN_POINT('Ctrl Pts',(-0.180906343559476,-5.28566119252549,
5.95289175400528));
#47620=CARTESIAN_POINT('Ctrl Pts',(2.36921498499841,-4.72839948631341,6.03226364405867));
#47621=CARTESIAN_POINT('Ctrl Pts',(4.3422007873791,-3.01931013137013,6.1116355341121));
#47622=CARTESIAN_POINT('Ctrl Pts',(5.25743608925265,-0.574723511554695,
6.19100742416548));
#47623=CARTESIAN_POINT('Ctrl Pts',(4.89197159692165,2.00986448354653,6.2703793142189));
#47624=CARTESIAN_POINT('Ctrl Pts',(3.33483365177601,4.10485393921541,6.34975120427228));
#47625=CARTESIAN_POINT('Ctrl Pts',(0.96533761058682,5.19991006123149,6.42912309432572));
#47626=CARTESIAN_POINT('Ctrl Pts',(-1.63931253580277,5.02827960213728,6.50849498437909));
#47627=CARTESIAN_POINT('Ctrl Pts',(-3.84462977702757,3.63177136187054,6.58786687443252));
#47628=CARTESIAN_POINT('Ctrl Pts',(-5.11340371451209,1.35057165664169,6.6672387644859));
#47629=CARTESIAN_POINT('Ctrl Pts',(-5.13656382546863,-1.25962431470543,
6.74661065453933));
#47630=CARTESIAN_POINT('Ctrl Pts',(-3.90846835813217,-3.56297859112141,
6.82598254459271));
#47631=CARTESIAN_POINT('Ctrl Pts',(-1.72827865000271,-4.99839916925957,
6.90535443464612));
#47632=CARTESIAN_POINT('Ctrl Pts',(0.872915911787522,-5.21622077353501,
6.98472632469953));
#47633=CARTESIAN_POINT('Ctrl Pts',(3.26147008963291,-4.16338254328616,7.06409821475292));
#47634=CARTESIAN_POINT('Ctrl Pts',(4.85553737278532,-2.09635354098373,7.14347010480633));
#47635=CARTESIAN_POINT('Ctrl Pts',(5.26680649947689,0.481342543702463,7.22284199485974));
#47636=CARTESIAN_POINT('Ctrl Pts',(4.39509322077433,2.9417846501764,7.30221388491313));
#47637=CARTESIAN_POINT('Ctrl Pts',(2.45274496186498,4.68561452739722,7.38158577496654));
#47638=CARTESIAN_POINT('Ctrl Pts',(-0.0870865406957981,5.28803907717593,
7.46095766501995));
#47639=CARTESIAN_POINT('Ctrl Pts',(-2.60570395470586,4.60230901263053,7.54032955507335));
#47640=CARTESIAN_POINT('Ctrl Pts',(-4.48957765297745,2.79546665964655,7.61970144512676));
#47641=CARTESIAN_POINT('Ctrl Pts',(-5.27980017249532,0.307654816033177,
7.69907333518014));
#47642=CARTESIAN_POINT('Ctrl Pts',(-4.78387505663278,-2.25510105978351,
7.77844522523357));
#47643=CARTESIAN_POINT('Ctrl Pts',(-3.12260856590233,-4.26851930901846,
7.85781711528695));
#47644=CARTESIAN_POINT('Ctrl Pts',(-0.70068154029489,-5.24213570278374,
7.93718900534038));
#47645=CARTESIAN_POINT('Ctrl Pts',(1.8919299575961,-4.93877944262147,8.01656089539376));
#47646=CARTESIAN_POINT('Ctrl Pts',(4.02367150553262,-3.43234744203947,8.09593278544719));
#47647=CARTESIAN_POINT('Ctrl Pts',(5.1752555809672,-1.08980320194883,8.17530467550057));
#47648=CARTESIAN_POINT('Ctrl Pts',(5.06615885211206,1.51821468589804,8.25467656555398));
#47649=CARTESIAN_POINT('Ctrl Pts',(3.72295704063487,3.75639883677136,8.33404845560738));
#47650=CARTESIAN_POINT('Ctrl Pts',(1.47285113468463,5.07953254565499,8.41342034566079));
#47651=CARTESIAN_POINT('Ctrl Pts',(-1.1360380475741,5.16530336977162,8.49279223571419));
#47652=CARTESIAN_POINT('Ctrl Pts',(-3.46819087602133,3.99281772621695,8.57216412576759));
#47653=CARTESIAN_POINT('Ctrl Pts',(-4.95550008378004,1.84769052250801,8.651536015821));
#47654=CARTESIAN_POINT('Ctrl Pts',(-5.23566043994335,-0.74753000269027,
8.7309079058744));
#47655=CARTESIAN_POINT('Ctrl Pts',(-4.24042550187429,-3.16065387386283,
8.81027979592781));
#47656=CARTESIAN_POINT('Ctrl Pts',(-2.21223229757129,-4.8038494573511,8.88965168598121));
#47657=CARTESIAN_POINT('Ctrl Pts',(0.354855797726969,-5.27683794616905,
8.96902357603462));
#47658=CARTESIAN_POINT('Ctrl Pts',(2.83550180615889,-4.46440039138287,9.04839546608801));
#47659=CARTESIAN_POINT('Ctrl Pts',(4.6254258508873,-2.56444478303851,9.12776735614143));
#47660=CARTESIAN_POINT('Ctrl Pts',(5.28860639654605,-0.0397961018481786,
9.20713924619482));
#47661=CARTESIAN_POINT('Ctrl Pts',(4.66349413013784,2.49454682166519,9.28651113624823));
#47662=CARTESIAN_POINT('Ctrl Pts',(2.90236501609723,4.42122366100663,9.36588302630163));
#47663=CARTESIAN_POINT('Ctrl Pts',(0.434226208411351,5.27090020273944,9.44525491635504));
#47664=CARTESIAN_POINT('Ctrl Pts',(-2.13968914250016,4.83659712202464,9.52462680640844));
#47665=CARTESIAN_POINT('Ctrl Pts',(-4.1923809544202,3.22410968801074,9.60399869646184));
#47666=CARTESIAN_POINT('Ctrl Pts',(-5.22381804552131,0.826236270443201,
9.68337058651526));
#47667=CARTESIAN_POINT('Ctrl Pts',(-4.98274462345855,-1.77290647376134,
9.76274247656865));
#47668=CARTESIAN_POINT('Ctrl Pts',(-3.52788564023945,-3.94017312521954,
9.84211436662205));
#47669=CARTESIAN_POINT('Ctrl Pts',(-1.21364152390043,-5.14762232479954,
9.92148625667546));
#47670=CARTESIAN_POINT('Ctrl Pts',(1.39624298131078,-5.10112212012714,10.0008581467289));
#47671=CARTESIAN_POINT('Ctrl Pts',(3.66600578680612,-3.81199985813406,10.0802300367823));
#47672=CARTESIAN_POINT('Ctrl Pts',(5.04273769720163,-1.5942828684181,10.1596019268357));
#47673=CARTESIAN_POINT('Ctrl Pts',(5.19106986646944,1.01179789915923,10.2389738168891));
#47674=CARTESIAN_POINT('Ctrl Pts',(4.07486890650351,3.37140693807807,10.3183457069425));
#47675=CARTESIAN_POINT('Ctrl Pts',(1.96603890048266,4.90974870936374,10.3977175969959));
#47676=CARTESIAN_POINT('Ctrl Pts',(-0.621713829942471,5.25208656259283,
10.4770894870493));
#47677=CARTESIAN_POINT('Ctrl Pts',(-3.05801844753381,4.31502775447074,10.5564613771027));
#47678=CARTESIAN_POINT('Ctrl Pts',(-4.74939654011498,2.32683773651149,10.6358332671561));
#47679=CARTESIAN_POINT('Ctrl Pts',(-5.28383214813503,-0.228164803694007,
10.7152051572095));
#47680=CARTESIAN_POINT('Ctrl Pts',(-4.53113794043347,-2.72758690275384,
10.7945770472629));
#47681=CARTESIAN_POINT('Ctrl Pts',(-2.67466855994604,-4.56257486971405,
10.8739489373163));
#47682=CARTESIAN_POINT('Ctrl Pts',(-0.166655838534166,-5.2861296975001,
10.9533208273697));
#47683=CARTESIAN_POINT('Ctrl Pts',(2.38195387625819,-4.72199503162473,11.0326927174231));
#47684=CARTESIAN_POINT('Ctrl Pts',(4.3503248991595,-3.00759282800428,11.1120646074765));
#47685=CARTESIAN_POINT('Ctrl Pts',(5.2589664059064,-0.560547668675828,11.1914364975299));
#47686=CARTESIAN_POINT('Ctrl Pts',(4.8865353366992,2.02304566199086,11.2708083875833));
#47687=CARTESIAN_POINT('Ctrl Pts',(3.32375507563458,4.11382954733217,11.3501802776367));
#47688=CARTESIAN_POINT('Ctrl Pts',(0.951315435152466,5.20249366075065,11.4295521676901));
#47689=CARTESIAN_POINT('Ctrl Pts',(-1.6528625396318,5.02384183393465,11.5089240577436));
#47690=CARTESIAN_POINT('Ctrl Pts',(-3.85440685831092,3.62139325645746,11.5882959477969));
#47691=CARTESIAN_POINT('Ctrl Pts',(-5.11702619789041,1.33678129752526,11.6676678378503));
#47692=CARTESIAN_POINT('Ctrl Pts',(-5.13314928200913,-1.27346762656892,
11.7470397279037));
#47693=CARTESIAN_POINT('Ctrl Pts',(-3.89884856306365,-3.57350265560368,
11.8264116179572));
#47694=CARTESIAN_POINT('Ctrl Pts',(-1.71479696411077,-5.00304034754732,
11.9057835080105));
#47695=CARTESIAN_POINT('Ctrl Pts',(0.886975379660772,-5.21384848487043,
11.985155398064));
#47696=CARTESIAN_POINT('Ctrl Pts',(3.27268248423369,-4.15457467193696,12.0645272881174));
#47697=CARTESIAN_POINT('Ctrl Pts',(4.86117137960707,-2.08325566491467,12.1438991781708));
#47698=CARTESIAN_POINT('Ctrl Pts',(5.26548968692849,0.495539810872594,12.2232710682242));
#47699=CARTESIAN_POINT('Ctrl Pts',(4.38714636147788,2.95362288559007,12.3026429582776));
#47700=CARTESIAN_POINT('Ctrl Pts',(2.44010389315499,4.69220996311119,12.382014848331));
#47701=CARTESIAN_POINT('Ctrl Pts',(-0.101342482462103,5.28778507964898,
12.4613867383844));
#47702=CARTESIAN_POINT('Ctrl Pts',(-2.61810205366918,4.59526745509803,12.5407586284378));
#47703=CARTESIAN_POINT('Ctrl Pts',(-4.49709775967304,2.78335284993721,12.6201305184912));
#47704=CARTESIAN_POINT('Ctrl Pts',(-5.28061040557763,0.293419651378745,
12.6995024085446));
#47705=CARTESIAN_POINT('Ctrl Pts',(-4.7777780451164,-2.26798992478223,12.778874298598));
#47706=CARTESIAN_POINT('Ctrl Pts',(-3.11108952829712,-4.27692217537683,
12.8582461886514));
#47707=CARTESIAN_POINT('Ctrl Pts',(-0.686546488664521,-5.24400565085626,
12.9376180787048));
#47708=CARTESIAN_POINT('Ctrl Pts',(1.90523775596186,-4.93366095719673,13.0169899687582));
#47709=CARTESIAN_POINT('Ctrl Pts',(4.03291030040817,-3.42148737483739,13.0963618588116));
#47710=CARTESIAN_POINT('Ctrl Pts',(5.17817482237061,-1.07584704130148,13.175733748865));
#47711=CARTESIAN_POINT('Ctrl Pts',(5.06204741929909,1.53186725014844,13.2551056389184));
#47712=CARTESIAN_POINT('Ctrl Pts',(3.71281646953824,3.76642207019282,13.3344775289718));
#47713=CARTESIAN_POINT('Ctrl Pts',(1.45915164597774,5.08348481077208,13.4138494190252));
#47714=CARTESIAN_POINT('Ctrl Pts',(-1.14995928876559,5.16222190355004,13.4932213090786));
#47715=CARTESIAN_POINT('Ctrl Pts',(-3.47894268615732,3.98345316700755,13.572593199132));
#47716=CARTESIAN_POINT('Ctrl Pts',(-4.96046334571011,1.83432405620607,13.6519650891854));
#47717=CARTESIAN_POINT('Ctrl Pts',(-5.23362611404733,-0.761642334479749,
13.7313369792388));
#47718=CARTESIAN_POINT('Ctrl Pts',(-4.23188914543755,-3.17207433835303,
13.8107088692922));
#47719=CARTESIAN_POINT('Ctrl Pts',(-2.19927334812693,-4.80979605467098,
13.8900807593456));
#47720=CARTESIAN_POINT('Ctrl Pts',(0.369080568778457,-5.27586209837409,
13.9694526493991));
#47721=CARTESIAN_POINT('Ctrl Pts',(2.84752727607539,-4.45673981283591,14.0488245394524));
#47722=CARTESIAN_POINT('Ctrl Pts',(4.63232264181505,-2.55196557371717,14.1281964295059));
#47723=CARTESIAN_POINT('Ctrl Pts',(5.28869446548083,-0.0255381695209159,
14.2075683195592));
#47724=CARTESIAN_POINT('Ctrl Pts',(4.65675202368211,2.50711027624288,14.2869402096127));
#47725=CARTESIAN_POINT('Ctrl Pts',(2.89043509646017,4.42903220810837,14.3663120996661));
#47726=CARTESIAN_POINT('Ctrl Pts',(0.420014577610126,5.27205169757513,14.4456839897195));
#47727=CARTESIAN_POINT('Ctrl Pts',(-2.15272056265924,4.83081106300113,14.5250558797729));
#47728=CARTESIAN_POINT('Ctrl Pts',(-4.201057738831,3.21279554629894,14.6044277698263));
#47729=CARTESIAN_POINT('Ctrl Pts',(-5.22602654870706,0.81215014592063,14.6837996598797));
#47730=CARTESIAN_POINT('Ctrl Pts',(-4.97794685893165,-1.78633323234006,
14.7631715499331));
#47731=CARTESIAN_POINT('Ctrl Pts',(-3.51725033281897,-3.94966978918425,
14.8425434399865));
#47732=CARTESIAN_POINT('Ctrl Pts',(-1.19975941093315,-5.15087552782897,
14.9219153300399));
#47733=CARTESIAN_POINT('Ctrl Pts',(1.40999024783357,-5.09733938916413,15.0012872200933));
#47734=CARTESIAN_POINT('Ctrl Pts',(3.67626940318851,-3.8021026580683,15.0806591101467));
#47735=CARTESIAN_POINT('Ctrl Pts',(5.04701746921103,-1.5806821352785,15.1600310002001));
#47736=CARTESIAN_POINT('Ctrl Pts',(5.18832325111744,1.02578905688456,15.2394028902535));
#47737=CARTESIAN_POINT('Ctrl Pts',(4.06576497321036,3.38238030533612,15.3187747803069));
#47738=CARTESIAN_POINT('Ctrl Pts',(1.95279534724736,4.91503119817963,15.3981466703603));
#47739=CARTESIAN_POINT('Ctrl Pts',(-0.635870902865948,5.2503913703836,15.4775185604137));
#47740=CARTESIAN_POINT('Ctrl Pts',(-3.06964040851742,4.30676782630626,15.5568904504671));
#47741=CARTESIAN_POINT('Ctrl Pts',(-4.75565230518791,2.31402517260967,15.6362623405205));
#47742=CARTESIAN_POINT('Ctrl Pts',(-5.28319782677237,-0.24240889112691,
15.7156342305739));
#47743=CARTESIAN_POINT('Ctrl Pts',(-4.52376805191524,-2.73979268554778,
15.7950061206273));
#47744=CARTESIAN_POINT('Ctrl Pts',(-2.66235839280204,-4.56976904619777,
15.8743780106807));
#47745=CARTESIAN_POINT('Ctrl Pts',(-0.15240412223312,-5.28655978220556,
15.9537499007341));
#47746=CARTESIAN_POINT('Ctrl Pts',(2.39467545517194,-4.71555625687092,16.0331217907875));
#47747=CARTESIAN_POINT('Ctrl Pts',(4.35841739221953,-2.99585366506689,16.112493680841));
#47748=CARTESIAN_POINT('Ctrl Pts',(5.26045849971912,-0.546367751666672,
16.1918655708943));
#47749=CARTESIAN_POINT('Ctrl Pts',(4.88106356050808,2.03621213668353,16.2712374609478));
#47750=CARTESIAN_POINT('Ctrl Pts',(3.31265234202039,4.12277525560071,16.3506093510011));
#47751=CARTESIAN_POINT('Ctrl Pts',(0.937286345425132,5.20503944789207,16.4299812410546));
#47752=CARTESIAN_POINT('Ctrl Pts',(-1.66640053022416,5.01936755177917,16.509353131108));
#47753=CARTESIAN_POINT('Ctrl Pts',(-3.86415592530783,3.6109888303424,16.5887250211614));
#47754=CARTESIAN_POINT('Ctrl Pts',(-5.12061148999576,1.32298122241861,16.6680969112148));
#47755=CARTESIAN_POINT('Ctrl Pts',(-5.1296974302943,-1.28730168253218,16.7474688012682));
#47756=CARTESIAN_POINT('Ctrl Pts',(-3.88920043041393,-3.58400074773889,
16.8268406913216));
#47757=CARTESIAN_POINT('Ctrl Pts',(-1.70130281532588,-5.00764516247516,
16.906212581375));
#47758=CARTESIAN_POINT('Ctrl Pts',(0.90102840177319,-5.21143830245825,16.9855844714284));
#47759=CARTESIAN_POINT('Ctrl Pts',(3.28387109087768,-4.1457366023928,17.0649563614818));
#47760=CARTESIAN_POINT('Ctrl Pts',(4.86677005798476,-2.07014265165526,17.1443282515352));
#47761=CARTESIAN_POINT('Ctrl Pts',(5.26413459813378,0.50973348428664,17.2237001415886));
#47762=CARTESIAN_POINT('Ctrl Pts',(4.37916762715237,2.96543963879408,17.303072031642));
#47763=CARTESIAN_POINT('Ctrl Pts',(2.42744506809458,4.69877132337447,17.3824439216954));
#47764=CARTESIAN_POINT('Ctrl Pts',(-0.115597647321682,5.28749259670007,
17.4618158117488));
#47765=CARTESIAN_POINT('Ctrl Pts',(-2.63048120009413,4.58819259887652,17.5411877018022));
#47766=CARTESIAN_POINT('Ctrl Pts',(-4.5045850370732,2.7712186210673,17.6205595918556));
#47767=CARTESIAN_POINT('Ctrl Pts',(-5.28138253005218,0.27918271172893,17.699931481909));
#47768=CARTESIAN_POINT('Ctrl Pts',(-4.77164579536179,-2.28086298099153,
17.7793033719624));
#47769=CARTESIAN_POINT('Ctrl Pts',(-3.09954884704088,-4.28529268150238,
17.8586752620158));
#47770=CARTESIAN_POINT('Ctrl Pts',(-0.672404619068171,-5.24583989230806,
17.9380471520692));
#47771=CARTESIAN_POINT('Ctrl Pts',(1.91852825506979,-4.9285020674696,18.0174190421226));
#47772=CARTESIAN_POINT('Ctrl Pts',(4.04212630117149,-3.41061102326166,18.096790932176));
#47773=CARTESIAN_POINT('Ctrl Pts',(5.18104412158612,-1.06186685398811,18.1761628222294));
#47774=CARTESIAN_POINT('Ctrl Pts',(5.05792243214194,1.54547807796858,18.2555347122829));
#47775=CARTESIAN_POINT('Ctrl Pts',(3.70260503654169,3.77647571272922,18.3349066023362));
#47776=CARTESIAN_POINT('Ctrl Pts',(1.44552439996779,5.08729102078633,18.4142784923897));
#47777=CARTESIAN_POINT('Ctrl Pts',(-1.16402860508455,5.15930893371508,18.4936503824431));
#47778=CARTESIAN_POINT('Ctrl Pts',(-3.48937383888192,3.97367066688439,18.5730222724965));
#47779=CARTESIAN_POINT('Ctrl Pts',(-4.96594823061187,1.82167865277138,18.6523941625499));
#47780=CARTESIAN_POINT('Ctrl Pts',(-5.23050112077116,-0.77713504302674,
18.7317660526033));
#47781=CARTESIAN_POINT('Ctrl Pts',(-4.22530652207786,-3.18086119603167,
18.8111379426567));
#47782=CARTESIAN_POINT('Ctrl Pts',(-2.18257651229225,-4.82058518621618,
18.8905098327101));
#47783=CARTESIAN_POINT('Ctrl Pts',(0.37648005341871,-5.26605971579227,18.9698817227635));
#47784=CARTESIAN_POINT('Ctrl Pts',(3.70230252414111,-4.19446206534953,19.0757109095013));
#47785=CARTESIAN_POINT('Ctrl Pts',(5.99600976813328,-0.0197068834824163,
19.2079973929237));
#47786=CARTESIAN_POINT('Ctrl Pts',(3.26379011618947,5.03400372054209,19.3667411730305));
#47787=CARTESIAN_POINT('Ctrl Pts',(-2.45559119020206,5.46873373673905,19.5254849531373));
#47788=CARTESIAN_POINT('Ctrl Pts',(-5.92771323046149,0.905806267444168,
19.6842287332441));
#47789=CARTESIAN_POINT('Ctrl Pts',(-3.97578039972873,-4.48936692070992,
19.8429725133509));
#47790=CARTESIAN_POINT('Ctrl Pts',(1.61419617037569,-5.77483540889728,20.0017162934577));
#47791=CARTESIAN_POINT('Ctrl Pts',(5.72720375155094,-1.77677009197941,20.1604600735645));
#47792=CARTESIAN_POINT('Ctrl Pts',(4.59927593805412,3.84720861430021,20.3192038536713));
#47793=CARTESIAN_POINT('Ctrl Pts',(-0.73672307947618,5.95134306184733,20.4779476337782));
#47794=CARTESIAN_POINT('Ctrl Pts',(-5.3995463563661,2.60828838171381,20.6366914138849));
#47795=CARTESIAN_POINT('Ctrl Pts',(-5.1196790448508,-3.11863163173554,20.7954351939918));
#47796=CARTESIAN_POINT('Ctrl Pts',(-0.158509478954971,-5.99736559883163,
20.9541789740985));
#47797=CARTESIAN_POINT('Ctrl Pts',(4.95432466322423,-3.37745298000941,21.1129227542054));
#47798=CARTESIAN_POINT('Ctrl Pts',(5.4262515554071,1.3624793779577,21.2452092376277));
#47799=CARTESIAN_POINT('Ctrl Pts',(3.29092685490723,4.12830747359771,21.3510384243656));
#47800=CARTESIAN_POINT('Ctrl Pts',(0.929079443196039,5.20946188754723,21.430410314419));
#47801=CARTESIAN_POINT('Ctrl Pts',(-1.68303999757346,5.01382783115869,21.5097822044724));
#47802=CARTESIAN_POINT('Ctrl Pts',(-3.8722246926078,3.60110493868854,21.5891540945258));
#47803=CARTESIAN_POINT('Ctrl Pts',(-5.12503498129818,1.30888173016128,21.6685259845792));
#47804=CARTESIAN_POINT('Ctrl Pts',(-5.12574462250326,-1.300972874894,21.7478978746326));
#47805=CARTESIAN_POINT('Ctrl Pts',(-3.87976959979778,-3.59455409188016,
21.827269764686));
#47806=CARTESIAN_POINT('Ctrl Pts',(-1.68766624540451,-5.01217052435348,
21.9066416547394));
#47807=CARTESIAN_POINT('Ctrl Pts',(0.915005995631755,-5.2090130440819,21.9860135447928));
#47808=CARTESIAN_POINT('Ctrl Pts',(3.29507231119182,-4.13685632854986,22.0653854348462));
#47809=CARTESIAN_POINT('Ctrl Pts',(4.87231403886192,-2.05702097999265,22.1447573248996));
#47810=CARTESIAN_POINT('Ctrl Pts',(5.26275149225388,0.523926824466718,22.2241292149531));
#47811=CARTESIAN_POINT('Ctrl Pts',(4.37115162329097,2.97723307464397,22.3035011050064));
#47812=CARTESIAN_POINT('Ctrl Pts',(2.4147715124657,4.70529942618521,22.3828729950599));
#47813=CARTESIAN_POINT('Ctrl Pts',(-0.129853572474074,5.28716128664959,
22.4622448851132));
#47814=CARTESIAN_POINT('Ctrl Pts',(-2.64284027062663,4.58108446095525,22.5416167751666));
#47815=CARTESIAN_POINT('Ctrl Pts',(-4.51204028846786,2.7590644882843,22.62098866522));
#47816=CARTESIAN_POINT('Ctrl Pts',(-5.28211549991429,0.264943102456049,
22.7003605552734));
#47817=CARTESIAN_POINT('Ctrl Pts',(-4.76548000969985,-2.2937181486802,22.7797324453269));
#47818=CARTESIAN_POINT('Ctrl Pts',(-3.08798363825926,-4.29363457062517,
22.8591043353802));
#47819=CARTESIAN_POINT('Ctrl Pts',(-0.658261551986295,-5.24763120247219,
22.9384762254337));
#47820=CARTESIAN_POINT('Ctrl Pts',(1.93181173129385,-4.92331644248731,23.017848115487));
#47821=CARTESIAN_POINT('Ctrl Pts',(4.05129987868926,-3.39969271923279,23.0972200055405));
#47822=CARTESIAN_POINT('Ctrl Pts',(5.18390038229797,-1.0479113616667,23.1765918955939));
#47823=CARTESIAN_POINT('Ctrl Pts',(5.05371420635457,1.55913887720483,23.2559637856473));
#47824=CARTESIAN_POINT('Ctrl Pts',(3.69245444696201,3.78638634033052,23.3353356757007));
#47825=CARTESIAN_POINT('Ctrl Pts',(1.43172095156667,5.09127847004479,23.4147075657541));
#47826=CARTESIAN_POINT('Ctrl Pts',(-1.17777659548102,5.1559464348325,23.4940794558075));
#47827=CARTESIAN_POINT('Ctrl Pts',(-3.50037037246962,3.96463726004727,23.5734513458609));
#47828=CARTESIAN_POINT('Ctrl Pts',(-4.97028167379665,1.80755122457705,23.6528232359143));
#47829=CARTESIAN_POINT('Ctrl Pts',(-5.22944336137752,-0.789850288405212,
23.7321951259677));
#47830=CARTESIAN_POINT('Ctrl Pts',(-4.21472422106041,-3.19484601935549,
23.8115670160211));
#47831=CARTESIAN_POINT('Ctrl Pts',(-2.17330758975551,-4.82158433170509,
23.8909389060745));
#47832=CARTESIAN_POINT('Ctrl Pts',(0.397521959947206,-5.27379537322471,
23.9703107961279));
#47833=CARTESIAN_POINT('Ctrl Pts',(2.87151604007067,-4.4413215351868,24.0496826861813));
#47834=CARTESIAN_POINT('Ctrl Pts',(4.64601516884499,-2.5269516018695,24.1290545762347));
#47835=CARTESIAN_POINT('Ctrl Pts',(5.28875528625864,0.00297814834736192,
24.2084264662881));
#47836=CARTESIAN_POINT('Ctrl Pts',(4.64316632240633,2.53218242822061,24.2877983563415));
#47837=CARTESIAN_POINT('Ctrl Pts',(2.86651231988729,4.4445526734691,24.3671702463949));
#47838=CARTESIAN_POINT('Ctrl Pts',(0.391582261162602,5.27423972531146,24.4465421364484));
#47839=CARTESIAN_POINT('Ctrl Pts',(-2.1787363696294,4.81913365439931,24.5259140265017));
#47840=CARTESIAN_POINT('Ctrl Pts',(-4.21831964333045,3.19009729224708,24.6052859165552));
#47841=CARTESIAN_POINT('Ctrl Pts',(-5.23032958900859,0.783960290863936,
24.6846578066085));
#47842=CARTESIAN_POINT('Ctrl Pts',(-4.9682428239423,-1.81314770210696,24.764029696662));
#47843=CARTESIAN_POINT('Ctrl Pts',(-3.49590310398264,-3.96857692817898,
24.8434015867153));
#47844=CARTESIAN_POINT('Ctrl Pts',(-1.17196912594307,-5.15726959884261,
24.9227734767688));
#47845=CARTESIAN_POINT('Ctrl Pts',(1.43745393706658,-5.08966281065081,25.0021453668222));
#47846=CARTESIAN_POINT('Ctrl Pts',(3.69671640275713,-3.78222542756197,25.0815172568756));
#47847=CARTESIAN_POINT('Ctrl Pts',(5.05546693527898,-1.55344630213307,25.160889146929));
#47848=CARTESIAN_POINT('Ctrl Pts',(5.18271691245315,1.05374890400037,25.2402610369824));
#47849=CARTESIAN_POINT('Ctrl Pts',(4.04746852150308,3.40425320955296,25.3196329270358));
#47850=CARTESIAN_POINT('Ctrl Pts',(1.92626575763449,4.92548896844514,25.3990048170892));
#47851=CARTESIAN_POINT('Ctrl Pts',(-0.664171081076968,5.24688651700902,
25.4783767071426));
#47852=CARTESIAN_POINT('Ctrl Pts',(-3.09281731455583,4.2901541238158,25.5577485971959));
#47853=CARTESIAN_POINT('Ctrl Pts',(-4.76806009604388,2.2883496821561,25.6371204872494));
#47854=CARTESIAN_POINT('Ctrl Pts',(-5.28181399205765,-0.2708916769007,25.7164923773028));
#47855=CARTESIAN_POINT('Ctrl Pts',(-4.50892969070311,-2.76414442307307,
25.7958642673562));
#47856=CARTESIAN_POINT('Ctrl Pts',(-2.63768009703987,-4.58405770611471,
25.8752361574096));
#47857=CARTESIAN_POINT('Ctrl Pts',(-0.123897470143628,-5.28730467858643,
25.9546080474629));
#47858=CARTESIAN_POINT('Ctrl Pts',(2.42006630623721,-4.70257593460492,26.0339799375165));
#47859=CARTESIAN_POINT('Ctrl Pts',(4.37450728714461,-2.97231010192892,26.1133518275698));
#47860=CARTESIAN_POINT('Ctrl Pts',(5.26332797571122,-0.517996107519831,
26.1927237176232));
#47861=CARTESIAN_POINT('Ctrl Pts',(4.8700136195734,2.06250059211614,26.2720956076766));
#47862=CARTESIAN_POINT('Ctrl Pts',(3.29037472529985,4.14057671278022,26.35146749773));
#47863=CARTESIAN_POINT('Ctrl Pts',(0.909207831064193,5.21001751122215,26.4308393877834));
#47864=CARTESIAN_POINT('Ctrl Pts',(-1.69344007832135,5.01030957610855,26.5102112778369));
#47865=CARTESIAN_POINT('Ctrl Pts',(-3.88356973299385,3.59010131838702,26.5895831678902));
#47866=CARTESIAN_POINT('Ctrl Pts',(-5.12767039684481,1.29535232606086,26.6689550579437));
#47867=CARTESIAN_POINT('Ctrl Pts',(-5.12268190193029,-1.31494162567991,
26.748326947997));
#47868=CARTESIAN_POINT('Ctrl Pts',(-3.86981943456965,-3.604918707979,26.8276988380504));
#47869=CARTESIAN_POINT('Ctrl Pts',(-1.67427751864785,-5.01674557236666,
26.9070707281038));
#47870=CARTESIAN_POINT('Ctrl Pts',(0.929114694866165,-5.20650431970375,
26.9864426181573));
#47871=CARTESIAN_POINT('Ctrl Pts',(3.30617662527125,-4.12797013916282,27.0658145082107));
#47872=CARTESIAN_POINT('Ctrl Pts',(4.8778612478581,-2.04387156982875,27.145186398264));
#47873=CARTESIAN_POINT('Ctrl Pts',(5.26130966742943,0.538109589882639,27.2245582883175));
#47874=CARTESIAN_POINT('Ctrl Pts',(4.36311469772634,2.98900844458398,27.3039301783709));
#47875=CARTESIAN_POINT('Ctrl Pts',(2.40207464524773,4.7117914582426,27.3833020684242));
#47876=CARTESIAN_POINT('Ctrl Pts',(-0.144105473911181,5.28679250204684,
27.4626739584777));
#47877=CARTESIAN_POINT('Ctrl Pts',(-2.65518181859737,4.57394259446923,27.542045848531));
#47878=CARTESIAN_POINT('Ctrl Pts',(-4.51946174941854,2.74689039512913,27.6214177385845));
#47879=CARTESIAN_POINT('Ctrl Pts',(-5.28281080174027,0.25070177567431,27.7007896286378));
#47880=CARTESIAN_POINT('Ctrl Pts',(-4.75927883606144,-2.30655724141581,
27.7801615186913));
#47881=CARTESIAN_POINT('Ctrl Pts',(-3.07639708040302,-4.30194401997489,
27.8595334087447));
#47882=CARTESIAN_POINT('Ctrl Pts',(-0.644111805447875,-5.24938675745965,
27.9389052987981));
#47883=CARTESIAN_POINT('Ctrl Pts',(1.94507767959709,-4.91809050014772,28.0182771888515));
#47884=CARTESIAN_POINT('Ctrl Pts',(4.06045054724861,-3.38875828300845,28.0976490789049));
#47885=CARTESIAN_POINT('Ctrl Pts',(5.18670664924518,-1.03393204901761,28.1770209689583));
#47886=CARTESIAN_POINT('Ctrl Pts',(5.0494924920661,1.57275774354414,28.2563928590118));
#47887=CARTESIAN_POINT('Ctrl Pts',(3.68223314068176,3.79632723101881,28.3357647490651));
#47888=CARTESIAN_POINT('Ctrl Pts',(1.41798994671214,5.09511980804509,28.4151366391186));
#47889=CARTESIAN_POINT('Ctrl Pts',(-1.19167245960906,5.15275247768794,28.4945085291719));
#47890=CARTESIAN_POINT('Ctrl Pts',(-3.51104609249168,3.9551860491902,28.5738804192253));
#47891=CARTESIAN_POINT('Ctrl Pts',(-4.97513666881207,1.79414505376557,28.6532523092787));
#47892=CARTESIAN_POINT('Ctrl Pts',(-5.22729496488809,-0.803945705483672,
28.7326241993322));
#47893=CARTESIAN_POINT('Ctrl Pts',(-4.2060957779385,-3.20619707038074,28.8119960893855));
#47894=CARTESIAN_POINT('Ctrl Pts',(-2.16030096951815,-4.82742592572986,
28.891367979439));
#47895=CARTESIAN_POINT('Ctrl Pts',(0.41173837333167,-5.27270451089724,28.9707398694923));
#47896=CARTESIAN_POINT('Ctrl Pts',(2.88347915980534,-4.43356394814356,29.0501117595458));
#47897=CARTESIAN_POINT('Ctrl Pts',(4.65281080542333,-2.51441702114943,29.1294836495991));
#47898=CARTESIAN_POINT('Ctrl Pts',(5.28872803766221,0.0172363266290461,
29.2088555396526));
#47899=CARTESIAN_POINT('Ctrl Pts',(4.6363228263275,2.54469094339263,29.2882274297059));
#47900=CARTESIAN_POINT('Ctrl Pts',(2.85451963682592,4.45226447892365,29.3675993197594));
#47901=CARTESIAN_POINT('Ctrl Pts',(0.377361782165573,5.2752762423091,29.4469712098127));
#47902=CARTESIAN_POINT('Ctrl Pts',(-2.19172056735417,4.81324238969394,29.5263430998662));
#47903=CARTESIAN_POINT('Ctrl Pts',(-4.22690463795758,3.17871334488069,29.6057149899195));
#47904=CARTESIAN_POINT('Ctrl Pts',(-5.23242409484928,0.769856765217166,
29.6850868799731));
#47905=CARTESIAN_POINT('Ctrl Pts',(-4.96333662400999,-1.82653521840426,
29.7644587700263));
#47906=CARTESIAN_POINT('Ctrl Pts',(-3.48519133772112,-3.97798726578954,
29.8438306600798));
#47907=CARTESIAN_POINT('Ctrl Pts',(-1.15806115590354,-5.16041042035391,
29.9232025501331));
#47908=CARTESIAN_POINT('Ctrl Pts',(1.45117016016719,-5.08576901889481,30.0025744401866));
#47909=CARTESIAN_POINT('Ctrl Pts',(3.70689963733188,-3.77224554159173,30.08194633024));
#47910=CARTESIAN_POINT('Ctrl Pts',(5.05963656792573,-1.53981140008078,30.1613182202934));
#47911=CARTESIAN_POINT('Ctrl Pts',(5.17985722988845,1.06771739017516,30.2406901103468));
#47912=CARTESIAN_POINT('Ctrl Pts',(4.0382761360698,3.41515258753676,30.3200620004003));
#47913=CARTESIAN_POINT('Ctrl Pts',(1.91297991407722,4.93066417388641,30.3994338904535));
#47914=CARTESIAN_POINT('Ctrl Pts',(-0.678313980675348,5.24507688131741,
30.4788057805071));
#47915=CARTESIAN_POINT('Ctrl Pts',(-3.10437209115798,4.28180047024023,30.5581776705604));
#47916=CARTESIAN_POINT('Ctrl Pts',(-4.77421203164559,2.2754869422171,30.6375495606138));
#47917=CARTESIAN_POINT('Ctrl Pts',(-5.28106448876339,-0.285130168225216,
30.7169214506672));
#47918=CARTESIAN_POINT('Ctrl Pts',(-4.50146132585641,-2.77629020081278,
30.7962933407206));
#47919=CARTESIAN_POINT('Ctrl Pts',(-2.62531214778642,-4.59115208569648,
30.8756652307741));
#47920=CARTESIAN_POINT('Ctrl Pts',(-0.109642741545517,-5.28761948484725,
30.9550371208274));
#47921=CARTESIAN_POINT('Ctrl Pts',(2.43273539384572,-4.69603448143646,31.0344090108809));
#47922=CARTESIAN_POINT('Ctrl Pts',(4.38250457206463,-2.96050587284378,31.1137809009342));
#47923=CARTESIAN_POINT('Ctrl Pts',(5.26470533703794,-0.503804586594991,
31.1931527909877));
#47924=CARTESIAN_POINT('Ctrl Pts',(4.86443553513645,2.07562238179582,31.272524681041));
#47925=CARTESIAN_POINT('Ctrl Pts',(3.27920000412114,4.14943233229341,31.3518965710945));
#47926=CARTESIAN_POINT('Ctrl Pts',(0.895158610487983,5.21244975125701,31.4312684611478));
#47927=CARTESIAN_POINT('Ctrl Pts',(-1.70694143926006,5.00572594837619,31.5106403512013));
#47928=CARTESIAN_POINT('Ctrl Pts',(-3.89323433265515,3.57961838445739,31.5900122412546));
#47929=CARTESIAN_POINT('Ctrl Pts',(-5.13114396014345,1.28152370543563,31.6693841313081));
#47930=CARTESIAN_POINT('Ctrl Pts',(-5.11911827653528,-1.32874731162563,
31.7487560213615));
#47931=CARTESIAN_POINT('Ctrl Pts',(-3.86008671173927,-3.61533842470713,
31.8281279114149));
#47932=CARTESIAN_POINT('Ctrl Pts',(-1.6607465681206,-5.02124109994587,31.9074998014683));
#47933=CARTESIAN_POINT('Ctrl Pts',(0.943147763492109,-5.20398055756647,
31.9868716915216));
#47934=CARTESIAN_POINT('Ctrl Pts',(3.31729338754031,-4.11904187017945,32.0662435815751));
#47935=CARTESIAN_POINT('Ctrl Pts',(4.88335368508803,-2.03071370056122,32.1456154716285));
#47936=CARTESIAN_POINT('Ctrl Pts',(5.25983983406835,0.552291831605133,32.2249873616819));
#47937=CARTESIAN_POINT('Ctrl Pts',(4.35504064192764,3.00076029606972,32.3043592517354));
#47938=CARTESIAN_POINT('Ctrl Pts',(2.3893631891323,4.71825019448202,32.3837311417886));
#47939=CARTESIAN_POINT('Ctrl Pts',(-0.158357847769981,5.28638478918814,
32.4631030318421));
#47940=CARTESIAN_POINT('Ctrl Pts',(-2.66750326347463,4.56676775046226,32.5424749218955));
#47941=CARTESIAN_POINT('Ctrl Pts',(-4.52685078861515,2.73469619609277,32.6218468119489));
#47942=CARTESIAN_POINT('Ctrl Pts',(-5.28346748166331,0.23645870150246,32.7012187020024));
#47943=CARTESIAN_POINT('Ctrl Pts',(-4.75304319093522,-2.31937960938145,
32.7805905920557));
#47944=CARTESIAN_POINT('Ctrl Pts',(-3.06478809957792,-4.3102221812797,32.8599624821091));
#47945=CARTESIAN_POINT('Ctrl Pts',(-0.629957410956834,-5.25110417033318,
32.9393343721625));
#47946=CARTESIAN_POINT('Ctrl Pts',(1.95832950858626,-4.91282880661543,33.0187062622159));
#47947=CARTESIAN_POINT('Ctrl Pts',(4.06957169452659,-3.37779921996823,33.0980781522693));
#47948=CARTESIAN_POINT('Ctrl Pts',(5.18947522352436,-1.01994521996853,33.1774500423228));
#47949=CARTESIAN_POINT('Ctrl Pts',(5.04523407478018,1.586365178005,33.2568219323761));
#47950=CARTESIAN_POINT('Ctrl Pts',(3.67198507285579,3.80624052997629,33.3361938224296));
#47951=CARTESIAN_POINT('Ctrl Pts',(1.40424863498483,5.09892411381589,33.4155657124829));
#47952=CARTESIAN_POINT('Ctrl Pts',(-1.20555966211678,5.14952106980705,33.4949376025364));
#47953=CARTESIAN_POINT('Ctrl Pts',(-3.52169629398785,3.94570609146478,33.5743094925897));
#47954=CARTESIAN_POINT('Ctrl Pts',(-4.979955503786,1.78072584291395,33.6536813826432));
#47955=CARTESIAN_POINT('Ctrl Pts',(-5.22510857580638,-0.818035279400921,
33.7330532726965));
#47956=CARTESIAN_POINT('Ctrl Pts',(-4.19743676434199,-3.2175248183441,33.81242516275));
#47957=CARTESIAN_POINT('Ctrl Pts',(-2.14727864795256,-4.83323243340904,
33.8917970528034));
#47958=CARTESIAN_POINT('Ctrl Pts',(0.425951794157462,-5.27157532587404,
33.9711689428568));
#47959=CARTESIAN_POINT('Ctrl Pts',(2.89542132203897,-4.4257741373902,34.0505408329101));
#47960=CARTESIAN_POINT('Ctrl Pts',(4.6595726247782,-2.50186416532303,34.1299127229636));
#47961=CARTESIAN_POINT('Ctrl Pts',(5.28866234991056,0.0314943796344648,
34.209284613017));
#47962=CARTESIAN_POINT('Ctrl Pts',(4.62944563286023,2.55718096342464,34.2886565030704));
#47963=CARTESIAN_POINT('Ctrl Pts',(2.84250620674923,4.45994392474861,34.3680283931238));
#47964=CARTESIAN_POINT('Ctrl Pts',(0.363138560454883,5.27627441792225,34.4474002831772));
#47965=CARTESIAN_POINT('Ctrl Pts',(-2.20468883537271,4.80731614172534,34.5267721732306));
#47966=CARTESIAN_POINT('Ctrl Pts',(-4.23545891089946,3.1673062942179,34.606144063284));
#47967=CARTESIAN_POINT('Ctrl Pts',(-5.23448057076036,0.755747644152594,
34.6855159533374));
#47968=CARTESIAN_POINT('Ctrl Pts',(-4.95839434991029,-1.83990945920924,
34.7648878433908));
#47969=CARTESIAN_POINT('Ctrl Pts',(-3.47445424064183,-3.98736869087822,
34.8442597334442));
#47970=CARTESIAN_POINT('Ctrl Pts',(-1.14414476892706,-5.16351373534018,
34.9236316234976));
#47971=CARTESIAN_POINT('Ctrl Pts',(1.4648758359769,-5.0818382631171,35.003003513551));
#47972=CARTESIAN_POINT('Ctrl Pts',(3.71705592968454,-3.76223823845686,35.0823754036044));
#47973=CARTESIAN_POINT('Ctrl Pts',(5.06376942648477,-1.52616530648161,35.1617472936578));
#47974=CARTESIAN_POINT('Ctrl Pts',(5.1769598994568,1.08167811604296,35.2411191837112));
#47975=CARTESIAN_POINT('Ctrl Pts',(4.02905439992751,3.42602714375337,35.3204910737646));
#47976=CARTESIAN_POINT('Ctrl Pts',(1.8996801667365,4.93580354262787,35.3998629638181));
#47977=CARTESIAN_POINT('Ctrl Pts',(-0.69245195020073,5.24322912373406,35.4792348538714));
#47978=CARTESIAN_POINT('Ctrl Pts',(-3.11590430478548,4.27341569598948,35.5586067439249));
#47979=CARTESIAN_POINT('Ctrl Pts',(-4.78032926766171,2.26260766374704,35.6379786339782));
#47980=CARTESIAN_POINT('Ctrl Pts',(-5.28027660201491,-0.299366587187078,
35.7173505240316));
#47981=CARTESIAN_POINT('Ctrl Pts',(-4.49396024381123,-2.78841580011912,
35.7967224140851));
#47982=CARTESIAN_POINT('Ctrl Pts',(-2.61292511742748,-4.59821309619579,
35.8760943041384));
#47983=CARTESIAN_POINT('Ctrl Pts',(-0.0953872160500441,-5.28789586001125,
35.9554661941919));
#47984=CARTESIAN_POINT('Ctrl Pts',(2.4453868000212,-4.68945889688694,36.0348380842453));
#47985=CARTESIAN_POINT('Ctrl Pts',(4.39047000437915,-2.94868012642215,36.1142099742987));
#47986=CARTESIAN_POINT('Ctrl Pts',(5.26604443381084,-0.489609403953667,
36.1935818643521));
#47987=CARTESIAN_POINT('Ctrl Pts',(4.85882209535785,2.08872908558584,36.2729537544055));
#47988=CARTESIAN_POINT('Ctrl Pts',(3.26800144929601,4.15825779320007,36.3523256444589));
#47989=CARTESIAN_POINT('Ctrl Pts',(0.881102883784141,5.2148441065383,36.4316975345123));
#47990=CARTESIAN_POINT('Ctrl Pts',(-1.72043039392939,5.00110593838543,36.5110694245656));
#47991=CARTESIAN_POINT('Ctrl Pts',(-3.90287063578981,3.56910943340206,36.5904413146191));
#47992=CARTESIAN_POINT('Ctrl Pts',(-5.13458022962944,1.26768577053169,36.6698132046725));
#47993=CARTESIAN_POINT('Ctrl Pts',(-5.11551744473188,-1.34254334006536,
36.7491850947259));
#47994=CARTESIAN_POINT('Ctrl Pts',(-3.85032593330342,-3.62573186469175,
36.8285569847793));
#47995=CARTESIAN_POINT('Ctrl Pts',(-1.64720354707418,-5.02570013250056,
36.9079288748327));
#47996=CARTESIAN_POINT('Ctrl Pts',(0.957173977199105,-5.20141897223083,
36.9873007648861));
#47997=CARTESIAN_POINT('Ctrl Pts',(3.32838603929536,-4.11008366347129,37.0666726549395));
#47998=CARTESIAN_POINT('Ctrl Pts',(4.88881062947681,-2.01754107180608,37.1460445449929));
#47999=CARTESIAN_POINT('Ctrl Pts',(5.25833177151655,0.566470059199757,37.2254164350463));
#48000=CARTESIAN_POINT('Ctrl Pts',(4.34693493313475,3.01249033764469,37.3047883250998));
#48001=CARTESIAN_POINT('Ctrl Pts',(2.37663436681862,4.72467463787371,37.3841602151531));
#48002=CARTESIAN_POINT('Ctrl Pts',(-0.17260907066365,5.28593865420645,37.4635321052065));
#48003=CARTESIAN_POINT('Ctrl Pts',(-2.67980532059584,4.55955971460153,37.54290399526));
#48004=CARTESIAN_POINT('Ctrl Pts',(-4.53420692607955,2.72248212093334,37.6222758853133));
#48005=CARTESIAN_POINT('Ctrl Pts',(-5.28408576066665,0.222213908718847,
37.7016477753668));
#48006=CARTESIAN_POINT('Ctrl Pts',(-4.74677300008161,-2.33218511979937,
37.7810196654201));
#48007=CARTESIAN_POINT('Ctrl Pts',(-3.05315684347904,-4.31846901533503,
37.8603915554736));
#48008=CARTESIAN_POINT('Ctrl Pts',(-0.615798437855754,-5.25278341751105,
37.9397634455269));
#48009=CARTESIAN_POINT('Ctrl Pts',(1.97156710418767,-4.90753140600709,38.0191353355804));
#48010=CARTESIAN_POINT('Ctrl Pts',(4.07866326363087,-3.36681560666115,38.0985072256337));
#48011=CARTESIAN_POINT('Ctrl Pts',(5.19220608004019,-1.00595097780572,38.1778791156872));
#48012=CARTESIAN_POINT('Ctrl Pts',(5.04093898806991,1.59996108252017,38.2572510057405));
#48013=CARTESIAN_POINT('Ctrl Pts',(3.66171031660113,3.81612616476472,38.336622895794));
#48014=CARTESIAN_POINT('Ctrl Pts',(1.39049711694169,5.10269135980963,38.4159947858473));
#48015=CARTESIAN_POINT('Ctrl Pts',(-1.21943810235573,5.14625223481529,38.4953666759008));
#48016=CARTESIAN_POINT('Ctrl Pts',(-3.53232089954511,3.93619745533324,38.5747385659542));
#48017=CARTESIAN_POINT('Ctrl Pts',(-4.98473814342406,1.76729369047725,38.6541104560076));
#48018=CARTESIAN_POINT('Ctrl Pts',(-5.22288421068334,-0.832118909543577,
38.733482346061));
#48019=CARTESIAN_POINT('Ctrl Pts',(-4.18874724188046,-3.22882917750522,
38.8128542361144));
#48020=CARTESIAN_POINT('Ctrl Pts',(-2.13424072225093,-4.83900381899058,
38.8922261261678));
#48021=CARTESIAN_POINT('Ctrl Pts',(0.440162123945958,-5.27040781417516,
38.9715980162212));
#48022=CARTESIAN_POINT('Ctrl Pts',(2.90734243084964,-4.41795218255951,39.0509699062746));
#48023=CARTESIAN_POINT('Ctrl Pts',(4.66630059499982,-2.48929308216594,39.130341796328));
#48024=CARTESIAN_POINT('Ctrl Pts',(5.288558190933,0.0457521216721363,39.2097136863814));
#48025=CARTESIAN_POINT('Ctrl Pts',(4.62253485344793,2.56965255248844,39.2890855764349));
#48026=CARTESIAN_POINT('Ctrl Pts',(2.83047200092405,4.46759066254981,39.3684574664882));
#48027=CARTESIAN_POINT('Ctrl Pts',(0.34891291852996,5.27723479734496,39.4478293565417));
#48028=CARTESIAN_POINT('Ctrl Pts',(-2.21764149317963,4.80135391043001,39.527201246595));
#48029=CARTESIAN_POINT('Ctrl Pts',(-4.24398161873814,3.15587819282133,39.6065731366485));
#48030=CARTESIAN_POINT('Ctrl Pts',(-5.23650047694821,0.74162931109825,39.6859450267018));
#48031=CARTESIAN_POINT('Ctrl Pts',(-4.9534132521342,-1.85326330477585,39.7653169167553));
#48032=CARTESIAN_POINT('Ctrl Pts',(-3.46369715057683,-3.99673439595749,
39.8446888068086));
#48033=CARTESIAN_POINT('Ctrl Pts',(-1.13021013185916,-5.16655447652188,
39.9240606968621));
#48034=CARTESIAN_POINT('Ctrl Pts',(1.47855208450035,-5.0779179090888,40.0034325869154));
#48035=CARTESIAN_POINT('Ctrl Pts',(3.72722085031374,-3.75211381890458,40.0828044769689));
#48036=CARTESIAN_POINT('Ctrl Pts',(5.06779668194711,-1.51268081279862,40.1621763670222));
#48037=CARTESIAN_POINT('Ctrl Pts',(5.17416686787614,1.09598291074358,40.2415482570757));
#48038=CARTESIAN_POINT('Ctrl Pts',(4.40436067122798,2.65600709442752,40.2944628504446));
#48039=CARTESIAN_POINT('Ctrl Pts',(3.85627053850219,3.29705846079199,40.3209201471291));
#48040=CARTESIAN_POINT('Ctrl Pts',(1.26508527942741,-4.72177922709091,-0.106973382376351));
#48041=CARTESIAN_POINT('Ctrl Pts',(2.05001543279104,-4.51147638686031,-0.0805160856918833));
#48042=CARTESIAN_POINT('Ctrl Pts',(3.5121928105948,-3.69213734276823,-0.0276014923229477));
#48043=CARTESIAN_POINT('Ctrl Pts',(4.85026808817394,-1.56206090154413,0.0517703977304561));
#48044=CARTESIAN_POINT('Ctrl Pts',(5.00665954563268,0.947775616877177,0.13114228778386));
#48045=CARTESIAN_POINT('Ctrl Pts',(3.94352649879584,3.22711800485082,0.210514177837264));
#48046=CARTESIAN_POINT('Ctrl Pts',(1.91971357759781,4.72014150668349,0.289886067890667));
#48047=CARTESIAN_POINT('Ctrl Pts',(-0.571713243107534,5.06345468357225,
0.369257957944071));
#48048=CARTESIAN_POINT('Ctrl Pts',(-2.92388473013463,4.17326556172555,0.448629847997474));
#48049=CARTESIAN_POINT('Ctrl Pts',(-4.56379761866667,2.26650781142313,0.528001738050878));
#48050=CARTESIAN_POINT('Ctrl Pts',(-5.091983083909,-0.192381913949067,0.607373628104282));
#48051=CARTESIAN_POINT('Ctrl Pts',(-4.37977084759389,-2.6043995219968,0.686745518157685));
#48052=CARTESIAN_POINT('Ctrl Pts',(-2.60065712992448,-4.3819955716546,0.766117408211089));
#48053=CARTESIAN_POINT('Ctrl Pts',(-0.188028560849166,-5.09214486895681,
0.845489298264494));
#48054=CARTESIAN_POINT('Ctrl Pts',(2.27040306822816,-4.56186018168567,0.924861188317896));
#48055=CARTESIAN_POINT('Ctrl Pts',(4.17576968427582,-2.92031579800744,1.0042330783713));
#48056=CARTESIAN_POINT('Ctrl Pts',(5.06392796926476,-0.567389296122094,
1.0836049684247));
#48057=CARTESIAN_POINT('Ctrl Pts',(4.71852465152963,1.92375216574099,1.16297685847811));
#48058=CARTESIAN_POINT('Ctrl Pts',(3.22369915083516,3.94627176108661,1.24234874853151));
#48059=CARTESIAN_POINT('Ctrl Pts',(0.943587684251177,5.00748834177841,1.32172063858492));
#48060=CARTESIAN_POINT('Ctrl Pts',(-1.5663796598258,4.84889181906687,1.40109252863832));
#48061=CARTESIAN_POINT('Ctrl Pts',(-3.69478038260539,3.50911599649364,1.48046441869172));
#48062=CARTESIAN_POINT('Ctrl Pts',(-4.92314078418047,1.3145272768326,1.55983630874512));
#48063=CARTESIAN_POINT('Ctrl Pts',(-4.9522349869947,-1.20027737376273,1.63920819879853));
#48064=CARTESIAN_POINT('Ctrl Pts',(-3.77497570905141,-3.4226971150208,1.71858008885193));
#48065=CARTESIAN_POINT('Ctrl Pts',(-1.67814070389166,-4.81135541393673,
1.79795197890534));
#48066=CARTESIAN_POINT('Ctrl Pts',(0.827485662097738,-5.02797818437314,
1.87732386895874));
#48067=CARTESIAN_POINT('Ctrl Pts',(3.13153835248109,-4.01979659801894,1.95669575901214));
#48068=CARTESIAN_POINT('Ctrl Pts',(4.6727552317042,-2.03240145822472,2.03606764906555));
#48069=CARTESIAN_POINT('Ctrl Pts',(5.07569927947279,0.450082178237972,2.11543953911895));
#48070=CARTESIAN_POINT('Ctrl Pts',(4.24221421762082,2.82292679227462,2.19481142917235));
#48071=CARTESIAN_POINT('Ctrl Pts',(2.37533516234403,4.50811268818069,2.27418331922576));
#48072=CARTESIAN_POINT('Ctrl Pts',(-0.0701702807675918,5.09513231177087,
2.35355520927916));
#48073=CARTESIAN_POINT('Ctrl Pts',(-2.49858239880191,4.44098898210475,2.43292709933257));
#48074=CARTESIAN_POINT('Ctrl Pts',(-4.31834537500726,2.70503056635658,2.51229898938597));
#48075=CARTESIAN_POINT('Ctrl Pts',(-5.08616897635574,0.310132692129504,
2.59167087943937));
#48076=CARTESIAN_POINT('Ctrl Pts',(-4.61501307310829,-2.16031281943427,
2.67104276949278));
#48077=CARTESIAN_POINT('Ctrl Pts',(-3.01965020040969,-4.10451090995464,
2.75041465954618));
#48078=CARTESIAN_POINT('Ctrl Pts',(-0.688707222773715,-5.04885922799114,
2.82978654959958));
#48079=CARTESIAN_POINT('Ctrl Pts',(1.8100033099024,-4.7633166135492,2.90915843965299));
#48080=CARTESIAN_POINT('Ctrl Pts',(3.86780104266064,-3.31744061546923,2.98853032970639));
#48081=CARTESIAN_POINT('Ctrl Pts',(4.98341100265916,-1.06344342649117,3.0679022197598));
#48082=CARTESIAN_POINT('Ctrl Pts',(4.88507307300304,1.44960622728803,3.1472741098132));
#48083=CARTESIAN_POINT('Ctrl Pts',(3.59674215568923,3.60953501274882,3.2266459998666));
#48084=CARTESIAN_POINT('Ctrl Pts',(1.43225281050325,4.89018905867422,3.30601788992001));
#48085=CARTESIAN_POINT('Ctrl Pts',(-1.0811301490835,4.97960387415649,3.38538977997341));
#48086=CARTESIAN_POINT('Ctrl Pts',(-3.3311521973945,3.85599820806045,3.46476167002682));
#48087=CARTESIAN_POINT('Ctrl Pts',(-4.76971294380054,1.79307991358813,3.54413356008021));
#48088=CARTESIAN_POINT('Ctrl Pts',(-5.04638217467727,-0.706628678919173,
3.62350545013362));
#48089=CARTESIAN_POINT('Ctrl Pts',(-4.09376387778011,-3.03420408933784,
3.70287734018702));
#48090=CARTESIAN_POINT('Ctrl Pts',(-2.14391376164834,-4.62265409969061,
3.78224923024043));
#48091=CARTESIAN_POINT('Ctrl Pts',(0.328189001348338,-5.08503580343006,
3.86162112029383));
#48092=CARTESIAN_POINT('Ctrl Pts',(2.72034565005059,-4.30871404098977,3.94099301034724));
#48093=CARTESIAN_POINT('Ctrl Pts',(4.44983211978348,-2.48279907534115,4.02036490040064));
#48094=CARTESIAN_POINT('Ctrl Pts',(5.09534933467345,-0.0520797505219637,
4.09973679045404));
#48095=CARTESIAN_POINT('Ctrl Pts',(4.49965073000142,2.39132608624781,4.17910868050745));
#48096=CARTESIAN_POINT('Ctrl Pts',(2.80784716730899,4.25221018151813,4.25848057056085));
#48097=CARTESIAN_POINT('Ctrl Pts',(0.432058249724383,5.07726528867822,4.33785246061425));
#48098=CARTESIAN_POINT('Ctrl Pts',(-2.04897910114838,4.66550980985238,4.41722435066766));
#48099=CARTESIAN_POINT('Ctrl Pts',(-4.03088967831969,3.1172464682773,4.49659624072106));
#48100=CARTESIAN_POINT('Ctrl Pts',(-5.0308844520753,0.809628786937908,4.57596813077447));
#48101=CARTESIAN_POINT('Ctrl Pts',(-4.80536690897923,-1.69521267481664,
4.65534002082787));
#48102=CARTESIAN_POINT('Ctrl Pts',(-3.40927262335505,-3.78710408127548,
4.73471191088127));
#48103=CARTESIAN_POINT('Ctrl Pts',(-1.18268707297853,-4.9564653161483,4.81408380093467));
#48104=CARTESIAN_POINT('Ctrl Pts',(1.33199843054213,-4.91844257095729,4.89345569098808));
#48105=CARTESIAN_POINT('Ctrl Pts',(3.52221206471124,-3.68229810226904,4.97282758104148));
#48106=CARTESIAN_POINT('Ctrl Pts',(4.85442263620086,-1.54915396649666,5.05219947109489));
#48107=CARTESIAN_POINT('Ctrl Pts',(5.00410659859419,0.961360646520152,5.13157136114829));
#48108=CARTESIAN_POINT('Ctrl Pts',(3.93480126997208,3.23768993398037,5.21094325120169));
#48109=CARTESIAN_POINT('Ctrl Pts',(1.90698706151963,4.72532512002807,5.2903151412551));
#48110=CARTESIAN_POINT('Ctrl Pts',(-0.585364974074726,5.06188156616668,
5.3696870313085));
#48111=CARTESIAN_POINT('Ctrl Pts',(-2.93512339766788,4.1653748670719,5.44905892136191));
#48112=CARTESIAN_POINT('Ctrl Pts',(-4.56989225837456,2.25419207025927,5.52843081141531));
#48113=CARTESIAN_POINT('Ctrl Pts',(-5.09144548022617,-0.206106925298976,
5.60780270146872));
#48114=CARTESIAN_POINT('Ctrl Pts',(-4.37273385281808,-2.61619873006436,
5.68717459152211));
#48115=CARTESIAN_POINT('Ctrl Pts',(-2.58883393774572,-4.38899031504372,
5.76654648157553));
#48116=CARTESIAN_POINT('Ctrl Pts',(-0.174299805725225,-5.09263357414371,
5.84591837162892));
#48117=CARTESIAN_POINT('Ctrl Pts',(2.28269337316386,-4.5557225669355,5.92529026168233));
#48118=CARTESIAN_POINT('Ctrl Pts',(4.18362749900631,-2.90904762634266,6.00466215173574));
#48119=CARTESIAN_POINT('Ctrl Pts',(5.0654392263932,-0.553735123040447,6.08403404178913));
#48120=CARTESIAN_POINT('Ctrl Pts',(4.71332117039027,1.9364660305625,6.16340593184254));
#48121=CARTESIAN_POINT('Ctrl Pts',(3.21304851003972,3.95494834541529,6.24277782189595));
#48122=CARTESIAN_POINT('Ctrl Pts',(0.93008434460575,5.01001399745458,6.32214971194934));
#48123=CARTESIAN_POINT('Ctrl Pts',(-1.57944630846742,4.84465132919185,6.40152160200275));
#48124=CARTESIAN_POINT('Ctrl Pts',(-3.70422733684302,3.49914232059178,6.48089349205615));
#48125=CARTESIAN_POINT('Ctrl Pts',(-4.92666678513181,1.30124998791572,6.56026538210956));
#48126=CARTESIAN_POINT('Ctrl Pts',(-4.94898110955443,-1.21362396154863,
6.63963727216295));
#48127=CARTESIAN_POINT('Ctrl Pts',(-3.76573459007348,-3.43286180029078,
6.71900916221637));
#48128=CARTESIAN_POINT('Ctrl Pts',(-1.66516345976277,-4.81586210299283,
6.79838105226976));
#48129=CARTESIAN_POINT('Ctrl Pts',(0.841037803569352,-5.02572905713577,
6.87775294232318));
#48130=CARTESIAN_POINT('Ctrl Pts',(3.14236411955759,-4.01133953722303,6.95712483237658));
#48131=CARTESIAN_POINT('Ctrl Pts',(4.6782174915266,-2.0197965849922,7.03649672242998));
#48132=CARTESIAN_POINT('Ctrl Pts',(5.0744674376185,0.463764344598802,7.11586861248339));
#48133=CARTESIAN_POINT('Ctrl Pts',(4.23458834804968,2.83435330637052,7.19524050253678));
#48134=CARTESIAN_POINT('Ctrl Pts',(2.36317290999828,4.51450007644499,7.2746123925902));
#48135=CARTESIAN_POINT('Ctrl Pts',(-0.0839062181341898,5.09492462057389,
7.35398428264359));
#48136=CARTESIAN_POINT('Ctrl Pts',(-2.51054597725242,4.43423680455535,7.433356172697));
#48137=CARTESIAN_POINT('Ctrl Pts',(-4.32562229331123,2.69337871796382,7.5127280627504));
#48138=CARTESIAN_POINT('Ctrl Pts',(-5.08698659332198,0.296419537368979,
7.5920999528038));
#48139=CARTESIAN_POINT('Ctrl Pts',(-4.60917221905333,-2.17274678641544,
7.67147184285721));
#48140=CARTESIAN_POINT('Ctrl Pts',(-3.00857369445294,-4.11263680232249,
7.75084373291061));
#48141=CARTESIAN_POINT('Ctrl Pts',(-0.675093277248738,-5.05069759635094,
7.83021562296402));
#48142=CARTESIAN_POINT('Ctrl Pts',(1.82283836799964,-4.7584196354378,7.90958751301742));
#48143=CARTESIAN_POINT('Ctrl Pts',(3.8767306215876,-3.30700118391521,7.98895940307083));
#48144=CARTESIAN_POINT('Ctrl Pts',(4.9862598767545,-1.05000456391383,8.06833129312422));
#48145=CARTESIAN_POINT('Ctrl Pts',(4.881147262843,1.46277084371127,8.14770318317763));
#48146=CARTESIAN_POINT('Ctrl Pts',(3.58699797993919,3.61921851159664,8.22707507323104));
#48147=CARTESIAN_POINT('Ctrl Pts',(1.41906392880751,4.89403256106139,8.30644696328444));
#48148=CARTESIAN_POINT('Ctrl Pts',(-1.09455095433695,4.97667111140887,8.38581885333784));
#48149=CARTESIAN_POINT('Ctrl Pts',(-3.34153564775234,3.84700359469183,8.46519074339125));
#48150=CARTESIAN_POINT('Ctrl Pts',(-4.77452965373897,1.7802145175059,8.54456263344465));
#48151=CARTESIAN_POINT('Ctrl Pts',(-5.04445880431694,-0.720230875706447,
8.62393452349805));
#48152=CARTESIAN_POINT('Ctrl Pts',(-4.08556895588349,-3.04522962180074,
8.70330641355146));
#48153=CARTESIAN_POINT('Ctrl Pts',(-2.1314435530503,-4.62841717252583,8.78267830360486));
#48154=CARTESIAN_POINT('Ctrl Pts',(0.341896781435676,-5.08413254485124,
8.86205019365827));
#48155=CARTESIAN_POINT('Ctrl Pts',(2.73195181673958,-4.30136448278739,8.94142208371167));
#48156=CARTESIAN_POINT('Ctrl Pts',(4.45650943655852,-2.47079355362535,9.02079397376506));
#48157=CARTESIAN_POINT('Ctrl Pts',(5.09547122194811,-0.0383427838088964,
9.10016586381848));
#48158=CARTESIAN_POINT('Ctrl Pts',(4.49318749630538,2.40344820327308,9.17953775387187));
#48159=CARTESIAN_POINT('Ctrl Pts',(2.79637324206448,4.25976452798008,9.25890964392529));
#48160=CARTESIAN_POINT('Ctrl Pts',(0.418368655723882,5.07841164249998,9.33828153397869));
#48161=CARTESIAN_POINT('Ctrl Pts',(-2.06154960910779,4.65996892178041,9.41765342403209));
#48162=CARTESIAN_POINT('Ctrl Pts',(-4.03927895232343,3.10636808638134,9.49702531408549));
#48163=CARTESIAN_POINT('Ctrl Pts',(-5.03304888354539,0.79606286096894,9.5763972041389));
#48164=CARTESIAN_POINT('Ctrl Pts',(-4.80077924720044,-1.70816151532024,
9.6557690941923));
#48165=CARTESIAN_POINT('Ctrl Pts',(-3.39905041258209,-3.7962815274288,9.7351409842457));
#48166=CARTESIAN_POINT('Ctrl Pts',(-1.16932042112922,-4.95963576238233,
9.81451287429911));
#48167=CARTESIAN_POINT('Ctrl Pts',(1.34525343666388,-4.91483370358709,9.89388476435251));
#48168=CARTESIAN_POINT('Ctrl Pts',(3.53212653495364,-3.67278903339792,9.97325665440591));
#48169=CARTESIAN_POINT('Ctrl Pts',(4.85858142755815,-1.53606108425365,10.0526285444593));
#48170=CARTESIAN_POINT('Ctrl Pts',(5.00149663869711,0.974847945001263,10.1320004345127));
#48171=CARTESIAN_POINT('Ctrl Pts',(3.92605833927446,3.24828617264322,10.2113723245661));
#48172=CARTESIAN_POINT('Ctrl Pts',(1.89424091858727,4.73044907858876,10.2907442146195));
#48173=CARTESIAN_POINT('Ctrl Pts',(-0.599009397036607,5.0602850596615,10.3701161046729));
#48174=CARTESIAN_POINT('Ctrl Pts',(-2.94634234942717,4.15744680095171,10.4494879947264));
#48175=CARTESIAN_POINT('Ctrl Pts',(-4.57595282711548,2.24186370388246,10.5288598847797));
#48176=CARTESIAN_POINT('Ctrl Pts',(-5.09087132481819,-0.219832429171425,
10.6082317748331));
#48177=CARTESIAN_POINT('Ctrl Pts',(-4.36566483624775,-2.62797786906995,
10.6876036648866));
#48178=CARTESIAN_POINT('Ctrl Pts',(-2.57699205680257,-4.39595371699339,
10.7669755549399));
#48179=CARTESIAN_POINT('Ctrl Pts',(-0.160569716395434,-5.09308496973576,
10.8463474449934));
#48180=CARTESIAN_POINT('Ctrl Pts',(2.2949670515106,-4.54955199720284,10.9257193350468));
#48181=CARTESIAN_POINT('Ctrl Pts',(4.19145492549203,-2.89775822841384,11.0050912251002));
#48182=CARTESIAN_POINT('Ctrl Pts',(5.06691365725173,-0.540076969262297,
11.0844631151535));
#48183=CARTESIAN_POINT('Ctrl Pts',(4.70808343752805,1.94916584416147,11.163835005207));
#48184=CARTESIAN_POINT('Ctrl Pts',(3.20237451358847,3.96359617235289,11.2432068952604));
#48185=CARTESIAN_POINT('Ctrl Pts',(0.916574246474504,5.01250324623051,11.3225787853138));
#48186=CARTESIAN_POINT('Ctrl Pts',(-1.59250147827797,4.84037562431409,11.4019506753672));
#48187=CARTESIAN_POINT('Ctrl Pts',(-3.71364736786416,3.4891432143045,11.4813225654206));
#48188=CARTESIAN_POINT('Ctrl Pts',(-4.93015697865768,1.28796324037784,11.560694455474));
#48189=CARTESIAN_POINT('Ctrl Pts',(-4.94569126216756,-1.22696172804661,
11.6400663455274));
#48190=CARTESIAN_POINT('Ctrl Pts',(-3.75646610131532,-3.44300153535262,
11.7194382355808));
#48191=CARTESIAN_POINT('Ctrl Pts',(-1.65217411297936,-4.82033378960134,
11.7988101256342));
#48192=CARTESIAN_POINT('Ctrl Pts',(0.854583832252985,-5.02344340233105,
11.8781820156876));
#48193=CARTESIAN_POINT('Ctrl Pts',(3.15316704753777,-4.00285332145629,11.957553905741));
#48194=CARTESIAN_POINT('Ctrl Pts',(4.6836457494592,-2.00717703164028,12.0369257957944));
#48195=CARTESIAN_POINT('Ctrl Pts',(5.07319871388639,0.477443140272258,12.1162976858478));
#48196=CARTESIAN_POINT('Ctrl Pts',(4.22693170094574,2.84575922001696,12.1956695759012));
#48197=CARTESIAN_POINT('Ctrl Pts',(2.35099348180933,4.52085465274672,12.2750414659546));
#48198=CARTESIAN_POINT('Ctrl Pts',(-0.0976415456600611,5.09467989880942,
12.354413356008));
#48199=CARTESIAN_POINT('Ctrl Pts',(-2.52249130873252,4.4274523984048,12.4337852460614));
#48200=CARTESIAN_POINT('Ctrl Pts',(-4.33286777243754,2.68170729374847,12.5131571361148));
#48201=CARTESIAN_POINT('Ctrl Pts',(-5.08776723741693,0.282704228193439,
12.5925290261682));
#48202=CARTESIAN_POINT('Ctrl Pts',(-4.60329786494335,-2.18516496159434,
12.6719009162216));
#48203=CARTESIAN_POINT('Ctrl Pts',(-2.99747532179655,-4.12073280351837,
12.751272806275));
#48204=CARTESIAN_POINT('Ctrl Pts',(-0.661474425059184,-5.05249925559264,
12.8306446963284));
#48205=CARTESIAN_POINT('Ctrl Pts',(1.83566017747378,-4.75348807252195,12.9100165863819));
#48206=CARTESIAN_POINT('Ctrl Pts',(3.885632023939,-3.29653771665232,12.9893884764353));
#48207=CARTESIAN_POINT('Ctrl Pts',(4.98907251007332,-1.03655806976862,13.0687603664887));
#48208=CARTESIAN_POINT('Ctrl Pts',(4.87718597587842,1.47592482852836,13.1481322565421));
#48209=CARTESIAN_POINT('Ctrl Pts',(3.5772277334276,3.62887570549998,13.2275041465955));
#48210=CARTESIAN_POINT('Ctrl Pts',(1.4058647331731,4.89784049299196,13.3068760366489));
#48211=CARTESIAN_POINT('Ctrl Pts',(-1.10796380425358,4.97370217757714,13.3862479267023));
#48212=CARTESIAN_POINT('Ctrl Pts',(-3.35189481140037,3.83798102080754,13.4656198167557));
#48213=CARTESIAN_POINT('Ctrl Pts',(-4.77931166178332,1.76733618259613,13.5449917068091));
#48214=CARTESIAN_POINT('Ctrl Pts',(-5.0424987701828,-0.733827837763376,
13.6243635968625));
#48215=CARTESIAN_POINT('Ctrl Pts',(-4.07734433954749,-3.0562330211441,13.7037354869159));
#48216=CARTESIAN_POINT('Ctrl Pts',(-2.11895785284703,-4.6341466054312,13.7831073769693));
#48217=CARTESIAN_POINT('Ctrl Pts',(0.355602076573349,-5.08319233414479,
13.8624792670227));
#48218=CARTESIAN_POINT('Ctrl Pts',(2.74353812725229,-4.29398366171607,13.9418511570761));
#48219=CARTESIAN_POINT('Ctrl Pts',(4.4631543628512,-2.45877007386494,14.0212230471295));
#48220=CARTESIAN_POINT('Ctrl Pts',(5.09555607468418,-0.024605538415575,
14.1005949371829));
#48221=CARTESIAN_POINT('Ctrl Pts',(4.48669160554615,2.41555285172843,14.1799668272363));
#48222=CARTESIAN_POINT('Ctrl Pts',(2.78487899242048,4.26728791392691,14.2593387172897));
#48223=CARTESIAN_POINT('Ctrl Pts',(0.404676020966283,5.07952108577437,14.3387106073431));
#48224=CARTESIAN_POINT('Ctrl Pts',(-2.07410513346011,4.65439416445642,14.4180824973965));
#48225=CARTESIAN_POINT('Ctrl Pts',(-4.0476388683295,3.09546712700361,14.4974543874499));
#48226=CARTESIAN_POINT('Ctrl Pts',(-5.03517673417046,0.782491149112972,
14.5768262775033));
#48227=CARTESIAN_POINT('Ctrl Pts',(-4.79615669274215,-1.72109794068678,
14.6561981675567));
#48228=CARTESIAN_POINT('Ctrl Pts',(-3.38880349707463,-3.80543138172091,
14.7355700576101));
#48229=CARTESIAN_POINT('Ctrl Pts',(-1.15594527050905,-4.96277016134733,
14.8149419476636));
#48230=CARTESIAN_POINT('Ctrl Pts',(1.35849866531108,-4.91118911457496,14.8943138377169));
#48231=CARTESIAN_POINT('Ctrl Pts',(3.54201533324722,-3.66325327022487,14.9736857277704));
#48232=CARTESIAN_POINT('Ctrl Pts',(4.86270490612231,-1.52295703772157,15.0530576178238));
#48233=CARTESIAN_POINT('Ctrl Pts',(4.99885032728073,0.988328158162469,15.1324295078772));
#48234=CARTESIAN_POINT('Ctrl Pts',(3.91728687348112,3.25885880234541,15.2118013979306));
#48235=CARTESIAN_POINT('Ctrl Pts',(1.8814810080689,4.73553865563863,15.291173287984));
#48236=CARTESIAN_POINT('Ctrl Pts',(-0.612649466321345,5.05865177435528,
15.3705451780374));
#48237=CARTESIAN_POINT('Ctrl Pts',(-2.95753988679226,4.14948851797474,15.4499170680908));
#48238=CARTESIAN_POINT('Ctrl Pts',(-4.58198013724412,2.22951904335266,15.5292889581442));
#48239=CARTESIAN_POINT('Ctrl Pts',(-5.09026016830427,-0.233556335273548,
15.6086608481976));
#48240=CARTESIAN_POINT('Ctrl Pts',(-4.35856408946536,-2.63973790759512,
15.688032738251));
#48241=CARTESIAN_POINT('Ctrl Pts',(-2.56513144595043,-4.40288516858759,
15.7674046283044));
#48242=CARTESIAN_POINT('Ctrl Pts',(-0.146838460024607,-5.09349934813251,
15.8467765183578));
#48243=CARTESIAN_POINT('Ctrl Pts',(2.3072240497427,-4.54334836074314,15.9261484084112));
#48244=CARTESIAN_POINT('Ctrl Pts',(4.19925188794477,-2.88644776920547,16.0055202984646));
#48245=CARTESIAN_POINT('Ctrl Pts',(5.06835126113318,-0.526414890137456,
16.084892188518));
#48246=CARTESIAN_POINT('Ctrl Pts',(4.70281148570858,1.96185149097663,16.1642640785714));
#48247=CARTESIAN_POINT('Ctrl Pts',(3.19167724187374,3.97221519135797,16.2436359686248));
#48248=CARTESIAN_POINT('Ctrl Pts',(0.90305748655408,5.01495606350291,16.3230078586782));
#48249=CARTESIAN_POINT('Ctrl Pts',(-1.60554507356452,4.83606473894038,16.4023797487316));
#48250=CARTESIAN_POINT('Ctrl Pts',(-3.72304040765551,3.47911874852373,16.481751638785));
#48251=CARTESIAN_POINT('Ctrl Pts',(-4.93361133910263,1.27466713166901,16.5611235288384));
#48252=CARTESIAN_POINT('Ctrl Pts',(-4.94236546898943,-1.24029057666156,
16.6404954188918));
#48253=CARTESIAN_POINT('Ctrl Pts',(-3.74717030983909,-3.45311624655429,
16.7198673089452));
#48254=CARTESIAN_POINT('Ctrl Pts',(-1.6391727584367,-4.82477044080732,16.7992391989986));
#48255=CARTESIAN_POINT('Ctrl Pts',(0.868123650569205,-5.02112123762451,
16.8786110890521));
#48256=CARTESIAN_POINT('Ctrl Pts',(3.16394705627606,-3.99433801030565,16.9579829791054));
#48257=CARTESIAN_POINT('Ctrl Pts',(4.68903996911093,-1.99454289389466,17.0373548691589));
#48258=CARTESIAN_POINT('Ctrl Pts',(5.07189311172224,0.491118473430398,17.1167267592122));
#48259=CARTESIAN_POINT('Ctrl Pts',(4.21924434286031,2.85714443596481,17.1960986492657));
#48260=CARTESIAN_POINT('Ctrl Pts',(2.33879694571596,4.52717639800277,17.275470539319));
#48261=CARTESIAN_POINT('Ctrl Pts',(-0.11137612465114,5.09439809707615,17.3548424293725));
#48262=CARTESIAN_POINT('Ctrl Pts',(-2.53441837980398,4.42063590960358,17.4342143194259));
#48263=CARTESIAN_POINT('Ctrl Pts',(-4.34008162116489,2.67001619606203,17.5135862094793));
#48264=CARTESIAN_POINT('Ctrl Pts',(-5.08851116459639,0.268987208843763,
17.5929580995327));
#48265=CARTESIAN_POINT('Ctrl Pts',(-4.59738955946409,-2.19756790530666,
17.6723299895861));
#48266=CARTESIAN_POINT('Ctrl Pts',(-2.98635609589589,-4.12879762624818,
17.7517018796395));
#48267=CARTESIAN_POINT('Ctrl Pts',(-0.647849003889666,-5.05426651218747,
17.8310737696929));
#48268=CARTESIAN_POINT('Ctrl Pts',(1.84846531944351,-4.7485175808327,17.9104456597463));
#48269=CARTESIAN_POINT('Ctrl Pts',(3.89451146459875,-3.28605855970652,17.9898175497997));
#48270=CARTESIAN_POINT('Ctrl Pts',(4.99183702504825,-1.02308842638974,18.0691894398531));
#48271=CARTESIAN_POINT('Ctrl Pts',(4.87321162956217,1.48903860109228,18.1485613299065));
#48272=CARTESIAN_POINT('Ctrl Pts',(3.5673892128293,3.63856219800459,18.2279332199599));
#48273=CARTESIAN_POINT('Ctrl Pts',(1.39273514199697,4.90150770362139,18.3073051100133));
#48274=CARTESIAN_POINT('Ctrl Pts',(-1.12151932172649,4.97089558679471,18.3866770000667));
#48275=CARTESIAN_POINT('Ctrl Pts',(-3.36194502775882,3.82855576883779,18.4660488901201));
#48276=CARTESIAN_POINT('Ctrl Pts',(-4.78459624359504,1.75515257798274,18.5454207801735));
#48277=CARTESIAN_POINT('Ctrl Pts',(-5.03948789886558,-0.748754766453475,
18.6247926702269));
#48278=CARTESIAN_POINT('Ctrl Pts',(-4.0710021077043,-3.06469899064074,18.7041645602803));
#48279=CARTESIAN_POINT('Ctrl Pts',(-2.10287077052062,-4.64454172754396,
18.7835364503337));
#48280=CARTESIAN_POINT('Ctrl Pts',(0.36273133865386,-5.07374792580598,18.8629083403871));
#48281=CARTESIAN_POINT('Ctrl Pts',(3.56709774791096,-4.04128406294332,18.968737527125));
#48282=CARTESIAN_POINT('Ctrl Pts',(5.77704085522352,-0.0189872057267309,
19.1010240105473));
#48283=CARTESIAN_POINT('Ctrl Pts',(3.14459942081972,4.8501664079131,19.2597677906541));
#48284=CARTESIAN_POINT('Ctrl Pts',(-2.36591519662263,5.26902047281295,19.418511570761));
#48285=CARTESIAN_POINT('Ctrl Pts',(-5.71123844601178,0.872727032859995,
19.5772553508678));
#48286=CARTESIAN_POINT('Ctrl Pts',(-3.83058845612596,-4.3254192567976,19.7359991309746));
#48287=CARTESIAN_POINT('Ctrl Pts',(1.55524717023751,-5.5639435857319,19.8947429110814));
#48288=CARTESIAN_POINT('Ctrl Pts',(5.51805139390222,-1.71188403765725,20.0534866911882));
#48289=CARTESIAN_POINT('Ctrl Pts',(4.43131449514919,3.70671199728542,20.212230471295));
#48290=CARTESIAN_POINT('Ctrl Pts',(-0.709818611660639,5.73400533709385,
20.3709742514018));
#48291=CARTESIAN_POINT('Ctrl Pts',(-5.20235975367858,2.51303602329798,20.5297180315086));
#48292=CARTESIAN_POINT('Ctrl Pts',(-4.93271294602024,-3.0047419943643,20.6884618116154));
#48293=CARTESIAN_POINT('Ctrl Pts',(-0.152720854580618,-5.77834717219765,
20.8472055917222));
#48294=CARTESIAN_POINT('Ctrl Pts',(4.77339715849037,-3.25411141853181,21.005949371829));
#48295=CARTESIAN_POINT('Ctrl Pts',(5.22808970274015,1.3127228499015,21.1382358552514));
#48296=CARTESIAN_POINT('Ctrl Pts',(3.1707451501151,3.97754537770267,21.2440650419892));
#48297=CARTESIAN_POINT('Ctrl Pts',(0.895150293052777,5.019216999618,21.3234369320426));
#48298=CARTESIAN_POINT('Ctrl Pts',(-1.62157688245131,4.83072732396133,21.402808822096));
#48299=CARTESIAN_POINT('Ctrl Pts',(-3.73081451079173,3.46959580775127,21.4821807121495));
#48300=CARTESIAN_POINT('Ctrl Pts',(-4.93787328845979,1.26108254025601,21.5615526022028));
#48301=CARTESIAN_POINT('Ctrl Pts',(-4.93855701420288,-1.25346250930809,
21.6409244922563));
#48302=CARTESIAN_POINT('Ctrl Pts',(-3.73808388472054,-3.46328419200818,
21.7202963823096));
#48303=CARTESIAN_POINT('Ctrl Pts',(-1.62603418385006,-4.82913054051807,
21.7996682723631));
#48304=CARTESIAN_POINT('Ctrl Pts',(0.881590795203928,-5.01878454751451,
21.8790401624164));
#48305=CARTESIAN_POINT('Ctrl Pts',(3.17473921804455,-3.98578203611947,21.9584120524699));
#48306=CARTESIAN_POINT('Ctrl Pts',(4.69438148876591,-1.98190041394297,22.0377839425233));
#48307=CARTESIAN_POINT('Ctrl Pts',(5.0705605156318,0.504793485523968,22.1171558325767));
#48308=CARTESIAN_POINT('Ctrl Pts',(4.21152107628908,2.86850718608746,22.1965277226301));
#48309=CARTESIAN_POINT('Ctrl Pts',(2.32658621700133,4.53346610033867,22.2758996126835));
#48310=CARTESIAN_POINT('Ctrl Pts',(-0.125111436169825,5.09407888617233,
22.3552715027369));
#48311=CARTESIAN_POINT('Ctrl Pts',(-2.54632610813663,4.41378735452051,22.4346433927903));
#48312=CARTESIAN_POINT('Ctrl Pts',(-4.34726461344783,2.6583059213356,22.5140152828437));
#48313=CARTESIAN_POINT('Ctrl Pts',(-5.08921736705482,0.255267617363269,
22.5933871728972));
#48314=CARTESIAN_POINT('Ctrl Pts',(-4.59144894277882,-2.20995361377114,
22.6727590629504));
#48315=CARTESIAN_POINT('Ctrl Pts',(-2.97521323819314,-4.13683487704257,
22.7521309530039));
#48316=CARTESIAN_POINT('Ctrl Pts',(-0.634222428965717,-5.05599240530685,
22.8315028430573));
#48317=CARTESIAN_POINT('Ctrl Pts',(1.8612636949988,-4.74352133023588,22.9108747331107));
#48318=CARTESIAN_POINT('Ctrl Pts',(3.90335003127195,-3.27553898237365,22.9902466231641));
#48319=CARTESIAN_POINT('Ctrl Pts',(4.99458897767401,-1.00964257616381,23.0696185132175));
#48320=CARTESIAN_POINT('Ctrl Pts',(4.86915708441603,1.5022005201609,23.1489904032709));
#48321=CARTESIAN_POINT('Ctrl Pts',(3.55760931370069,3.6481108983516,23.2283622933243));
#48322=CARTESIAN_POINT('Ctrl Pts',(1.37943578318338,4.90534953479997,23.3077341833777));
#48323=CARTESIAN_POINT('Ctrl Pts',(-1.13476524781216,4.96765588336336,23.3871060734311));
#48324=CARTESIAN_POINT('Ctrl Pts',(-3.37253997777701,3.81985225393738,23.4664779634845));
#48325=CARTESIAN_POINT('Ctrl Pts',(-4.78877143331127,1.74154107082816,23.545849853538));
#48326=CARTESIAN_POINT('Ctrl Pts',(-5.03846876789875,-0.76100566244534,
23.6252217435914));
#48327=CARTESIAN_POINT('Ctrl Pts',(-4.06080626285345,-3.07817310072711,
23.7045936336447));
#48328=CARTESIAN_POINT('Ctrl Pts',(-2.09394034074327,-4.64550438513341,
23.7839655236982));
#48329=CARTESIAN_POINT('Ctrl Pts',(0.383004813579298,-5.08120108394905,
23.8633374137515));
#48330=CARTESIAN_POINT('Ctrl Pts',(2.76665084304599,-4.27912844577405,23.942709303805));
#48331=CARTESIAN_POINT('Ctrl Pts',(4.47634685104287,-2.43466958989253,24.0220811938583));
#48332=CARTESIAN_POINT('Ctrl Pts',(5.0956146743416,0.00286938903386649,
24.1014530839118));
#48333=CARTESIAN_POINT('Ctrl Pts',(4.47360204192767,2.4397093911446,24.1808249739652));
#48334=CARTESIAN_POINT('Ctrl Pts',(2.76182985424755,4.28224158577674,24.2601968640186));
#48335=CARTESIAN_POINT('Ctrl Pts',(0.377282027280861,5.08162920869509,24.339568754072));
#48336=CARTESIAN_POINT('Ctrl Pts',(-2.09917086643256,4.64314320437055,24.4189406441253));
#48337=CARTESIAN_POINT('Ctrl Pts',(-4.06427038351852,3.07359779288466,24.4983125341788));
#48338=CARTESIAN_POINT('Ctrl Pts',(-5.03932263128953,0.755330762345285,
24.5776844242322));
#48339=CARTESIAN_POINT('Ctrl Pts',(-4.78680704042971,-1.74693317000509,
24.6570563142856));
#48340=CARTESIAN_POINT('Ctrl Pts',(-3.36823584993892,-3.82364804891321,
24.736428204339));
#48341=CARTESIAN_POINT('Ctrl Pts',(-1.12916986186658,-4.96893072660747,
24.8158000943924));
#48342=CARTESIAN_POINT('Ctrl Pts',(1.38495940518137,-4.90379287784174,24.8951719844458));
#48343=CARTESIAN_POINT('Ctrl Pts',(3.56171562668277,-3.64410193839515,24.9745438744992));
#48344=CARTESIAN_POINT('Ctrl Pts',(4.87084580524804,-1.49671583283838,25.0539157645526));
#48345=CARTESIAN_POINT('Ctrl Pts',(4.99344872708924,1.01526693667351,25.133287654606));
#48346=CARTESIAN_POINT('Ctrl Pts',(3.8996585918228,3.27993292766699,25.2126595446594));
#48347=CARTESIAN_POINT('Ctrl Pts',(1.85592025533624,4.7456145174892,25.2920314347128));
#48348=CARTESIAN_POINT('Ctrl Pts',(-0.639916147340462,5.05527491509063,
25.3714033247662));
#48349=CARTESIAN_POINT('Ctrl Pts',(-2.9798703929554,4.13348153303719,25.4507752148196));
#48350=CARTESIAN_POINT('Ctrl Pts',(-4.59393480667762,2.20478119884206,25.5301471048731));
#48351=CARTESIAN_POINT('Ctrl Pts',(-5.08892686999539,-0.260998955190596,
25.6095189949264));
#48352=CARTESIAN_POINT('Ctrl Pts',(-4.34426761193083,-2.66320034145021,
25.6888908849798));
#48353=CARTESIAN_POINT('Ctrl Pts',(-2.54135437947314,-4.41665201942651,
25.7682627750333));
#48354=CARTESIAN_POINT('Ctrl Pts',(-0.119372845368366,-5.09421704156391,
25.8476346650866));
#48355=CARTESIAN_POINT('Ctrl Pts',(2.33168764964084,-4.53084206823456,25.9270065551401));
#48356=CARTESIAN_POINT('Ctrl Pts',(4.21475419430065,-2.86376399593205,26.0063784451934));
#48357=CARTESIAN_POINT('Ctrl Pts',(5.07111594642898,-0.49907935305457,26.0857503352469));
#48358=CARTESIAN_POINT('Ctrl Pts',(4.69216507873193,1.98717991553359,26.1651222253003));
#48359=CARTESIAN_POINT('Ctrl Pts',(3.17021318378706,3.98936655524586,26.2444941153537));
#48360=CARTESIAN_POINT('Ctrl Pts',(0.876004374419533,5.01975233241337,26.3238660054071));
#48361=CARTESIAN_POINT('Ctrl Pts',(-1.63159716155383,4.82733755243831,26.4032378954604));
#48362=CARTESIAN_POINT('Ctrl Pts',(-3.74174524045176,3.4589940298197,26.4826097855139));
#48363=CARTESIAN_POINT('Ctrl Pts',(-4.94041246098821,1.2480472178904,26.5619816755672));
#48364=CARTESIAN_POINT('Ctrl Pts',(-4.93560614144543,-1.26692113381128,
26.6413535656207));
#48365=CARTESIAN_POINT('Ctrl Pts',(-3.72849709062547,-3.4732703015989,26.7207254556741));
#48366=CARTESIAN_POINT('Ctrl Pts',(-1.61313440141745,-4.8335385118705,26.8000973457275));
#48367=CARTESIAN_POINT('Ctrl Pts',(0.895184257363441,-5.01636743950643,
26.8794692357809));
#48368=CARTESIAN_POINT('Ctrl Pts',(3.18543801250735,-3.97722036241957,26.9588411258343));
#48369=CARTESIAN_POINT('Ctrl Pts',(4.69972611865188,-1.96923120847525,27.0382130158877));
#48370=CARTESIAN_POINT('Ctrl Pts',(5.06917134496014,0.51845830903431,27.1175849059411));
#48371=CARTESIAN_POINT('Ctrl Pts',(4.20377765205651,2.8798525300511,27.1969567959945));
#48372=CARTESIAN_POINT('Ctrl Pts',(2.31435302801598,4.53972104919287,27.2763286860479));
#48373=CARTESIAN_POINT('Ctrl Pts',(-0.138842870915707,5.09372356925338,
27.3557005761014));
#48374=CARTESIAN_POINT('Ctrl Pts',(-2.5582169538158,4.40690630260968,27.4350724661547));
#48375=CARTESIAN_POINT('Ctrl Pts',(-4.35441504928357,2.64657641517193,27.5144443562082));
#48376=CARTESIAN_POINT('Ctrl Pts',(-5.08988727708012,0.241546371095803,
27.5938162462615));
#48377=CARTESIAN_POINT('Ctrl Pts',(-4.58547423045432,-2.22232383432546,
27.6731881363149));
#48378=CARTESIAN_POINT('Ctrl Pts',(-2.96404981106488,-4.14484087273538,
27.7525600263683));
#48379=CARTESIAN_POINT('Ctrl Pts',(-0.620589418513009,-5.05768384899663,
27.8319319164217));
#48380=CARTESIAN_POINT('Ctrl Pts',(1.87404518273727,-4.73848623463559,27.9113038064751));
#48381=CARTESIAN_POINT('Ctrl Pts',(3.91216652560138,-3.26500386197866,27.9906756965286));
#48382=CARTESIAN_POINT('Ctrl Pts',(4.9972927622627,-0.99617377550726,28.0700475865819));
#48383=CARTESIAN_POINT('Ctrl Pts',(4.86508954335677,1.51532203768447,28.1494194766354));
#48384=CARTESIAN_POINT('Ctrl Pts',(3.54776128038217,3.65768875660473,28.2287913666887));
#48385=CARTESIAN_POINT('Ctrl Pts',(1.36620622234286,4.90905059057282,28.3081632567422));
#48386=CARTESIAN_POINT('Ctrl Pts',(-1.148153647413,4.96457856667651,28.3875351467955));
#48387=CARTESIAN_POINT('Ctrl Pts',(-3.382825830054,3.81074619284609,28.466907036849));
#48388=CARTESIAN_POINT('Ctrl Pts',(-4.79344912825184,1.72862448138202,28.5462789269024));
#48389=CARTESIAN_POINT('Ctrl Pts',(-5.03639882892723,-0.774586327501372,
28.6256508169557));
#48390=CARTESIAN_POINT('Ctrl Pts',(-4.05249292275565,-3.08910962152317,
28.7050227070092));
#48391=CARTESIAN_POINT('Ctrl Pts',(-2.0814087106417,-4.65113264937009,28.7843945970626));
#48392=CARTESIAN_POINT('Ctrl Pts',(0.39670205626447,-5.08015005893792,28.863766487116));
#48393=CARTESIAN_POINT('Ctrl Pts',(2.77817708034974,-4.27165415886996,28.9431383771694));
#48394=CARTESIAN_POINT('Ctrl Pts',(4.48289431705251,-2.42259276084734,29.0225102672228));
#48395=CARTESIAN_POINT('Ctrl Pts',(5.09558842083954,0.016606871399571,29.1018821572762));
#48396=CARTESIAN_POINT('Ctrl Pts',(4.46700846420369,2.45176110653224,29.1812540473296));
#48397=CARTESIAN_POINT('Ctrl Pts',(2.75027513324334,4.28967176299481,29.260625937383));
#48398=CARTESIAN_POINT('Ctrl Pts',(0.363580867455653,5.08262787301922,29.3399978274364));
#48399=CARTESIAN_POINT('Ctrl Pts',(-2.11168089287163,4.6374670833821,29.4193697174898));
#48400=CARTESIAN_POINT('Ctrl Pts',(-4.07254186182172,3.0626295770924,29.4987416075432));
#48401=CARTESIAN_POINT('Ctrl Pts',(-5.04134064765058,0.741742284838609,
29.5781134975966));
#48402=CARTESIAN_POINT('Ctrl Pts',(-4.78208001053002,-1.75983178618322,
29.6574853876501));
#48403=CARTESIAN_POINT('Ctrl Pts',(-3.35791526779889,-3.8327147294124,29.7368572777034));
#48404=CARTESIAN_POINT('Ctrl Pts',(-1.11576979845131,-4.97195684812685,
29.8162291677569));
#48405=CARTESIAN_POINT('Ctrl Pts',(1.3981747240844,-4.90004128387741,29.8956010578102));
#48406=CARTESIAN_POINT('Ctrl Pts',(3.57152697864042,-3.63448650893289,29.9749729478637));
#48407=CARTESIAN_POINT('Ctrl Pts',(4.87486316664055,-1.48357886521172,30.054344837917));
#48408=CARTESIAN_POINT('Ctrl Pts',(4.99069347757362,1.02872530622892,30.1337167279705));
#48409=CARTESIAN_POINT('Ctrl Pts',(3.89080190408237,3.29043427011703,30.2130886180238));
#48410=CARTESIAN_POINT('Ctrl Pts',(1.84311959890063,4.75060072905731,30.2924605080773));
#48411=CARTESIAN_POINT('Ctrl Pts',(-0.653542560897256,5.05353136567563,
30.3718323981307));
#48412=CARTESIAN_POINT('Ctrl Pts',(-2.99100319945254,4.12543294741732,30.4512042881841));
#48413=CARTESIAN_POINT('Ctrl Pts',(-4.59986207909447,2.19238819465906,30.5305761782375));
#48414=CARTESIAN_POINT('Ctrl Pts',(-5.08820473789096,-0.274717469549192,
30.6099480682909));
#48415=CARTESIAN_POINT('Ctrl Pts',(-4.33707198508738,-2.67490256625206,
30.6893199583443));
#48416=CARTESIAN_POINT('Ctrl Pts',(-2.52943809666249,-4.42348731861233,
30.7686918483976));
#48417=CARTESIAN_POINT('Ctrl Pts',(-0.10563868670687,-5.09452035138171,
30.8480637384511));
#48418=CARTESIAN_POINT('Ctrl Pts',(2.34389407350322,-4.52453950308404,30.9274356285044));
#48419=CARTESIAN_POINT('Ctrl Pts',(4.22245942552948,-2.85239084673345,31.006807518558));
#48420=CARTESIAN_POINT('Ctrl Pts',(5.07244300775219,-0.485406093778655,
31.0861794086112));
#48421=CARTESIAN_POINT('Ctrl Pts',(4.68679070094865,1.99982250919246,31.1655512986648));
#48422=CARTESIAN_POINT('Ctrl Pts',(3.15944655342927,3.99789877545637,31.2449231887181));
#48423=CARTESIAN_POINT('Ctrl Pts',(0.862468218810821,5.02209574921795,31.3242950787715));
#48424=CARTESIAN_POINT('Ctrl Pts',(-1.64460546486892,4.82292131469039,31.4036669688249));
#48425=CARTESIAN_POINT('Ctrl Pts',(-3.75105689757904,3.44889392325951,31.4830388588783));
#48426=CARTESIAN_POINT('Ctrl Pts',(-4.94375917286251,1.23472360611981,31.5624107489317));
#48427=CARTESIAN_POINT('Ctrl Pts',(-4.93217265646195,-1.28022264845634,
31.6417826389851));
#48428=CARTESIAN_POINT('Ctrl Pts',(-3.7191197981263,-3.48330949959324,31.7211545290385));
#48429=CARTESIAN_POINT('Ctrl Pts',(-1.60009758909914,-4.83786986680406,
31.8005264190919));
#48430=CARTESIAN_POINT('Ctrl Pts',(0.908704850876668,-5.01393584290474,
31.8798983091453));
#48431=CARTESIAN_POINT('Ctrl Pts',(3.196148800563,-3.96861814583255,31.9592701991988));
#48432=CARTESIAN_POINT('Ctrl Pts',(4.70501797698753,-1.9565538528228,32.0386420892521));
#48433=CARTESIAN_POINT('Ctrl Pts',(5.06775518859854,0.532122627976042,32.1180139793055));
#48434=CARTESIAN_POINT('Ctrl Pts',(4.19599845355282,2.89117521443338,32.1973858693589));
#48435=CARTESIAN_POINT('Ctrl Pts',(2.30210578290666,4.54594391816259,32.2767577594124));
#48436=CARTESIAN_POINT('Ctrl Pts',(-0.152574760830862,5.09333074570355,
32.3561296494657));
#48437=CARTESIAN_POINT('Ctrl Pts',(-2.57008843054848,4.39999347748749,32.4355015395192));
#48438=CARTESIAN_POINT('Ctrl Pts',(-4.3615342473787,2.63482753737587,32.5148734295725));
#48439=CARTESIAN_POINT('Ctrl Pts',(-5.09051997563981,0.227823441251348,
32.594245319626));
#48440=CARTESIAN_POINT('Ctrl Pts',(-4.57946630550992,-2.23467794088343,
32.6736172096794));
#48441=CARTESIAN_POINT('Ctrl Pts',(-2.95286477983452,-4.1528167229947,32.7529890997328));
#48442=CARTESIAN_POINT('Ctrl Pts',(-0.60695192984675,-5.05933854348835,
32.8323609897862));
#48443=CARTESIAN_POINT('Ctrl Pts',(1.88681306678638,-4.73341669344416,32.9117328798396));
#48444=CARTESIAN_POINT('Ctrl Pts',(3.92095457674023,-3.25444501411708,32.991104769893));
#48445=CARTESIAN_POINT('Ctrl Pts',(4.99996023068588,-0.982697732942914,
33.0704766599464));
#48446=CARTESIAN_POINT('Ctrl Pts',(4.8609866396607,1.52843254081155,33.1498485499997));
#48447=CARTESIAN_POINT('Ctrl Pts',(3.53788746282564,3.66724003075238,33.2292204400532));
#48448=CARTESIAN_POINT('Ctrl Pts',(1.35296673102733,4.91271596650007,33.3085923301066));
#48449=CARTESIAN_POINT('Ctrl Pts',(-1.16153370170815,4.96146516692072,33.38796422016));
#48450=CARTESIAN_POINT('Ctrl Pts',(-3.39308709571883,3.80161243469636,33.4673361102134));
#48451=CARTESIAN_POINT('Ctrl Pts',(-4.79809198368328,1.71569532810634,33.5467080002668));
#48452=CARTESIAN_POINT('Ctrl Pts',(-5.03429228481892,-0.788161362783202,
33.6260798903202));
#48453=CARTESIAN_POINT('Ctrl Pts',(-4.04415012858963,-3.10002369026433,
33.7054517803737));
#48454=CARTESIAN_POINT('Ctrl Pts',(-2.06886195261037,-4.65672710858312,
33.784823670427));
#48455=CARTESIAN_POINT('Ctrl Pts',(0.41039641567654,-5.07906211074165,33.8641955604805));
#48456=CARTESIAN_POINT('Ctrl Pts',(2.78968312550164,-4.26414882503682,33.9435674505338));
#48457=CARTESIAN_POINT('Ctrl Pts',(4.48940920081343,-2.41049832408638,34.0229393405872));
#48458=CARTESIAN_POINT('Ctrl Pts',(5.09552513194581,0.0303442330639926,
34.1023112306406));
#48459=CARTESIAN_POINT('Ctrl Pts',(4.46038241968974,2.46379500220581,34.181683120694));
#48460=CARTESIAN_POINT('Ctrl Pts',(2.73870042288625,4.29707076232801,34.2610550107475));
#48461=CARTESIAN_POINT('Ctrl Pts',(0.349877065078239,5.0835895961519,34.3404269008008));
#48462=CARTESIAN_POINT('Ctrl Pts',(-2.1241755713431,4.63175725668789,34.4197987908543));
#48463=CARTESIAN_POINT('Ctrl Pts',(-4.08078374036812,3.05163910171546,34.4991706809076));
#48464=CARTESIAN_POINT('Ctrl Pts',(-5.04332202290104,0.728148416253786,
34.5785425709611));
#48465=CARTESIAN_POINT('Ctrl Pts',(-4.77731822385925,-1.77271761167814,
34.6579144610144));
#48466=CARTESIAN_POINT('Ctrl Pts',(-3.3475702798999,-3.84175355324914,34.7372863510679));
#48467=CARTESIAN_POINT('Ctrl Pts',(-1.10236162547809,-4.97494683282594,
34.8166582411212));
#48468=CARTESIAN_POINT('Ctrl Pts',(1.41137988087415,-4.8962540757844,34.8960301311747));
#48469=CARTESIAN_POINT('Ctrl Pts',(3.58131237228184,-3.62484466355631,34.9754020212281));
#48470=CARTESIAN_POINT('Ctrl Pts',(4.87884509690211,-1.47043111474347,35.0547739112815));
#48471=CARTESIAN_POINT('Ctrl Pts',(4.98790195505749,1.04217619887681,35.1341458013349));
#48472=CARTESIAN_POINT('Ctrl Pts',(3.88191693749454,3.3009116972686,35.2135176913883));
#48473=CARTESIAN_POINT('Ctrl Pts',(1.8303055464353,4.75555241264984,35.2928895814417));
#48474=CARTESIAN_POINT('Ctrl Pts',(-0.667164224422912,5.05175108654629,
35.3722614714951));
#48475=CARTESIAN_POINT('Ctrl Pts',(-3.00211426695468,4.11735437762148,35.4516333615485));
#48476=CARTESIAN_POINT('Ctrl Pts',(-4.60575591912355,2.17997925591738,35.5310052516019));
#48477=CARTESIAN_POINT('Ctrl Pts',(-5.08744562406171,-0.288433987225976,
35.6103771416553));
#48478=CARTESIAN_POINT('Ctrl Pts',(-4.32984483584829,-2.68658534951887,
35.6897490317088));
#48479=CARTESIAN_POINT('Ctrl Pts',(-2.51750342957125,-4.43029046732475,
35.7691209217621));
#48480=CARTESIAN_POINT('Ctrl Pts',(-0.0919037602499935,-5.09478663357195,
35.8484928118156));
#48481=CARTESIAN_POINT('Ctrl Pts',(2.35608346164268,-4.51820405299999,35.9278647018689));
#48482=CARTESIAN_POINT('Ctrl Pts',(4.23013396738149,-2.84099696599223,36.0072365919223));
#48483=CARTESIAN_POINT('Ctrl Pts',(5.07373320190884,-0.471729306508876,
36.0866084819757));
#48484=CARTESIAN_POINT('Ctrl Pts',(4.68138225896918,2.01245056788487,36.1659803720291));
#48485=CARTESIAN_POINT('Ctrl Pts',(3.14865695980852,4.00640193842567,36.2453522620825));
#48486=CARTESIAN_POINT('Ctrl Pts',(0.84892579467244,5.02440266478627,36.3247241521359));
#48487=CARTESIAN_POINT('Ctrl Pts',(-1.65760181498048,4.81847002333159,36.4040960421893));
#48488=CARTESIAN_POINT('Ctrl Pts',(-3.76034129154353,3.43876874969578,36.4834679322427));
#48489=CARTESIAN_POINT('Ctrl Pts',(-4.94706995286084,1.22139102021962,36.5628398222961));
#48490=CARTESIAN_POINT('Ctrl Pts',(-4.92870332381484,-1.2935148582789,36.6422117123495));
#48491=CARTESIAN_POINT('Ctrl Pts',(-3.70971547458727,-3.49332338044723,
36.721583602403));
#48492=CARTESIAN_POINT('Ctrl Pts',(-1.58704914706622,-4.84216605947875,
36.8009554924563));
#48493=CARTESIAN_POINT('Ctrl Pts',(0.922218839806455,-5.01146780437405,
36.8803273825098));
#48494=CARTESIAN_POINT('Ctrl Pts',(3.20683635859905,-3.95998708481968,36.9596992725631));
#48495=CARTESIAN_POINT('Ctrl Pts',(4.71027563864883,-1.94386227668601,37.0390711626166));
#48496=CARTESIAN_POINT('Ctrl Pts',(5.06630219914206,0.545783079382256,37.1184430526699));
#48497=CARTESIAN_POINT('Ctrl Pts',(4.18818875799396,2.90247688538333,37.1978149427234));
#48498=CARTESIAN_POINT('Ctrl Pts',(2.28984180579711,4.55213374662869,37.2771868327768));
#48499=CARTESIAN_POINT('Ctrl Pts',(-0.1663055418131,5.0929009031723,37.3565587228302));
#48500=CARTESIAN_POINT('Ctrl Pts',(-2.58194122754862,4.39304867264833,37.4359306128836));
#48501=CARTESIAN_POINT('Ctrl Pts',(-4.36862174528344,2.62305950931498,37.515302502937));
#48502=CARTESIAN_POINT('Ctrl Pts',(-5.09111567564704,0.214098855557291,
37.5946743929904));
#48503=CARTESIAN_POINT('Ctrl Pts',(-4.57342509641719,-2.24701580551625,
37.6740462830439));
#48504=CARTESIAN_POINT('Ctrl Pts',(-2.94165828680345,-4.16076239004767,
37.7534181730971));
#48505=CARTESIAN_POINT('Ctrl Pts',(-0.593310029777194,-5.06095646606148,
37.8327900631507));
#48506=CARTESIAN_POINT('Ctrl Pts',(1.89956723723832,-4.72831274916718,37.912161953204));
#48507=CARTESIAN_POINT('Ctrl Pts',(3.92971412987383,-3.2438625125424,37.9915338432574));
#48508=CARTESIAN_POINT('Ctrl Pts',(5.00259135876467,-0.969214547985126,
38.0709057333108));
#48509=CARTESIAN_POINT('Ctrl Pts',(4.85684840567486,1.54153193505625,38.1502776233642));
#48510=CARTESIAN_POINT('Ctrl Pts',(3.52798793147795,3.67676465100168,38.2296495134176));
#48511=CARTESIAN_POINT('Ctrl Pts',(1.3397174061215,4.91634563604017,38.309021403471));
#48512=CARTESIAN_POINT('Ctrl Pts',(-1.17490531372475,4.95831570685867,38.3883932935245));
#48513=CARTESIAN_POINT('Ctrl Pts',(-3.40332370018554,3.79245104545026,38.4677651835778));
#48514=CARTESIAN_POINT('Ctrl Pts',(-4.80269996560014,1.70275370586069,38.5471370736313));
#48515=CARTESIAN_POINT('Ctrl Pts',(-5.03214915152033,-0.801730671351773,
38.6265089636846));
#48516=CARTESIAN_POINT('Ctrl Pts',(-4.03577793971505,-3.11091522434137,
38.705880853738));
#48517=CARTESIAN_POINT('Ctrl Pts',(-2.05630016029208,-4.6622877283261,38.7852527437914));
#48518=CARTESIAN_POINT('Ctrl Pts',(0.424087796933226,-5.0779372355256,38.8646246338449));
#48519=CARTESIAN_POINT('Ctrl Pts',(2.80116888608276,-4.2566125209993,38.9439965238982));
#48520=CARTESIAN_POINT('Ctrl Pts',(4.49589147158116,-2.39838632564053,39.0233684139517));
#48521=CARTESIAN_POINT('Ctrl Pts',(5.09542477676094,0.0440812951169324,
39.1027403040051));
#48522=CARTESIAN_POINT('Ctrl Pts',(4.45372401575944,2.47581113999364,39.1821121940585));
#48523=CARTESIAN_POINT('Ctrl Pts',(2.72710569549243,4.30443824810521,39.2614840841118));
#48524=CARTESIAN_POINT('Ctrl Pts',(0.336170930870647,5.08451490337722,39.3408559741653));
#48525=CARTESIAN_POINT('Ctrl Pts',(-2.1366552096739,4.62601276074587,39.4202278642187));
#48526=CARTESIAN_POINT('Ctrl Pts',(-4.08899520654064,3.04062834435872,39.4995997542721));
#48527=CARTESIAN_POINT('Ctrl Pts',(-5.04526816392185,0.714545672092809,
39.5789716443255));
#48528=CARTESIAN_POINT('Ctrl Pts',(-4.77251903131803,-1.78558378675053,
39.6583435343789));
#48529=CARTESIAN_POINT('Ctrl Pts',(-3.33720602914116,-3.85077723115716,
39.7377154244323));
#48530=CARTESIAN_POINT('Ctrl Pts',(-1.08893586889047,-4.97787652885981,
39.8170873144857));
#48531=CARTESIAN_POINT('Ctrl Pts',(1.42455668503583,-4.8924768895782,39.8964592045391));
#48532=CARTESIAN_POINT('Ctrl Pts',(3.59110607910284,-3.61508997874913,39.9758310945925));
#48533=CARTESIAN_POINT('Ctrl Pts',(4.88272528059762,-1.45743906270703,40.0552029846459));
#48534=CARTESIAN_POINT('Ctrl Pts',(4.98521092249161,1.05595859527154,40.1345748746994));
#48535=CARTESIAN_POINT('Ctrl Pts',(4.2435173595031,2.5590120913109,40.1874894680683));
#48536=CARTESIAN_POINT('Ctrl Pts',(3.71544298812202,3.17665283523806,40.2139467647527));
#48537=CARTESIAN_POINT('Ctrl Pts',(1.21713437249832,-4.5428082122986,-0.213946764752702));
#48538=CARTESIAN_POINT('Ctrl Pts',(1.97231308274437,-4.34047654372165,-0.187489468068234));
#48539=CARTESIAN_POINT('Ctrl Pts',(3.37906911267772,-3.55219315325666,-0.134574874699299));
#48540=CARTESIAN_POINT('Ctrl Pts',(4.66642692152752,-1.5028536385038,-0.055202984645895));
#48541=CARTESIAN_POINT('Ctrl Pts',(4.81689062664967,0.911851793295018,0.0241689054075086));
#48542=CARTESIAN_POINT('Ctrl Pts',(3.79405383067521,3.10479958283122,0.103540795460912));
#48543=CARTESIAN_POINT('Ctrl Pts',(1.84695009786499,4.54123256689918,0.182912685514316));
#48544=CARTESIAN_POINT('Ctrl Pts',(-0.550043424514128,4.8715330414348,0.26228457556772));
#48545=CARTESIAN_POINT('Ctrl Pts',(-2.81305984991034,4.01508502497055,0.341656465621123));
#48546=CARTESIAN_POINT('Ctrl Pts',(-4.39081462818011,2.18059968579164,0.421028355674527));
#48547=CARTESIAN_POINT('Ctrl Pts',(-4.89898012125377,-0.18509000454136,
0.500400245727931));
#48548=CARTESIAN_POINT('Ctrl Pts',(-4.21376307902768,-2.5056841854766,0.579772135781334));
#48549=CARTESIAN_POINT('Ctrl Pts',(-2.50208364241389,-4.21590347870479,
0.659144025834738));
#48550=CARTESIAN_POINT('Ctrl Pts',(-0.180901657890204,-4.89913577411436,
0.738515915888141));
#48551=CARTESIAN_POINT('Ctrl Pts',(2.18434729950923,-4.38895062645432,0.817887805941546));
#48552=CARTESIAN_POINT('Ctrl Pts',(4.01749423301245,-2.8096261920884,0.897259695994948));
#48553=CARTESIAN_POINT('Ctrl Pts',(4.87198838803769,-0.545883369388664,
0.976631586048353));
#48554=CARTESIAN_POINT('Ctrl Pts',(4.53967699589134,1.85083561019003,1.05600347610176));
#48555=CARTESIAN_POINT('Ctrl Pts',(3.10151031466513,3.79669503846566,1.13537536615516));
#48556=CARTESIAN_POINT('Ctrl Pts',(0.907822597135906,4.81768800868641,1.21474725620856));
#48557=CARTESIAN_POINT('Ctrl Pts',(-1.50700870159448,4.66510281756135,1.29411914626197));
#48558=CARTESIAN_POINT('Ctrl Pts',(-3.55473601316185,3.37610891998462,1.37349103631537));
#48559=CARTESIAN_POINT('Ctrl Pts',(-4.73653750187219,1.26470235504102,1.45286292636877));
#48560=CARTESIAN_POINT('Ctrl Pts',(-4.76452893838759,-1.15478290032736,
1.53223481642218));
#48561=CARTESIAN_POINT('Ctrl Pts',(-3.63189167208734,-3.29296559930584,
1.61160670647558));
#48562=CARTESIAN_POINT('Ctrl Pts',(-1.61453363327375,-4.62898916605748,
1.69097859652899));
#48563=CARTESIAN_POINT('Ctrl Pts',(0.796121224764031,-4.8374012186294,1.77035048658239));
#48564=CARTESIAN_POINT('Ctrl Pts',(3.01284271470348,-3.86743304144296,1.8497223766358));
#48565=CARTESIAN_POINT('Ctrl Pts',(4.49564238811846,-1.95536673594104,1.92909426668919));
#48566=CARTESIAN_POINT('Ctrl Pts',(4.88331352674298,0.433022578391154,2.0084661567426));
#48567=CARTESIAN_POINT('Ctrl Pts',(4.08142029927371,2.71592855106099,2.087838046796));
#48568=CARTESIAN_POINT('Ctrl Pts',(2.28530212097744,4.33724034032234,2.16720993684941));
#48569=CARTESIAN_POINT('Ctrl Pts',(-0.067510595561391,4.90200998298708,
2.24658182690281));
#48570=CARTESIAN_POINT('Ctrl Pts',(-2.4038778804521,4.27266084421796,2.32595371695622));
#48571=CARTESIAN_POINT('Ctrl Pts',(-4.15466583455893,2.60250098116813,2.40532560700962));
#48572=CARTESIAN_POINT('Ctrl Pts',(-4.8933863875636,0.298377639645852,2.48469749706302));
#48573=CARTESIAN_POINT('Ctrl Pts',(-4.44008884788507,-2.07842983444745,
2.56406938711643));
#48574=CARTESIAN_POINT('Ctrl Pts',(-2.90519549283157,-3.94893640139523,
2.64344127716983));
#48575=CARTESIAN_POINT('Ctrl Pts',(-0.662602946265526,-4.85749080178588,
2.72281316722323));
#48576=CARTESIAN_POINT('Ctrl Pts',(1.7413982113641,-4.58277119473486,2.80218505727664));
#48577=CARTESIAN_POINT('Ctrl Pts',(3.72119861922498,-3.19169866843848,2.88155694733003));
#48578=CARTESIAN_POINT('Ctrl Pts',(4.79452328017608,-1.02313541121562,2.96092883738345));
#48579=CARTESIAN_POINT('Ctrl Pts',(4.69991268257356,1.39466136750753,3.04030072743684));
#48580=CARTESIAN_POINT('Ctrl Pts',(3.46041375857639,3.47272172413642,3.11967261749026));
#48581=CARTESIAN_POINT('Ctrl Pts',(1.37796570248595,4.70483475550482,3.19904450754365));
#48582=CARTESIAN_POINT('Ctrl Pts',(-1.04015174865471,4.79086045440737,3.27841639759706));
#48583=CARTESIAN_POINT('Ctrl Pts',(-3.20489053615995,3.70984315100601,3.35778828765046));
#48584=CARTESIAN_POINT('Ctrl Pts',(-4.5889250829615,1.72511626761812,3.43716017770387));
#48585=CARTESIAN_POINT('Ctrl Pts',(-4.85510763696699,-0.679845120081458,
3.51653206775727));
#48586=CARTESIAN_POINT('Ctrl Pts',(-3.9385967172058,-2.91919774134084,3.59590395781068));
#48587=CARTESIAN_POINT('Ctrl Pts',(-2.06265235506924,-4.44744025434419,
3.67527584786408));
#48588=CARTESIAN_POINT('Ctrl Pts',(0.315749555158651,-4.89229616563132,
3.75464773791748));
#48589=CARTESIAN_POINT('Ctrl Pts',(2.61723557264967,-4.14539955988454,3.83401962797088));
#48590=CARTESIAN_POINT('Ctrl Pts',(4.2811687977959,-2.38869279703619,3.91339151802429));
#48591=CARTESIAN_POINT('Ctrl Pts',(4.90221878000547,-0.0501057561116431,
3.99276340807769));
#48592=CARTESIAN_POINT('Ctrl Pts',(4.32909911828292,2.3006869360945,4.0721352981311));
#48593=CARTESIAN_POINT('Ctrl Pts',(2.701420493645,4.09103738315217,4.1515071881845));
#48594=CARTESIAN_POINT('Ctrl Pts',(0.415681816248014,4.88482017903163,4.2308790782379));
#48595=CARTESIAN_POINT('Ctrl Pts',(-1.97131603149091,4.48867159166503,4.31025096829131));
#48596=CARTESIAN_POINT('Ctrl Pts',(-3.87810565739265,2.9990925400749,4.38962285834471));
#48597=CARTESIAN_POINT('Ctrl Pts',(-4.84019732919483,0.778941184101248,
4.46899474839812));
#48598=CARTESIAN_POINT('Ctrl Pts',(-4.62322764520021,-1.63095852016239,
4.54836663845152));
#48599=CARTESIAN_POINT('Ctrl Pts',(-3.28004994017564,-3.64356033897994,
4.62773852850492));
#48600=CARTESIAN_POINT('Ctrl Pts',(-1.13785932999167,-4.76859892410598,
4.70711041855833));
#48601=CARTESIAN_POINT('Ctrl Pts',(1.28151129436936,-4.73201736643448,4.78648230861172));
#48602=CARTESIAN_POINT('Ctrl Pts',(3.38870860399915,-3.54272685244233,4.86585419866514));
#48603=CARTESIAN_POINT('Ctrl Pts',(4.67042399847401,-1.4904359188881,4.94522608871853));
#48604=CARTESIAN_POINT('Ctrl Pts',(4.81443444472878,0.924921905483315,5.02459797877194));
#48605=CARTESIAN_POINT('Ctrl Pts',(3.78565931681752,3.1149708009589,5.10396986882535));
#48606=CARTESIAN_POINT('Ctrl Pts',(1.83470595874426,4.54621970419184,5.18334175887875));
#48607=CARTESIAN_POINT('Ctrl Pts',(-0.563177709826337,4.87001955037026,
5.26271364893215));
#48608=CARTESIAN_POINT('Ctrl Pts',(-2.82387253485596,4.00749341368393,5.34208553898556));
#48609=CARTESIAN_POINT('Ctrl Pts',(-4.39667826093048,2.1687507518604,5.42145742903895));
#48610=CARTESIAN_POINT('Ctrl Pts',(-4.89846289452463,-0.198294792667946,
5.50082931909237));
#48611=CARTESIAN_POINT('Ctrl Pts',(-4.20699280957627,-2.51703616462048,
5.58020120914576));
#48612=CARTESIAN_POINT('Ctrl Pts',(-2.49070858823577,-4.2226330982365,5.65957309919917));
#48613=CARTESIAN_POINT('Ctrl Pts',(-0.16769326789098,-4.89960595576194,
5.73894498925257));
#48614=CARTESIAN_POINT('Ctrl Pts',(2.19617176132931,-4.38304564755759,5.81831687930597));
#48615=CARTESIAN_POINT('Ctrl Pts',(4.0250542106335,-2.7987851213152,5.89768876935939));
#48616=CARTESIAN_POINT('Ctrl Pts',(4.87344236353376,-0.532746734526196,
5.97706065941277));
#48617=CARTESIAN_POINT('Ctrl Pts',(4.53467074385888,1.86306757757847,6.05643254946619));
#48618=CARTESIAN_POINT('Ctrl Pts',(3.09126336830344,3.80504275161517,6.13580443951959));
#48619=CARTESIAN_POINT('Ctrl Pts',(0.894831078624676,4.82011793367768,6.215176329573));
#48620=CARTESIAN_POINT('Ctrl Pts',(-1.51958008113206,4.6610230562464,6.2945482196264));
#48621=CARTESIAN_POINT('Ctrl Pts',(-3.56382489665849,3.36651327931302,6.3739201096798));
#48622=CARTESIAN_POINT('Ctrl Pts',(-4.73992985575151,1.25192831918974,6.45329199973321));
#48623=CARTESIAN_POINT('Ctrl Pts',(-4.76139839364024,-1.16762360839183,
6.53266388978661));
#48624=CARTESIAN_POINT('Ctrl Pts',(-3.62300082201479,-3.30274500946015,
6.61203577984002));
#48625=CARTESIAN_POINT('Ctrl Pts',(-1.60204826952283,-4.63332503672608,
6.69140766989341));
#48626=CARTESIAN_POINT('Ctrl Pts',(0.809159695351183,-4.83523734073654,
6.77077955994682));
#48627=CARTESIAN_POINT('Ctrl Pts',(3.02325814948227,-3.8592965311599,6.85015145000022));
#48628=CARTESIAN_POINT('Ctrl Pts',(4.50089761026788,-1.94323962900068,6.92952334005363));
#48629=CARTESIAN_POINT('Ctrl Pts',(4.8821283757601,0.446186145495144,7.00889523010703));
#48630=CARTESIAN_POINT('Ctrl Pts',(4.07408347532503,2.72692196256463,7.08826712016044));
#48631=CARTESIAN_POINT('Ctrl Pts',(2.27360085813158,4.34338562549276,7.16763901021384));
#48632=CARTESIAN_POINT('Ctrl Pts',(-0.0807258955725768,4.90181016397186,
7.24701090026724));
#48633=CARTESIAN_POINT('Ctrl Pts',(-2.41538799979899,4.26616459648018,7.32638279032065));
#48634=CARTESIAN_POINT('Ctrl Pts',(-4.16166693364502,2.59129077628108,7.40575468037405));
#48635=CARTESIAN_POINT('Ctrl Pts',(-4.89417301414864,0.285184258704783,
7.48512657042745));
#48636=CARTESIAN_POINT('Ctrl Pts',(-4.43446938147388,-2.09039251304738,
7.56449846048085));
#48637=CARTESIAN_POINT('Ctrl Pts',(-2.89453882300355,-3.95675429562653,
7.64387035053426));
#48638=CARTESIAN_POINT('Ctrl Pts',(-0.649505014202585,-4.85925948991814,
7.72324224058766));
#48639=CARTESIAN_POINT('Ctrl Pts',(1.75374677840318,-4.57805982825413,7.80261413064107));
#48640=CARTESIAN_POINT('Ctrl Pts',(3.72978973764259,-3.18165492579096,7.88198602069447));
#48641=CARTESIAN_POINT('Ctrl Pts',(4.79726417254181,-1.01020592587881,7.96135791074788));
#48642=CARTESIAN_POINT('Ctrl Pts',(4.69613567357394,1.40732700152449,8.04072980080128));
#48643=CARTESIAN_POINT('Ctrl Pts',(3.45103891924351,3.48203818642192,8.12010169085468));
#48644=CARTESIAN_POINT('Ctrl Pts',(1.36527672293039,4.70853257646778,8.19947358090808));
#48645=CARTESIAN_POINT('Ctrl Pts',(-1.05306386109979,4.78803885304614,8.2788454709615));
#48646=CARTESIAN_POINT('Ctrl Pts',(-3.21488041948337,3.7011894631667,8.35821736101489));
#48647=CARTESIAN_POINT('Ctrl Pts',(-4.5935592236979,1.7127385125038,8.4375892510683));
#48648=CARTESIAN_POINT('Ctrl Pts',(-4.85325716869052,-0.692931748722623,
8.51696114112171));
#48649=CARTESIAN_POINT('Ctrl Pts',(-3.93071240989269,-2.92980536973865,
8.59633303117509));
#48650=CARTESIAN_POINT('Ctrl Pts',(-2.05065480852931,-4.45298488770055,
8.67570492122852));
#48651=CARTESIAN_POINT('Ctrl Pts',(0.328937765144378,-4.89142714353344,
8.7550768112819));
#48652=CARTESIAN_POINT('Ctrl Pts',(2.62840182732027,-4.1383285741919,8.83444870133532));
#48653=CARTESIAN_POINT('Ctrl Pts',(4.28759302222971,-2.37714232421218,8.91382059138872));
#48654=CARTESIAN_POINT('Ctrl Pts',(4.90233604735019,-0.0368894657696129,
8.99319248144213));
#48655=CARTESIAN_POINT('Ctrl Pts',(4.32288086247292,2.31234958488097,9.07256437149553));
#48656=CARTESIAN_POINT('Ctrl Pts',(2.69038146803174,4.09830539495352,9.15193626154892));
#48657=CARTESIAN_POINT('Ctrl Pts',(0.402511103036409,4.88592308226053,9.23130815160233));
#48658=CARTESIAN_POINT('Ctrl Pts',(-1.9834100757154,4.48334072153617,9.31068004165575));
#48659=CARTESIAN_POINT('Ctrl Pts',(-3.88617695022667,2.98862648475194,9.39005193170914));
#48660=CARTESIAN_POINT('Ctrl Pts',(-4.84227972156947,0.765889451494674,
9.46942382176256));
#48661=CARTESIAN_POINT('Ctrl Pts',(-4.61881387094234,-1.64341655687914,
9.54879571181594));
#48662=CARTESIAN_POINT('Ctrl Pts',(-3.27021518492473,-3.65238992963806,
9.62816760186936));
#48663=CARTESIAN_POINT('Ctrl Pts',(-1.124999318358,-4.77164919996512,9.70753949192275));
#48664=CARTESIAN_POINT('Ctrl Pts',(1.29426389201697,-4.72854528704705,9.78691138197616));
#48665=CARTESIAN_POINT('Ctrl Pts',(3.39824728310117,-3.53357820866179,9.86628327202957));
#48666=CARTESIAN_POINT('Ctrl Pts',(4.67442515791466,-1.4778393000892,9.94565516208296));
#48667=CARTESIAN_POINT('Ctrl Pts',(4.81192341092478,0.937897990843289,10.0250270521364));
#48668=CARTESIAN_POINT('Ctrl Pts',(3.7772477720454,3.12516540720838,10.1043989421898));
#48669=CARTESIAN_POINT('Ctrl Pts',(1.82244293669188,4.55114944781378,10.1837708322432));
#48670=CARTESIAN_POINT('Ctrl Pts',(-0.576304964130747,4.86848355673017,
10.2631427222966));
#48671=CARTESIAN_POINT('Ctrl Pts',(-2.83466625132052,3.99986584743267,10.34251461235));
#48672=CARTESIAN_POINT('Ctrl Pts',(-4.40250911411597,2.15688967125344,10.4218865024034));
#48673=CARTESIAN_POINT('Ctrl Pts',(-4.89791050150136,-0.211500054648842,
10.5012583924568));
#48674=CARTESIAN_POINT('Ctrl Pts',(-4.20019173206204,-2.52836883538606,
10.5806302825102));
#48675=CARTESIAN_POINT('Ctrl Pts',(-2.47931555365911,-4.22933256427274,
10.6600021725636));
#48676=CARTESIAN_POINT('Ctrl Pts',(-0.154483594256702,-4.90004024197143,
10.739374062617));
#48677=CARTESIAN_POINT('Ctrl Pts',(2.20798022676301,-4.37710896278096,10.8187459526704));
#48678=CARTESIAN_POINT('Ctrl Pts',(4.03258495182456,-2.7879236288234,10.8981178427238));
#48679=CARTESIAN_POINT('Ctrl Pts',(4.87486090859705,-0.519606269848766,
10.9774897327772));
#48680=CARTESIAN_POINT('Ctrl Pts',(4.52963153835691,1.87528602633207,11.0568616228306));
#48681=CARTESIAN_POINT('Ctrl Pts',(3.08099395154235,3.81336279737362,11.136233512884));
#48682=CARTESIAN_POINT('Ctrl Pts',(0.881833057796546,4.82251283171035,11.2156054029374));
#48683=CARTESIAN_POINT('Ctrl Pts',(-1.53214041692415,4.65690941469354,11.2949772929908));
#48684=CARTESIAN_POINT('Ctrl Pts',(-3.5728878774174,3.35689317215153,11.3743491830443));
#48685=CARTESIAN_POINT('Ctrl Pts',(-4.74328775942496,1.23914518323042,11.4537210730976));
#48686=CARTESIAN_POINT('Ctrl Pts',(-4.75823324232597,-1.1804558295243,11.533092963151));
#48687=CARTESIAN_POINT('Ctrl Pts',(-3.614083639567,-3.31250041510156,11.6124648532044));
#48688=CARTESIAN_POINT('Ctrl Pts',(-1.58955126184795,-4.63762723165536,
11.6918367432579));
#48689=CARTESIAN_POINT('Ctrl Pts',(0.822192284845203,-4.83303831979168,
11.7712086333112));
#48690=CARTESIAN_POINT('Ctrl Pts',(3.03365161084184,-3.85113197097562,11.8505805233647));
#48691=CARTESIAN_POINT('Ctrl Pts',(4.50612011931135,-1.9310983983659,11.9299524134181));
#48692=CARTESIAN_POINT('Ctrl Pts',(4.88090774084429,0.459346469671929,12.0093243034715));
#48693=CARTESIAN_POINT('Ctrl Pts',(4.06671704041361,2.73789555444384,12.0886961935249));
#48694=CARTESIAN_POINT('Ctrl Pts',(2.26188307046365,4.34949934238227,12.1680680835783));
#48695=CARTESIAN_POINT('Ctrl Pts',(-0.0939406088580155,4.90157471796985,
12.2474399736317));
#48696=CARTESIAN_POINT('Ctrl Pts',(-2.42688056379585,4.25963734171157,12.3268118636851));
#48697=CARTESIAN_POINT('Ctrl Pts',(-4.16863778520202,2.58006173755973,12.4061837537385));
#48698=CARTESIAN_POINT('Ctrl Pts',(-4.89492406925624,0.271988805008134,
12.4855556437919));
#48699=CARTESIAN_POINT('Ctrl Pts',(-4.4288176847703,-2.10233999840645,12.5649275338453));
#48700=CARTESIAN_POINT('Ctrl Pts',(-2.88386111529598,-3.96454343165991,
12.6442994238987));
#48701=CARTESIAN_POINT('Ctrl Pts',(-0.636402361453836,-4.86099286032903,
12.7236713139521));
#48702=CARTESIAN_POINT('Ctrl Pts',(1.76608259898569,-4.57331518784718,12.8030432040055));
#48703=CARTESIAN_POINT('Ctrl Pts',(3.73835374746984,-3.17158805846724,12.8824150940589));
#48704=CARTESIAN_POINT('Ctrl Pts',(4.79997019777602,-0.997269098235751,
12.9617869841123));
#48705=CARTESIAN_POINT('Ctrl Pts',(4.69232453245774,1.41998240690827,13.0411588741657));
#48706=CARTESIAN_POINT('Ctrl Pts',(3.44163899731696,3.49132934080715,13.1205307642191));
#48707=CARTESIAN_POINT('Ctrl Pts',(1.35257782036847,4.71219617521183,13.1999026542725));
#48708=CARTESIAN_POINT('Ctrl Pts',(-1.06596831974157,4.78518245160425,13.2792745443259));
#48709=CARTESIAN_POINT('Ctrl Pts',(-3.22484693664342,3.69250887460753,13.3586464343793));
#48710=CARTESIAN_POINT('Ctrl Pts',(-4.59815997785652,1.70034830898619,13.4380183244327));
#48711=CARTESIAN_POINT('Ctrl Pts',(-4.85137142631828,-0.706013341047003,
13.5173902144861));
#48712=CARTESIAN_POINT('Ctrl Pts',(-3.92279953365742,-2.94039170393519,
13.5967621045396));
#48713=CARTESIAN_POINT('Ctrl Pts',(-2.03864235756713,-4.45849715619141,
13.6761339945929));
#48714=CARTESIAN_POINT('Ctrl Pts',(0.342123584368241,-4.8905225699155,13.7555058846463));
#48715=CARTESIAN_POINT('Ctrl Pts',(2.63954897842921,-4.13122751059623,13.8348777746997));
#48716=CARTESIAN_POINT('Ctrl Pts',(4.29398608388735,-2.36557457401273,13.9142496647532));
#48717=CARTESIAN_POINT('Ctrl Pts',(4.90241768388754,-0.0236729073102294,
13.9936215548065));
#48718=CARTESIAN_POINT('Ctrl Pts',(4.31663118741021,2.32399542721397,14.07299344486));
#48719=CARTESIAN_POINT('Ctrl Pts',(2.67932288838078,4.10554361974547,14.1523653349134));
#48720=CARTESIAN_POINT('Ctrl Pts',(0.389337464322444,4.8869904739736,14.2317372249668));
#48721=CARTESIAN_POINT('Ctrl Pts',(-1.99548970426098,4.47797726591172,14.3111091150202));
#48722=CARTESIAN_POINT('Ctrl Pts',(-3.894219997828,2.97813870770829,14.3904810050736));
#48723=CARTESIAN_POINT('Ctrl Pts',(-4.84432691963384,0.752832152305313,
14.469852895127));
#48724=CARTESIAN_POINT('Ctrl Pts',(-4.61436652655265,-1.6558626490335,14.5492247851804));
#48725=CARTESIAN_POINT('Ctrl Pts',(-3.26035666133029,-3.66119297425757,
14.6285966752338));
#48726=CARTESIAN_POINT('Ctrl Pts',(-1.11213113008494,-4.77466479486569,
14.7079685652872));
#48727=CARTESIAN_POINT('Ctrl Pts',(1.30700708278859,-4.72503883998578,14.7873404553406));
#48728=CARTESIAN_POINT('Ctrl Pts',(3.40776126330594,-3.52440388238144,14.866712345394));
#48729=CARTESIAN_POINT('Ctrl Pts',(4.67839234303357,-1.46523194016464,14.9460842354474));
#48730=CARTESIAN_POINT('Ctrl Pts',(4.80937740344404,0.95086725944037,15.0254561255008));
#48731=CARTESIAN_POINT('Ctrl Pts',(3.76880877375186,3.13533729935469,15.1048280155542));
#48732=CARTESIAN_POINT('Ctrl Pts',(1.81016666889045,4.55604611309762,15.1841999056076));
#48733=CARTESIAN_POINT('Ctrl Pts',(-0.58942802977675,4.86691217832697,15.263571795661));
#48734=CARTESIAN_POINT('Ctrl Pts',(-2.84543936506709,3.99220920964323,15.3429436857144));
#48735=CARTESIAN_POINT('Ctrl Pts',(-4.40830796930035,2.14501291409566,15.4223155757678));
#48736=CARTESIAN_POINT('Ctrl Pts',(-4.89732250983615,-0.224703779420184,
15.5016874658212));
#48737=CARTESIAN_POINT('Ctrl Pts',(-4.19336012701549,-2.53968312964247,
15.5810593558746));
#48738=CARTESIAN_POINT('Ctrl Pts',(-2.46790449909881,-4.23600129097741,
15.6604312459281));
#48739=CARTESIAN_POINT('Ctrl Pts',(-0.141272797816101,-4.90043891405947,
15.7398031359814));
#48740=CARTESIAN_POINT('Ctrl Pts',(2.21977264431347,-4.37114046461536,15.8191750260349));
#48741=CARTESIAN_POINT('Ctrl Pts',(4.04008638367001,-2.77704187334405,15.8985469160882));
#48742=CARTESIAN_POINT('Ctrl Pts',(4.87624402254724,-0.50646202860824,15.9779188061417));
#48743=CARTESIAN_POINT('Ctrl Pts',(4.52455941090906,1.88749084526974,16.057290696195));
#48744=CARTESIAN_POINT('Ctrl Pts',(3.0707021417271,3.82165512711525,16.1366625862485));
#48745=CARTESIAN_POINT('Ctrl Pts',(0.868828627683026,4.82487267911372,16.2160344763019));
#48746=CARTESIAN_POINT('Ctrl Pts',(-1.54468961690488,4.65276192610161,16.2954063663553));
#48747=CARTESIAN_POINT('Ctrl Pts',(-3.58192489000319,3.34724866670505,16.3747782564087));
#48748=CARTESIAN_POINT('Ctrl Pts',(-4.74661118820951,1.22635304091943,16.4541501464621));
#48749=CARTESIAN_POINT('Ctrl Pts',(-4.75503350768456,-1.19327947079094,
16.5335220365155));
#48750=CARTESIAN_POINT('Ctrl Pts',(-3.60514018926425,-3.32223174536968,
16.6128939265689));
#48751=CARTESIAN_POINT('Ctrl Pts',(-1.57704270154751,-4.64189571913949,
16.6922658166223));
#48752=CARTESIAN_POINT('Ctrl Pts',(0.835218899365215,-4.83080417279076,
16.7716377066757));
#48753=CARTESIAN_POINT('Ctrl Pts',(3.04402302167444,-3.84293941821851,16.8510095967291));
#48754=CARTESIAN_POINT('Ctrl Pts',(4.5113098802371,-1.91894313613405,16.9303814867825));
#48755=CARTESIAN_POINT('Ctrl Pts',(4.87965162531072,0.47250346257415,17.0097533768359));
#48756=CARTESIAN_POINT('Ctrl Pts',(4.05932105856824,2.74884923313555,17.0891252668893));
#48757=CARTESIAN_POINT('Ctrl Pts',(2.25014882333735,4.35558147263106,17.1684971569427));
#48758=CARTESIAN_POINT('Ctrl Pts',(-0.107154601980602,4.90130359745223,
17.2478690469961));
#48759=CARTESIAN_POINT('Ctrl Pts',(-2.43835555951383,4.25307922033065,17.3272409370495));
#48760=CARTESIAN_POINT('Ctrl Pts',(-4.17557820525659,2.56881377105676,17.4066128271029));
#48761=CARTESIAN_POINT('Ctrl Pts',(-4.8956397991406,0.258791705958601,17.4859847171563));
#48762=CARTESIAN_POINT('Ctrl Pts',(-4.42313332356637,-2.11427282962181,
17.5653566072097));
#48763=CARTESIAN_POINT('Ctrl Pts',(-2.8731633447509,-3.97230257099397,17.6447284972631));
#48764=CARTESIAN_POINT('Ctrl Pts',(-0.623293388711154,-4.8626931320669,
17.7241003873165));
#48765=CARTESIAN_POINT('Ctrl Pts',(1.77840238381723,-4.56853309419578,17.8034722773699));
#48766=CARTESIAN_POINT('Ctrl Pts',(3.74689662802603,-3.1615060961514,17.8828441674233));
#48767=CARTESIAN_POINT('Ctrl Pts',(4.80262992851038,-0.984309998791364,
17.9622160574768));
#48768=CARTESIAN_POINT('Ctrl Pts',(4.6885008269824,1.43259912421597,18.0415879475301));
#48769=CARTESIAN_POINT('Ctrl Pts',(3.43217338911689,3.50064868327997,18.1209598375836));
#48770=CARTESIAN_POINT('Ctrl Pts',(1.33994588402617,4.71572438645645,18.2003317276369));
#48771=CARTESIAN_POINT('Ctrl Pts',(-1.07901003836845,4.78248223987434,18.2797036176904));
#48772=CARTESIAN_POINT('Ctrl Pts',(-3.23451621663571,3.68344087079119,18.3590755077438));
#48773=CARTESIAN_POINT('Ctrl Pts',(-4.60324425657823,1.68862650319409,18.4384473977972));
#48774=CARTESIAN_POINT('Ctrl Pts',(-4.84847467695998,-0.720374489880202,
18.5178192878506));
#48775=CARTESIAN_POINT('Ctrl Pts',(-3.91669769333075,-2.94853678524982,
18.597191177904));
#48776=CARTESIAN_POINT('Ctrl Pts',(-2.02316502874899,-4.46849826887172,
18.6765630679574));
#48777=CARTESIAN_POINT('Ctrl Pts',(0.348982623889014,-4.88143613581971,
18.7559349580108));
#48778=CARTESIAN_POINT('Ctrl Pts',(3.43189297168081,-3.8881060605371,18.8617641447486));
#48779=CARTESIAN_POINT('Ctrl Pts',(5.55807194231376,-0.0182675279710476,
18.994050628171));
#48780=CARTESIAN_POINT('Ctrl Pts',(3.02540872544997,4.66632909528411,19.1527944082778));
#48781=CARTESIAN_POINT('Ctrl Pts',(-2.2762392030432,5.06930720888685,19.3115381883846));
#48782=CARTESIAN_POINT('Ctrl Pts',(-5.49476366156208,0.839647798275813,
19.4702819684914));
#48783=CARTESIAN_POINT('Ctrl Pts',(-3.68539651252317,-4.16147159288528,
19.6290257485982));
#48784=CARTESIAN_POINT('Ctrl Pts',(1.49629817009931,-5.35305176256653,19.787769528705));
#48785=CARTESIAN_POINT('Ctrl Pts',(5.30889903625351,-1.64699798333508,19.9465133088118));
#48786=CARTESIAN_POINT('Ctrl Pts',(4.26335305224425,3.56621538027062,20.1052570889186));
#48787=CARTESIAN_POINT('Ctrl Pts',(-0.682914143845088,5.51666761234037,
20.2640008690254));
#48788=CARTESIAN_POINT('Ctrl Pts',(-5.00517315099108,2.41778366488215,20.4227446491323));
#48789=CARTESIAN_POINT('Ctrl Pts',(-4.74574684718966,-2.89085235699305,
20.581488429239));
#48790=CARTESIAN_POINT('Ctrl Pts',(-0.146932230206273,-5.55932874556366,
20.7402322093459));
#48791=CARTESIAN_POINT('Ctrl Pts',(4.59246965375652,-3.13076985705421,20.8989759894527));
#48792=CARTESIAN_POINT('Ctrl Pts',(5.0299278500732,1.2629663218453,21.031262472875));
#48793=CARTESIAN_POINT('Ctrl Pts',(3.05056344532296,3.82678328180762,21.1370916596129));
#48794=CARTESIAN_POINT('Ctrl Pts',(0.861221142909519,4.82897211168878,21.2164635496663));
#48795=CARTESIAN_POINT('Ctrl Pts',(-1.56011376732917,4.64762681676397,21.2958354397197));
#48796=CARTESIAN_POINT('Ctrl Pts',(-3.58940432897566,3.338086676814,21.3752073297731));
#48797=CARTESIAN_POINT('Ctrl Pts',(-4.75071159562141,1.21328335035074,21.4545792198265));
#48798=CARTESIAN_POINT('Ctrl Pts',(-4.75136940590249,-1.2059521437222,21.5339511098799));
#48799=CARTESIAN_POINT('Ctrl Pts',(-3.59639816964331,-3.33201429213618,
21.6133229999333));
#48800=CARTESIAN_POINT('Ctrl Pts',(-1.56440212229559,-4.64609055668268,
21.6926948899867));
#48801=CARTESIAN_POINT('Ctrl Pts',(0.848175594776096,-4.82855605094712,
21.7720667800401));
#48802=CARTESIAN_POINT('Ctrl Pts',(3.05440612489727,-3.83470774368908,21.8514386700935));
#48803=CARTESIAN_POINT('Ctrl Pts',(4.5164489386699,-1.90677984789329,21.9308105601469));
#48804=CARTESIAN_POINT('Ctrl Pts',(4.87836953900972,0.485660146581216,22.0101824502003));
#48805=CARTESIAN_POINT('Ctrl Pts',(4.0518905292872,2.75978129753096,22.0895543402537));
#48806=CARTESIAN_POINT('Ctrl Pts',(2.23840092153696,4.36163277449212,22.1689262303071));
#48807=CARTESIAN_POINT('Ctrl Pts',(-0.120369299865574,4.90099648569508,
22.2482981203605));
#48808=CARTESIAN_POINT('Ctrl Pts',(-2.44981194564663,4.24649024808576,22.327670010414));
#48809=CARTESIAN_POINT('Ctrl Pts',(-4.18248893842781,2.55754735438689,22.4070419004673));
#48810=CARTESIAN_POINT('Ctrl Pts',(-4.89631923419535,0.245592132270486,
22.4864137905208));
#48811=CARTESIAN_POINT('Ctrl Pts',(-4.41741787585779,-2.12618907886207,
22.5657856805741));
#48812=CARTESIAN_POINT('Ctrl Pts',(-2.86244283812702,-3.98003518345998,
22.6451575706276));
#48813=CARTESIAN_POINT('Ctrl Pts',(-0.610183305945143,-4.86435360814152,
22.724529460681));
#48814=CARTESIAN_POINT('Ctrl Pts',(1.79071565870375,-4.56372621798445,22.8039013507344));
#48815=CARTESIAN_POINT('Ctrl Pts',(3.75540018385464,-3.15138524551451,22.8832732407878));
#48816=CARTESIAN_POINT('Ctrl Pts',(4.80527757305005,-0.971373790660912,
22.9626451308412));
#48817=CARTESIAN_POINT('Ctrl Pts',(4.68459996247748,1.44526216311697,23.0420170208946));
#48818=CARTESIAN_POINT('Ctrl Pts',(3.42276418043937,3.50983545637268,23.121388910948));
#48819=CARTESIAN_POINT('Ctrl Pts',(1.3271506148001,4.71942059955514,23.2007608010014));
#48820=CARTESIAN_POINT('Ctrl Pts',(-1.09175390014331,4.7793653318942,23.2801326910548));
#48821=CARTESIAN_POINT('Ctrl Pts',(-3.2447095830844,3.67506724782751,23.3595045811082));
#48822=CARTESIAN_POINT('Ctrl Pts',(-4.60726119282589,1.67553091707926,23.4388764711616));
#48823=CARTESIAN_POINT('Ctrl Pts',(-4.84749417441997,-0.732161036485464,
23.518248361215));
#48824=CARTESIAN_POINT('Ctrl Pts',(-3.90688830464649,-2.96150018209874,
23.5976202512684));
#48825=CARTESIAN_POINT('Ctrl Pts',(-2.01457309173102,-4.46942443856173,
23.6769921413218));
#48826=CARTESIAN_POINT('Ctrl Pts',(0.368487667211392,-4.88860679467339,
23.7563640313752));
#48827=CARTESIAN_POINT('Ctrl Pts',(2.66178564602131,-4.1169353563613,23.8357359214286));
#48828=CARTESIAN_POINT('Ctrl Pts',(4.30667853324075,-2.34238757791555,23.915107811482));
#48829=CARTESIAN_POINT('Ctrl Pts',(4.90247406242456,0.00276062972037378,
23.9944797015354));
#48830=CARTESIAN_POINT('Ctrl Pts',(4.30403776144901,2.34723635406859,24.0738515915888));
#48831=CARTESIAN_POINT('Ctrl Pts',(2.65714738860781,4.1199304980844,24.1532234816422));
#48832=CARTESIAN_POINT('Ctrl Pts',(0.362981793399119,4.88901869207872,24.2325953716956));
#48833=CARTESIAN_POINT('Ctrl Pts',(-2.01960536323572,4.46715275434179,24.311967261749));
#48834=CARTESIAN_POINT('Ctrl Pts',(-3.9102211237066,2.95709829352223,24.3913391518025));
#48835=CARTESIAN_POINT('Ctrl Pts',(-4.84831567357046,0.726701233826634,
24.4707110418558));
#48836=CARTESIAN_POINT('Ctrl Pts',(-4.60537125691712,-1.68071863790322,
24.5500829319093));
#48837=CARTESIAN_POINT('Ctrl Pts',(-3.2405685958952,-3.67871916964745,24.6294548219626));
#48838=CARTESIAN_POINT('Ctrl Pts',(-1.08637059779009,-4.78059185437233,
24.7088267120161));
#48839=CARTESIAN_POINT('Ctrl Pts',(1.33246487329615,-4.71792294503267,24.7881986020694));
#48840=CARTESIAN_POINT('Ctrl Pts',(3.42671485060842,-3.50597844922833,24.8675704921229));
#48841=CARTESIAN_POINT('Ctrl Pts',(4.68622467521711,-1.43998536354369,24.9469423821763));
#48842=CARTESIAN_POINT('Ctrl Pts',(4.80418054172532,0.976784969346655,25.0263142722297));
#48843=CARTESIAN_POINT('Ctrl Pts',(3.75184866214253,3.15561264578101,25.105686162283));
#48844=CARTESIAN_POINT('Ctrl Pts',(1.785574753038,4.56574006653325,25.1850580523365));
#48845=CARTESIAN_POINT('Ctrl Pts',(-0.615661213603954,4.86366331317224,
25.2644299423898));
#48846=CARTESIAN_POINT('Ctrl Pts',(-2.86692347135497,3.97680894225859,25.3438018324433));
#48847=CARTESIAN_POINT('Ctrl Pts',(-4.41980951731136,2.12121271552801,25.4231737224967));
#48848=CARTESIAN_POINT('Ctrl Pts',(-4.89603974793313,-0.25110623348048,
25.5025456125501));
#48849=CARTESIAN_POINT('Ctrl Pts',(-4.17960553315853,-2.56225625982736,
25.5819175026035));
#48850=CARTESIAN_POINT('Ctrl Pts',(-2.44502866190641,-4.24924633273829,
25.6612893926569));
#48851=CARTESIAN_POINT('Ctrl Pts',(-0.114848220593104,-4.9011294045414,
25.7406612827103));
#48852=CARTESIAN_POINT('Ctrl Pts',(2.24330899304448,-4.35910820186418,25.8200331727637));
#48853=CARTESIAN_POINT('Ctrl Pts',(4.05500110145669,-2.75521788993518,25.8994050628171));
#48854=CARTESIAN_POINT('Ctrl Pts',(4.87890391714675,-0.480162598589303,
25.9787769528705));
#48855=CARTESIAN_POINT('Ctrl Pts',(4.51431653789045,1.91185923895103,26.0581488429239));
#48856=CARTESIAN_POINT('Ctrl Pts',(3.05005164227427,3.83815639771151,26.1375207329773));
#48857=CARTESIAN_POINT('Ctrl Pts',(0.842800917774871,4.82948715360457,26.2168926230307));
#48858=CARTESIAN_POINT('Ctrl Pts',(-1.56975424478632,4.64436552876808,26.2962645130841));
#48859=CARTESIAN_POINT('Ctrl Pts',(-3.59992074790968,3.32788674125238,26.3756364031376));
#48860=CARTESIAN_POINT('Ctrl Pts',(-4.7531545251316,1.20074210971995,26.4550082931909));
#48861=CARTESIAN_POINT('Ctrl Pts',(-4.74853038096058,-1.21890064194263,
26.5343801832443));
#48862=CARTESIAN_POINT('Ctrl Pts',(-3.58717474668129,-3.34162189521881,
26.6137520732977));
#48863=CARTESIAN_POINT('Ctrl Pts',(-1.55199128418706,-4.65033145137433,
26.6931239633511));
#48864=CARTESIAN_POINT('Ctrl Pts',(0.861253819860729,-4.82623055930912,
26.7724958534045));
#48865=CARTESIAN_POINT('Ctrl Pts',(3.06469939974342,-3.82647058567632,26.851867743458));
#48866=CARTESIAN_POINT('Ctrl Pts',(4.52159098944567,-1.89459084712176,26.9312396335114));
#48867=CARTESIAN_POINT('Ctrl Pts',(4.87703302249084,0.49880702818598,27.0106115235648));
#48868=CARTESIAN_POINT('Ctrl Pts',(4.0444406063867,2.77069661551822,27.0899834136182));
#48869=CARTESIAN_POINT('Ctrl Pts',(2.22663141078423,4.36765064014314,27.1693553036716));
#48870=CARTESIAN_POINT('Ctrl Pts',(-0.133580267920228,4.90065463645992,
27.248727193725));
#48871=CARTESIAN_POINT('Ctrl Pts',(-2.46125208903423,4.23987001075014,27.3280990837784));
#48872=CARTESIAN_POINT('Ctrl Pts',(-4.1893683491486,2.54626243521474,27.4074709738318));
#48873=CARTESIAN_POINT('Ctrl Pts',(-4.89696375241997,0.232390966517291,
27.4868428638852));
#48874=CARTESIAN_POINT('Ctrl Pts',(-4.41166962484721,-2.13809042723509,
27.5662147539386));
#48875=CARTESIAN_POINT('Ctrl Pts',(-2.85170254172674,-3.98773772549588,
27.645586643992));
#48876=CARTESIAN_POINT('Ctrl Pts',(-0.597067031578144,-4.8659809405336,
27.7249585340454));
#48877=CARTESIAN_POINT('Ctrl Pts',(1.80301268587744,-4.55888196912345,27.8043304240988));
#48878=CARTESIAN_POINT('Ctrl Pts',(3.76388250395415,-3.14124944094887,27.8837023141522));
#48879=CARTESIAN_POINT('Ctrl Pts',(4.80787887528022,-0.958415501996903,
27.9630742042056));
#48880=CARTESIAN_POINT('Ctrl Pts',(4.68068659464744,1.45788633182479,28.042446094259));
#48881=CARTESIAN_POINT('Ctrl Pts',(3.41328942008259,3.51905028219065,28.1218179843124));
#48882=CARTESIAN_POINT('Ctrl Pts',(1.31442249797358,4.72298137310056,28.2011898743658));
#48883=CARTESIAN_POINT('Ctrl Pts',(-1.10463483521695,4.77640465566507,28.2805617644192));
#48884=CARTESIAN_POINT('Ctrl Pts',(-3.25460556761632,3.66630633650198,28.3599336544726));
#48885=CARTESIAN_POINT('Ctrl Pts',(-4.6117615876916,1.66310390899846,28.439305544526));
#48886=CARTESIAN_POINT('Ctrl Pts',(-4.84550269296638,-0.745226949519058,
28.5186774345794));
#48887=CARTESIAN_POINT('Ctrl Pts',(-3.89889006757279,-2.97202217266562,
28.5980493246329));
#48888=CARTESIAN_POINT('Ctrl Pts',(-2.00251645176526,-4.4748393730103,28.6774212146862));
#48889=CARTESIAN_POINT('Ctrl Pts',(0.381665739197275,-4.88759560697863,
28.7567931047396));
#48890=CARTESIAN_POINT('Ctrl Pts',(2.67287500089413,-4.10974436959635,28.8361649947931));
#48891=CARTESIAN_POINT('Ctrl Pts',(4.31297782868169,-2.33076850054527,28.9155368848464));
#48892=CARTESIAN_POINT('Ctrl Pts',(4.90244880401687,0.015977416170102,28.9949087748999));
#48893=CARTESIAN_POINT('Ctrl Pts',(4.29769410207987,2.35883126967183,29.0742806649532));
#48894=CARTESIAN_POINT('Ctrl Pts',(2.64603062966077,4.12707904706596,29.1536525550067));
#48895=CARTESIAN_POINT('Ctrl Pts',(0.349799952745733,4.88997950372933,29.23302444506));
#48896=CARTESIAN_POINT('Ctrl Pts',(-2.03164121838909,4.46169177707024,29.3123963351135));
#48897=CARTESIAN_POINT('Ctrl Pts',(-3.91817908568586,2.94654580930412,29.3917682251669));
#48898=CARTESIAN_POINT('Ctrl Pts',(-4.85025720045188,0.71362780446005,29.4711401152203));
#48899=CARTESIAN_POINT('Ctrl Pts',(-4.60082339705005,-1.69312835396218,
29.5505120052737));
#48900=CARTESIAN_POINT('Ctrl Pts',(-3.23063919787666,-3.68744219303526,
29.6298838953271));
#48901=CARTESIAN_POINT('Ctrl Pts',(-1.07347844099907,-4.78350327589979,
29.7092557853805));
#48902=CARTESIAN_POINT('Ctrl Pts',(1.34517928800161,-4.71431354886002,29.7886276754339));
#48903=CARTESIAN_POINT('Ctrl Pts',(3.43615431994896,-3.49672747627405,29.8679995654873));
#48904=CARTESIAN_POINT('Ctrl Pts',(4.69008976535537,-1.42734633034267,29.9473714555407));
#48905=CARTESIAN_POINT('Ctrl Pts',(4.8015297252588,0.989733222282683,30.0267433455941));
#48906=CARTESIAN_POINT('Ctrl Pts',(3.74332767209493,3.16571595269729,30.1061152356475));
#48907=CARTESIAN_POINT('Ctrl Pts',(1.77325928372404,4.57053728422822,30.1854871257009));
#48908=CARTESIAN_POINT('Ctrl Pts',(-0.628771141119161,4.86198585003386,
30.2648590157543));
#48909=CARTESIAN_POINT('Ctrl Pts',(-2.8776343077471,3.9690654245944,30.3442309058078));
#48910=CARTESIAN_POINT('Ctrl Pts',(-4.42551212654334,2.10928944710103,30.4236027958611));
#48911=CARTESIAN_POINT('Ctrl Pts',(-4.89534498701853,-0.264304770873174,
30.5029746859146));
#48912=CARTESIAN_POINT('Ctrl Pts',(-4.17268264431835,-2.57351493169134,
30.5823465759679));
#48913=CARTESIAN_POINT('Ctrl Pts',(-2.43356404553856,-4.25582255152819,
30.6617184660214));
#48914=CARTESIAN_POINT('Ctrl Pts',(-0.101634631868219,-4.90142121791616,
30.7410903560747));
#48915=CARTESIAN_POINT('Ctrl Pts',(2.25505275316072,-4.35304452473163,30.8204622461282));
#48916=CARTESIAN_POINT('Ctrl Pts',(4.06241427899435,-2.74427582062311,30.8998341361815));
#48917=CARTESIAN_POINT('Ctrl Pts',(4.88018067846643,-0.467007600962325,
30.979206026235));
#48918=CARTESIAN_POINT('Ctrl Pts',(4.50914586676086,1.9240226365891,31.0585779162884));
#48919=CARTESIAN_POINT('Ctrl Pts',(3.0396931027374,3.84636521861933,31.1379498063418));
#48920=CARTESIAN_POINT('Ctrl Pts',(0.829777827133663,4.83174174717888,31.2173216963951));
#48921=CARTESIAN_POINT('Ctrl Pts',(-1.58226949047778,4.64011668100458,31.2966935864486));
#48922=CARTESIAN_POINT('Ctrl Pts',(-3.60887946250293,3.31816946206164,31.376065476502));
#48923=CARTESIAN_POINT('Ctrl Pts',(-4.75637438558157,1.18792350680397,31.4554373665554));
#48924=CARTESIAN_POINT('Ctrl Pts',(-4.74522703638862,-1.23169798528705,
31.5348092566087));
#48925=CARTESIAN_POINT('Ctrl Pts',(-3.57815288451333,-3.35128057447936,
31.6141811466622));
#48926=CARTESIAN_POINT('Ctrl Pts',(-1.53944861007768,-4.65449863366224,
31.6935530367156));
#48927=CARTESIAN_POINT('Ctrl Pts',(0.874261938261232,-4.823891128243,31.772924926769));
#48928=CARTESIAN_POINT('Ctrl Pts',(3.07500421358568,-3.81819442148565,31.8522968168224));
#48929=CARTESIAN_POINT('Ctrl Pts',(4.52668226888703,-1.88239400508438,31.9316687068758));
#48930=CARTESIAN_POINT('Ctrl Pts',(4.87567054312872,0.511953424346944,32.0110405969291));
#48931=CARTESIAN_POINT('Ctrl Pts',(4.036956265178,2.78159013279705,32.0904124869827));
#48932=CARTESIAN_POINT('Ctrl Pts',(2.21484837668102,4.37363764184315,32.169784377036));
#48933=CARTESIAN_POINT('Ctrl Pts',(-0.146791673891742,4.90027670221896,
32.2491562670894));
#48934=CARTESIAN_POINT('Ctrl Pts',(-2.47267359762233,4.23321920451271,32.3285281571428));
#48935=CARTESIAN_POINT('Ctrl Pts',(-4.19621770614226,2.53495887865897,32.4079000471962));
#48936=CARTESIAN_POINT('Ctrl Pts',(-4.89757246961631,0.219188181000233,
32.4872719372496));
#48937=CARTESIAN_POINT('Ctrl Pts',(-4.40588942008463,-2.1499762723854,32.566643827303));
#48938=CARTESIAN_POINT('Ctrl Pts',(-2.84094146009112,-3.99541126470971,
32.6460157173564));
#48939=CARTESIAN_POINT('Ctrl Pts',(-0.583946448736662,-4.86757291664353,
32.7253876074098));
#48940=CARTESIAN_POINT('Ctrl Pts',(1.81529662498649,-4.55400458027289,32.8047594974633));
#48941=CARTESIAN_POINT('Ctrl Pts',(3.77233745895388,-3.13109080826592,32.8841313875166));
#48942=CARTESIAN_POINT('Ctrl Pts',(4.81044523784739,-0.945450245917296,
32.96350327757));
#48943=CARTESIAN_POINT('Ctrl Pts',(4.67673920454123,1.4704999036181,33.0428751676234));
#48944=CARTESIAN_POINT('Ctrl Pts',(3.40378985279549,3.52823953152847,33.1222470576768));
#48945=CARTESIAN_POINT('Ctrl Pts',(1.30168482706983,4.72650781918426,33.2016189477302));
#48946=CARTESIAN_POINT('Ctrl Pts',(-1.11750774129953,4.7734092640344,33.2809908377837));
#48947=CARTESIAN_POINT('Ctrl Pts',(-3.2644778974498,3.65751877792795,33.360362727837));
#48948=CARTESIAN_POINT('Ctrl Pts',(-4.61622846358057,1.65066481329873,33.4397346178904));
#48949=CARTESIAN_POINT('Ctrl Pts',(-4.84347599383145,-0.75828744616548,
33.5191065079439));
#48950=CARTESIAN_POINT('Ctrl Pts',(-3.89086349283728,-2.98252256218456,
33.5984783979973));
#48951=CARTESIAN_POINT('Ctrl Pts',(-1.99044525726817,-4.4802217837572,33.6778502880507));
#48952=CARTESIAN_POINT('Ctrl Pts',(0.394841037195618,-4.88654889560926,
33.7572221781041));
#48953=CARTESIAN_POINT('Ctrl Pts',(2.68394492896431,-4.10252351268344,33.8365940681574));
#48954=CARTESIAN_POINT('Ctrl Pts',(4.31924577684866,-2.31913248284973,33.9159659582109));
#48955=CARTESIAN_POINT('Ctrl Pts',(4.90238791398107,0.029194086493524,33.9953378482642));
#48956=CARTESIAN_POINT('Ctrl Pts',(4.29131920651926,2.37040904098698,34.0747097383177));
#48957=CARTESIAN_POINT('Ctrl Pts',(2.63489463902328,4.13419759990741,34.1540816283711));
#48958=CARTESIAN_POINT('Ctrl Pts',(0.336615569701593,4.89090477438156,34.2334535184245));
#48959=CARTESIAN_POINT('Ctrl Pts',(-2.04366230731349,4.45619837165044,34.3128254084779));
#48960=CARTESIAN_POINT('Ctrl Pts',(-3.92610856983677,2.93597190921303,34.3921972985313));
#48961=CARTESIAN_POINT('Ctrl Pts',(-4.85216347504172,0.700549188354975,
34.4715691885847));
#48962=CARTESIAN_POINT('Ctrl Pts',(-4.59624209780822,-1.70552576414703,
34.5509410786381));
#48963=CARTESIAN_POINT('Ctrl Pts',(-3.22068631915797,-3.69613841562006,
34.6303129686915));
#48964=CARTESIAN_POINT('Ctrl Pts',(-1.06057848202912,-4.7863799303117,34.709684858745));
#48965=CARTESIAN_POINT('Ctrl Pts',(1.35788392577142,-4.71066988845169,34.7890567487982));
#48966=CARTESIAN_POINT('Ctrl Pts',(3.44556881487913,-3.48745108865577,34.8684286388518));
#48967=CARTESIAN_POINT('Ctrl Pts',(4.69392076731947,-1.41469692300534,34.9478005289051));
#48968=CARTESIAN_POINT('Ctrl Pts',(4.79884401065818,1.00267428171067,35.0271724189586));
#48969=CARTESIAN_POINT('Ctrl Pts',(3.73477947506157,3.17579625078383,35.1065443090119));
#48970=CARTESIAN_POINT('Ctrl Pts',(1.76093092613411,4.57530128267181,35.1859161990653));
#48971=CARTESIAN_POINT('Ctrl Pts',(-0.64187649864509,4.86027304935852,35.2652880891187));
#48972=CARTESIAN_POINT('Ctrl Pts',(-2.88832422912388,3.96129305925348,35.3446599791721));
#48973=CARTESIAN_POINT('Ctrl Pts',(-4.43118257058537,2.09735084808771,35.4240318692256));
#48974=CARTESIAN_POINT('Ctrl Pts',(-4.89461464610851,-0.277501387264873,
35.5034037592789));
#48975=CARTESIAN_POINT('Ctrl Pts',(-4.16572942788534,-2.58475489891863,
35.5827756493324));
#48976=CARTESIAN_POINT('Ctrl Pts',(-2.42208174171502,-4.2623678384537,35.6621475393857));
#48977=CARTESIAN_POINT('Ctrl Pts',(-0.0884203044499451,-4.90167740713266,
35.7415194294392));
#48978=CARTESIAN_POINT('Ctrl Pts',(2.26678012326416,-4.34694920911302,35.8208913194925));
#48979=CARTESIAN_POINT('Ctrl Pts',(4.06979793038381,-2.73331380556231,35.900263209546));
#48980=CARTESIAN_POINT('Ctrl Pts',(4.88142197000686,-0.453849209064084,
35.9796350995994));
#48981=CARTESIAN_POINT('Ctrl Pts',(4.50394242258051,1.9361720501839,36.0590069896528));
#48982=CARTESIAN_POINT('Ctrl Pts',(3.02931247032103,3.85454608365127,36.1383788797062));
#48983=CARTESIAN_POINT('Ctrl Pts',(0.816748705560739,4.83396122303424,36.2177507697595));
#48984=CARTESIAN_POINT('Ctrl Pts',(-1.59477323603157,4.63583410827775,36.297122659813));
#48985=CARTESIAN_POINT('Ctrl Pts',(-3.61781194729725,3.3084280659895,36.3764945498664));
#48986=CARTESIAN_POINT('Ctrl Pts',(-4.75955967609224,1.17509626990754,36.4558664399198));
#48987=CARTESIAN_POINT('Ctrl Pts',(-4.74188920289779,-1.24448637649244,
36.5352383299732));
#48988=CARTESIAN_POINT('Ctrl Pts',(-3.56910501587113,-3.36091489620272,
36.6146102200266));
#48989=CARTESIAN_POINT('Ctrl Pts',(-1.52689474705826,-4.65863198645693,
36.69398211008));
#48990=CARTESIAN_POINT('Ctrl Pts',(0.887263702413796,-4.82151663651726,
36.7733540001334));
#48991=CARTESIAN_POINT('Ctrl Pts',(3.08528667790275,-3.80989050616806,36.8527258901868));
#48992=CARTESIAN_POINT('Ctrl Pts',(4.53174064782084,-1.87018348156595,36.9320977802402));
#48993=CARTESIAN_POINT('Ctrl Pts',(4.87427262676759,0.525096099564754,37.0114696702936));
#48994=CARTESIAN_POINT('Ctrl Pts',(4.02944258285317,2.79246343312197,37.090841560347));
#48995=CARTESIAN_POINT('Ctrl Pts',(2.20304924477561,4.37959285538367,37.1702134504005));
#48996=CARTESIAN_POINT('Ctrl Pts',(-0.160002012962556,4.89986315213815,
37.2495853404538));
#48997=CARTESIAN_POINT('Ctrl Pts',(-2.48407713450139,4.22653763069513,37.3289572305073));
#48998=CARTESIAN_POINT('Ctrl Pts',(-4.20303656448734,2.52363689769662,37.4083291205606));
#48999=CARTESIAN_POINT('Ctrl Pts',(-4.89814559062741,0.20598380239574,37.4877010106141));
#49000=CARTESIAN_POINT('Ctrl Pts',(-4.40007719275278,-2.16184649123314,
37.5670729006674));
#49001=CARTESIAN_POINT('Ctrl Pts',(-2.83015973012786,-4.0030557647603,37.6464447907209));
#49002=CARTESIAN_POINT('Ctrl Pts',(-0.570821621698638,-4.86912951461192,
37.7258166807742));
#49003=CARTESIAN_POINT('Ctrl Pts',(1.82756737028896,-4.54909409232726,37.8051885708277));
#49004=CARTESIAN_POINT('Ctrl Pts',(3.78076499611679,-3.12090941842365,37.884560460881));
#49005=CARTESIAN_POINT('Ctrl Pts',(4.81297663748916,-0.932478118164531,
37.9639323509345));
#49006=CARTESIAN_POINT('Ctrl Pts',(4.6727578232798,1.48310278759233,38.0433042409879));
#49007=CARTESIAN_POINT('Ctrl Pts',(3.39426554635479,3.53740313723864,38.1226761310413));
#49008=CARTESIAN_POINT('Ctrl Pts',(1.2889376953013,4.72999991227071,38.2020480210947));
#49009=CARTESIAN_POINT('Ctrl Pts',(-1.13037252509376,4.77037917890205,38.2814199111481));
#49010=CARTESIAN_POINT('Ctrl Pts',(-3.27432650082598,3.64870463556727,38.3607918012015));
#49011=CARTESIAN_POINT('Ctrl Pts',(-4.62066178777622,1.63821372124413,38.4401636912549));
#49012=CARTESIAN_POINT('Ctrl Pts',(-4.84141409235733,-0.771342433159972,
38.5195355813083));
#49013=CARTESIAN_POINT('Ctrl Pts',(-3.88280863754963,-2.99300127117752,
38.5989074713617));
#49014=CARTESIAN_POINT('Ctrl Pts',(-1.97835959833324,-4.48557163766163,
38.6782793614151));
#49015=CARTESIAN_POINT('Ctrl Pts',(0.4080134699205,-4.88546665687603,38.7576512514685));
#49016=CARTESIAN_POINT('Ctrl Pts',(2.69499534131588,-4.09527285943909,38.8370231415219));
#49017=CARTESIAN_POINT('Ctrl Pts',(4.32548234816251,-2.30747956911512,38.9163950315754));
#49018=CARTESIAN_POINT('Ctrl Pts',(4.90229136258888,0.0424104685617285,
38.9957669216287));
#49019=CARTESIAN_POINT('Ctrl Pts',(4.28491317807095,2.38196972749885,39.0751388116822));
#49020=CARTESIAN_POINT('Ctrl Pts',(2.62373939006081,4.14128583366062,39.1545107017355));
#49021=CARTESIAN_POINT('Ctrl Pts',(0.323428943211332,4.89179500940948,39.233882591789));
#49022=CARTESIAN_POINT('Ctrl Pts',(-2.05566892616818,4.45067161106171,39.3132544818423));
#49023=CARTESIAN_POINT('Ctrl Pts',(-3.93400879434316,2.92537849589611,39.3926263718958));
#49024=CARTESIAN_POINT('Ctrl Pts',(-4.85403585089548,0.68746203308737,39.4719982619491));
#49025=CARTESIAN_POINT('Ctrl Pts',(-4.59162481050186,-1.71790426872522,
39.5513701520026));
#49026=CARTESIAN_POINT('Ctrl Pts',(-3.21071490770548,-3.70482006635682,
39.6307420420559));
#49027=CARTESIAN_POINT('Ctrl Pts',(-1.04766160592177,-4.78919858119775,
39.7101139321094));
#49028=CARTESIAN_POINT('Ctrl Pts',(1.37056128557131,-4.7070358700676,39.7894858221627));
#49029=CARTESIAN_POINT('Ctrl Pts',(3.45499130789194,-3.47806613859367,39.8688577122162));
#49030=CARTESIAN_POINT('Ctrl Pts',(4.69765387924814,-1.40219731261544,39.9482296022695));
#49031=CARTESIAN_POINT('Ctrl Pts',(4.79625497710706,1.0159342797995,40.027601492323));
#49032=CARTESIAN_POINT('Ctrl Pts',(4.08267404777822,2.46201708819427,40.0805160856919));
#49033=CARTESIAN_POINT('Ctrl Pts',(3.57461543774186,3.05624720968413,40.1069733823764));
#49034=CARTESIAN_POINT('Ctrl Pts',(1.16918346556923,-4.36383719750629,-0.320920147129053));
#49035=CARTESIAN_POINT('Ctrl Pts',(1.8946107326977,-4.16947670058299,-0.294462850444586));
#49036=CARTESIAN_POINT('Ctrl Pts',(3.24594541476064,-3.41224896374509,-0.24154825707565));
#49037=CARTESIAN_POINT('Ctrl Pts',(4.48258575488109,-1.44364637546346,-0.162176367022246));
#49038=CARTESIAN_POINT('Ctrl Pts',(4.62712170766666,0.875927969712858,-0.0828044769688426));
#49039=CARTESIAN_POINT('Ctrl Pts',(3.64458116255458,2.98248116081162,-0.00343258691543892));
#49040=CARTESIAN_POINT('Ctrl Pts',(1.77418661813218,4.36232362711486,0.0759393031379646));
#49041=CARTESIAN_POINT('Ctrl Pts',(-0.52837360592073,4.67961139929734,0.155311193191369));
#49042=CARTESIAN_POINT('Ctrl Pts',(-2.70223496968603,3.85690448821556,0.234683083244771));
#49043=CARTESIAN_POINT('Ctrl Pts',(-4.21783163769356,2.09469156016015,0.314054973298176));
#49044=CARTESIAN_POINT('Ctrl Pts',(-4.70597715859854,-0.177798095133649,
0.393426863351579));
#49045=CARTESIAN_POINT('Ctrl Pts',(-4.04775531046147,-2.4069688489564,0.472798753404983));
#49046=CARTESIAN_POINT('Ctrl Pts',(-2.40351015490329,-4.04981138575499,
0.552170643458387));
#49047=CARTESIAN_POINT('Ctrl Pts',(-0.173774754931243,-4.70612667927193,
0.631542533511791));
#49048=CARTESIAN_POINT('Ctrl Pts',(2.0982915307903,-4.21604107122297,0.710914423565194));
#49049=CARTESIAN_POINT('Ctrl Pts',(3.85921878174909,-2.69893658616936,0.790286313618597));
#49050=CARTESIAN_POINT('Ctrl Pts',(4.68004880681062,-0.524377442655228,
0.869658203672002));
#49051=CARTESIAN_POINT('Ctrl Pts',(4.36082934025305,1.77791905463906,0.949030093725404));
#49052=CARTESIAN_POINT('Ctrl Pts',(2.97932147849509,3.64711831584472,1.02840198377881));
#49053=CARTESIAN_POINT('Ctrl Pts',(0.872057510020645,4.62788767559441,1.10777387383221));
#49054=CARTESIAN_POINT('Ctrl Pts',(-1.44763774336318,4.48131381605584,1.18714576388562));
#49055=CARTESIAN_POINT('Ctrl Pts',(-3.4146916437183,3.2431018434756,1.26651765393902));
#49056=CARTESIAN_POINT('Ctrl Pts',(-4.54993421956391,1.21487743324944,1.34588954399242));
#49057=CARTESIAN_POINT('Ctrl Pts',(-4.57682288978047,-1.10928842689199,
1.42526143404583));
#49058=CARTESIAN_POINT('Ctrl Pts',(-3.48880763512327,-3.16323408359086,
1.50463332409923));
#49059=CARTESIAN_POINT('Ctrl Pts',(-1.55092656265583,-4.44662291817823,
1.58400521415264));
#49060=CARTESIAN_POINT('Ctrl Pts',(0.764756787430318,-4.64682425288564,
1.66337710420604));
#49061=CARTESIAN_POINT('Ctrl Pts',(2.89414707692588,-3.71506948486699,1.74274899425944));
#49062=CARTESIAN_POINT('Ctrl Pts',(4.31852954453272,-1.87833201365734,1.82212088431284));
#49063=CARTESIAN_POINT('Ctrl Pts',(4.69092777401317,0.415962978544339,1.90149277436625));
#49064=CARTESIAN_POINT('Ctrl Pts',(3.92062638092659,2.60893030984735,1.98086466441965));
#49065=CARTESIAN_POINT('Ctrl Pts',(2.19526907961086,4.166367992464,2.06023655447306));
#49066=CARTESIAN_POINT('Ctrl Pts',(-0.0648509103551908,4.70888765420329,
2.13960844452646));
#49067=CARTESIAN_POINT('Ctrl Pts',(-2.30917336210229,4.10433270633116,2.21898033457986));
#49068=CARTESIAN_POINT('Ctrl Pts',(-3.99098629411059,2.49997139597969,2.29835222463327));
#49069=CARTESIAN_POINT('Ctrl Pts',(-4.70060379877146,0.286622587162194,
2.37772411468667));
#49070=CARTESIAN_POINT('Ctrl Pts',(-4.26516462266185,-1.99654684946062,
2.45709600474007));
#49071=CARTESIAN_POINT('Ctrl Pts',(-2.79074078525346,-3.79336189283582,
2.53646789479348));
#49072=CARTESIAN_POINT('Ctrl Pts',(-0.636498669757338,-4.66612237558061,
2.61583978484688));
#49073=CARTESIAN_POINT('Ctrl Pts',(1.6727931128258,-4.40222577592052,2.69521167490029));
#49074=CARTESIAN_POINT('Ctrl Pts',(3.5745961957893,-3.06595672140773,2.77458356495369));
#49075=CARTESIAN_POINT('Ctrl Pts',(4.60563555769302,-0.982827395940078,
2.85395545500709));
#49076=CARTESIAN_POINT('Ctrl Pts',(4.51475229214408,1.33971650772703,2.9333273450605));
#49077=CARTESIAN_POINT('Ctrl Pts',(3.32408536146356,3.33590843552402,3.0126992351139));
#49078=CARTESIAN_POINT('Ctrl Pts',(1.32367859446866,4.51948045233543,3.0920711251673));
#49079=CARTESIAN_POINT('Ctrl Pts',(-0.99917334822593,4.60211703465825,3.17144301522071));
#49080=CARTESIAN_POINT('Ctrl Pts',(-3.07862887492539,3.56368809395157,3.25081490527411));
#49081=CARTESIAN_POINT('Ctrl Pts',(-4.40813722212245,1.65715262164811,3.33018679532752));
#49082=CARTESIAN_POINT('Ctrl Pts',(-4.66383309925671,-0.653061561243739,
3.40955868538092));
#49083=CARTESIAN_POINT('Ctrl Pts',(-3.7834295566315,-2.80419139334385,3.48893057543432));
#49084=CARTESIAN_POINT('Ctrl Pts',(-1.98139094849014,-4.27222640899777,
3.56830246548773));
#49085=CARTESIAN_POINT('Ctrl Pts',(0.303310108968963,-4.69955652783259,
3.64767435554113));
#49086=CARTESIAN_POINT('Ctrl Pts',(2.51412549524875,-3.98208507877931,3.72704624559453));
#49087=CARTESIAN_POINT('Ctrl Pts',(4.11250547580833,-2.29458651873122,3.80641813564794));
#49088=CARTESIAN_POINT('Ctrl Pts',(4.70908822533748,-0.0481317617013215,
3.88579002570134));
#49089=CARTESIAN_POINT('Ctrl Pts',(4.15854750656441,2.21004778594118,3.96516191575474));
#49090=CARTESIAN_POINT('Ctrl Pts',(2.59499381998102,3.92986458478622,4.04453380580815));
#49091=CARTESIAN_POINT('Ctrl Pts',(0.399305382771643,4.69237506938503,4.12390569586155));
#49092=CARTESIAN_POINT('Ctrl Pts',(-1.89365296183344,4.3118333734777,4.20327758591496));
#49093=CARTESIAN_POINT('Ctrl Pts',(-3.72532163646561,2.88093861187248,4.28264947596836));
#49094=CARTESIAN_POINT('Ctrl Pts',(-4.64951020631435,0.748253581264596,
4.36202136602176));
#49095=CARTESIAN_POINT('Ctrl Pts',(-4.44108838142119,-1.56670436550815,
4.44139325607517));
#49096=CARTESIAN_POINT('Ctrl Pts',(-3.15082725699623,-3.5000165966844,4.52076514612857));
#49097=CARTESIAN_POINT('Ctrl Pts',(-1.09303158700481,-4.58073253206366,
4.60013703618198));
#49098=CARTESIAN_POINT('Ctrl Pts',(1.23102415819659,-4.54559216191169,4.67950892623538));
#49099=CARTESIAN_POINT('Ctrl Pts',(3.25520514328707,-3.40315560261561,4.75888081628878));
#49100=CARTESIAN_POINT('Ctrl Pts',(4.48642536074717,-1.43171787127954,4.83825270634219));
#49101=CARTESIAN_POINT('Ctrl Pts',(4.62476229086337,0.888483164446475,4.91762459639559));
#49102=CARTESIAN_POINT('Ctrl Pts',(3.63651736366295,2.99225166793745,4.99699648644899));
#49103=CARTESIAN_POINT('Ctrl Pts',(1.76242485596889,4.36711428835561,5.0763683765024));
#49104=CARTESIAN_POINT('Ctrl Pts',(-0.540990445577951,4.67815753457383,
5.15574026655579));
#49105=CARTESIAN_POINT('Ctrl Pts',(-2.71262167204403,3.84961196029596,5.23511215660921));
#49106=CARTESIAN_POINT('Ctrl Pts',(-4.22346426348642,2.08330943346152,5.3144840466626));
#49107=CARTESIAN_POINT('Ctrl Pts',(-4.70548030882309,-0.190482660036918,
5.39385593671601));
#49108=CARTESIAN_POINT('Ctrl Pts',(-4.04125176633447,-2.41787359917659,
5.47322782676941));
#49109=CARTESIAN_POINT('Ctrl Pts',(-2.39258323872581,-4.05627588142928,
5.55259971682282));
#49110=CARTESIAN_POINT('Ctrl Pts',(-0.161086730056731,-4.70657833738016,
5.63197160687622));
#49111=CARTESIAN_POINT('Ctrl Pts',(2.10965014949475,-4.21036872817968,5.71134349692963));
#49112=CARTESIAN_POINT('Ctrl Pts',(3.86648092226071,-2.68852261628773,5.79071538698303));
#49113=CARTESIAN_POINT('Ctrl Pts',(4.68144550067431,-0.511758346011949,
5.87008727703643));
#49114=CARTESIAN_POINT('Ctrl Pts',(4.3560203173275,1.78966912459444,5.94945916708984));
#49115=CARTESIAN_POINT('Ctrl Pts',(2.96947822656715,3.65513715781504,6.02883105714324));
#49116=CARTESIAN_POINT('Ctrl Pts',(0.859577812643608,4.63022186990077,6.10820294719665));
#49117=CARTESIAN_POINT('Ctrl Pts',(-1.45971385379671,4.47739478330096,6.18757483725004));
#49118=CARTESIAN_POINT('Ctrl Pts',(-3.42342245647396,3.23388423803426,6.26694672730346));
#49119=CARTESIAN_POINT('Ctrl Pts',(-4.55319292637122,1.20260665046377,6.34631861735685));
#49120=CARTESIAN_POINT('Ctrl Pts',(-4.57381567772605,-1.12162325523503,
6.42569050741026));
#49121=CARTESIAN_POINT('Ctrl Pts',(-3.48026705395609,-3.17262821862952,
6.50506239746367));
#49122=CARTESIAN_POINT('Ctrl Pts',(-1.5389330792829,-4.45078797045933,6.58443428751706));
#49123=CARTESIAN_POINT('Ctrl Pts',(0.777281587133017,-4.64474562433731,
6.66380617757047));
#49124=CARTESIAN_POINT('Ctrl Pts',(2.90415217940695,-3.70725352509678,6.74317806762387));
#49125=CARTESIAN_POINT('Ctrl Pts',(4.32357772900916,-1.86668267300916,6.82254995767728));
#49126=CARTESIAN_POINT('Ctrl Pts',(4.68978931390171,0.428607946391479,6.90192184773068));
#49127=CARTESIAN_POINT('Ctrl Pts',(3.91357860260037,2.61949061875875,6.98129373778408));
#49128=CARTESIAN_POINT('Ctrl Pts',(2.18402880626489,4.17227117454053,7.06066562783749));
#49129=CARTESIAN_POINT('Ctrl Pts',(-0.0775455730109682,4.70869570736982,
7.14003751789088));
#49130=CARTESIAN_POINT('Ctrl Pts',(-2.32023002234555,4.09809238840499,7.2194094079443));
#49131=CARTESIAN_POINT('Ctrl Pts',(-3.9977115739788,2.48920283459836,7.29878129799769));
#49132=CARTESIAN_POINT('Ctrl Pts',(-4.70135943497531,0.273948980040579,
7.37815318805111));
#49133=CARTESIAN_POINT('Ctrl Pts',(-4.25976654389442,-2.00803823967931,
7.4575250781045));
#49134=CARTESIAN_POINT('Ctrl Pts',(-2.78050395155417,-3.80087178893057,
7.53689696815791));
#49135=CARTESIAN_POINT('Ctrl Pts',(-0.623916751156424,-4.66782138348534,
7.61626885821132));
#49136=CARTESIAN_POINT('Ctrl Pts',(1.68465518880672,-4.39770002107047,7.69564074826471));
#49137=CARTESIAN_POINT('Ctrl Pts',(3.58284885369757,-3.05630866766671,7.77501263831812));
#49138=CARTESIAN_POINT('Ctrl Pts',(4.6082684683291,-0.970407287843808,7.85438452837152));
#49139=CARTESIAN_POINT('Ctrl Pts',(4.51112408430488,1.35188315933773,7.93375641842493));
#49140=CARTESIAN_POINT('Ctrl Pts',(3.31507985854782,3.3448578612472,8.01312830847833));
#49141=CARTESIAN_POINT('Ctrl Pts',(1.31148951705327,4.52303259187419,8.09250019853174));
#49142=CARTESIAN_POINT('Ctrl Pts',(-1.01157676786264,4.5994065946834,8.17187208858514));
#49143=CARTESIAN_POINT('Ctrl Pts',(-3.08822519121439,3.55537533164157,8.25124397863854));
#49144=CARTESIAN_POINT('Ctrl Pts',(-4.41258879365683,1.64526250750169,8.33061586869195));
#49145=CARTESIAN_POINT('Ctrl Pts',(-4.66205553306411,-0.665632621738795,
8.40998775874535));
#49146=CARTESIAN_POINT('Ctrl Pts',(-3.77585586390188,-2.81438111767656,
8.48935964879875));
#49147=CARTESIAN_POINT('Ctrl Pts',(-1.96986606400833,-4.27755260287526,
8.56873153885216));
#49148=CARTESIAN_POINT('Ctrl Pts',(0.315978748853086,-4.69872174221563,
8.64810342890556));
#49149=CARTESIAN_POINT('Ctrl Pts',(2.52485183790096,-3.97529266559641,8.72747531895897));
#49150=CARTESIAN_POINT('Ctrl Pts',(4.11867660790092,-2.28349109479901,8.80684720901236));
#49151=CARTESIAN_POINT('Ctrl Pts',(4.70920087275226,-0.0354361477303297,
8.88621909906579));
#49152=CARTESIAN_POINT('Ctrl Pts',(4.15257422864046,2.22125096648886,8.96559098911916));
#49153=CARTESIAN_POINT('Ctrl Pts',(2.58438969399899,3.93684626192698,9.04496287917259));
#49154=CARTESIAN_POINT('Ctrl Pts',(0.386653550348944,4.69343452202107,9.12433476922598));
#49155=CARTESIAN_POINT('Ctrl Pts',(-1.90527054232303,4.30671252129195,9.20370665927939));
#49156=CARTESIAN_POINT('Ctrl Pts',(-3.7330749481299,2.87088488312254,9.28307854933279));
#49157=CARTESIAN_POINT('Ctrl Pts',(-4.65151055959357,0.735716042020416,
9.3624504393862));
#49158=CARTESIAN_POINT('Ctrl Pts',(-4.43684849468422,-1.57867159843805,
9.4418223294396));
#49159=CARTESIAN_POINT('Ctrl Pts',(-3.14137995726738,-3.50849833184732,
9.52119421949301));
#49160=CARTESIAN_POINT('Ctrl Pts',(-1.08067821558679,-4.58366263754791,
9.6005661095464));
#49161=CARTESIAN_POINT('Ctrl Pts',(1.24327434737007,-4.54225687050701,9.67993799959982));
#49162=CARTESIAN_POINT('Ctrl Pts',(3.26436803124868,-3.39436738392564,9.75930988965321));
#49163=CARTESIAN_POINT('Ctrl Pts',(4.49026888827119,-1.41961751592476,9.83868177970662));
#49164=CARTESIAN_POINT('Ctrl Pts',(4.62235018315245,0.900948036685318,9.91805366976003));
#49165=CARTESIAN_POINT('Ctrl Pts',(3.62843720481635,3.00204464177353,9.99742555981342));
#49166=CARTESIAN_POINT('Ctrl Pts',(1.7506449547965,4.37184981703879,10.0767974498668));
#49167=CARTESIAN_POINT('Ctrl Pts',(-0.553600531224886,4.67668205379884,
10.1561693399202));
#49168=CARTESIAN_POINT('Ctrl Pts',(-2.72299015321387,3.84228489391363,10.2355412299736));
#49169=CARTESIAN_POINT('Ctrl Pts',(-4.22906540111646,2.07191563862441,10.314913120027));
#49170=CARTESIAN_POINT('Ctrl Pts',(-4.70494967818453,-0.203167680126261,
10.3942850100804));
#49171=CARTESIAN_POINT('Ctrl Pts',(-4.03471862787632,-2.42875980170217,
10.4736569001339));
#49172=CARTESIAN_POINT('Ctrl Pts',(-2.38163905051565,-4.06271141155209,
10.5530287901872));
#49173=CARTESIAN_POINT('Ctrl Pts',(-0.148397472117971,-4.70699551420709,
10.6324006802407));
#49174=CARTESIAN_POINT('Ctrl Pts',(2.12099340201542,-4.20466592835908,10.7117725702941));
#49175=CARTESIAN_POINT('Ctrl Pts',(3.87371497815709,-2.67808902923296,10.7911444603475));
#49176=CARTESIAN_POINT('Ctrl Pts',(4.68280815994238,-0.499135570435235,
10.8705163504009));
#49177=CARTESIAN_POINT('Ctrl Pts',(4.35117963918574,1.80140620850268,10.9498882404543));
#49178=CARTESIAN_POINT('Ctrl Pts',(2.95961338949625,3.66312942239435,11.0292601305077));
#49179=CARTESIAN_POINT('Ctrl Pts',(0.847091869118581,4.6325224171902,11.1086320205611));
#49180=CARTESIAN_POINT('Ctrl Pts',(-1.47177935557031,4.47344320507298,11.1880039106145));
#49181=CARTESIAN_POINT('Ctrl Pts',(-3.43212838697064,3.22464312999856,11.2673758006679));
#49182=CARTESIAN_POINT('Ctrl Pts',(-4.55641854019224,1.19032712608301,11.3467476907213));
#49183=CARTESIAN_POINT('Ctrl Pts',(-4.5707752224844,-1.13394993100199,11.4261195807747));
#49184=CARTESIAN_POINT('Ctrl Pts',(-3.47170117781866,-3.1819992948505,11.5054914708281));
#49185=CARTESIAN_POINT('Ctrl Pts',(-1.52692841071655,-4.45492067370938,
11.5848633608815));
#49186=CARTESIAN_POINT('Ctrl Pts',(0.789800737437414,-4.64263323725232,
11.6642352509349));
#49187=CARTESIAN_POINT('Ctrl Pts',(2.91413617414593,-3.69941062049495,11.7436071409883));
#49188=CARTESIAN_POINT('Ctrl Pts',(4.32859448916348,-1.85501976509151,11.8229790310417));
#49189=CARTESIAN_POINT('Ctrl Pts',(4.68861676780219,0.441249799071602,11.9023509210951));
#49190=CARTESIAN_POINT('Ctrl Pts',(3.90650237988148,2.63003188887072,11.9817228111485));
#49191=CARTESIAN_POINT('Ctrl Pts',(2.17277265911798,4.17814403201782,12.0610947012019));
#49192=CARTESIAN_POINT('Ctrl Pts',(-0.0902396720559702,4.70846953713027,
12.1404665912553));
#49193=CARTESIAN_POINT('Ctrl Pts',(-2.33126981885919,4.09182228501836,12.2198384813087));
#49194=CARTESIAN_POINT('Ctrl Pts',(-4.00440779796651,2.47841618137099,12.2992103713621));
#49195=CARTESIAN_POINT('Ctrl Pts',(-4.70208090109554,0.261273381822832,
12.3785822614155));
#49196=CARTESIAN_POINT('Ctrl Pts',(-4.25433750459725,-2.01951503521857,
12.4579541514689));
#49197=CARTESIAN_POINT('Ctrl Pts',(-2.7702469087954,-3.80835405980145,12.5373260415224));
#49198=CARTESIAN_POINT('Ctrl Pts',(-0.611330297848498,-4.66948646506541,
12.6166979315757));
#49199=CARTESIAN_POINT('Ctrl Pts',(1.69650502049761,-4.3931423031724,12.6960698216292));
#49200=CARTESIAN_POINT('Ctrl Pts',(3.59107547100067,-3.04663840028217,12.7754417116826));
#49201=CARTESIAN_POINT('Ctrl Pts',(4.61086788547872,-0.957980126702884,
12.854813601736));
#49202=CARTESIAN_POINT('Ctrl Pts',(4.50746308903707,1.36403998528818,12.9341854917894));
#49203=CARTESIAN_POINT('Ctrl Pts',(3.30605026120632,3.35378297611432,13.0135573818428));
#49204=CARTESIAN_POINT('Ctrl Pts',(1.29929090756384,4.52655185743172,13.0929292718962));
#49205=CARTESIAN_POINT('Ctrl Pts',(-1.02397283522957,4.59666272563134,13.1723011619496));
#49206=CARTESIAN_POINT('Ctrl Pts',(-3.09779906188647,3.54703672840752,13.251673052003));
#49207=CARTESIAN_POINT('Ctrl Pts',(-4.41700829392973,1.63336043537625,13.3310449420564));
#49208=CARTESIAN_POINT('Ctrl Pts',(-4.66024408245374,-0.67819884433063,
13.4104168321098));
#49209=CARTESIAN_POINT('Ctrl Pts',(-3.76825472776737,-2.82455038672626,
13.4897887221632));
#49210=CARTESIAN_POINT('Ctrl Pts',(-1.95832686228722,-4.28284770695163,
13.5691606122166));
#49211=CARTESIAN_POINT('Ctrl Pts',(0.328645092163131,-4.69785280568621,
13.64853250227));
#49212=CARTESIAN_POINT('Ctrl Pts',(2.53555982960612,-3.96847135947639,13.7279043923234));
#49213=CARTESIAN_POINT('Ctrl Pts',(4.12481780492351,-2.2723790741605,13.8072762823768));
#49214=CARTESIAN_POINT('Ctrl Pts',(4.7092792930909,-0.0227402762048894,
13.8866481724302));
#49215=CARTESIAN_POINT('Ctrl Pts',(4.14657076927425,2.23243800269952,13.9660200624836));
#49216=CARTESIAN_POINT('Ctrl Pts',(2.57376678434109,3.94379932556401,14.045391952537));
#49217=CARTESIAN_POINT('Ctrl Pts',(0.373998907678603,4.69445986217284,14.1247638425904));
#49218=CARTESIAN_POINT('Ctrl Pts',(-1.91687427506185,4.30156036736702,14.2041357326438));
#49219=CARTESIAN_POINT('Ctrl Pts',(-3.7408011273265,2.86081028841297,14.2835076226972));
#49220=CARTESIAN_POINT('Ctrl Pts',(-4.65347710509724,0.723173155497658,
14.3628795127506));
#49221=CARTESIAN_POINT('Ctrl Pts',(-4.43257636036315,-1.59062735738022,
14.442251402804));
#49222=CARTESIAN_POINT('Ctrl Pts',(-3.13190982558595,-3.51695456679423,
14.5216232928574));
#49223=CARTESIAN_POINT('Ctrl Pts',(-1.06831698966085,-4.58655942838405,
14.6009951829108));
#49224=CARTESIAN_POINT('Ctrl Pts',(1.25551550026611,-4.53888856539661,14.6803670729642));
#49225=CARTESIAN_POINT('Ctrl Pts',(3.27350719336465,-3.38555449453801,14.7597389630177));
#49226=CARTESIAN_POINT('Ctrl Pts',(4.49407977994485,-1.40750684260771,14.839110853071));
#49227=CARTESIAN_POINT('Ctrl Pts',(4.61990447960734,0.913406360718275,14.9184827431245));
#49228=CARTESIAN_POINT('Ctrl Pts',(3.62033067402261,3.01181579636398,14.9978546331779));
#49229=CARTESIAN_POINT('Ctrl Pts',(1.73885232971199,4.37655357055661,15.0772265232313));
#49230=CARTESIAN_POINT('Ctrl Pts',(-0.566206593232149,4.67517258229866,
15.1565984132847));
#49231=CARTESIAN_POINT('Ctrl Pts',(-2.73333884334193,3.83492990131171,15.2359703033381));
#49232=CARTESIAN_POINT('Ctrl Pts',(-4.23463580135657,2.06050678483865,15.3153421933915));
#49233=CARTESIAN_POINT('Ctrl Pts',(-4.70438485136804,-0.21585122356682,
15.3947140834449));
#49234=CARTESIAN_POINT('Ctrl Pts',(-4.02815616456562,-2.43962835168982,
15.4740859734983));
#49235=CARTESIAN_POINT('Ctrl Pts',(-2.3706775522472,-4.06911741336723,15.5534578635517));
#49236=CARTESIAN_POINT('Ctrl Pts',(-0.135707135607595,-4.70737847998642,
15.6328297536051));
#49237=CARTESIAN_POINT('Ctrl Pts',(2.13232123888424,-4.19893256848759,15.7122016436585));
#49238=CARTESIAN_POINT('Ctrl Pts',(3.88092087939525,-2.66763597748263,15.7915735337119));
#49239=CARTESIAN_POINT('Ctrl Pts',(4.6841367839613,-0.486509167079024,15.8709454237653));
#49240=CARTESIAN_POINT('Ctrl Pts',(4.34630733610955,1.81313019956284,15.9503173138187));
#49241=CARTESIAN_POINT('Ctrl Pts',(2.94972704158046,3.67109506287253,16.0296892038721));
#49242=CARTESIAN_POINT('Ctrl Pts',(0.834599768811967,4.63478929472454,16.1090610939255));
#49243=CARTESIAN_POINT('Ctrl Pts',(-1.48383416024523,4.46945911326284,16.1884329839789));
#49244=CARTESIAN_POINT('Ctrl Pts',(-3.44080937235088,3.21537858488636,16.2678048740323));
#49245=CARTESIAN_POINT('Ctrl Pts',(-4.55961103731638,1.17803895016983,16.3471767640857));
#49246=CARTESIAN_POINT('Ctrl Pts',(-4.5677015463797,-1.14626836492032,16.4265486541391));
#49247=CARTESIAN_POINT('Ctrl Pts',(-3.4631100686894,-3.19134724418507,16.5059205441925));
#49248=CARTESIAN_POINT('Ctrl Pts',(-1.51491264465833,-4.45902099747165,
16.5852924342459));
#49249=CARTESIAN_POINT('Ctrl Pts',(0.802314148161232,-4.64048710795702,
16.6646643242993));
#49250=CARTESIAN_POINT('Ctrl Pts',(2.92409898707282,-3.69154082613136,16.7440362143527));
#49251=CARTESIAN_POINT('Ctrl Pts',(4.33357979136326,-1.84334337837345,16.8234081044061));
#49252=CARTESIAN_POINT('Ctrl Pts',(4.68741013889918,0.453888451717908,16.9027799944596));
#49253=CARTESIAN_POINT('Ctrl Pts',(3.89939777427618,2.64055403030628,16.9821518845129));
#49254=CARTESIAN_POINT('Ctrl Pts',(2.16150070095874,4.18398654725935,17.0615237745663));
#49255=CARTESIAN_POINT('Ctrl Pts',(-0.102933079310061,4.70820909782832,
17.1408956646198));
#49256=CARTESIAN_POINT('Ctrl Pts',(-2.34229273922368,4.08552253105771,17.2202675546731));
#49257=CARTESIAN_POINT('Ctrl Pts',(-4.01107478934828,2.46761134605149,17.2996394447266));
#49258=CARTESIAN_POINT('Ctrl Pts',(-4.70276843368481,0.248596203073432,
17.37901133478));
#49259=CARTESIAN_POINT('Ctrl Pts',(-4.24887708766866,-2.03097775393694,
17.4583832248334));
#49260=CARTESIAN_POINT('Ctrl Pts',(-2.75997059360591,-3.81580751573978,
17.5377551148868));
#49261=CARTESIAN_POINT('Ctrl Pts',(-0.598737773532647,-4.6711197519463,
17.6171270049402));
#49262=CARTESIAN_POINT('Ctrl Pts',(1.70833944819094,-4.38854860755889,17.6964988949936));
#49263=CARTESIAN_POINT('Ctrl Pts',(3.5992817914533,-3.03695363259626,17.775870785047));
#49264=CARTESIAN_POINT('Ctrl Pts',(4.61342283197251,-0.945531571192997,
17.8552426751004));
#49265=CARTESIAN_POINT('Ctrl Pts',(4.50379002440264,1.37615964733967,17.9346145651538));
#49266=CARTESIAN_POINT('Ctrl Pts',(3.29695756540449,3.36273516855535,18.0139864552072));
#49267=CARTESIAN_POINT('Ctrl Pts',(1.28715662605536,4.52994106929151,18.0933583452606));
#49268=CARTESIAN_POINT('Ctrl Pts',(-1.03650075501039,4.59406889295398,18.172730235314));
#49269=CARTESIAN_POINT('Ctrl Pts',(-3.10708740551261,3.53832597274458,18.2521021253674));
#49270=CARTESIAN_POINT('Ctrl Pts',(-4.42189226956141,1.62210042840545,18.3314740154208));
#49271=CARTESIAN_POINT('Ctrl Pts',(-4.65746145505438,-0.691994213306935,
18.4108459054742));
#49272=CARTESIAN_POINT('Ctrl Pts',(-3.7623932789572,-2.83237457985889,18.4902177955276));
#49273=CARTESIAN_POINT('Ctrl Pts',(-1.94345928697736,-4.29245481019949,
18.569589685581));
#49274=CARTESIAN_POINT('Ctrl Pts',(0.335233909124166,-4.68912434583344,
18.6489615756345));
#49275=CARTESIAN_POINT('Ctrl Pts',(3.29668819545067,-3.73492805813089,18.7547907623723));
#49276=CARTESIAN_POINT('Ctrl Pts',(5.339103029404,-0.0175478502153651,18.8870772457947));
#49277=CARTESIAN_POINT('Ctrl Pts',(2.90621803008022,4.48249178265512,19.0458210259014));
#49278=CARTESIAN_POINT('Ctrl Pts',(-2.18656320946377,4.86959394496076,19.2045648060083));
#49279=CARTESIAN_POINT('Ctrl Pts',(-5.27828887711238,0.806568563691633,
19.363308586115));
#49280=CARTESIAN_POINT('Ctrl Pts',(-3.54020456892039,-3.99752392897296,
19.5220523662219));
#49281=CARTESIAN_POINT('Ctrl Pts',(1.43734916996113,-5.14215993940115,19.6807961463287));
#49282=CARTESIAN_POINT('Ctrl Pts',(5.09974667860479,-1.58211192901293,19.8395399264355));
#49283=CARTESIAN_POINT('Ctrl Pts',(4.09539160933933,3.42571876325583,19.9982837065423));
#49284=CARTESIAN_POINT('Ctrl Pts',(-0.656009676029552,5.29932988758688,
20.1570274866491));
#49285=CARTESIAN_POINT('Ctrl Pts',(-4.80798654830356,2.32253130646633,20.3157712667559));
#49286=CARTESIAN_POINT('Ctrl Pts',(-4.5587807483591,-2.77696271962182,20.4745150468627));
#49287=CARTESIAN_POINT('Ctrl Pts',(-0.141143605831918,-5.34031031892967,
20.6332588269695));
#49288=CARTESIAN_POINT('Ctrl Pts',(4.41154214902265,-3.00742829557661,20.7920026070763));
#49289=CARTESIAN_POINT('Ctrl Pts',(4.83176599740626,1.2132097937891,20.9242890904987));
#49290=CARTESIAN_POINT('Ctrl Pts',(2.93038174053082,3.67602118591258,21.0301182772365));
#49291=CARTESIAN_POINT('Ctrl Pts',(0.82729199276626,4.63872722375956,21.1094901672899));
#49292=CARTESIAN_POINT('Ctrl Pts',(-1.49865065220701,4.46452630956661,21.1888620573433));
#49293=CARTESIAN_POINT('Ctrl Pts',(-3.44799414715959,3.20657754587673,21.2682339473967));
#49294=CARTESIAN_POINT('Ctrl Pts',(-4.56354990278301,1.16548416044547,21.3476058374502));
#49295=CARTESIAN_POINT('Ctrl Pts',(-4.56418179760212,-1.1584417781363,21.4269777275035));
#49296=CARTESIAN_POINT('Ctrl Pts',(-3.45471245456607,-3.20074439226419,
21.506349617557));
#49297=CARTESIAN_POINT('Ctrl Pts',(-1.50277006074114,-4.46305057284728,
21.5857215076104));
#49298=CARTESIAN_POINT('Ctrl Pts',(0.814760394348267,-4.63832755437973,
21.6650933976638));
#49299=CARTESIAN_POINT('Ctrl Pts',(2.93407303175,-3.6836334512587,21.7444652877172));
#49300=CARTESIAN_POINT('Ctrl Pts',(4.33851638857388,-1.83165928184362,21.8238371777706));
#49301=CARTESIAN_POINT('Ctrl Pts',(4.68617856238765,0.466526807638465,21.903209067824));
#49302=CARTESIAN_POINT('Ctrl Pts',(3.89225998228531,2.65105540897445,21.9825809578774));
#49303=CARTESIAN_POINT('Ctrl Pts',(2.1502156260726,4.18979944864558,22.0619528479308));
#49304=CARTESIAN_POINT('Ctrl Pts',(-0.115627163561327,4.70791408521783,
22.1413247379842));
#49305=CARTESIAN_POINT('Ctrl Pts',(-2.35329778315663,4.07919314165102,22.2206966280376));
#49306=CARTESIAN_POINT('Ctrl Pts',(-4.01771326340777,2.45678878743819,22.300068518091));
#49307=CARTESIAN_POINT('Ctrl Pts',(-4.7034211013359,0.235916647177708,22.3794404081444));
#49308=CARTESIAN_POINT('Ctrl Pts',(-4.24338680893675,-2.04242454395301,
22.4588122981978));
#49309=CARTESIAN_POINT('Ctrl Pts',(-2.74967243806091,-3.82323548987737,
22.5381841882512));
#49310=CARTESIAN_POINT('Ctrl Pts',(-0.586144182924564,-4.67271481097619,
22.6175560783046));
#49311=CARTESIAN_POINT('Ctrl Pts',(1.7201676224087,-4.38393110573301,22.696927968358));
#49312=CARTESIAN_POINT('Ctrl Pts',(3.60745033643733,-3.02723150865538,22.7762998584114));
#49313=CARTESIAN_POINT('Ctrl Pts',(4.61596616842609,-0.933105005158016,
22.8556717484649));
#49314=CARTESIAN_POINT('Ctrl Pts',(4.50004284053894,1.38832380607303,22.9350436385182));
#49315=CARTESIAN_POINT('Ctrl Pts',(3.28791904717806,3.37156001439376,23.0144155285717));
#49316=CARTESIAN_POINT('Ctrl Pts',(1.27486544641681,4.53349166431032,23.093787418625));
#49317=CARTESIAN_POINT('Ctrl Pts',(-1.04874255247445,4.59107478042505,23.1731593086785));
#49318=CARTESIAN_POINT('Ctrl Pts',(-3.11687918839179,3.53028224171763,23.2525311987318));
#49319=CARTESIAN_POINT('Ctrl Pts',(-4.42575095234051,1.60952076333037,23.3319030887853));
#49320=CARTESIAN_POINT('Ctrl Pts',(-4.6565195809412,-0.703316410525592,
23.4112749788386));
#49321=CARTESIAN_POINT('Ctrl Pts',(-3.75297034643954,-2.84482726347037,
23.4906468688921));
#49322=CARTESIAN_POINT('Ctrl Pts',(-1.93520584271877,-4.29334449199004,
23.5700187589454));
#49323=CARTESIAN_POINT('Ctrl Pts',(0.353970520843478,-4.69601250539774,
23.6493906489989));
#49324=CARTESIAN_POINT('Ctrl Pts',(2.55692044899663,-3.95474226694855,23.7287625390522));
#49325=CARTESIAN_POINT('Ctrl Pts',(4.13701021543862,-2.25010556593857,23.8081344291057));
#49326=CARTESIAN_POINT('Ctrl Pts',(4.70933345050753,0.00265187040687223,
23.887506319159));
#49327=CARTESIAN_POINT('Ctrl Pts',(4.13447348097035,2.25476331699259,23.9668782092125));
#49328=CARTESIAN_POINT('Ctrl Pts',(2.55246492296808,3.95761941039203,24.0462500992659));
#49329=CARTESIAN_POINT('Ctrl Pts',(0.348681559517371,4.69640817546236,24.1256219893193));
#49330=CARTESIAN_POINT('Ctrl Pts',(-1.94003986003887,4.29116230431301,24.2049938793727));
#49331=CARTESIAN_POINT('Ctrl Pts',(-3.75617186389469,2.84059879415982,24.2843657694261));
#49332=CARTESIAN_POINT('Ctrl Pts',(-4.65730871585138,0.698071705307978,
24.3637376594795));
#49333=CARTESIAN_POINT('Ctrl Pts',(-4.42393547340455,-1.61450410580135,
24.4431095495329));
#49334=CARTESIAN_POINT('Ctrl Pts',(-3.11290134185147,-3.5337902903817,24.5224814395863));
#49335=CARTESIAN_POINT('Ctrl Pts',(-1.0435713337136,-4.59225298213718,24.6018533296397));
#49336=CARTESIAN_POINT('Ctrl Pts',(1.27997034141094,-4.5320530122236,24.6812252196931));
#49337=CARTESIAN_POINT('Ctrl Pts',(3.29171407453406,-3.36785496006151,24.7605971097465));
#49338=CARTESIAN_POINT('Ctrl Pts',(4.50160354518617,-1.38325489424899,24.8399689997999));
#49339=CARTESIAN_POINT('Ctrl Pts',(4.61491235636141,0.938303002019797,24.9193408898533));
#49340=CARTESIAN_POINT('Ctrl Pts',(3.60403873246226,3.03129236389504,24.9987127799067));
#49341=CARTESIAN_POINT('Ctrl Pts',(1.71522925073975,4.3858656155773,25.0780846699601));
#49342=CARTESIAN_POINT('Ctrl Pts',(-0.591406279867446,4.67205171125385,
25.1574565600135));
#49343=CARTESIAN_POINT('Ctrl Pts',(-2.75397654975454,3.82013635147998,25.2368284500669));
#49344=CARTESIAN_POINT('Ctrl Pts',(-4.2456842279451,2.03764423221396,25.3162003401203));
#49345=CARTESIAN_POINT('Ctrl Pts',(-4.70315262587087,-0.24121351177037,
25.3955722301737));
#49346=CARTESIAN_POINT('Ctrl Pts',(-4.01494345438624,-2.4613121782045,25.4749441202271));
#49347=CARTESIAN_POINT('Ctrl Pts',(-2.34870294433969,-4.08184064605008,
25.5543160102806));
#49348=CARTESIAN_POINT('Ctrl Pts',(-0.110323595817837,-4.70804176751889,
25.6336879003339));
#49349=CARTESIAN_POINT('Ctrl Pts',(2.15493033644811,-4.1873743354938,25.7130597903874));
#49350=CARTESIAN_POINT('Ctrl Pts',(3.89524800861274,-2.64667178393831,25.7924316804407));
#49351=CARTESIAN_POINT('Ctrl Pts',(4.68669188786451,-0.461245844124039,
25.8718035704942));
#49352=CARTESIAN_POINT('Ctrl Pts',(4.33646799704899,1.83653856236848,25.9511754605475));
#49353=CARTESIAN_POINT('Ctrl Pts',(2.92989010076147,3.68694624017715,26.030547350601));
#49354=CARTESIAN_POINT('Ctrl Pts',(0.809597461130217,4.63922197479579,26.1099192406544));
#49355=CARTESIAN_POINT('Ctrl Pts',(-1.50791132801882,4.46139350509784,26.1892911307078));
#49356=CARTESIAN_POINT('Ctrl Pts',(-3.45809625536759,3.19677945268506,26.2686630207611));
#49357=CARTESIAN_POINT('Ctrl Pts',(-4.56589658927499,1.15343700154949,26.3480349108146));
#49358=CARTESIAN_POINT('Ctrl Pts',(-4.56145462047572,-1.170880150074,26.427406800868));
#49359=CARTESIAN_POINT('Ctrl Pts',(-3.44585240273711,-3.20997348883872,
26.5067786909214));
#49360=CARTESIAN_POINT('Ctrl Pts',(-1.49084816695666,-4.46712439087817,
26.5861505809748));
#49361=CARTESIAN_POINT('Ctrl Pts',(0.827323382358012,-4.6360936791118,26.6655224710282));
#49362=CARTESIAN_POINT('Ctrl Pts',(2.9439607869795,-3.67572080893307,26.7448943610816));
#49363=CARTESIAN_POINT('Ctrl Pts',(4.34345586023946,-1.81995048576826,26.824266251135));
#49364=CARTESIAN_POINT('Ctrl Pts',(4.68489470002155,0.479155747337646,26.9036381411885));
#49365=CARTESIAN_POINT('Ctrl Pts',(3.88510356071688,2.66154070098535,26.9830100312418));
#49366=CARTESIAN_POINT('Ctrl Pts',(2.13890979355249,4.1955802310934,27.0623819212952));
#49367=CARTESIAN_POINT('Ctrl Pts',(-0.128317664924755,4.70758570366646,
27.1417538113486));
#49368=CARTESIAN_POINT('Ctrl Pts',(-2.36428722425266,4.07283371889059,27.221125701402));
#49369=CARTESIAN_POINT('Ctrl Pts',(-4.02432164901364,2.44594845525754,27.3004975914554));
#49370=CARTESIAN_POINT('Ctrl Pts',(-4.70404022775981,0.223235561938782,
27.3798694815088));
#49371=CARTESIAN_POINT('Ctrl Pts',(-4.2378650192401,-2.05385702014473,27.4592413715622));
#49372=CARTESIAN_POINT('Ctrl Pts',(-2.73935527238859,-3.83063457825638,
27.5386132616157));
#49373=CARTESIAN_POINT('Ctrl Pts',(-0.573544644643281,-4.67427803207058,
27.617985151669));
#49374=CARTESIAN_POINT('Ctrl Pts',(1.73198018901762,-4.37927770361132,27.6973570417225));
#49375=CARTESIAN_POINT('Ctrl Pts',(3.61559848230692,-3.01749501991908,27.7767289317758));
#49376=CARTESIAN_POINT('Ctrl Pts',(4.61846498829774,-0.920657228486544,
27.8561008218292));
#49377=CARTESIAN_POINT('Ctrl Pts',(4.49628364593812,1.4004506259651,27.9354727118827));
#49378=CARTESIAN_POINT('Ctrl Pts',(3.278817559783,3.38041180777658,28.014844601936));
#49379=CARTESIAN_POINT('Ctrl Pts',(1.2626387736043,4.53691215562828,28.0942164919895));
#49380=CARTESIAN_POINT('Ctrl Pts',(-1.0611160230209,4.58823074465364,28.1735883820429));
#49381=CARTESIAN_POINT('Ctrl Pts',(-3.12638530517863,3.52186648015787,28.2529602720962));
#49382=CARTESIAN_POINT('Ctrl Pts',(-4.43007404713138,1.59758333661492,28.3323321621497));
#49383=CARTESIAN_POINT('Ctrl Pts',(-4.65460655700551,-0.715867571536754,
28.4117040522031));
#49384=CARTESIAN_POINT('Ctrl Pts',(-3.74528721238995,-2.85493472380806,
28.4910759422565));
#49385=CARTESIAN_POINT('Ctrl Pts',(-1.9236241928888,-4.29854609665053,28.5704478323099));
#49386=CARTESIAN_POINT('Ctrl Pts',(0.366629422130075,-4.69504115501931,
28.6498197223633));
#49387=CARTESIAN_POINT('Ctrl Pts',(2.56757292143854,-3.94783458032276,28.7291916124167));
#49388=CARTESIAN_POINT('Ctrl Pts',(4.14306134031087,-2.23894424024318,28.8085635024701));
#49389=CARTESIAN_POINT('Ctrl Pts',(4.70930918719419,0.0153479609406268,
28.8879353925235));
#49390=CARTESIAN_POINT('Ctrl Pts',(4.12837973995606,2.26590143281143,28.9673072825769));
#49391=CARTESIAN_POINT('Ctrl Pts',(2.54178612607819,3.96448633113712,29.0466791726303));
#49392=CARTESIAN_POINT('Ctrl Pts',(0.336019038035816,4.69733113443944,29.1260510626837));
#49393=CARTESIAN_POINT('Ctrl Pts',(-1.95160154390656,4.2859164707584,29.2054229527371));
#49394=CARTESIAN_POINT('Ctrl Pts',(-3.76381630954999,2.83046204151583,29.2847948427905));
#49395=CARTESIAN_POINT('Ctrl Pts',(-4.65917375325318,0.68551332408149,29.364166732844));
#49396=CARTESIAN_POINT('Ctrl Pts',(-4.41956678357008,-1.62642492174114,
29.4435386228973));
#49397=CARTESIAN_POINT('Ctrl Pts',(-3.10336312795443,-3.54216965665813,
29.5229105129507));
#49398=CARTESIAN_POINT('Ctrl Pts',(-1.03118708354684,-4.59504970367272,
29.6022824030041));
#49399=CARTESIAN_POINT('Ctrl Pts',(1.29218385191882,-4.52858581384264,29.6816542930575));
#49400=CARTESIAN_POINT('Ctrl Pts',(3.30078166125751,-3.3589684436152,29.761026183111));
#49401=CARTESIAN_POINT('Ctrl Pts',(4.50531636407018,-1.37111379547362,29.8403980731643));
#49402=CARTESIAN_POINT('Ctrl Pts',(4.61236597294397,0.950741138336453,29.9197699632178));
#49403=CARTESIAN_POINT('Ctrl Pts',(3.59585344010749,3.04099763527755,29.9991418532711));
#49404=CARTESIAN_POINT('Ctrl Pts',(1.70339896854746,4.39047383939912,30.0785137433246));
#49405=CARTESIAN_POINT('Ctrl Pts',(-0.603999721341074,4.67044033439209,
30.157885633378));
#49406=CARTESIAN_POINT('Ctrl Pts',(-2.76426541604165,3.81269790177148,30.2372575234314));
#49407=CARTESIAN_POINT('Ctrl Pts',(-4.25116217399222,2.02619069954299,30.3166294134847));
#49408=CARTESIAN_POINT('Ctrl Pts',(-4.70248523614609,-0.253892072197153,
30.3960013035382));
#49409=CARTESIAN_POINT('Ctrl Pts',(-4.00829330354932,-2.47212729713062,
30.4753731935915));
#49410=CARTESIAN_POINT('Ctrl Pts',(-2.33768999441463,-4.08815778444404,
30.554745083645));
#49411=CARTESIAN_POINT('Ctrl Pts',(-0.0976305770295779,-4.70832208445062,
30.6341169736984));
#49412=CARTESIAN_POINT('Ctrl Pts',(2.16621143281822,-4.18154954637921,30.7134888637517));
#49413=CARTESIAN_POINT('Ctrl Pts',(3.90236913245919,-2.63616079451278,30.7928607538052));
#49414=CARTESIAN_POINT('Ctrl Pts',(4.68791834918069,-0.448609108145992,
30.8722326438586));
#49415=CARTESIAN_POINT('Ctrl Pts',(4.33150103257305,1.84822276398574,30.951604533912));
#49416=CARTESIAN_POINT('Ctrl Pts',(2.91993965204555,3.69483166178228,31.0309764239654));
#49417=CARTESIAN_POINT('Ctrl Pts',(0.797087435456495,4.64138774513982,31.1103483140188));
#49418=CARTESIAN_POINT('Ctrl Pts',(-1.51993351608663,4.45731204731877,31.1897202040722));
#49419=CARTESIAN_POINT('Ctrl Pts',(-3.46670202742684,3.18744500086376,31.2690920941256));
#49420=CARTESIAN_POINT('Ctrl Pts',(-4.56898959830062,1.14112340748814,31.348463984179));
#49421=CARTESIAN_POINT('Ctrl Pts',(-4.5582814163153,-1.18317332211776,31.4278358742324));
#49422=CARTESIAN_POINT('Ctrl Pts',(-3.43718597090036,-3.21925164936547,
31.5072077642858));
#49423=CARTESIAN_POINT('Ctrl Pts',(-1.47879963105622,-4.47112740052042,
31.5865796543392));
#49424=CARTESIAN_POINT('Ctrl Pts',(0.839819025645787,-4.63384641358128,
31.6659515443926));
#49425=CARTESIAN_POINT('Ctrl Pts',(2.95385962660838,-3.66777069713875,31.745323434446));
#49426=CARTESIAN_POINT('Ctrl Pts',(4.34834656078651,-1.80823415734596,31.8246953244994));
#49427=CARTESIAN_POINT('Ctrl Pts',(4.68358589765892,0.491784220717852,31.9040672145528));
#49428=CARTESIAN_POINT('Ctrl Pts',(3.87791407680318,2.67200505116071,31.9834391046062));
#49429=CARTESIAN_POINT('Ctrl Pts',(2.12759097045539,4.20133136552371,32.0628109946597));
#49430=CARTESIAN_POINT('Ctrl Pts',(-0.141008586952624,4.70722265873437,
32.142182884713));
#49431=CARTESIAN_POINT('Ctrl Pts',(-2.37525876469618,4.06644493153793,32.2215547747665));
#49432=CARTESIAN_POINT('Ctrl Pts',(-4.03090116490581,2.43509021994207,32.3009266648198));
#49433=CARTESIAN_POINT('Ctrl Pts',(-4.7046249635928,0.21055292074912,32.3802985548733));
#49434=CARTESIAN_POINT('Ctrl Pts',(-4.23231253465933,-2.06527460388738,
32.4596704449267));
#49435=CARTESIAN_POINT('Ctrl Pts',(-2.72901814034772,-3.83800580642471,
32.5390423349801));
#49436=CARTESIAN_POINT('Ctrl Pts',(-0.560940967626579,-4.67580728979871,
32.6184142250335));
#49437=CARTESIAN_POINT('Ctrl Pts',(1.74378018318661,-4.37459246710163,32.6977861150869));
#49438=CARTESIAN_POINT('Ctrl Pts',(3.62372034116752,-3.00773660241476,32.7771580051403));
#49439=CARTESIAN_POINT('Ctrl Pts',(4.62093024500891,-0.90820275889168,32.8565298951936));
#49440=CARTESIAN_POINT('Ctrl Pts',(4.49249176942175,1.41256726642465,32.9359017852471));
#49441=CARTESIAN_POINT('Ctrl Pts',(3.26969224276534,3.38923903230456,33.0152736753005));
#49442=CARTESIAN_POINT('Ctrl Pts',(1.25040292311233,4.54029967186844,33.0946455653539));
#49443=CARTESIAN_POINT('Ctrl Pts',(-1.0734817808909,4.58535336114807,33.1740174554073));
#49444=CARTESIAN_POINT('Ctrl Pts',(-3.13586869918079,3.51342512115953,33.2533893454607));
#49445=CARTESIAN_POINT('Ctrl Pts',(-4.43436494347784,1.58563429849111,33.3327612355141));
#49446=CARTESIAN_POINT('Ctrl Pts',(-4.65265970284399,-0.728413529547759,
33.4121331255675));
#49447=CARTESIAN_POINT('Ctrl Pts',(-3.73757685708491,-2.8650214341048,33.4915050156209));
#49448=CARTESIAN_POINT('Ctrl Pts',(-1.91202856192598,-4.30371645893127,
33.5708769056743));
#49449=CARTESIAN_POINT('Ctrl Pts',(0.379285658714694,-4.69403568047687,
33.6502487957277));
#49450=CARTESIAN_POINT('Ctrl Pts',(2.57820673242699,-3.94089820033005,33.7296206857811));
#49451=CARTESIAN_POINT('Ctrl Pts',(4.14908235288389,-2.22776664161308,33.8089925758346));
#49452=CARTESIAN_POINT('Ctrl Pts',(4.70925069601633,0.0280439399230538,
33.8883644658879));
#49453=CARTESIAN_POINT('Ctrl Pts',(4.12225599334877,2.27702307976815,33.9677363559414));
#49454=CARTESIAN_POINT('Ctrl Pts',(2.53108885516031,3.9713244374868,34.0471082459947));
#49455=CARTESIAN_POINT('Ctrl Pts',(0.323354074324944,4.69821995261122,34.1264801360482));
#49456=CARTESIAN_POINT('Ctrl Pts',(-1.96314904328387,4.28063948661298,34.2058520261016));
#49457=CARTESIAN_POINT('Ctrl Pts',(-3.77143339930544,2.8203047167106,34.2852239161549));
#49458=CARTESIAN_POINT('Ctrl Pts',(-4.66100492718239,0.672949960456159,
34.3645958062084));
#49459=CARTESIAN_POINT('Ctrl Pts',(-4.41516597175719,-1.63833391661592,
34.4439676962618));
#49460=CARTESIAN_POINT('Ctrl Pts',(-3.09380235841604,-3.55052327799099,
34.5233395863151));
#49461=CARTESIAN_POINT('Ctrl Pts',(-1.01879533858015,-4.59781302779744,
34.6027114763686));
#49462=CARTESIAN_POINT('Ctrl Pts',(1.30438797066869,-4.52508570111899,34.6820833664219));
#49463=CARTESIAN_POINT('Ctrl Pts',(3.30982525747642,-3.35005751375522,34.7614552564754));
#49464=CARTESIAN_POINT('Ctrl Pts',(4.50899643773683,-1.3589627312672,34.8408271465288));
#49465=CARTESIAN_POINT('Ctrl Pts',(4.60978606625886,0.963172364544519,34.9201990365822));
#49466=CARTESIAN_POINT('Ctrl Pts',(3.58764201262861,3.05068080429907,34.9995709266356));
#49467=CARTESIAN_POINT('Ctrl Pts',(1.69155630583291,4.39505015269376,35.078942816689));
#49468=CARTESIAN_POINT('Ctrl Pts',(-0.616588772867267,4.66879501217076,
35.1583147067424));
#49469=CARTESIAN_POINT('Ctrl Pts',(-2.77453419129308,3.80523174088547,35.2376865967958));
#49470=CARTESIAN_POINT('Ctrl Pts',(-4.2566092220472,2.01472244025804,35.3170584868492));
#49471=CARTESIAN_POINT('Ctrl Pts',(-4.70178366815532,-0.266568787303772,
35.3964303769026));
#49472=CARTESIAN_POINT('Ctrl Pts',(-4.00161401992238,-2.48292444831838,
35.475802266956));
#49473=CARTESIAN_POINT('Ctrl Pts',(-2.3266600538588,-4.09444520958265,35.5551741570094));
#49474=CARTESIAN_POINT('Ctrl Pts',(-0.0849368486498902,-4.70856818069336,
35.6345460470628));
#49475=CARTESIAN_POINT('Ctrl Pts',(2.17747678488564,-4.17569436522607,35.7139179371162));
#49476=CARTESIAN_POINT('Ctrl Pts',(3.90946189338614,-2.62563064513239,35.7932898271696));
#49477=CARTESIAN_POINT('Ctrl Pts',(4.68911073810487,-0.435969111619298,
35.872661717223));
#49478=CARTESIAN_POINT('Ctrl Pts',(4.32650258619184,1.85989353248294,35.9520336072764));
#49479=CARTESIAN_POINT('Ctrl Pts',(2.90996798083354,3.70269022887686,36.0314054973299));
#49480=CARTESIAN_POINT('Ctrl Pts',(0.784571616449035,4.64351978128221,36.1107773873832));
#49481=CARTESIAN_POINT('Ctrl Pts',(-1.53194465708265,4.4531981932239,36.1901492774366));
#49482=CARTESIAN_POINT('Ctrl Pts',(-3.47528260305097,3.17808738228323,36.2695211674901));
#49483=CARTESIAN_POINT('Ctrl Pts',(-4.57204939932363,1.12880151959547,36.3488930575434));
#49484=CARTESIAN_POINT('Ctrl Pts',(-4.55507508198074,-1.19545789470598,
36.4282649475969));
#49485=CARTESIAN_POINT('Ctrl Pts',(-3.42849455715498,-3.2285064119582,36.5076368376502));
#49486=CARTESIAN_POINT('Ctrl Pts',(-1.4667403470503,-4.47509791343512,36.5870087277037));
#49487=CARTESIAN_POINT('Ctrl Pts',(0.852308565021146,-4.63156546866048,
36.6663806177571));
#49488=CARTESIAN_POINT('Ctrl Pts',(2.96373699720644,-3.65979392751645,36.7457525078104));
#49489=CARTESIAN_POINT('Ctrl Pts',(4.35320565699285,-1.79650468644589,36.8251243978639));
#49490=CARTESIAN_POINT('Ctrl Pts',(4.68224305439311,0.504409119747259,36.9044962879172));
#49491=CARTESIAN_POINT('Ctrl Pts',(3.87069640771237,2.68244998086059,36.9838681779707));
#49492=CARTESIAN_POINT('Ctrl Pts',(2.1162566837541,4.20705196413867,37.0632400680241));
#49493=CARTESIAN_POINT('Ctrl Pts',(-0.153698484112011,4.70682540110399,
37.1426119580775));
#49494=CARTESIAN_POINT('Ctrl Pts',(-2.38621304145417,4.06002658874194,37.2219838481309));
#49495=CARTESIAN_POINT('Ctrl Pts',(-4.03745138369124,2.42421428607825,37.3013557381843));
#49496=CARTESIAN_POINT('Ctrl Pts',(-4.7051755056078,0.197868749234187,37.3807276282377));
#49497=CARTESIAN_POINT('Ctrl Pts',(-4.22672928908836,-2.07667717695002,
37.4600995182911));
#49498=CARTESIAN_POINT('Ctrl Pts',(-2.71866117345227,-3.84534913947293,
37.5394714083445));
#49499=CARTESIAN_POINT('Ctrl Pts',(-0.548333213620079,-4.67730256316236,
37.6188432983979));
#49500=CARTESIAN_POINT('Ctrl Pts',(1.75556750333961,-4.36987543548734,37.6982151884513));
#49501=CARTESIAN_POINT('Ctrl Pts',(3.63181586235974,-2.99795632430491,37.7775870785047));
#49502=CARTESIAN_POINT('Ctrl Pts',(4.62336191621364,-0.895741688343936,
37.8569589685581));
#49503=CARTESIAN_POINT('Ctrl Pts',(4.48866724088475,1.42467364012841,37.9363308586115));
#49504=CARTESIAN_POINT('Ctrl Pts',(3.26054316123161,3.3980416234756,38.0157027486649));
#49505=CARTESIAN_POINT('Ctrl Pts',(1.23815798448111,4.54365418850126,38.0950746387183));
#49506=CARTESIAN_POINT('Ctrl Pts',(-1.08583973646279,4.58244265094544,38.1744465287717));
#49507=CARTESIAN_POINT('Ctrl Pts',(-3.1453293014664,3.50495822568428,38.2538184188251));
#49508=CARTESIAN_POINT('Ctrl Pts',(-4.43862360995231,1.57367373662757,38.3331903088785));
#49509=CARTESIAN_POINT('Ctrl Pts',(-4.65067903319431,-0.740954194968168,
38.412562198932));
#49510=CARTESIAN_POINT('Ctrl Pts',(-3.72983933538423,-2.87508731801368,
38.4919340889853));
#49511=CARTESIAN_POINT('Ctrl Pts',(-1.9004190363744,-4.30885554699714,38.5713059790388));
#49512=CARTESIAN_POINT('Ctrl Pts',(0.391939142907767,-4.69299607822647,
38.6506778690921));
#49513=CARTESIAN_POINT('Ctrl Pts',(2.588821796549,-3.93393319787887,38.7300497591456));
#49514=CARTESIAN_POINT('Ctrl Pts',(4.15507322474385,-2.21657281258971,38.8094216491989));
#49515=CARTESIAN_POINT('Ctrl Pts',(4.70915794841682,0.040739642006525,38.8887935392524));
#49516=CARTESIAN_POINT('Ctrl Pts',(4.11610234038245,2.28812831500406,38.9681654293058));
#49517=CARTESIAN_POINT('Ctrl Pts',(2.52037308462918,3.97813341921603,39.0475373193591));
#49518=CARTESIAN_POINT('Ctrl Pts',(0.310686955552019,4.69907511544173,39.1269092094126));
#49519=CARTESIAN_POINT('Ctrl Pts',(-1.97468264266246,4.27533046137757,39.2062810994659));
#49520=CARTESIAN_POINT('Ctrl Pts',(-3.77902238214566,2.81012864743349,39.2856529895194));
#49521=CARTESIAN_POINT('Ctrl Pts',(-4.66280353786911,0.660378394081937,
39.3650248795728));
#49522=CARTESIAN_POINT('Ctrl Pts',(-4.41073058968569,-1.65022475069991,
39.4443967696262));
#49523=CARTESIAN_POINT('Ctrl Pts',(-3.0842237862698,-3.55886290155649,39.5237686596796));
#49524=CARTESIAN_POINT('Ctrl Pts',(-1.00638734295308,-4.60052063353569,
39.603140549733));
#49525=CARTESIAN_POINT('Ctrl Pts',(1.3165658861068,-4.521594850557,39.6825124397864));
#49526=CARTESIAN_POINT('Ctrl Pts',(3.31887653668104,-3.34104229843822,39.7618843298398));
#49527=CARTESIAN_POINT('Ctrl Pts',(4.51258247789865,-1.34695556252384,39.8412562198932));
#49528=CARTESIAN_POINT('Ctrl Pts',(4.60729903172253,0.975909964327458,39.9206281099466));
#49529=CARTESIAN_POINT('Ctrl Pts',(3.92183073605334,2.36502208507764,39.9735427033156));
#49530=CARTESIAN_POINT('Ctrl Pts',(3.43378788736169,2.9358415841302,40.));
#49531=CARTESIAN_POINT('Ctrl Pts',(4.5177656910975,-0.000116631996953637,
0.887416697508071));
#49532=CARTESIAN_POINT('Ctrl Pts',(4.51716522512143,0.582848551743655,0.907954496247182));
#49533=CARTESIAN_POINT('Ctrl Pts',(4.40381632429852,1.16604045169665,0.928492294986294));
#49534=CARTESIAN_POINT('Ctrl Pts',(4.18378127438632,1.70573618195762,0.949030093725405));
#49535=CARTESIAN_POINT('Ctrl Pts',(3.90032671966707,2.40098547504095,0.975487390409873));
#49536=CARTESIAN_POINT('Ctrl Pts',(3.43982409908107,3.02405189544283,1.00194468709434));
#49537=CARTESIAN_POINT('Ctrl Pts',(2.85836212737567,3.49904666560206,1.02840198377881));
#49538=CARTESIAN_POINT('Ctrl Pts',(2.27690015567027,3.97404143576128,1.05485928046328));
#49539=CARTESIAN_POINT('Ctrl Pts',(1.57447883284546,4.30096455567785,1.08131657714775));
#49540=CARTESIAN_POINT('Ctrl Pts',(0.83665229586908,4.43999713904637,1.10777387383221));
#49541=CARTESIAN_POINT('Ctrl Pts',(0.0988257588927,4.57902972241489,1.13423117051668));
#49542=CARTESIAN_POINT('Ctrl Pts',(-0.674405992235245,4.53017176923536,
1.16068846720115));
#49543=CARTESIAN_POINT('Ctrl Pts',(-1.38886418452507,4.29937413054889,1.18714576388562));
#49544=CARTESIAN_POINT('Ctrl Pts',(-2.1033223768149,4.06857649186242,1.21360306057009));
#49545=CARTESIAN_POINT('Ctrl Pts',(-2.7590070102666,3.65583916766901,1.24006035725455));
#49546=CARTESIAN_POINT('Ctrl Pts',(-3.27605642296673,3.11143310386793,1.26651765393902));
#49547=CARTESIAN_POINT('Ctrl Pts',(-3.79310583566684,2.56702704006687,1.29297495062349));
#49548=CARTESIAN_POINT('Ctrl Pts',(-4.17152002761538,1.89095223665816,1.31943224730795));
#49549=CARTESIAN_POINT('Ctrl Pts',(-4.36520856862574,1.16555385826357,1.34588954399242));
#49550=CARTESIAN_POINT('Ctrl Pts',(-4.5588971096361,0.440155479868968,1.37234684067689));
#49551=CARTESIAN_POINT('Ctrl Pts',(-4.56785999970828,-0.334566473511511,
1.39880413736136));
#49552=CARTESIAN_POINT('Ctrl Pts',(-4.39100556896818,-1.06425172631823,
1.42526143404583));
#49553=CARTESIAN_POINT('Ctrl Pts',(-4.21415113822807,-1.79393697912495,
1.4517187307303));
#49554=CARTESIAN_POINT('Ctrl Pts',(-3.85147938667567,-2.4785855313579,1.47817602741476));
#49555=CARTESIAN_POINT('Ctrl Pts',(-3.3471633321549,-3.03480794657228,1.50463332409923));
#49556=CARTESIAN_POINT('Ctrl Pts',(-2.84284727763412,-3.59103036178665,
1.5310906207837));
#49557=CARTESIAN_POINT('Ctrl Pts',(-2.19688692014498,-4.01882663998244,
1.55754791746817));
#49558=CARTESIAN_POINT('Ctrl Pts',(-1.48795951638605,-4.26609166819824,
1.58400521415264));
#49559=CARTESIAN_POINT('Ctrl Pts',(-0.779032112627116,-4.51335669641404,
1.6104625108371));
#49560=CARTESIAN_POINT('Ctrl Pts',(-0.0071376625983989,-4.58009047464984,
1.63691980752157));
#49561=CARTESIAN_POINT('Ctrl Pts',(0.733707943998554,-4.4581649024313,1.66337710420604));
#49562=CARTESIAN_POINT('Ctrl Pts',(1.47455355059551,-4.33623933021276,1.68983440089051));
#49563=CARTESIAN_POINT('Ctrl Pts',(2.18435031376069,-4.02565440753988,1.71629169757498));
#49564=CARTESIAN_POINT('Ctrl Pts',(2.77664577327776,-3.56423903433516,1.74274899425944));
#49565=CARTESIAN_POINT('Ctrl Pts',(3.36894123279483,-3.10282366113044,1.76920629094391));
#49566=CARTESIAN_POINT('Ctrl Pts',(3.84373538866378,-2.49057783739389,1.79566358762838));
#49567=CARTESIAN_POINT('Ctrl Pts',(4.14319883817832,-1.80207242682533,1.82212088431285));
#49568=CARTESIAN_POINT('Ctrl Pts',(4.38955443642782,-1.23566887208905,1.84388615537792));
#49569=CARTESIAN_POINT('Ctrl Pts',(4.51725253079926,-0.617655577060232,
1.865651426443));
#49570=CARTESIAN_POINT('Ctrl Pts',(4.51787557461174,0.000108094638884985,
1.88741669750807));
#49571=CARTESIAN_POINT('Ctrl Pts',(1.3130361863565,-4.90075024188322,0.));
#49572=CARTESIAN_POINT('Ctrl Pts',(1.45293783176837,-4.85499972547219,-2.12441198790355E-17));
#49573=CARTESIAN_POINT('Ctrl Pts',(1.59048961161953,-4.80314405262584,1.00940613638452E-17));
#49574=CARTESIAN_POINT('Ctrl Pts',(1.72536214292615,-4.74546564178603,1.90819582357449E-17));
#49575=CARTESIAN_POINT('Ctrl Pts',(1.86158804346972,-4.68720846085782,2.81600435471549E-17));
#49576=CARTESIAN_POINT('Ctrl Pts',(1.9950813260058,-4.62301070705921,2.02661125299078E-16));
#49577=CARTESIAN_POINT('Ctrl Pts',(2.12548189098024,-4.5531145507957,1.45716771982052E-16));
#49578=CARTESIAN_POINT('Ctrl Pts',(2.25528319940241,-4.4835396027235,8.90341067708004E-17));
#49579=CARTESIAN_POINT('Ctrl Pts',(2.38202075670042,-4.40831802172382,2.31151513749735E-16));
#49580=CARTESIAN_POINT('Ctrl Pts',(2.50530950004123,-4.32764726500609,1.45716771982052E-16));
#49581=CARTESIAN_POINT('Ctrl Pts',(2.62711997854446,-4.24794377212644,6.13064155008212E-17));
#49582=CARTESIAN_POINT('Ctrl Pts',(2.74556437761014,-4.16292050991704,2.71959880884896E-17));
#49583=CARTESIAN_POINT('Ctrl Pts',(2.86023373369319,-4.07273466802712,-6.93889390390723E-17));
#49584=CARTESIAN_POINT('Ctrl Pts',(2.90383704830196,-4.03844127202745,-1.06115603492979E-16));
#49585=CARTESIAN_POINT('Ctrl Pts',(2.94689409015111,-4.00340109988822,-3.37664978924697E-16));
#49586=CARTESIAN_POINT('Ctrl Pts',(2.98938067979849,-3.96762172921426,-3.7470027081099E-16));
#49587=CARTESIAN_POINT('Ctrl Pts',(3.0045493035191,-3.95484772651792,-3.87922664316067E-16));
#49588=CARTESIAN_POINT('Ctrl Pts',(3.0196457209465,-3.94197897848992,-6.77418652234536E-17));
#49589=CARTESIAN_POINT('Ctrl Pts',(3.03465663588118,-3.92902653262601,-5.55111512312578E-17));
#49590=CARTESIAN_POINT('Ctrl Pts',(3.14512636784121,-3.83370567916447,3.44982654016709E-17));
#49591=CARTESIAN_POINT('Ctrl Pts',(3.25112830521826,-3.73372148501147,-5.43481287766778E-16));
#49592=CARTESIAN_POINT('Ctrl Pts',(3.35231677944077,-3.62929621080565,-5.13478148889135E-16));
#49593=CARTESIAN_POINT('Ctrl Pts',(3.36921809466263,-3.61185425914028,-5.08466782607427E-16));
#49594=CARTESIAN_POINT('Ctrl Pts',(3.38598504383309,-3.59428832049142,-2.69772873285687E-16));
#49595=CARTESIAN_POINT('Ctrl Pts',(3.40261591802407,-3.57659932769537,-2.63677968348475E-16));
#49596=CARTESIAN_POINT('Ctrl Pts',(3.50230123740107,-3.4705716543402,-2.26333319460949E-16));
#49597=CARTESIAN_POINT('Ctrl Pts',(3.59710111637371,-3.36012540834712,3.61502860778476E-17));
#49598=CARTESIAN_POINT('Ctrl Pts',(3.68681562587056,-3.2456540248488,-6.93889390390723E-17));
#49599=CARTESIAN_POINT('Ctrl Pts',(3.77658274630639,-3.13111551233192,-1.74990055122844E-16));
#49600=CARTESIAN_POINT('Ctrl Pts',(3.86125888590103,-3.01254641429341,-2.14930374901985E-16));
#49601=CARTESIAN_POINT('Ctrl Pts',(3.94059800782458,-2.89031628889591,-9.71445146547012E-17));
#49602=CARTESIAN_POINT('Ctrl Pts',(4.01127293754548,-2.78143424794555,7.77859507059291E-18));
#49603=CARTESIAN_POINT('Ctrl Pts',(4.07771240145114,-2.66964644715424,3.21618427330635E-16));
#49604=CARTESIAN_POINT('Ctrl Pts',(4.13970845878657,-2.55520469810914,3.46944695195361E-16));
#49605=CARTESIAN_POINT('Ctrl Pts',(4.1548365715119,-2.52727892743195,3.53124743599032E-16));
#49606=CARTESIAN_POINT('Ctrl Pts',(4.16969994577116,-2.49919510449128,-5.38761705143296E-16));
#49607=CARTESIAN_POINT('Ctrl Pts',(4.18429524804614,-2.47095685207318,-5.41233724504764E-16));
#49608=CARTESIAN_POINT('Ctrl Pts',(4.1935591046312,-2.45303361104087,-5.42802752155488E-16));
#49609=CARTESIAN_POINT('Ctrl Pts',(4.20271084368267,-2.4350560800449,-1.54877819716967E-16));
#49610=CARTESIAN_POINT('Ctrl Pts',(4.21174771778014,-2.41702978670704,-1.66533453693773E-16));
#49611=CARTESIAN_POINT('Ctrl Pts',(4.27617843190164,-2.28850670005169,-2.49635288749205E-16));
#49612=CARTESIAN_POINT('Ctrl Pts',(4.33481139244535,-2.15743447779131,-2.0244448216388E-16));
#49613=CARTESIAN_POINT('Ctrl Pts',(4.38745860743762,-2.0241905870822,-2.77555756156289E-16));
#49614=CARTESIAN_POINT('Ctrl Pts',(4.43978289169495,-1.89176399596928,-3.52206307982929E-16));
#49615=CARTESIAN_POINT('Ctrl Pts',(4.48619490051256,-1.75719157307499,-5.94819252645897E-16));
#49616=CARTESIAN_POINT('Ctrl Pts',(4.52646203441684,-1.6208264292839,-5.55111512312578E-16));
#49617=CARTESIAN_POINT('Ctrl Pts',(4.54111387023209,-1.5712078072459,-5.40663220727154E-16));
#49618=CARTESIAN_POINT('Ctrl Pts',(4.55495165294679,-1.52135171714656,-2.34210881400015E-17));
#49619=CARTESIAN_POINT('Ctrl Pts',(4.56796247846719,-1.47127487515823,-2.77555756156289E-17));
#49620=CARTESIAN_POINT('Ctrl Pts',(4.60395075905375,-1.33276103239401,-1.11900177134892E-17));
#49621=CARTESIAN_POINT('Ctrl Pts',(4.63361579821919,-1.19255796729143,2.91143634808383E-16));
#49622=CARTESIAN_POINT('Ctrl Pts',(4.65692008513065,-1.05110298842804,2.77555756156289E-16));
#49623=CARTESIAN_POINT('Ctrl Pts',(4.67001847025983,-0.971596938805809,
2.69918566125548E-16));
#49624=CARTESIAN_POINT('Ctrl Pts',(4.68110649292123,-0.891695424459561,
-5.05694400348962E-17));
#49625=CARTESIAN_POINT('Ctrl Pts',(4.69017032387523,-0.811477248591749,
-5.55111512312578E-17));
#49626=CARTESIAN_POINT('Ctrl Pts',(4.69376322527145,-0.779678774244579,
-5.74700448985431E-17));
#49627=CARTESIAN_POINT('Ctrl Pts',(4.69703800287417,-0.74783055663592,9.2602246089847E-18));
#49628=CARTESIAN_POINT('Ctrl Pts',(4.69999357182281,-0.715937571621207,
0.));
#49629=CARTESIAN_POINT('Ctrl Pts',(4.7021844555123,-0.692296160477742,-6.86435519161465E-18));
#49630=CARTESIAN_POINT('Ctrl Pts',(4.70420012738525,-0.668626688781088,
-5.81512878434173E-17));
#49631=CARTESIAN_POINT('Ctrl Pts',(4.70603832259692,-0.644957088113592,
-5.55111512312578E-17));
#49632=CARTESIAN_POINT('Ctrl Pts',(4.7169850543804,-0.50400101974599,-3.97887365597508E-17));
#49633=CARTESIAN_POINT('Ctrl Pts',(4.72166050160268,-0.362862391559157,
3.85433575684503E-16));
#49634=CARTESIAN_POINT('Ctrl Pts',(4.72009704228143,-0.221963242879035,
3.88578058618805E-16));
#49635=CARTESIAN_POINT('Ctrl Pts',(4.71853510529174,-0.0812012869083159,
3.91719479787741E-16));
#49636=CARTESIAN_POINT('Ctrl Pts',(4.71074633224057,0.0593224521016401,
3.13145818824179E-16));
#49637=CARTESIAN_POINT('Ctrl Pts',(4.69671116060458,0.199185274316974,2.22044604925031E-16));
#49638=CARTESIAN_POINT('Ctrl Pts',(4.68289306772495,0.336884870581422,1.3235243244906E-16));
#49639=CARTESIAN_POINT('Ctrl Pts',(4.6630201315191,0.473944543714825,-1.38004669694731E-16));
#49640=CARTESIAN_POINT('Ctrl Pts',(4.63702542177262,0.609947964574148,-1.38777878078145E-16));
#49641=CARTESIAN_POINT('Ctrl Pts',(4.62055356019607,0.696128173708246,-1.39267830902609E-16));
#49642=CARTESIAN_POINT('Ctrl Pts',(4.60162268181677,0.781883974967431,8.79945197126988E-17));
#49643=CARTESIAN_POINT('Ctrl Pts',(4.58020591978812,0.867104757427645,1.11022302462516E-16));
#49644=CARTESIAN_POINT('Ctrl Pts',(4.56733705680351,0.918312058113609,6.78760316859931E-17));
#49645=CARTESIAN_POINT('Ctrl Pts',(4.55357049340461,0.96932610659445,-4.99175148350681E-16));
#49646=CARTESIAN_POINT('Ctrl Pts',(4.53891402393445,1.0201248132638,-5.55111512312578E-16));
#49647=CARTESIAN_POINT('Ctrl Pts',(4.5307224586103,1.04851643410481,-5.86374592437204E-16));
#49648=CARTESIAN_POINT('Ctrl Pts',(4.52225289509851,1.0768407763045,9.91752405205522E-17));
#49649=CARTESIAN_POINT('Ctrl Pts',(4.51350658698018,1.10509389044702,1.11022302462516E-16));
#49650=CARTESIAN_POINT('Ctrl Pts',(4.50742875670279,1.12472704654475,1.19254853933931E-16));
#49651=CARTESIAN_POINT('Ctrl Pts',(4.50121763562789,1.14432449467847,-5.35474147175706E-16));
#49652=CARTESIAN_POINT('Ctrl Pts',(4.49487767268156,1.16387312026907,-5.27355936696949E-16));
#49653=CARTESIAN_POINT('Ctrl Pts',(4.45189774593679,1.2963973168547,-4.72320900273343E-16));
#49654=CARTESIAN_POINT('Ctrl Pts',(4.40295499932666,1.42682794112182,5.0484926233065E-16));
#49655=CARTESIAN_POINT('Ctrl Pts',(4.34826585417728,1.55478882374,3.88578058618805E-16));
#49656=CARTESIAN_POINT('Ctrl Pts',(4.29692960608226,1.67490464560194,2.79435241634665E-16));
#49657=CARTESIAN_POINT('Ctrl Pts',(4.24052923074577,1.79284458992044,2.95867102710926E-16));
#49658=CARTESIAN_POINT('Ctrl Pts',(4.17920839057011,1.90827559700852,4.9960036108132E-16));
#49659=CARTESIAN_POINT('Ctrl Pts',(4.15338816346376,1.95687986938296,5.85385862147007E-16));
#49660=CARTESIAN_POINT('Ctrl Pts',(4.12669516016291,2.0050390084677,-2.10958088174218E-16));
#49661=CARTESIAN_POINT('Ctrl Pts',(4.09913850024111,2.05272668507128,-1.66533453693773E-16));
#49662=CARTESIAN_POINT('Ctrl Pts',(4.08221130669435,2.08201973197734,-1.3924479141655E-16));
#49663=CARTESIAN_POINT('Ctrl Pts',(4.06495515473503,2.11113968242291,3.92725569055683E-16));
#49664=CARTESIAN_POINT('Ctrl Pts',(4.04738928099658,2.14005245629164,3.33066907387547E-16));
#49665=CARTESIAN_POINT('Ctrl Pts',(3.97588097586157,2.2577524629574,9.02045342409376E-17));
#49666=CARTESIAN_POINT('Ctrl Pts',(3.89920169633387,2.37209762967783,1.73844745989399E-16));
#49667=CARTESIAN_POINT('Ctrl Pts',(3.81753428055142,2.4827050770719,1.11022302462516E-16));
#49668=CARTESIAN_POINT('Ctrl Pts',(3.73700167373633,2.59177557950503,4.90728077314622E-17));
#49669=CARTESIAN_POINT('Ctrl Pts',(3.65161810526706,2.69721206501942,-2.17511715066662E-16));
#49670=CARTESIAN_POINT('Ctrl Pts',(3.56152350731999,2.79861134980753,-2.22044604925031E-16));
#49671=CARTESIAN_POINT('Ctrl Pts',(3.54164701408898,2.82098186084422,-2.23044642181868E-16));
#49672=CARTESIAN_POINT('Ctrl Pts',(3.52154110171521,2.8431557130462,3.77586732270394E-16));
#49673=CARTESIAN_POINT('Ctrl Pts',(3.50120707213069,2.86512829543052,4.44089209850063E-16));
#49674=CARTESIAN_POINT('Ctrl Pts',(3.47910313325541,2.88901340959032,5.16017817963063E-16));
#49675=CARTESIAN_POINT('Ctrl Pts',(3.45672963690434,2.91266069254474,2.77193395410128E-16));
#49676=CARTESIAN_POINT('Ctrl Pts',(3.43409108914483,2.93606647242265,2.77555756156289E-16));
#49677=CARTESIAN_POINT('Origin',(0.,0.,20.5));
#49678=CARTESIAN_POINT('Origin',(0.,0.,41.));
#49679=CARTESIAN_POINT('',(-4.,4.89858719658941E-16,41.));
#49680=CARTESIAN_POINT('Origin',(0.,0.,41.));
#49681=CARTESIAN_POINT('Origin',(-4.45462538595717E-16,-1.65775395963113E-16,
375.));
#49682=CARTESIAN_POINT('Ctrl Pts',(-3.43378788736335,2.93584158412826,375.));
#49683=CARTESIAN_POINT('Ctrl Pts',(-3.52812472271588,2.83822707478694,375.));
#49684=CARTESIAN_POINT('Ctrl Pts',(-3.61783741229297,2.73641228828402,375.));
#49685=CARTESIAN_POINT('Ctrl Pts',(-3.70278930559469,2.6308098016192,375.));
#49686=CARTESIAN_POINT('Ctrl Pts',(-3.78883118430305,2.52385236964479,375.));
#49687=CARTESIAN_POINT('Ctrl Pts',(-3.86998980756465,2.41300886934011,375.));
#49688=CARTESIAN_POINT('Ctrl Pts',(-3.94608965952372,2.29866645157891,375.));
#49689=CARTESIAN_POINT('Ctrl Pts',(-3.98412572654406,2.24151606621978,375.));
#49690=CARTESIAN_POINT('Ctrl Pts',(-4.02089745503991,2.18349099620346,375.));
#49691=CARTESIAN_POINT('Ctrl Pts',(-4.0563792513302,2.12463643972661,375.));
#49692=CARTESIAN_POINT('Ctrl Pts',(-4.0706431485814,2.10097655116059,375.));
#49693=CARTESIAN_POINT('Ctrl Pts',(-4.08469915763129,2.07718134398868,375.));
#49694=CARTESIAN_POINT('Ctrl Pts',(-4.09853534340515,2.05327180953563,375.));
#49695=CARTESIAN_POINT('Ctrl Pts',(-4.16827482663706,1.93275893089092,375.));
#49696=CARTESIAN_POINT('Ctrl Pts',(-4.23249571495574,1.80924176863962,375.));
#49697=CARTESIAN_POINT('Ctrl Pts',(-4.29102780012401,1.68312480250504,375.));
#49698=CARTESIAN_POINT('Ctrl Pts',(-4.34427585815273,1.56839313846413,375.));
#49699=CARTESIAN_POINT('Ctrl Pts',(-4.3928156984662,1.45150902581472,375.));
#49700=CARTESIAN_POINT('Ctrl Pts',(-4.4364893782082,1.33275463175064,375.));
#49701=CARTESIAN_POINT('Ctrl Pts',(-4.46204208504677,1.2632735109649,375.));
#49702=CARTESIAN_POINT('Ctrl Pts',(-4.48592844490179,1.19315178813539,375.));
#49703=CARTESIAN_POINT('Ctrl Pts',(-4.50811171504532,1.12244350259313,375.));
#49704=CARTESIAN_POINT('Ctrl Pts',(-4.5141904988611,1.10306762252609,375.));
#49705=CARTESIAN_POINT('Ctrl Pts',(-4.52013855791141,1.08365664730297,375.));
#49706=CARTESIAN_POINT('Ctrl Pts',(-4.52595509671778,1.06421299497352,375.));
#49707=CARTESIAN_POINT('Ctrl Pts',(-4.53519138586709,1.0333377268782,375.));
#49708=CARTESIAN_POINT('Ctrl Pts',(-4.54409635013865,1.00237910104441,375.));
#49709=CARTESIAN_POINT('Ctrl Pts',(-4.55266817723945,0.971342071123453,
375.));
#49710=CARTESIAN_POINT('Ctrl Pts',(-4.58939773349738,0.838351015289689,
375.));
#49711=CARTESIAN_POINT('Ctrl Pts',(-4.62001434120323,0.703922655316075,
375.));
#49712=CARTESIAN_POINT('Ctrl Pts',(-4.6446125449424,0.568489655194437,375.));
#49713=CARTESIAN_POINT('Ctrl Pts',(-4.6695978975114,0.43092508774079,375.));
#49714=CARTESIAN_POINT('Ctrl Pts',(-4.68837408722962,0.292323323451818,
375.));
#49715=CARTESIAN_POINT('Ctrl Pts',(-4.7009917947161,0.153114389433896,375.));
#49716=CARTESIAN_POINT('Ctrl Pts',(-4.71369611133585,0.0129499121739395,
375.));
#49717=CARTESIAN_POINT('Ctrl Pts',(-4.72015723771216,-0.127830868720726,
375.));
#49718=CARTESIAN_POINT('Ctrl Pts',(-4.72037601386282,-0.2688014592115,375.));
#49719=CARTESIAN_POINT('Ctrl Pts',(-4.72051776383518,-0.360139464952745,
375.));
#49720=CARTESIAN_POINT('Ctrl Pts',(-4.71803791594725,-0.451557379168488,
375.));
#49721=CARTESIAN_POINT('Ctrl Pts',(-4.7129250253839,-0.542939603201634,
375.));
#49722=CARTESIAN_POINT('Ctrl Pts',(-4.71050429468246,-0.586205100974703,
375.));
#49723=CARTESIAN_POINT('Ctrl Pts',(-4.70749320436126,-0.629462591214061,
375.));
#49724=CARTESIAN_POINT('Ctrl Pts',(-4.70388981020381,-0.672699721412066,
375.));
#49725=CARTESIAN_POINT('Ctrl Pts',(-4.70250698353675,-0.689292260011098,
375.));
#49726=CARTESIAN_POINT('Ctrl Pts',(-4.7010370790231,-0.705879562100339,
375.));
#49727=CARTESIAN_POINT('Ctrl Pts',(-4.69948096449077,-0.722452069367425,
375.));
#49728=CARTESIAN_POINT('Ctrl Pts',(-4.68606574819498,-0.865323153038659,
375.));
#49729=CARTESIAN_POINT('Ctrl Pts',(-4.66623214709618,-1.0072815713457,375.));
#49730=CARTESIAN_POINT('Ctrl Pts',(-4.64004375541204,-1.14788248706686,
375.));
#49731=CARTESIAN_POINT('Ctrl Pts',(-4.6270279916287,-1.21776185685865,375.));
#49732=CARTESIAN_POINT('Ctrl Pts',(-4.61244171628795,-1.28730612660771,
375.));
#49733=CARTESIAN_POINT('Ctrl Pts',(-4.59628803251995,-1.35646150527604,
375.));
#49734=CARTESIAN_POINT('Ctrl Pts',(-4.56399682193468,-1.4947030932479,375.));
#49735=CARTESIAN_POINT('Ctrl Pts',(-4.52544561415923,-1.63139110841489,
375.));
#49736=CARTESIAN_POINT('Ctrl Pts',(-4.48088607305284,-1.76617553752727,
375.));
#49737=CARTESIAN_POINT('Ctrl Pts',(-4.43597574851398,-1.90202102210641,
375.));
#49738=CARTESIAN_POINT('Ctrl Pts',(-4.38496188398045,-2.03593355195248,
375.));
#49739=CARTESIAN_POINT('Ctrl Pts',(-4.32805045687434,-2.16754392308446,
375.));
#49740=CARTESIAN_POINT('Ctrl Pts',(-4.30216783694698,-2.22739870775111,
375.));
#49741=CARTESIAN_POINT('Ctrl Pts',(-4.27506473176287,-2.28677711825493,
375.));
#49742=CARTESIAN_POINT('Ctrl Pts',(-4.24675722722924,-2.34564306219817,
375.));
#49743=CARTESIAN_POINT('Ctrl Pts',(-4.22863084786129,-2.38333718074896,
375.));
#49744=CARTESIAN_POINT('Ctrl Pts',(-4.21001058428347,-2.42082115169986,
375.));
#49745=CARTESIAN_POINT('Ctrl Pts',(-4.190900240747,-2.45808525714998,375.));
#49746=CARTESIAN_POINT('Ctrl Pts',(-4.18310501328873,-2.47328551649951,
375.));
#49747=CARTESIAN_POINT('Ctrl Pts',(-4.17522954608524,-2.48844657780472,
375.));
#49748=CARTESIAN_POINT('Ctrl Pts',(-4.16727814768109,-2.50356042854303,
375.));
#49749=CARTESIAN_POINT('Ctrl Pts',(-4.09969026676857,-2.63203005010014,
375.));
#49750=CARTESIAN_POINT('Ctrl Pts',(-4.02654009074559,-2.75724655837471,
375.));
#49751=CARTESIAN_POINT('Ctrl Pts',(-3.94810710693448,-2.87885707775794,
375.));
#49752=CARTESIAN_POINT('Ctrl Pts',(-3.86905485941559,-3.00142776692534,
375.));
#49753=CARTESIAN_POINT('Ctrl Pts',(-3.78463578072622,-3.12033603731368,
375.));
#49754=CARTESIAN_POINT('Ctrl Pts',(-3.69508499761951,-3.23520722691392,
375.));
#49755=CARTESIAN_POINT('Ctrl Pts',(-3.62943480927899,-3.31941994924341,
375.));
#49756=CARTESIAN_POINT('Ctrl Pts',(-3.56102553573526,-3.40146273807253,
375.));
#49757=CARTESIAN_POINT('Ctrl Pts',(-3.48993392179959,-3.48117995730746,
375.));
#49758=CARTESIAN_POINT('Ctrl Pts',(-3.39320786765338,-3.58964186493951,
375.));
#49759=CARTESIAN_POINT('Ctrl Pts',(-3.29151757709749,-3.69380035593463,
375.));
#49760=CARTESIAN_POINT('Ctrl Pts',(-3.18521993250538,-3.79343311373674,
375.));
#49761=CARTESIAN_POINT('Ctrl Pts',(-3.1484894856507,-3.82786055311678,375.));
#49762=CARTESIAN_POINT('Ctrl Pts',(-3.1112085895158,-3.86174730075506,375.));
#49763=CARTESIAN_POINT('Ctrl Pts',(-3.07339099123149,-3.89508311993719,
375.));
#49764=CARTESIAN_POINT('Ctrl Pts',(-3.05466088259105,-3.91159351571128,
375.));
#49765=CARTESIAN_POINT('Ctrl Pts',(-3.03579911530405,-3.92796876126283,
375.));
#49766=CARTESIAN_POINT('Ctrl Pts',(-3.01680731961894,-3.94420755857869,
375.));
#49767=CARTESIAN_POINT('Ctrl Pts',(-3.00397674416022,-3.95517824917451,
375.));
#49768=CARTESIAN_POINT('Ctrl Pts',(-2.99108750647465,-3.96608603020355,
375.));
#49769=CARTESIAN_POINT('Ctrl Pts',(-2.97814807270005,-3.97692398964623,
375.));
#49770=CARTESIAN_POINT('Ctrl Pts',(-2.86441519405387,-4.07218567941864,
375.));
#49771=CARTESIAN_POINT('Ctrl Pts',(-2.74664729621727,-4.16219378118691,
375.));
#49772=CARTESIAN_POINT('Ctrl Pts',(-2.62528201158405,-4.24677543677276,
375.));
#49773=CARTESIAN_POINT('Ctrl Pts',(-2.50379141827822,-4.33144442223239,
375.));
#49774=CARTESIAN_POINT('Ctrl Pts',(-2.3786953776454,-4.41067622052404,375.));
#49775=CARTESIAN_POINT('Ctrl Pts',(-2.25039003171722,-4.4842647871821,375.));
#49776=CARTESIAN_POINT('Ctrl Pts',(-2.12228319217728,-4.5577395019934,375.));
#49777=CARTESIAN_POINT('Ctrl Pts',(-1.9909763337868,-4.62558889864692,375.));
#49778=CARTESIAN_POINT('Ctrl Pts',(-1.85683056691249,-4.68756837108862,
375.));
#49779=CARTESIAN_POINT('Ctrl Pts',(-1.72268480003817,-4.74954784353032,
375.));
#49780=CARTESIAN_POINT('Ctrl Pts',(-1.58569949586696,-4.80565788540407,
375.));
#49781=CARTESIAN_POINT('Ctrl Pts',(-1.44621200484621,-4.85560714827263,
375.));
#49782=CARTESIAN_POINT('Ctrl Pts',(-1.40211572701684,-4.87139764358304,
375.));
#49783=CARTESIAN_POINT('Ctrl Pts',(-1.35776924324391,-4.88657205481219,
375.));
#49784=CARTESIAN_POINT('Ctrl Pts',(-1.31318542874385,-4.90112866933901,
375.));
#49785=CARTESIAN_POINT('Ctrl Pts',(1.31303618635831,-4.90075024188273,375.));
#49786=CARTESIAN_POINT('Ctrl Pts',(1.45436548505342,-4.85453285551617,375.));
#49787=CARTESIAN_POINT('Ctrl Pts',(1.5934293761686,-4.80203848222433,375.));
#49788=CARTESIAN_POINT('Ctrl Pts',(1.72987023226972,-4.74352674861442,375.));
#49789=CARTESIAN_POINT('Ctrl Pts',(1.86675271207831,-4.68482562767973,375.));
#49790=CARTESIAN_POINT('Ctrl Pts',(2.00099581082903,-4.620067688427,375.));
#49791=CARTESIAN_POINT('Ctrl Pts',(2.13221219437754,-4.54946990611926,375.));
#49792=CARTESIAN_POINT('Ctrl Pts',(2.19270449791029,-4.5169234941499,375.));
#49793=CARTESIAN_POINT('Ctrl Pts',(2.25255310159603,-4.48313534130926,375.));
#49794=CARTESIAN_POINT('Ctrl Pts',(2.31171758991926,-4.44812388272337,375.));
#49795=CARTESIAN_POINT('Ctrl Pts',(2.3344624112488,-4.43466429923687,375.));
#49796=CARTESIAN_POINT('Ctrl Pts',(2.35710754237018,-4.42102302699321,375.));
#49797=CARTESIAN_POINT('Ctrl Pts',(2.37964612843956,-4.40720380568676,375.));
#49798=CARTESIAN_POINT('Ctrl Pts',(2.50549113115601,-4.33004368847728,375.));
#49799=CARTESIAN_POINT('Ctrl Pts',(2.62778788875034,-4.24748071485227,375.));
#49800=CARTESIAN_POINT('Ctrl Pts',(2.74616817727066,-4.15974114711123,375.));
#49801=CARTESIAN_POINT('Ctrl Pts',(2.86286389724632,-4.07325012604791,375.));
#49802=CARTESIAN_POINT('Ctrl Pts',(2.97575433427861,-3.98172826743118,375.));
#49803=CARTESIAN_POINT('Ctrl Pts',(3.08445220151971,-3.8853563473526,375.));
#49804=CARTESIAN_POINT('Ctrl Pts',(3.13995990370008,-3.83614301894012,375.));
#49805=CARTESIAN_POINT('Ctrl Pts',(3.19437368596074,-3.78566438686541,375.));
#49806=CARTESIAN_POINT('Ctrl Pts',(3.24763776430821,-3.73394147802337,375.));
#49807=CARTESIAN_POINT('Ctrl Pts',(3.2699643084639,-3.71226094127233,375.));
#49808=CARTESIAN_POINT('Ctrl Pts',(3.29209335275734,-3.69035703897681,375.));
#49809=CARTESIAN_POINT('Ctrl Pts',(3.31399620763943,-3.66825627851417,375.));
#49810=CARTESIAN_POINT('Ctrl Pts',(3.34216498231236,-3.63983298187436,375.));
#49811=CARTESIAN_POINT('Ctrl Pts',(3.36996576521876,-3.6110784436862,375.));
#49812=CARTESIAN_POINT('Ctrl Pts',(3.39739154337912,-3.58199736557932,375.));
#49813=CARTESIAN_POINT('Ctrl Pts',(3.49658091940006,-3.47682135290355,375.));
#49814=CARTESIAN_POINT('Ctrl Pts',(3.59086820857194,-3.3673769231021,375.));
#49815=CARTESIAN_POINT('Ctrl Pts',(3.6800850008747,-3.25406730243395,375.));
#49816=CARTESIAN_POINT('Ctrl Pts',(3.76996985501536,-3.13990921107455,375.));
#49817=CARTESIAN_POINT('Ctrl Pts',(3.85470838531078,-3.02182713075438,375.));
#49818=CARTESIAN_POINT('Ctrl Pts',(3.93408537345353,-2.90020291820586,375.));
#49819=CARTESIAN_POINT('Ctrl Pts',(4.01274556585136,-2.77967700530409,375.));
#49820=CARTESIAN_POINT('Ctrl Pts',(4.08614088023802,-2.65567191437214,375.));
#49821=CARTESIAN_POINT('Ctrl Pts',(4.15401504305787,-2.52854018053819,375.));
#49822=CARTESIAN_POINT('Ctrl Pts',(4.19807507197777,-2.44601352184147,375.));
#49823=CARTESIAN_POINT('Ctrl Pts',(4.23980760353704,-2.36216897889331,375.));
#49824=CARTESIAN_POINT('Ctrl Pts',(4.27913099033935,-2.27710078886137,375.));
#49825=CARTESIAN_POINT('Ctrl Pts',(4.29645860907187,-2.23961599207746,375.));
#49826=CARTESIAN_POINT('Ctrl Pts',(4.31331832747089,-2.20189359019125,375.));
#49827=CARTESIAN_POINT('Ctrl Pts',(4.32970256286081,-2.16394161183312,375.));
#49828=CARTESIAN_POINT('Ctrl Pts',(4.33919451441291,-2.14195472435813,375.));
#49829=CARTESIAN_POINT('Ctrl Pts',(4.34852813367479,-2.11988754210219,375.));
#49830=CARTESIAN_POINT('Ctrl Pts',(4.35769217797944,-2.0977656675703,375.));
#49831=CARTESIAN_POINT('Ctrl Pts',(4.41245445040556,-1.96557030933995,375.));
#49832=CARTESIAN_POINT('Ctrl Pts',(4.46123822222855,-1.83125898605536,375.));
#49833=CARTESIAN_POINT('Ctrl Pts',(4.50384926204605,-1.6951979775962,375.));
#49834=CARTESIAN_POINT('Ctrl Pts',(4.52559692351824,-1.62575567428212,375.));
#49835=CARTESIAN_POINT('Ctrl Pts',(4.54573592530189,-1.55585726815914,375.));
#49836=CARTESIAN_POINT('Ctrl Pts',(4.56423545664257,-1.48554983900212,375.));
#49837=CARTESIAN_POINT('Ctrl Pts',(4.60056463169787,-1.34748088717324,375.));
#49838=CARTESIAN_POINT('Ctrl Pts',(4.63057447100037,-1.20783464517222,375.));
#49839=CARTESIAN_POINT('Ctrl Pts',(4.65426082259252,-1.06704756524395,375.));
#49840=CARTESIAN_POINT('Ctrl Pts',(4.67788678995459,-0.926619397467839,
375.));
#49841=CARTESIAN_POINT('Ctrl Pts',(4.69522141344644,-0.785055397710089,
375.));
#49842=CARTESIAN_POINT('Ctrl Pts',(4.7062090782541,-0.642791899249072,375.));
#49843=CARTESIAN_POINT('Ctrl Pts',(4.71102657060836,-0.58041710641334,375.));
#49844=CARTESIAN_POINT('Ctrl Pts',(4.71462329627092,-0.5179079594038,375.));
#49845=CARTESIAN_POINT('Ctrl Pts',(4.71699147233722,-0.455302034234564,
375.));
#49846=CARTESIAN_POINT('Ctrl Pts',(4.71854674616479,-0.414186275042497,
375.));
#49847=CARTESIAN_POINT('Ctrl Pts',(4.71957210036622,-0.373028786701393,
375.));
#49848=CARTESIAN_POINT('Ctrl Pts',(4.72006488912048,-0.331840385723362,
375.));
#49849=CARTESIAN_POINT('Ctrl Pts',(4.72028902811531,-0.313106340528846,
375.));
#49850=CARTESIAN_POINT('Ctrl Pts',(4.72040288834379,-0.294371677101196,
375.));
#49851=CARTESIAN_POINT('Ctrl Pts',(4.72040648677608,-0.275644826658347,
375.));
#49852=CARTESIAN_POINT('Ctrl Pts',(4.72043355701338,-0.134766732053278,
375.));
#49853=CARTESIAN_POINT('Ctrl Pts',(4.71422662120245,0.0057990813089247,
375.));
#49854=CARTESIAN_POINT('Ctrl Pts',(4.70180390274057,0.145635587850549,375.));
#49855=CARTESIAN_POINT('Ctrl Pts',(4.68946458626375,0.284533278764535,375.));
#49856=CARTESIAN_POINT('Ctrl Pts',(4.67099254981089,0.422712188593173,375.));
#49857=CARTESIAN_POINT('Ctrl Pts',(4.6463550982981,0.559757549565289,375.));
#49858=CARTESIAN_POINT('Ctrl Pts',(4.62907635772754,0.655870219230258,375.));
#49859=CARTESIAN_POINT('Ctrl Pts',(4.60876410990094,0.751425238603689,375.));
#49860=CARTESIAN_POINT('Ctrl Pts',(4.58539251247819,0.846274706840598,375.));
#49861=CARTESIAN_POINT('Ctrl Pts',(4.55189132819966,0.982233300369681,375.));
#49862=CARTESIAN_POINT('Ctrl Pts',(4.51210568697928,1.11674373042915,375.));
#49863=CARTESIAN_POINT('Ctrl Pts',(4.46619637471526,1.24939846486887,375.));
#49864=CARTESIAN_POINT('Ctrl Pts',(4.4514821415469,1.29191517002461,375.));
#49865=CARTESIAN_POINT('Ctrl Pts',(4.43613853638538,1.33424101402745,375.));
#49866=CARTESIAN_POINT('Ctrl Pts',(4.42016997732094,1.37636185265469,375.));
#49867=CARTESIAN_POINT('Ctrl Pts',(4.41229563070378,1.39713229799154,375.));
#49868=CARTESIAN_POINT('Ctrl Pts',(4.40426931219602,1.41785288761014,375.));
#49869=CARTESIAN_POINT('Ctrl Pts',(4.39609151624634,1.43852188916379,375.));
#49870=CARTESIAN_POINT('Ctrl Pts',(4.38944561986513,1.45531908531226,375.));
#49871=CARTESIAN_POINT('Ctrl Pts',(4.38270019096179,1.4720807922257,375.));
#49872=CARTESIAN_POINT('Ctrl Pts',(4.37586028060643,1.48879486186589,375.));
#49873=CARTESIAN_POINT('Ctrl Pts',(4.32342038722716,1.61693748133431,375.));
#49874=CARTESIAN_POINT('Ctrl Pts',(4.26535943234438,1.74246391819237,375.));
#49875=CARTESIAN_POINT('Ctrl Pts',(4.20190818178381,1.86501937630542,375.));
#49876=CARTESIAN_POINT('Ctrl Pts',(4.13850743678452,1.98747728343019,375.));
#49877=CARTESIAN_POINT('Ctrl Pts',(4.06972452623307,2.10696961603591,375.));
#49878=CARTESIAN_POINT('Ctrl Pts',(3.99574428312086,2.22311713285455,375.));
#49879=CARTESIAN_POINT('Ctrl Pts',(3.9230204444275,2.3372921196134,375.));
#49880=CARTESIAN_POINT('Ctrl Pts',(3.84527380385539,2.44823547455532,375.));
#49881=CARTESIAN_POINT('Ctrl Pts',(3.7626432675861,2.55555363817714,375.));
#49882=CARTESIAN_POINT('Ctrl Pts',(3.68595020843944,2.65516037730487,375.));
#49883=CARTESIAN_POINT('Ctrl Pts',(3.60504931330013,2.75164424921775,375.));
#49884=CARTESIAN_POINT('Ctrl Pts',(3.52002795172102,2.84465807652531,375.));
#49885=CARTESIAN_POINT('Ctrl Pts',(3.49183173897392,2.87550488507407,375.));
#49886=CARTESIAN_POINT('Ctrl Pts',(3.46318217104164,2.90596975880766,375.));
#49887=CARTESIAN_POINT('Ctrl Pts',(3.43408816985932,2.93604417002309,375.));
#49888=CARTESIAN_POINT('Origin',(0.,0.,402.208336844637));
#49889=CARTESIAN_POINT('Ctrl Pts',(-5.07353386009457,0.000128968315485402,
399.708336844637));
#49890=CARTESIAN_POINT('Ctrl Pts',(-5.07374798994712,0.217328374468673,
399.701523610908));
#49891=CARTESIAN_POINT('Ctrl Pts',(-5.00706367321595,1.27523772951867,399.668334418693));
#49892=CARTESIAN_POINT('Ctrl Pts',(-4.28603436807985,3.09622957226831,399.608769267991));
#49893=CARTESIAN_POINT('Ctrl Pts',(-2.29040909926245,4.7655795591539,399.529641392531));
#49894=CARTESIAN_POINT('Ctrl Pts',(0.259800278618912,5.28102545063066,399.450513517072));
#49895=CARTESIAN_POINT('Ctrl Pts',(2.7471033957984,4.51775909222651,399.371385641611));
#49896=CARTESIAN_POINT('Ctrl Pts',(4.56924148852249,2.66059337678593,399.292257766152));
#49897=CARTESIAN_POINT('Ctrl Pts',(5.2850143906551,0.159209483399153,399.213129890692));
#49898=CARTESIAN_POINT('Ctrl Pts',(4.7211096918349,-2.38072426286758,399.134002015232));
#49899=CARTESIAN_POINT('Ctrl Pts',(3.01406746059458,-4.34420558161996,399.054874139772));
#49900=CARTESIAN_POINT('Ctrl Pts',(0.577219342712345,-5.25581036421826,
398.975746264313));
#49901=CARTESIAN_POINT('Ctrl Pts',(-1.99939275815206,-4.89480881878609,
398.896618388853));
#49902=CARTESIAN_POINT('Ctrl Pts',(-4.09188543486623,-3.34861140683646,
398.817490513394));
#49903=CARTESIAN_POINT('Ctrl Pts',(-4.96571105424643,-1.479143747598,398.754729998654));
#49904=CARTESIAN_POINT('Ctrl Pts',(-5.07346848196321,-0.319197162169717,
398.718345442402));
#49905=CARTESIAN_POINT('Ctrl Pts',(-5.07327504304777,-8.56681209025073E-5,
398.708336844637));
#49906=CARTESIAN_POINT('Ctrl Pts',(-5.07330191118131,0.000105688062508012,
399.791663155363));
#49907=CARTESIAN_POINT('Ctrl Pts',(-5.07350034043644,0.308800908665525,
399.781980894782));
#49908=CARTESIAN_POINT('Ctrl Pts',(-4.97021252404761,1.45829359598981,399.745922675715));
#49909=CARTESIAN_POINT('Ctrl Pts',(-4.11241943286933,3.32339561801255,399.683488498161));
#49910=CARTESIAN_POINT('Ctrl Pts',(-2.02945797892606,4.8824090247121,399.604360622701));
#49911=CARTESIAN_POINT('Ctrl Pts',(0.54487554882432,5.2592655238007,399.525232747241));
#49912=CARTESIAN_POINT('Ctrl Pts',(2.98728943775363,4.36266186092565,399.446104871781));
#49913=CARTESIAN_POINT('Ctrl Pts',(4.70637522433117,2.40972094089285,399.366976996322));
#49914=CARTESIAN_POINT('Ctrl Pts',(5.28589404837916,-0.126697339701679,
399.287849120862));
#49915=CARTESIAN_POINT('Ctrl Pts',(4.58552092441564,-2.6324361653814,399.208721245402));
#49916=CARTESIAN_POINT('Ctrl Pts',(2.77484145336967,-4.50077558224301,399.129593369943));
#49917=CARTESIAN_POINT('Ctrl Pts',(0.292280359106768,-5.27932726882375,
399.050465494482));
#49918=CARTESIAN_POINT('Ctrl Pts',(-2.26105137922953,-4.77957858969287,
398.971337619023));
#49919=CARTESIAN_POINT('Ctrl Pts',(-4.26690751412045,-3.12253502339944,
398.892209743563));
#49920=CARTESIAN_POINT('Ctrl Pts',(-5.00313619365009,-1.29606201606178,
398.832318255676));
#49921=CARTESIAN_POINT('Ctrl Pts',(-5.07372209014652,-0.227734309753026,
398.798802726276));
#49922=CARTESIAN_POINT('Ctrl Pts',(-5.07350261625086,-0.000127405426567848,
398.791663155363));
#49923=CARTESIAN_POINT('Ctrl Pts',(3.43378788736214,2.93584158412968,400.));
#49924=CARTESIAN_POINT('Ctrl Pts',(3.92033033613488,2.36677696691239,399.973624041513));
#49925=CARTESIAN_POINT('Ctrl Pts',(4.60446627899797,0.982571495138102,399.92087212454));
#49926=CARTESIAN_POINT('Ctrl Pts',(4.51560363134058,-1.33271150407048,399.84174424908));
#49927=CARTESIAN_POINT('Ctrl Pts',(3.3333277577492,-3.32493526877752,399.762616373621));
#49928=CARTESIAN_POINT('Ctrl Pts',(1.34394627169084,-4.51226606526834,399.683488498161));
#49929=CARTESIAN_POINT('Ctrl Pts',(-0.97085300939813,-4.60694214684371,
399.604360622701));
#49930=CARTESIAN_POINT('Ctrl Pts',(-3.05057500858779,-3.58616495104857,
399.525232747241));
#49931=CARTESIAN_POINT('Ctrl Pts',(-4.391652180308,-1.69703895278099,399.446104871782));
#49932=CARTESIAN_POINT('Ctrl Pts',(-4.66936408063869,0.602987533589634,
399.366976996322));
#49933=CARTESIAN_POINT('Ctrl Pts',(-3.81646794512629,2.7570149696695,399.287849120862));
#49934=CARTESIAN_POINT('Ctrl Pts',(-2.03947802510898,4.24347545201977,399.208721245402));
#49935=CARTESIAN_POINT('Ctrl Pts',(0.231337257318392,4.70245047492642,399.129593369942));
#49936=CARTESIAN_POINT('Ctrl Pts',(2.44613812014511,4.02280553037415,399.050465494483));
#49937=CARTESIAN_POINT('Ctrl Pts',(4.06864765349505,2.36910590664905,398.971337619023));
#49938=CARTESIAN_POINT('Ctrl Pts',(4.70600239738688,0.141766919667795,398.892209743563));
#49939=CARTESIAN_POINT('Ctrl Pts',(4.20387758402063,-2.11989850176798,398.813081868103));
#49940=CARTESIAN_POINT('Ctrl Pts',(2.68385431845262,-3.86826607662479,398.733953992643));
#49941=CARTESIAN_POINT('Ctrl Pts',(0.513980740606018,-4.67999788571173,
398.654826117184));
#49942=CARTESIAN_POINT('Ctrl Pts',(-1.78034465333125,-4.35854670077871,
398.575698241724));
#49943=CARTESIAN_POINT('Ctrl Pts',(-3.64358944799884,-2.98174652775848,
398.496570366264));
#49944=CARTESIAN_POINT('Ctrl Pts',(-4.62460016500653,-0.88296644150622,
398.417442490804));
#49945=CARTESIAN_POINT('Ctrl Pts',(-4.48584151198124,1.42960916071621,398.338314615345));
#49946=CARTESIAN_POINT('Ctrl Pts',(-3.2609115695794,3.39602888062287,398.259186739885));
#49947=CARTESIAN_POINT('Ctrl Pts',(-1.24640657987359,4.54015716254393,398.180058864425));
#49948=CARTESIAN_POINT('Ctrl Pts',(1.06989485946835,4.5849625311949,398.100930988966));
#49949=CARTESIAN_POINT('Ctrl Pts',(3.12713920196537,3.51959611807719,398.021803113505));
#49950=CARTESIAN_POINT('Ctrl Pts',(4.42719923245446,1.6020185326593,397.942675238046));
#49951=CARTESIAN_POINT('Ctrl Pts',(4.65528721806493,-0.70346097272927,397.863547362586));
#49952=CARTESIAN_POINT('Ctrl Pts',(3.75617547838133,-2.83860920142977,397.784419487126));
#49953=CARTESIAN_POINT('Ctrl Pts',(1.94756884202228,-4.28643581876784,397.705291611666));
#49954=CARTESIAN_POINT('Ctrl Pts',(-0.332608926446521,-4.69637389108681,
397.626163736207));
#49955=CARTESIAN_POINT('Ctrl Pts',(-2.53225102161336,-3.96916378931016,
397.547035860747));
#49956=CARTESIAN_POINT('Ctrl Pts',(-4.11875100068,-2.28088724342758,397.467907985287));
#49957=CARTESIAN_POINT('Ctrl Pts',(-4.70796450115822,-0.0403321046706491,
397.388780109827));
#49958=CARTESIAN_POINT('Ctrl Pts',(-4.15722335570028,2.20998877681613,397.309652234368));
#49959=CARTESIAN_POINT('Ctrl Pts',(-2.59988029611171,3.92519794006916,397.230524358908));
#49960=CARTESIAN_POINT('Ctrl Pts',(-0.413019825824474,4.6899862522516,397.151396483448));
#49961=CARTESIAN_POINT('Ctrl Pts',(1.87384646846516,4.31917304995456,397.072268607988));
#49962=CARTESIAN_POINT('Ctrl Pts',(3.70699226699225,2.90254453114723,396.993140732528));
#49963=CARTESIAN_POINT('Ctrl Pts',(4.6425520586224,0.783113533157272,396.914012857069));
#49964=CARTESIAN_POINT('Ctrl Pts',(4.45399573023398,-1.52593527316547,396.834884981609));
#49965=CARTESIAN_POINT('Ctrl Pts',(3.18697903443818,-3.46550444479366,396.755757106149));
#49966=CARTESIAN_POINT('Ctrl Pts',(1.14828881478399,-4.56595983563972,396.676629230689));
#49967=CARTESIAN_POINT('Ctrl Pts',(-1.16844028323631,-4.56084462872216,
396.597501355229));
#49968=CARTESIAN_POINT('Ctrl Pts',(-3.20225116276825,-3.45139738560812,
396.51837347977));
#49969=CARTESIAN_POINT('Ctrl Pts',(-4.46069062869795,-1.50625214950199,
396.43924560431));
#49970=CARTESIAN_POINT('Ctrl Pts',(-4.63904866983842,0.803606783012363,
396.36011772885));
#49971=CARTESIAN_POINT('Ctrl Pts',(-3.69413887779848,2.91888581043708,396.28098985339));
#49972=CARTESIAN_POINT('Ctrl Pts',(-1.85475531148862,4.32740559196129,396.201861977931));
#49973=CARTESIAN_POINT('Ctrl Pts',(0.433726147102728,4.68811668499756,396.122734102471));
#49974=CARTESIAN_POINT('Ctrl Pts',(2.61718809326315,3.9136789479101,396.043606227011));
#49975=CARTESIAN_POINT('Ctrl Pts',(4.16694183591648,2.19160949051653,395.964478351551));
#49976=CARTESIAN_POINT('Ctrl Pts',(4.70774049744502,-0.0611214491752849,
395.885350476092));
#49977=CARTESIAN_POINT('Ctrl Pts',(4.10863875177974,-2.29905285502682,395.806222600631));
#49978=CARTESIAN_POINT('Ctrl Pts',(2.5146990390031,-3.98030716981366,395.727094725172));
#49979=CARTESIAN_POINT('Ctrl Pts',(0.311867128348267,-4.69779685779291,
395.647966849712));
#49980=CARTESIAN_POINT('Ctrl Pts',(-1.96647817706303,-4.27779382415375,
395.568838974252));
#49981=CARTESIAN_POINT('Ctrl Pts',(-3.7686737720159,-2.82199475955442,395.489711098792));
#49982=CARTESIAN_POINT('Ctrl Pts',(-4.65834821810063,-0.682896992050643,
395.410583223333));
#49983=CARTESIAN_POINT('Ctrl Pts',(-4.42008176906904,1.62155282910444,395.331455347873));
#49984=CARTESIAN_POINT('Ctrl Pts',(-3.11156664954973,3.53337082801154,395.252327472413));
#49985=CARTESIAN_POINT('Ctrl Pts',(-1.0496378504197,4.58964233963818,395.173199596953));
#49986=CARTESIAN_POINT('Ctrl Pts',(1.2664431505466,4.53460893234099,395.094071721494));
#49987=CARTESIAN_POINT('Ctrl Pts',(3.27587618232697,3.381596022723,395.014943846034));
#49988=CARTESIAN_POINT('Ctrl Pts',(4.49211073679585,1.40978634948583,394.935815970574));
#49989=CARTESIAN_POINT('Ctrl Pts',(4.6206560142512,-0.903379444528889,394.856688095114));
#49990=CARTESIAN_POINT('Ctrl Pts',(3.63038693161045,-2.99780705677087,394.777560219655));
#49991=CARTESIAN_POINT('Ctrl Pts',(1.7610805392752,-4.36636596691336,394.698432344195));
#49992=CARTESIAN_POINT('Ctrl Pts',(-0.534641970284508,-4.6776825871839,
394.619304468735));
#49993=CARTESIAN_POINT('Ctrl Pts',(-2.7009098933051,-3.85637681912437,394.540176593275));
#49994=CARTESIAN_POINT('Ctrl Pts',(-4.21319778305003,-2.1013140802211,394.461048717815));
#49995=CARTESIAN_POINT('Ctrl Pts',(-4.7053304898376,0.162546621736014,394.381920842356));
#49996=CARTESIAN_POINT('Ctrl Pts',(-4.05814633235487,2.38704938533492,394.302792966896));
#49997=CARTESIAN_POINT('Ctrl Pts',(-2.42835010030815,4.03356817385879,394.223665091436));
#49998=CARTESIAN_POINT('Ctrl Pts',(-0.210569617716467,4.70342607669429,
394.144537215976));
#49999=CARTESIAN_POINT('Ctrl Pts',(2.05819676630879,4.23442823696295,394.065409340517));
#50000=CARTESIAN_POINT('Ctrl Pts',(3.82860532171676,2.74013461591856,393.986281465057));
#50001=CARTESIAN_POINT('Ctrl Pts',(4.67198130861809,0.582363352861709,393.907153589597));
#50002=CARTESIAN_POINT('Ctrl Pts',(4.38411537617703,-1.71641742918247,393.828025714137));
#50003=CARTESIAN_POINT('Ctrl Pts',(3.03470943208895,-3.59959651705903,393.748897838677));
#50004=CARTESIAN_POINT('Ctrl Pts',(0.950499494613711,-4.61119367773381,
393.669769963218));
#50005=CARTESIAN_POINT('Ctrl Pts',(-1.36385795450447,-4.50626762440581,
393.590642087758));
#50006=CARTESIAN_POINT('Ctrl Pts',(-3.34798007341745,-3.31022444115695,
393.511514212298));
#50007=CARTESIAN_POINT('Ctrl Pts',(-4.52144496705717,-1.31266592578101,
393.432386336838));
#50008=CARTESIAN_POINT('Ctrl Pts',(-4.60011779179461,1.00273262859438,393.353258461379));
#50009=CARTESIAN_POINT('Ctrl Pts',(-3.56494924255402,3.07533629394358,393.274130585919));
#50010=CARTESIAN_POINT('Ctrl Pts',(-1.6665880225581,4.40329885266706,393.195002710459));
#50011=CARTESIAN_POINT('Ctrl Pts',(0.635309536488234,4.6650764426406,393.115874834999));
#50012=CARTESIAN_POINT('Ctrl Pts',(2.78337754615093,3.79728401076558,393.03674695954));
#50013=CARTESIAN_POINT('Ctrl Pts',(4.25749736347943,2.01004294053605,392.957619084079));
#50014=CARTESIAN_POINT('Ctrl Pts',(4.70073559740488,-0.263896316995348,
392.87849120862));
#50015=CARTESIAN_POINT('Ctrl Pts',(4.00576954320095,-2.47393750721331,392.79936333316));
#50016=CARTESIAN_POINT('Ctrl Pts',(2.3408735755072,-4.08495622085785,392.7202354577));
#50017=CARTESIAN_POINT('Ctrl Pts',(0.109174330666369,-4.70687129507029,
392.64110758224));
#50018=CARTESIAN_POINT('Ctrl Pts',(-2.14895964736531,-4.18909642486643,
392.561979706781));
#50019=CARTESIAN_POINT('Ctrl Pts',(-3.88675908733054,-2.65700211138166,
392.482851831321));
#50020=CARTESIAN_POINT('Ctrl Pts',(-4.68344499975174,-0.481559297629621,
392.403723955861));
#50021=CARTESIAN_POINT('Ctrl Pts',(-4.34611325228191,1.81048502373608,392.324596080401));
#50022=CARTESIAN_POINT('Ctrl Pts',(-2.95644307012664,3.66415076053556,392.245468204942));
#50023=CARTESIAN_POINT('Ctrl Pts',(-0.850919781515802,4.63060384272486,
392.166340329482));
#50024=CARTESIAN_POINT('Ctrl Pts',(1.46063946127848,4.47583386498977,392.087212454022));
#50025=CARTESIAN_POINT('Ctrl Pts',(3.41852935514023,3.23731578176699,392.008084578562));
#50026=CARTESIAN_POINT('Ctrl Pts',(4.54867969835275,1.21493597552573,391.928956703102));
#50027=CARTESIAN_POINT('Ctrl Pts',(4.57744353923776,-1.10162020130516,391.849828827643));
#50028=CARTESIAN_POINT('Ctrl Pts',(3.4978561961279,-3.1514375218371,391.770700952183));
#50029=CARTESIAN_POINT('Ctrl Pts',(1.57132163822667,-4.43818709971468,391.691573076723));
#50030=CARTESIAN_POINT('Ctrl Pts',(-0.735682101486766,-4.65030410493606,
391.612445201263));
#50031=CARTESIAN_POINT('Ctrl Pts',(-2.86455275856638,-3.73642796213481,
391.533317325804));
#50032=CARTESIAN_POINT('Ctrl Pts',(-4.29982000702773,-1.91783845252855,
391.454189450344));
#50033=CARTESIAN_POINT('Ctrl Pts',(-4.6939579537506,0.36512347398464,391.375061574884));
#50034=CARTESIAN_POINT('Ctrl Pts',(-3.95153270508603,2.55967687481616,391.295933699424));
#50035=CARTESIAN_POINT('Ctrl Pts',(-2.25231008366655,4.13444744915776,391.216805823965));
#50036=CARTESIAN_POINT('Ctrl Pts',(-0.00772834933684394,4.70813091315965,
391.137677948505));
#50037=CARTESIAN_POINT('Ctrl Pts',(2.2387246751714,4.14181943735019,391.058550073045));
#50038=CARTESIAN_POINT('Ctrl Pts',(3.94310806559349,2.572635847897,390.979422197585));
#50039=CARTESIAN_POINT('Ctrl Pts',(4.69273396842282,0.380531633959359,390.900294322126));
#50040=CARTESIAN_POINT('Ctrl Pts',(4.30609304338418,-1.90371193318514,390.821166446665));
#50041=CARTESIAN_POINT('Ctrl Pts',(2.87680390605944,-3.72700358316359,390.742038571206));
#50042=CARTESIAN_POINT('Ctrl Pts',(0.750944950216976,-4.64786382164717,
390.662910695746));
#50043=CARTESIAN_POINT('Ctrl Pts',(-1.55674273110369,-4.4433217857802,390.583782820286));
#50044=CARTESIAN_POINT('Ctrl Pts',(-3.48749126846685,-3.16290389914089,
390.504654944827));
#50045=CARTESIAN_POINT('Ctrl Pts',(-4.57380228443991,-1.11664187888751,
390.425527069367));
#50046=CARTESIAN_POINT('Ctrl Pts',(-4.55264378519931,1.19999624496042,390.346399193907));
#50047=CARTESIAN_POINT('Ctrl Pts',(-3.42913894648368,3.22607540341852,390.267271318447));
#50048=CARTESIAN_POINT('Ctrl Pts',(-1.4753256225101,4.47101450796107,390.188143442987));
#50049=CARTESIAN_POINT('Ctrl Pts',(0.835713058034306,4.63337243349421,390.109015567528));
#50050=CARTESIAN_POINT('Ctrl Pts',(2.94439783745191,3.67383693128064,390.029887692068));
#50051=CARTESIAN_POINT('Ctrl Pts',(4.34014606149365,1.8247434306593,389.950759816608));
#50052=CARTESIAN_POINT('Ctrl Pts',(4.68500070602262,-0.466181088634749,
389.871631941148));
#50053=CARTESIAN_POINT('Ctrl Pts',(3.89546100247805,-2.64422767571286,389.792504065689));
#50054=CARTESIAN_POINT('Ctrl Pts',(2.16270074857769,-4.18201887787879,389.713376190229));
#50055=CARTESIAN_POINT('Ctrl Pts',(-0.0937212205934936,-4.70720434606822,
389.634248314769));
#50056=CARTESIAN_POINT('Ctrl Pts',(-2.32745016801145,-4.09261922712786,
389.555120439309));
#50057=CARTESIAN_POINT('Ctrl Pts',(-3.99762609128131,-2.48707500030459,
389.475992563849));
#50058=CARTESIAN_POINT('Ctrl Pts',(-4.69984390136856,-0.279327273286843,
389.39686468839));
#50059=CARTESIAN_POINT('Ctrl Pts',(-4.26407333256687,1.99605486831531,389.31773681293));
#50060=CARTESIAN_POINT('Ctrl Pts',(-2.79582891973421,3.78812579970769,389.23860893747));
#50061=CARTESIAN_POINT('Ctrl Pts',(-0.650621423278113,4.6629655999594,389.159481062011));
#50062=CARTESIAN_POINT('Ctrl Pts',(1.65212313914968,4.40874648351652,389.08035318655));
#50063=CARTESIAN_POINT('Ctrl Pts',(3.55483379145156,3.08702334587661,389.001225311091));
#50064=CARTESIAN_POINT('Ctrl Pts',(4.59680105983476,1.01782927799078,388.922097435631));
#50065=CARTESIAN_POINT('Ctrl Pts',(4.52573004525854,-1.29781507938429,388.842969560171));
#50066=CARTESIAN_POINT('Ctrl Pts',(3.35882940195932,-3.29921528114894,388.763841684711));
#50067=CARTESIAN_POINT('Ctrl Pts',(1.37864455043625,-4.50176583424611,388.684713809252));
#50068=CARTESIAN_POINT('Ctrl Pts',(-0.935355957508586,-4.61428929040934,
388.605585933792));
#50069=CARTESIAN_POINT('Ctrl Pts',(-3.02287570734582,-3.60953998187742,
388.526458058332));
#50070=CARTESIAN_POINT('Ctrl Pts',(-4.37845680177713,-1.73080110290138,
388.447330182872));
#50071=CARTESIAN_POINT('Ctrl Pts',(-4.67386801345155,0.567022235602428,
388.368202307413));
#50072=CARTESIAN_POINT('Ctrl Pts',(-3.83758047185038,2.72755064937495,388.289074431953));
#50073=CARTESIAN_POINT('Ctrl Pts',(-2.07208717966135,4.22764841758585,388.209946556493));
#50074=CARTESIAN_POINT('Ctrl Pts',(0.19512727177995,4.70409202404044,388.130818681033));
#50075=CARTESIAN_POINT('Ctrl Pts',(2.41509492687017,4.04151863994701,388.051690805573));
#50076=CARTESIAN_POINT('Ctrl Pts',(4.0502878493588,2.40035929814049,387.972562930114));
#50077=CARTESIAN_POINT('Ctrl Pts',(4.7047714971451,0.17799320909573,387.893435054654));
#50078=CARTESIAN_POINT('Ctrl Pts',(4.22007363136663,-2.08747095037925,387.814307179194));
#50079=CARTESIAN_POINT('Ctrl Pts',(2.71355571127686,-3.84748902852625,387.735179303735));
#50080=CARTESIAN_POINT('Ctrl Pts',(0.549995785174607,-4.67590216526428,
387.656051428274));
#50081=CARTESIAN_POINT('Ctrl Pts',(-1.74673639624114,-4.37212401298038,
387.576923552815));
#50082=CARTESIAN_POINT('Ctrl Pts',(-3.62052565410023,-3.00970935653847,
387.497795677355));
#50083=CARTESIAN_POINT('Ctrl Pts',(-4.61766534522889,-0.918544055723703,
387.418667801895));
#50084=CARTESIAN_POINT('Ctrl Pts',(-4.49671481660818,1.39503128313651,387.339539926435));
#50085=CARTESIAN_POINT('Ctrl Pts',(-3.28696021026318,3.37082319307611,387.260412050976));
#50086=CARTESIAN_POINT('Ctrl Pts',(-1.28132331513389,4.53042679942271,387.181284175516));
#50087=CARTESIAN_POINT('Ctrl Pts',(1.03456453147854,4.59306353679543,387.102156300057));
#50088=CARTESIAN_POINT('Ctrl Pts',(3.09994992763925,3.54356696973015,387.023028424596));
#50089=CARTESIAN_POINT('Ctrl Pts',(4.414734438574,1.63605509066836,386.943900549137));
#50090=CARTESIAN_POINT('Ctrl Pts',(4.66056504541948,-0.667600090059401,
386.864772673676));
#50091=CARTESIAN_POINT('Ctrl Pts',(3.77791798959212,-2.80960710540626,386.785644798217));
#50092=CARTESIAN_POINT('Ctrl Pts',(1.9805114526468,-4.27131488054533,386.706516922757));
#50093=CARTESIAN_POINT('Ctrl Pts',(-0.29644271708526,-4.69879539225962,
386.627389047298));
#50094=CARTESIAN_POINT('Ctrl Pts',(-2.50161825456297,-3.98854140398097,
386.548261171838));
#50095=CARTESIAN_POINT('Ctrl Pts',(-4.10106888673475,-2.31252900718875,
386.469133296378));
#50096=CARTESIAN_POINT('Ctrl Pts',(-4.70751446766038,-0.0765764950965269,
386.390005420918));
#50097=CARTESIAN_POINT('Ctrl Pts',(-4.1741143707138,2.17791773100677,386.310877545459));
#50098=CARTESIAN_POINT('Ctrl Pts',(-2.63002248363295,3.90506570475047,386.231749669998));
#50099=CARTESIAN_POINT('Ctrl Pts',(-0.449114760664552,4.68666751056509,
386.152621794539));
#50100=CARTESIAN_POINT('Ctrl Pts',(1.84053856942387,4.33347137954045,386.073493919079));
#50101=CARTESIAN_POINT('Ctrl Pts',(3.68453635289055,2.93099783129588,385.994366043619));
#50102=CARTESIAN_POINT('Ctrl Pts',(4.63638545244831,0.818832314432457,385.915238168159));
#50103=CARTESIAN_POINT('Ctrl Pts',(4.46561157225142,-1.49159971460418,385.8361102927));
#50104=CARTESIAN_POINT('Ctrl Pts',(3.21356474331376,-3.44086588860477,385.75698241724));
#50105=CARTESIAN_POINT('Ctrl Pts',(1.18340710698663,-4.55698409498724,385.67785454178));
#50106=CARTESIAN_POINT('Ctrl Pts',(-1.13329271318905,-4.56970502867152,
385.59872666632));
#50107=CARTESIAN_POINT('Ctrl Pts',(-3.17558470949784,-3.47594852891073,
385.519598790861));
#50108=CARTESIAN_POINT('Ctrl Pts',(-4.44896212663648,-1.54054938855827,
385.440470915401));
#50109=CARTESIAN_POINT('Ctrl Pts',(-4.64509797905953,0.767867949435454,
385.361343039941));
#50110=CARTESIAN_POINT('Ctrl Pts',(-3.71650125952819,2.89035894150857,385.282215164481));
#50111=CARTESIAN_POINT('Ctrl Pts',(-1.88801609003413,4.31299799056357,385.203087289022));
#50112=CARTESIAN_POINT('Ctrl Pts',(0.397620511444409,4.69131691017691,385.123959413562));
#50113=CARTESIAN_POINT('Ctrl Pts',(2.58697997463334,3.93371211881083,385.044831538102));
#50114=CARTESIAN_POINT('Ctrl Pts',(4.14994562361626,2.22362491078451,384.965703662642));
#50115=CARTESIAN_POINT('Ctrl Pts',(4.70807153923669,-0.0248757766222604,
384.886575787182));
#50116=CARTESIAN_POINT('Ctrl Pts',(4.12621689144541,-2.26735321191552,384.807447911723));
#50117=CARTESIAN_POINT('Ctrl Pts',(2.54526802482854,-3.96082909308373,384.728320036263));
#50118=CARTESIAN_POINT('Ctrl Pts',(0.348025193093154,-4.69525663705463,
384.649192160803));
#50119=CARTESIAN_POINT('Ctrl Pts',(-1.93348610236405,-4.29280653125647,
384.570064285343));
#50120=CARTESIAN_POINT('Ctrl Pts',(-3.74683616493588,-2.85092531925369,
384.490936409884));
#50121=CARTESIAN_POINT('Ctrl Pts',(-4.65295268895202,-0.718740354514286,
384.411808534423));
#50122=CARTESIAN_POINT('Ctrl Pts',(-4.43243475474589,1.58747553296225,384.332680658964));
#50123=CARTESIAN_POINT('Ctrl Pts',(-3.1386770817443,3.50931084393592,384.253552783504));
#50124=CARTESIAN_POINT('Ctrl Pts',(-1.08494139264941,4.58142538925924,384.174424908044));
#50125=CARTESIAN_POINT('Ctrl Pts',(1.23149465895138,4.54422461238519,384.095297032584));
#50126=CARTESIAN_POINT('Ctrl Pts',(3.24974493247929,3.40671605753374,384.016169157125));
#50127=CARTESIAN_POINT('Ctrl Pts',(4.48112397259501,1.44432834392579,383.937041281665));
#50128=CARTESIAN_POINT('Ctrl Pts',(4.62747399638768,-0.867779255104094,
383.857913406205));
#50129=CARTESIAN_POINT('Ctrl Pts',(3.65335880005533,-2.96976866117404,383.778785530746));
#50130=CARTESIAN_POINT('Ctrl Pts',(1.79464404134943,-4.35267839240186,383.699657655285));
#50131=CARTESIAN_POINT('Ctrl Pts',(-0.498613673709388,-4.68166005036923,
383.620529779826));
#50132=CARTESIAN_POINT('Ctrl Pts',(-2.6711404500085,-3.87705624400286,383.541401904366));
#50133=CARTESIAN_POINT('Ctrl Pts',(-4.19689536445816,-2.13368829087633,
383.462274028906));
#50134=CARTESIAN_POINT('Ctrl Pts',(-4.70644245320202,0.126316497461169,
383.383146153446));
#50135=CARTESIAN_POINT('Ctrl Pts',(-4.07640343439582,2.35573586441245,383.304018277987));
#50136=CARTESIAN_POINT('Ctrl Pts',(-2.45933168995915,4.01475330021607,383.224890402527));
#50137=CARTESIAN_POINT('Ctrl Pts',(-0.246774022640667,4.70166555643666,
383.145762527067));
#50138=CARTESIAN_POINT('Ctrl Pts',(2.02553583557396,4.25014835054481,383.066634651607));
#50139=CARTESIAN_POINT('Ctrl Pts',(3.80739616178709,2.76952900148059,382.987506776148));
#50140=CARTESIAN_POINT('Ctrl Pts',(4.66735936186835,0.618314652917929,382.908378900688));
#50141=CARTESIAN_POINT('Ctrl Pts',(4.39719976949725,-1.68261421899571,382.829251025228));
#50142=CARTESIAN_POINT('Ctrl Pts',(3.06233199907708,-3.57612627716942,382.750123149768));
#50143=CARTESIAN_POINT('Ctrl Pts',(0.985971893936046,-4.60373933310752,
382.670995274309));
#50144=CARTESIAN_POINT('Ctrl Pts',(-1.32912476943063,-4.51663411957612,
382.591867398849));
#50145=CARTESIAN_POINT('Ctrl Pts',(-3.32239616084197,-3.33590170317647,
382.512739523389));
#50146=CARTESIAN_POINT('Ctrl Pts',(-4.51120504233833,-1.34743663628917,
382.433611647929));
#50147=CARTESIAN_POINT('Ctrl Pts',(-4.6077012809677,0.967287614002028,382.354483772469));
#50148=CARTESIAN_POINT('Ctrl Pts',(-3.58851993089967,3.04779939109664,382.27535589701));
#50149=CARTESIAN_POINT('Ctrl Pts',(-1.70043866320114,4.39033766076413,382.19622802155));
#50150=CARTESIAN_POINT('Ctrl Pts',(0.599375308465022,4.66982929692676,382.11710014609));
#50151=CARTESIAN_POINT('Ctrl Pts',(2.75406060140474,3.81860008728635,382.03797227063));
#50152=CARTESIAN_POINT('Ctrl Pts',(4.24189630850143,2.0427609088572,381.95884439517));
#50153=CARTESIAN_POINT('Ctrl Pts',(4.70262796601022,-0.227698564184567,
381.879716519711));
#50154=CARTESIAN_POINT('Ctrl Pts',(4.02469713006905,-2.44302464867774,381.800588644251));
#50155=CARTESIAN_POINT('Ctrl Pts',(2.37225338291554,-4.06681328684744,381.721460768791));
#50156=CARTESIAN_POINT('Ctrl Pts',(0.145408264526719,-4.70589129277765,
381.642332893331));
#50157=CARTESIAN_POINT('Ctrl Pts',(-2.11664502645219,-4.20551664541093,
381.563205017872));
#50158=CARTESIAN_POINT('Ctrl Pts',(-3.86618822286509,-2.68684667374458,
381.484077142412));
#50159=CARTESIAN_POINT('Ctrl Pts',(-4.67959878156707,-0.517601841562701,
381.404949266952));
#50160=CARTESIAN_POINT('Ctrl Pts',(-4.35992297760592,1.77697159577105,381.325821391492));
#50161=CARTESIAN_POINT('Ctrl Pts',(-2.98456494557718,3.6412811630613,381.246693516033));
#50162=CARTESIAN_POINT('Ctrl Pts',(-0.886544566588966,4.62391556522009,
381.167565640573));
#50163=CARTESIAN_POINT('Ctrl Pts',(1.4261377108192,4.48694636168212,381.088437765113));
#50164=CARTESIAN_POINT('Ctrl Pts',(3.39350465953423,3.26353834795189,381.009309889653));
#50165=CARTESIAN_POINT('Ctrl Pts',(4.53919136794792,1.2499192565843,380.930182014193));
#50166=CARTESIAN_POINT('Ctrl Pts',(4.58578901411133,-1.06634682017112,380.851054138734));
#50167=CARTESIAN_POINT('Ctrl Pts',(3.52201475950248,-3.12441489829372,380.771926263274));
#50168=CARTESIAN_POINT('Ctrl Pts',(1.60544369914822,-4.42595830885227,380.692798387814));
#50169=CARTESIAN_POINT('Ctrl Pts',(-0.699858627803908,-4.65583014337095,
380.613670512354));
#50170=CARTESIAN_POINT('Ctrl Pts',(-2.83570192547335,-3.75837079233806,
380.534542636895));
#50171=CARTESIAN_POINT('Ctrl Pts',(-4.28492755989611,-1.95088498617316,
380.455414761435));
#50172=CARTESIAN_POINT('Ctrl Pts',(-4.69662984888973,0.32897490079206,380.376286885975));
#50173=CARTESIAN_POINT('Ctrl Pts',(-3.97112198789876,2.52917903282076,380.297159010515));
#50174=CARTESIAN_POINT('Ctrl Pts',(-2.28407353785474,4.11698487931458,380.218031135056));
#50175=CARTESIAN_POINT('Ctrl Pts',(-0.0439749871787381,4.70793188388869,
380.138903259595));
#50176=CARTESIAN_POINT('Ctrl Pts',(2.20677136913111,4.15893214025144,380.059775384136));
#50177=CARTESIAN_POINT('Ctrl Pts',(3.92318504851847,2.60291672896277,379.980647508676));
#50178=CARTESIAN_POINT('Ctrl Pts',(4.68966526476571,0.416648685685039,379.901519633216));
#50179=CARTESIAN_POINT('Ctrl Pts',(4.32062168826984,-1.8705038491501,379.822391757756));
#50180=CARTESIAN_POINT('Ctrl Pts',(2.90541203179102,-3.70474524743025,379.743263882297));
#50181=CARTESIAN_POINT('Ctrl Pts',(0.786705578939987,-4.64194471691529,
379.664136006837));
#50182=CARTESIAN_POINT('Ctrl Pts',(-1.52248843588733,-4.45517512399035,
379.585008131377));
#50183=CARTESIAN_POINT('Ctrl Pts',(-3.46303740985959,-3.18965959323972,
379.505880255917));
#50184=CARTESIAN_POINT('Ctrl Pts',(-4.56506995418396,-1.15182148627296,
379.426752380458));
#50185=CARTESIAN_POINT('Ctrl Pts',(-4.56174737061485,1.16491087621397,379.347624504998));
#50186=CARTESIAN_POINT('Ctrl Pts',(-3.45387416703998,3.19957960693074,379.268496629538));
#50187=CARTESIAN_POINT('Ctrl Pts',(-1.50970325938777,4.45952379648624,379.189368754078));
#50188=CARTESIAN_POINT('Ctrl Pts',(0.800016973052387,4.63966909010343,379.110240878619));
#50189=CARTESIAN_POINT('Ctrl Pts',(2.91602651267941,3.69639632617822,379.031113003159));
#50190=CARTESIAN_POINT('Ctrl Pts',(4.32596913740423,1.85810318471799,378.951985127699));
#50191=CARTESIAN_POINT('Ctrl Pts',(4.68845088702114,-0.430098480378534,
378.872857252239));
#50192=CARTESIAN_POINT('Ctrl Pts',(3.91570288509923,-2.61415901170123,378.79372937678));
#50193=CARTESIAN_POINT('Ctrl Pts',(2.19483310042462,-4.16524478081583,378.714601501319));
#50194=CARTESIAN_POINT('Ctrl Pts',(-0.0574787096237898,-4.70778638223669,
378.63547362586));
#50195=CARTESIAN_POINT('Ctrl Pts',(-2.29587301412136,-4.11041646623094,
378.5563457504));
#50196=CARTESIAN_POINT('Ctrl Pts',(-3.97836017269986,-2.5177781393738,378.47721787494));
#50197=CARTESIAN_POINT('Ctrl Pts',(-4.69755413716848,-0.315502062123824,
378.398089999481));
#50198=CARTESIAN_POINT('Ctrl Pts',(-4.27931415074721,1.96316754813432,378.318962124021));
#50199=CARTESIAN_POINT('Ctrl Pts',(-2.82491001177881,3.76648906120608,378.239834248561));
#50200=CARTESIAN_POINT('Ctrl Pts',(-0.686501290471962,4.65781841649216,
378.160706373101));
#50201=CARTESIAN_POINT('Ctrl Pts',(1.61813220490064,4.421335159236,378.081578497641));
#50202=CARTESIAN_POINT('Ctrl Pts',(3.5309621248084,3.11429974408401,378.002450622182));
#50203=CARTESIAN_POINT('Ctrl Pts',(4.58882878451957,1.05318887631696,377.923322746722));
#50204=CARTESIAN_POINT('Ctrl Pts',(4.53558751403461,-1.26293401465255,377.844194871262));
#50205=CARTESIAN_POINT('Ctrl Pts',(3.38412979408371,-3.27325861484057,377.765066995802));
#50206=CARTESIAN_POINT('Ctrl Pts',(1.41326180027294,-4.49101853778431,377.685939120342));
#50207=CARTESIAN_POINT('Ctrl Pts',(-0.899803836436171,-4.62135364138776,
377.606811244883));
#50208=CARTESIAN_POINT('Ctrl Pts',(-2.99499706490511,-3.63270546618397,
377.527683369423));
#50209=CARTESIAN_POINT('Ctrl Pts',(-4.36500198367802,-1.76445858702323,
377.448555493963));
#50210=CARTESIAN_POINT('Ctrl Pts',(-4.67809487824384,0.531022346970404,
377.369427618503));
#50211=CARTESIAN_POINT('Ctrl Pts',(-3.858465555114,2.69792512550514,377.290299743043));
#50212=CARTESIAN_POINT('Ctrl Pts',(-2.10457350875104,4.21157058222897,377.211171867584));
#50213=CARTESIAN_POINT('Ctrl Pts',(0.158905716619817,4.70545485538416,377.132043992124));
#50214=CARTESIAN_POINT('Ctrl Pts',(2.38390858774424,4.05999215123785,377.052916116664));
#50215=CARTESIAN_POINT('Ctrl Pts',(4.03168797525527,2.43147043844132,376.973788241204));
#50216=CARTESIAN_POINT('Ctrl Pts',(4.70326173563702,0.21420893755303,376.894660365745));
#50217=CARTESIAN_POINT('Ctrl Pts',(4.23601954588194,-2.0549196650327,376.815532490285));
#50218=CARTESIAN_POINT('Ctrl Pts',(2.74309626604883,-3.82648393411214,376.736404614825));
#50219=CARTESIAN_POINT('Ctrl Pts',(0.585978230290955,-4.67152929311995,
376.657276739365));
#50220=CARTESIAN_POINT('Ctrl Pts',(-1.71302460639056,-4.38544218074737,
376.578148863906));
#50221=CARTESIAN_POINT('Ctrl Pts',(-3.59724726405772,-3.03749379327437,
376.499020988446));
#50222=CARTESIAN_POINT('Ctrl Pts',(-4.61045682670426,-0.954067226005277,
376.419893112986));
#50223=CARTESIAN_POINT('Ctrl Pts',(-4.50732159153776,1.36037071913331,376.340765237526));
#50224=CARTESIAN_POINT('Ctrl Pts',(-3.31281402583599,3.34541770982772,376.261637362067));
#50225=CARTESIAN_POINT('Ctrl Pts',(-1.31616410382415,4.52042790819332,376.182509486607));
#50226=CARTESIAN_POINT('Ctrl Pts',(0.999172883001983,4.60089230230265,376.103381611147));
#50227=CARTESIAN_POINT('Ctrl Pts',(3.07257691207793,3.5673277858007,376.024253735687));
#50228=CARTESIAN_POINT('Ctrl Pts',(4.40200797556968,1.66999467821426,375.945125860228));
#50229=CARTESIAN_POINT('Ctrl Pts',(4.66556662820138,-0.631699641477607,
375.865997984767));
#50230=CARTESIAN_POINT('Ctrl Pts',(3.79943658220811,-2.78043846928895,375.786870109308));
#50231=CARTESIAN_POINT('Ctrl Pts',(2.01333666035538,-4.25594079109181,375.707742233848));
#50232=CARTESIAN_POINT('Ctrl Pts',(-0.260258907652536,-4.70093834665202,
375.628614358388));
#50233=CARTESIAN_POINT('Ctrl Pts',(-2.47083727331916,-4.00768269259632,
375.549486482929));
#50234=CARTESIAN_POINT('Ctrl Pts',(-4.08314356267804,-2.34403352650038,
375.470358607469));
#50235=CARTESIAN_POINT('Ctrl Pts',(-4.70678568739368,-0.112816719080636,
375.391230732009));
#50236=CARTESIAN_POINT('Ctrl Pts',(-4.19075739000426,2.14571838351356,375.312102856549));
#50237=CARTESIAN_POINT('Ctrl Pts',(-2.66001002678919,3.8847003407523,375.232974981089));
#50238=CARTESIAN_POINT('Ctrl Pts',(-0.48518044668226,4.68307451075752,375.153847105629));
#50239=CARTESIAN_POINT('Ctrl Pts',(1.80711601134657,4.34750540330396,375.07471923017));
#50240=CARTESIAN_POINT('Ctrl Pts',(3.66187380043387,2.9592933100083,374.99559135471));
#50241=CARTESIAN_POINT('Ctrl Pts',(4.62991897355734,0.854469882696709,374.91646347925));
#50242=CARTESIAN_POINT('Ctrl Pts',(4.477014386818,-1.45709927207541,374.837335603791));
#50243=CARTESIAN_POINT('Ctrl Pts',(3.23983968516725,-3.41613747848395,374.758207728331));
#50244=CARTESIAN_POINT('Ctrl Pts',(1.8923805371004,-4.17007422695688,374.705455811358));
#50245=CARTESIAN_POINT('Ctrl Pts',(1.16918346556986,-4.36383719750612,374.679079852871));
#50246=CARTESIAN_POINT('Ctrl Pts',(3.57461543774233,3.05624720968358,400.106973382376));
#50247=CARTESIAN_POINT('Ctrl Pts',(4.0811121130032,2.46384394177512,400.08059742389));
#50248=CARTESIAN_POINT('Ctrl Pts',(4.79330604666853,1.02286901533234,400.027845506917));
#50249=CARTESIAN_POINT('Ctrl Pts',(4.70079893715141,-1.38736907251624,399.948717631457));
#50250=CARTESIAN_POINT('Ctrl Pts',(3.47003520682193,-3.46129852254691,399.869589755997));
#50251=CARTESIAN_POINT('Ctrl Pts',(1.39906460383401,-4.69732448980706,399.790461880537));
#50252=CARTESIAN_POINT('Ctrl Pts',(-1.01066992750072,-4.79588345555735,
399.711334005077));
#50253=CARTESIAN_POINT('Ctrl Pts',(-3.17568611614676,-3.73324183578399,
399.632206129617));
#50254=CARTESIAN_POINT('Ctrl Pts',(-4.57176395161188,-1.76663842906183,
399.553078254158));
#50255=CARTESIAN_POINT('Ctrl Pts',(-4.86086545663507,0.627717441216646,
399.473950378698));
#50256=CARTESIAN_POINT('Ctrl Pts',(-3.97299008611081,2.8700865038691,399.394822503238));
#50257=CARTESIAN_POINT('Ctrl Pts',(-2.12312171649347,4.41751015439781,399.315694627778));
#50258=CARTESIAN_POINT('Ctrl Pts',(0.240824931085231,4.89530880016116,399.236566752319));
#50259=CARTESIAN_POINT('Ctrl Pts',(2.54645987869621,4.18779005099161,399.157438876859));
#50260=CARTESIAN_POINT('Ctrl Pts',(4.23551226517086,2.46626839669468,399.078311001399));
#50261=CARTESIAN_POINT('Ctrl Pts',(4.89900639514296,0.147581107578247,398.999183125939));
#50262=CARTESIAN_POINT('Ctrl Pts',(4.37628828662539,-2.20684042213451,398.920055250479));
#50263=CARTESIAN_POINT('Ctrl Pts',(2.79392536583327,-4.02691257828985,398.84092737502));
#50264=CARTESIAN_POINT('Ctrl Pts',(0.53506027464146,-4.87193537854724,398.76179949956));
#50265=CARTESIAN_POINT('Ctrl Pts',(-1.85336068827152,-4.53730074011451,
398.6826716241));
#50266=CARTESIAN_POINT('Ctrl Pts',(-3.7930214436213,-3.10403482078447,398.60354374864));
#50267=CARTESIAN_POINT('Ctrl Pts',(-4.81426566971713,-0.919178929028494,
398.524415873181));
#50268=CARTESIAN_POINT('Ctrl Pts',(-4.6698162047254,1.48824072524753,398.445287997721));
#50269=CARTESIAN_POINT('Ctrl Pts',(-3.39464906397748,3.53530784716552,398.366160122261));
#50270=CARTESIAN_POINT('Ctrl Pts',(-1.29752458459001,4.7263594652241,398.287032246801));
#50271=CARTESIAN_POINT('Ctrl Pts',(1.1137737119676,4.77300240524464,398.207904371341));
#50272=CARTESIAN_POINT('Ctrl Pts',(3.25539038344674,3.66394286164299,398.128776495882));
#50273=CARTESIAN_POINT('Ctrl Pts',(4.60876887024317,1.66772100264832,398.049648620422));
#50274=CARTESIAN_POINT('Ctrl Pts',(4.84621126950363,-0.732311527518088,
397.970520744962));
#50275=CARTESIAN_POINT('Ctrl Pts',(3.91022488643166,-2.95502710301166,397.891392869503));
#50276=CARTESIAN_POINT('Ctrl Pts',(2.02744312611193,-4.46223242473778,397.812264994043));
#50277=CARTESIAN_POINT('Ctrl Pts',(-0.346249984625578,-4.88898300162196,
397.733137118583));
#50278=CARTESIAN_POINT('Ctrl Pts',(-2.63610446859942,-4.13194833857237,
397.654009243123));
#50279=CARTESIAN_POINT('Ctrl Pts',(-4.28767046602801,-2.3744316828985,397.574881367663));
#50280=CARTESIAN_POINT('Ctrl Pts',(-4.90104896930931,-0.0419862171810207,
397.495753492204));
#50281=CARTESIAN_POINT('Ctrl Pts',(-4.3277206609419,2.30062550686931,397.416625616744));
#50282=CARTESIAN_POINT('Ctrl Pts',(-2.70650737541695,4.08617934858649,397.337497741284));
#50283=CARTESIAN_POINT('Ctrl Pts',(-0.429958720199221,4.88233339100534,
397.258369865824));
#50284=CARTESIAN_POINT('Ctrl Pts',(1.95069722820886,4.49631228517985,397.179241990364));
#50285=CARTESIAN_POINT('Ctrl Pts',(3.85902455825875,3.0215845678645,397.100114114904));
#50286=CARTESIAN_POINT('Ctrl Pts',(4.83295381183918,0.815230822914742,397.020986239445));
#50287=CARTESIAN_POINT('Ctrl Pts',(4.63666435411759,-1.58851739343839,396.941858363985));
#50288=CARTESIAN_POINT('Ctrl Pts',(3.31768438527967,-3.60763276424756,396.862730488525));
#50289=CARTESIAN_POINT('Ctrl Pts',(1.19538278395727,-4.75322036537541,396.783602613066));
#50290=CARTESIAN_POINT('Ctrl Pts',(-1.21636071054614,-4.7478953720402,396.704474737606));
#50291=CARTESIAN_POINT('Ctrl Pts',(-3.33358285876919,-3.59294714207171,
396.625346862146));
#50292=CARTESIAN_POINT('Ctrl Pts',(-4.64363382578808,-1.5680270195369,396.546218986686));
#50293=CARTESIAN_POINT('Ctrl Pts',(-4.82930674101173,0.836564548148951,
396.467091111227));
#50294=CARTESIAN_POINT('Ctrl Pts',(-3.84564402196864,3.03859604065724,396.387963235766));
#50295=CARTESIAN_POINT('Ctrl Pts',(-1.93082309891163,4.50488246269648,396.308835360307));
#50296=CARTESIAN_POINT('Ctrl Pts',(0.451514255406424,4.88038714849199,396.229707484847));
#50297=CARTESIAN_POINT('Ctrl Pts',(2.724525005195,4.07418793602703,396.150579609387));
#50298=CARTESIAN_POINT('Ctrl Pts',(4.33783771841656,2.28149244370514,396.071451733927));
#50299=CARTESIAN_POINT('Ctrl Pts',(4.90081577868788,-0.063628180588346,
395.992323858468));
#50300=CARTESIAN_POINT('Ctrl Pts',(4.27714349050859,-2.39334230807068,395.913195983008));
#50301=CARTESIAN_POINT('Ctrl Pts',(2.61783263875445,-4.14354873477711,395.834068107548));
#50302=CARTESIAN_POINT('Ctrl Pts',(0.324657517612272,-4.89046432747023,
395.754940232088));
#50303=CARTESIAN_POINT('Ctrl Pts',(-2.04712797653699,-4.45323600201927,
395.675812356629));
#50304=CARTESIAN_POINT('Ctrl Pts',(-3.92323576387579,-2.93773126460658,
395.596684481169));
#50305=CARTESIAN_POINT('Ctrl Pts',(-4.84939780820125,-0.710904170626361,
395.517556605709));
#50306=CARTESIAN_POINT('Ctrl Pts',(-4.6013595032905,1.68805644558445,395.438428730249));
#50307=CARTESIAN_POINT('Ctrl Pts',(-3.23917916478794,3.67828250415935,395.35930085479));
#50308=CARTESIAN_POINT('Ctrl Pts',(-1.09268591631945,4.77787414341129,395.28017297933));
#50309=CARTESIAN_POINT('Ctrl Pts',(1.31838290117699,4.72058368932118,395.20104510387));
#50310=CARTESIAN_POINT('Ctrl Pts',(3.41022740996214,3.52028306451966,395.12191722841));
#50311=CARTESIAN_POINT('Ctrl Pts',(4.6763425448897,1.46760493487027,395.04278935295));
#50312=CARTESIAN_POINT('Ctrl Pts',(4.81015976025467,-0.940429116322842,
394.963661477491));
#50313=CARTESIAN_POINT('Ctrl Pts',(3.77927746162617,-3.12075402908423,394.884533602031));
#50314=CARTESIAN_POINT('Ctrl Pts',(1.83330650852657,-4.54544069236363,394.805405726571));
#50315=CARTESIAN_POINT('Ctrl Pts',(-0.556568868938532,-4.8695251242939,
394.726277851111));
#50316=CARTESIAN_POINT('Ctrl Pts',(-2.81168042909494,-4.01453571495453,
394.647149975651));
#50317=CARTESIAN_POINT('Ctrl Pts',(-4.3859907284844,-2.18749381065409,394.568022100192));
#50318=CARTESIAN_POINT('Ctrl Pts',(-4.89830693111745,0.169213033090633,
394.488894224732));
#50319=CARTESIAN_POINT('Ctrl Pts',(-4.2245802606628,2.48494777877106,394.409766349272));
#50320=CARTESIAN_POINT('Ctrl Pts',(-2.52794233119419,4.19899409527539,394.330638473813));
#50321=CARTESIAN_POINT('Ctrl Pts',(-0.219205562748669,4.89632441360466,
394.251510598353));
#50322=CARTESIAN_POINT('Ctrl Pts',(2.14260815638517,4.40809189221286,394.172382722893));
#50323=CARTESIAN_POINT('Ctrl Pts',(3.98562524447155,2.85251384792995,394.093254847433));
#50324=CARTESIAN_POINT('Ctrl Pts',(4.86359002316223,0.606247415332937,394.014126971973));
#50325=CARTESIAN_POINT('Ctrl Pts',(4.56391804578379,-1.78681166141541,393.934999096514));
#50326=CARTESIAN_POINT('Ctrl Pts',(3.15916985581216,-3.74722426125376,393.855871221054));
#50327=CARTESIAN_POINT('Ctrl Pts',(0.989481668194294,-4.80030935152189,
393.776743345594));
#50328=CARTESIAN_POINT('Ctrl Pts',(-1.41979291062284,-4.69108003906842,
393.697615470134));
#50329=CARTESIAN_POINT('Ctrl Pts',(-3.48528844770473,-3.44598437000184,
393.618487594675));
#50330=CARTESIAN_POINT('Ctrl Pts',(-4.70687983950021,-1.3665013788897,393.539359719215));
#50331=CARTESIAN_POINT('Ctrl Pts',(-4.788779217989,1.04385700330924,393.460231843755));
#50332=CARTESIAN_POINT('Ctrl Pts',(-3.71115602221747,3.2014629188482,393.381103968295));
#50333=CARTESIAN_POINT('Ctrl Pts',(-1.7349386360522,4.58388828083041,393.301976092836));
#50334=CARTESIAN_POINT('Ctrl Pts',(0.661365043902099,4.85640197272687,393.222848217375));
#50335=CARTESIAN_POINT('Ctrl Pts',(2.89753027033354,3.95301937441519,393.143720341916));
#50336=CARTESIAN_POINT('Ctrl Pts',(4.43210713674341,2.09247943130372,393.064592466456));
#50337=CARTESIAN_POINT('Ctrl Pts',(4.89352359156256,-0.27471931279354,392.985464590996));
#50338=CARTESIAN_POINT('Ctrl Pts',(4.17005537874506,-2.57539938265902,392.906336715536));
#50339=CARTESIAN_POINT('Ctrl Pts',(2.43687819262455,-4.2524896844451,392.827208840076));
#50340=CARTESIAN_POINT('Ctrl Pts',(0.113651821430644,-4.89991092832171,
392.748080964617));
#50341=CARTESIAN_POINT('Ctrl Pts',(-2.23709343224997,-4.3609009180885,392.668953089157));
#50342=CARTESIAN_POINT('Ctrl Pts',(-4.04616402995999,-2.76597188790106,
392.589825213697));
#50343=CARTESIAN_POINT('Ctrl Pts',(-4.87552386667384,-0.501309153611575,
392.510697338238));
#50344=CARTESIAN_POINT('Ctrl Pts',(-4.52435736725662,1.88473718468963,392.431569462777));
#50345=CARTESIAN_POINT('Ctrl Pts',(-3.07769361007314,3.81442602294447,392.352441587318));
#50346=CARTESIAN_POINT('Ctrl Pts',(-0.885817961698088,4.82051557208708,
392.273313711858));
#50347=CARTESIAN_POINT('Ctrl Pts',(1.52054364990864,4.65939812107997,392.194185836399));
#50348=CARTESIAN_POINT('Ctrl Pts',(3.55873111796869,3.37008555855818,392.115057960939));
#50349=CARTESIAN_POINT('Ctrl Pts',(4.73523152985659,1.2647632982709,392.035930085479));
#50350=CARTESIAN_POINT('Ctrl Pts',(4.76517504210868,-1.14680018314682,391.956802210019));
#50351=CARTESIAN_POINT('Ctrl Pts',(3.64131133542052,-3.28068523338327,391.877674334559));
#50352=CARTESIAN_POINT('Ctrl Pts',(1.63576515787017,-4.62020737524832,391.7985464591));
#50353=CARTESIAN_POINT('Ctrl Pts',(-0.765854118981568,-4.84102378742762,
391.71941858364));
#50354=CARTESIAN_POINT('Ctrl Pts',(-2.98203466518281,-3.88966747905899,
391.64029070818));
#50355=CARTESIAN_POINT('Ctrl Pts',(-4.47616552938631,-1.99649342486641,
391.56116283272));
#50356=CARTESIAN_POINT('Ctrl Pts',(-4.88646798113091,0.380098028649711,
391.482034957261));
#50357=CARTESIAN_POINT('Ctrl Pts',(-4.11359416297415,2.66465511921264,391.402907081801));
#50358=CARTESIAN_POINT('Ctrl Pts',(-2.34468250799326,4.30401066201183,391.323779206341));
#50359=CARTESIAN_POINT('Ctrl Pts',(-0.00804530674402572,4.90122220625023,
391.244651330881));
#50360=CARTESIAN_POINT('Ctrl Pts',(2.33053993060416,4.31168499242009,391.165523455421));
#50361=CARTESIAN_POINT('Ctrl Pts',(4.10482400961136,2.67814556962822,391.086395579962));
#50362=CARTESIAN_POINT('Ctrl Pts',(4.88519379734561,0.396138112754947,391.007267704502));
#50363=CARTESIAN_POINT('Ctrl Pts',(4.48269583741255,-1.98178754442679,390.928139829042));
#50364=CARTESIAN_POINT('Ctrl Pts',(2.99478826045289,-3.87985658459878,390.849011953582));
#50365=CARTESIAN_POINT('Ctrl Pts',(0.781742932293461,-4.8384834225003,390.769884078122));
#50366=CARTESIAN_POINT('Ctrl Pts',(-1.62058833618616,-4.62555264661623,
390.690756202663));
#50367=CARTESIAN_POINT('Ctrl Pts',(-3.63052131820232,-3.29262187323105,
390.611628327203));
#50368=CARTESIAN_POINT('Ctrl Pts',(-4.76138445106458,-1.16243793432658,
390.532500451743));
#50369=CARTESIAN_POINT('Ctrl Pts',(-4.7393581930353,1.24921085494409,390.453372576283));
#50370=CARTESIAN_POINT('Ctrl Pts',(-3.56977583309043,3.35838418640342,390.374244700824));
#50371=CARTESIAN_POINT('Ctrl Pts',(-1.53583212443933,4.65438111111899,390.295116825364));
#50372=CARTESIAN_POINT('Ctrl Pts',(0.869987575460632,4.82339770914085,390.215988949904));
#50373=CARTESIAN_POINT('Ctrl Pts',(3.06515437466237,3.82450944586218,390.136861074444));
#50374=CARTESIAN_POINT('Ctrl Pts',(4.51814544822977,1.89958036172247,390.057733198985));
#50375=CARTESIAN_POINT('Ctrl Pts',(4.87714337604219,-0.485300248844855,
389.978605323525));
#50376=CARTESIAN_POINT('Ctrl Pts',(4.05522283069102,-2.75267354320184,389.899477448065));
#50377=CARTESIAN_POINT('Ctrl Pts',(2.25139808767325,-4.35353310459702,389.820349572605));
#50378=CARTESIAN_POINT('Ctrl Pts',(-0.0975649437201896,-4.9002576385082,
389.741221697145));
#50379=CARTESIAN_POINT('Ctrl Pts',(-2.42290426026896,-4.26046696825261,
389.662093821685));
#50380=CARTESIAN_POINT('Ctrl Pts',(-4.16157794510521,-2.58907567460185,
389.582965946226));
#50381=CARTESIAN_POINT('Ctrl Pts',(-4.89259532501792,-0.290783128145012,
389.503838070766));
#50382=CARTESIAN_POINT('Ctrl Pts',(-4.43895280146969,2.07791767602217,389.424710195306));
#50383=CARTESIAN_POINT('Ctrl Pts',(-2.91049230342699,3.9434855640275,389.345582319846));
#50384=CARTESIAN_POINT('Ctrl Pts',(-0.67730490643744,4.85420455952536,389.266454444387));
#50385=CARTESIAN_POINT('Ctrl Pts',(1.71988051445791,4.58955933156866,389.187326568927));
#50386=CARTESIAN_POINT('Ctrl Pts',(3.70062571316616,3.21362928370005,389.108198693467));
#50387=CARTESIAN_POINT('Ctrl Pts',(4.78532645921196,1.05957280106983,389.029070818007));
#50388=CARTESIAN_POINT('Ctrl Pts',(4.71134065862855,-1.35104146507597,388.949942942548));
#50389=CARTESIAN_POINT('Ctrl Pts',(3.49658273219959,-3.43452369898426,388.870815067087));
#50390=CARTESIAN_POINT('Ctrl Pts',(1.43518593891208,-4.68639362012519,388.791687191628));
#50391=CARTESIAN_POINT('Ctrl Pts',(-0.973717059752046,-4.80353192240344,
388.712559316168));
#50392=CARTESIAN_POINT('Ctrl Pts',(-3.14685080276043,-3.75757553046736,
388.633431440709));
#50393=CARTESIAN_POINT('Ctrl Pts',(-4.55802740021425,-1.80178524272377,
388.554303565248));
#50394=CARTESIAN_POINT('Ctrl Pts',(-4.8655541061066,0.590277123519319,388.475175689789));
#50395=CARTESIAN_POINT('Ctrl Pts',(-3.9949684861848,2.83941378393346,388.396047814329));
#50396=CARTESIAN_POINT('Ctrl Pts',(-2.15706824758342,4.401034016827,388.316919938869));
#50397=CARTESIAN_POINT('Ctrl Pts',(0.2031298906366,4.89701767298537,388.237792063409));
#50398=CARTESIAN_POINT('Ctrl Pts',(2.51414353256258,4.20727062829036,388.15866418795));
#50399=CARTESIAN_POINT('Ctrl Pts',(4.21639948317845,2.49880356175781,388.07953631249));
#50400=CARTESIAN_POINT('Ctrl Pts',(4.8977250128471,0.185293120576435,388.00040843703));
#50401=CARTESIAN_POINT('Ctrl Pts',(4.39314857117775,-2.17308294217223,387.92128056157));
#50402=CARTESIAN_POINT('Ctrl Pts',(2.82484488118912,-4.00528341559255,387.842152686111));
#50403=CARTESIAN_POINT('Ctrl Pts',(0.572552379142054,-4.86767168317048,
387.763024810651));
#50404=CARTESIAN_POINT('Ctrl Pts',(-1.8183740791475,-4.55143488916249,387.683896935191));
#50405=CARTESIAN_POINT('Ctrl Pts',(-3.76901175041157,-3.13314446958014,
387.604769059731));
#50406=CARTESIAN_POINT('Ctrl Pts',(-4.80704643700727,-0.956215663151738,
387.525641184272));
#50407=CARTESIAN_POINT('Ctrl Pts',(-4.68113544861982,1.45224472926429,387.446513308812));
#50408=CARTESIAN_POINT('Ctrl Pts',(-3.4217660194141,3.50906841631565,387.367385433352));
#50409=CARTESIAN_POINT('Ctrl Pts',(-1.33387333558782,4.71623003749912,387.288257557892));
#50410=CARTESIAN_POINT('Ctrl Pts',(1.07699440584981,4.78143565174407,387.209129682432));
#50411=CARTESIAN_POINT('Ctrl Pts',(3.22708601435485,3.68889681313483,387.130001806972));
#50412=CARTESIAN_POINT('Ctrl Pts',(4.59579286645524,1.70315347829848,387.050873931513));
#50413=CARTESIAN_POINT('Ctrl Pts',(4.85170555271451,-0.694979907450764,
386.971746056053));
#50414=CARTESIAN_POINT('Ctrl Pts',(3.93285910810722,-2.92483556422906,386.892618180594));
#50415=CARTESIAN_POINT('Ctrl Pts',(2.06173678907561,-4.44649134201037,386.813490305133));
#50416=CARTESIAN_POINT('Ctrl Pts',(-0.308600515715983,-4.89150381413537,
386.734362429674));
#50417=CARTESIAN_POINT('Ctrl Pts',(-2.60421538121517,-4.15212067385372,
386.655234554214));
#50418=CARTESIAN_POINT('Ctrl Pts',(-4.26926316786226,-2.40737114827269,
386.576106678754));
#50419=CARTESIAN_POINT('Ctrl Pts',(-4.90058047890116,-0.0797170735407659,
386.496978803294));
#50420=CARTESIAN_POINT('Ctrl Pts',(-4.34530441538657,2.26723915360136,386.417850927834));
#50421=CARTESIAN_POINT('Ctrl Pts',(-2.7378857634756,4.06522144392636,386.338723052375));
#50422=CARTESIAN_POINT('Ctrl Pts',(-0.46753399145535,4.87887854007813,386.259595176915));
#50423=CARTESIAN_POINT('Ctrl Pts',(1.91602329550907,4.51119702219572,386.180467301455));
#50424=CARTESIAN_POINT('Ctrl Pts',(3.83564767539653,3.05120480338935,386.101339425996));
#50425=CARTESIAN_POINT('Ctrl Pts',(4.82653429894221,0.852414513681883,386.022211550536));
#50426=CARTESIAN_POINT('Ctrl Pts',(4.6487565885712,-1.55277365453466,385.943083675076));
#50427=CARTESIAN_POINT('Ctrl Pts',(3.34536043531169,-3.58198372411883,385.863955799616));
#50428=CARTESIAN_POINT('Ctrl Pts',(1.23194135821188,-4.74387650892475,385.784827924157));
#50429=CARTESIAN_POINT('Ctrl Pts',(-1.17977165769507,-4.75711915739983,
385.705700048696));
#50430=CARTESIAN_POINT('Ctrl Pts',(-3.30582275282872,-3.61850518431036,
385.626572173237));
#50431=CARTESIAN_POINT('Ctrl Pts',(-4.63142431084255,-1.60373086736447,
385.547444297777));
#50432=CARTESIAN_POINT('Ctrl Pts',(-4.8356041463375,0.799359982689007,385.468316422318));
#50433=CARTESIAN_POINT('Ctrl Pts',(-3.86892353648086,3.00889921912741,385.389188546857));
#50434=CARTESIAN_POINT('Ctrl Pts',(-1.96544797859558,4.48988397238009,385.310060671398));
#50435=CARTESIAN_POINT('Ctrl Pts',(0.413927844466849,4.88371862227708,385.230932795938));
#50436=CARTESIAN_POINT('Ctrl Pts',(2.69307798204115,4.09504271340925,385.151804920478));
#50437=CARTESIAN_POINT('Ctrl Pts',(4.32014445230215,2.31482089010014,385.072677045018));
#50438=CARTESIAN_POINT('Ctrl Pts',(4.90116039726593,-0.0258959895184648,
384.993549169559));
#50439=CARTESIAN_POINT('Ctrl Pts',(4.29544255017007,-2.3603425895809,384.914421294099));
#50440=CARTESIAN_POINT('Ctrl Pts',(2.6496553290988,-4.12327181725621,384.835293418639));
#50441=CARTESIAN_POINT('Ctrl Pts',(0.362298507876016,-4.88781992642853,
384.756165543179));
#50442=CARTESIAN_POINT('Ctrl Pts',(-2.01278282086323,-4.46886441481938,
384.67703766772));
#50443=CARTESIAN_POINT('Ctrl Pts',(-3.90050254623037,-2.96784833319553,
384.59790979226));
#50444=CARTESIAN_POINT('Ctrl Pts',(-4.84378099597461,-0.748217551943446,
384.5187819168));
#50445=CARTESIAN_POINT('Ctrl Pts',(-4.61421911336287,1.65258156103648,384.43965404134));
#50446=CARTESIAN_POINT('Ctrl Pts',(-3.26740145825086,3.65323576471889,384.36052616588));
#50447=CARTESIAN_POINT('Ctrl Pts',(-1.12943733813143,4.76932019697102,384.281398290421));
#50448=CARTESIAN_POINT('Ctrl Pts',(1.28200109144381,4.730593730552,384.202270414961));
#50449=CARTESIAN_POINT('Ctrl Pts',(3.38302445736953,3.54643332981752,384.123142539501));
#50450=CARTESIAN_POINT('Ctrl Pts',(4.66490518818293,1.50356357606356,384.044014664042));
#50451=CARTESIAN_POINT('Ctrl Pts',(4.81725736354257,-0.903368881131035,
383.964886788581));
#50452=CARTESIAN_POINT('Ctrl Pts',(3.80319145930759,-3.09156571430251,383.885758913122));
#50453=CARTESIAN_POINT('Ctrl Pts',(1.86824652712842,-4.53119175889452,383.806631037662));
#50454=CARTESIAN_POINT('Ctrl Pts',(-0.519062968936094,-4.87366571240583,
383.727503162202));
#50455=CARTESIAN_POINT('Ctrl Pts',(-2.78069007236013,-4.03606325067867,
383.648375286742));
#50456=CARTESIAN_POINT('Ctrl Pts',(-4.36901971015636,-2.22119576225652,
383.569247411283));
#50457=CARTESIAN_POINT('Ctrl Pts',(-4.89946449866066,0.131497027969629,
383.490119535823));
#50458=CARTESIAN_POINT('Ctrl Pts',(-4.24358612851044,2.45235001823044,383.410991660363));
#50459=CARTESIAN_POINT('Ctrl Pts',(-2.56019454719736,4.17940758032786,383.331863784903));
#50460=CARTESIAN_POINT('Ctrl Pts',(-0.256894793709217,4.89449169035623,
383.252735909444));
#50461=CARTESIAN_POINT('Ctrl Pts',(2.10860772565226,4.4244567238612,383.173608033984));
#50462=CARTESIAN_POINT('Ctrl Pts',(3.96354624804163,2.88311376494861,383.094480158524));
#50463=CARTESIAN_POINT('Ctrl Pts',(4.85877851973045,0.643673161011885,383.015352283064));
#50464=CARTESIAN_POINT('Ctrl Pts',(4.57753906021165,-1.7516221037192,382.936224407605));
#50465=CARTESIAN_POINT('Ctrl Pts',(3.18792528789615,-3.72279145276676,382.857096532144));
#50466=CARTESIAN_POINT('Ctrl Pts',(1.0264088723172,-4.79254928705272,382.777968656685));
#50467=CARTESIAN_POINT('Ctrl Pts',(-1.38363523762741,-4.70187168808304,
382.698840781225));
#50468=CARTESIAN_POINT('Ctrl Pts',(-3.45865527994654,-3.47271471567979,
382.619712905766));
#50469=CARTESIAN_POINT('Ctrl Pts',(-4.69621995188282,-1.40269811632394,
382.540585030305));
#50470=CARTESIAN_POINT('Ctrl Pts',(-4.79667372352029,1.00695830702717,382.461457154846));
#50471=CARTESIAN_POINT('Ctrl Pts',(-3.73569339878306,3.17279666418915,382.382329279386));
#50472=CARTESIAN_POINT('Ctrl Pts',(-1.77017756943694,4.57039552059375,382.303201403927));
#50473=CARTESIAN_POINT('Ctrl Pts',(0.623957070419554,4.86134975251467,382.224073528466));
#50474=CARTESIAN_POINT('Ctrl Pts',(2.86701097015694,3.97520967233186,382.144945653007));
#50475=CARTESIAN_POINT('Ctrl Pts',(4.41586624656651,2.12653923886574,382.065817777547));
#50476=CARTESIAN_POINT('Ctrl Pts',(4.89549357056314,-0.237037006764906,
381.986689902087));
#50477=CARTESIAN_POINT('Ctrl Pts',(4.18975922954695,-2.54321871659263,381.907562026627));
#50478=CARTESIAN_POINT('Ctrl Pts',(2.46954495821251,-4.2336026669219,381.828434151167));
#50479=CARTESIAN_POINT('Ctrl Pts',(0.151371792377024,-4.89889073387779,
381.749306275708));
#50480=CARTESIAN_POINT('Ctrl Pts',(-2.20345351430222,-4.37799456969858,
381.670178400248));
#50481=CARTESIAN_POINT('Ctrl Pts',(-4.0247495069615,-2.79704044450812,381.591050524788));
#50482=CARTESIAN_POINT('Ctrl Pts',(-4.87151990622233,-0.53882988528894,
381.511922649328));
#50483=CARTESIAN_POINT('Ctrl Pts',(-4.53873346122441,1.84984929385154,381.432794773869));
#50484=CARTESIAN_POINT('Ctrl Pts',(-3.10696882840965,3.79061849060175,381.353666898409));
#50485=CARTESIAN_POINT('Ctrl Pts',(-0.922903801262455,4.8135529929166,381.274539022949));
#50486=CARTESIAN_POINT('Ctrl Pts',(1.48462690319438,4.67096636685734,381.195411147489));
#50487=CARTESIAN_POINT('Ctrl Pts',(3.53268010195595,3.39738357258133,381.11628327203));
#50488=CARTESIAN_POINT('Ctrl Pts',(4.72535406116718,1.30118132426344,381.03715539657));
#50489=CARTESIAN_POINT('Ctrl Pts',(4.77386278412913,-1.11008015940651,380.95802752111));
#50490=CARTESIAN_POINT('Ctrl Pts',(3.66646069712405,-3.25255434980657,380.87889964565));
#50491=CARTESIAN_POINT('Ctrl Pts',(1.67128664310421,-4.60747705350581,380.799771770191));
#50492=CARTESIAN_POINT('Ctrl Pts',(-0.728561442129978,-4.84677646142697,
380.72064389473));
#50493=CARTESIAN_POINT('Ctrl Pts',(-2.95200059297187,-3.91251023527028,
380.641516019271));
#50494=CARTESIAN_POINT('Ctrl Pts',(-4.46066230869571,-2.03089527297259,
380.562388143811));
#50495=CARTESIAN_POINT('Ctrl Pts',(-4.88924945684393,0.342466919208695,
380.483260268352));
#50496=CARTESIAN_POINT('Ctrl Pts',(-4.13398684739545,2.63290649047066,380.404132392891));
#50497=CARTESIAN_POINT('Ctrl Pts',(-2.37774865459918,4.28583191195745,380.325004517432));
#50498=CARTESIAN_POINT('Ctrl Pts',(-0.045778502691498,4.90101501433043,
380.245876641972));
#50499=CARTESIAN_POINT('Ctrl Pts',(2.29727614588441,4.32949952668338,380.166748766512));
#50500=CARTESIAN_POINT('Ctrl Pts',(4.08408390371697,2.70966833937311,380.087620891052));
#50501=CARTESIAN_POINT('Ctrl Pts',(4.88199923908331,0.433736407961101,380.008493015593));
#50502=CARTESIAN_POINT('Ctrl Pts',(4.49782033548913,-1.94721752037656,379.929365140133));
#50503=CARTESIAN_POINT('Ctrl Pts',(3.02456967131446,-3.8566853832489,379.850237264673));
#50504=CARTESIAN_POINT('Ctrl Pts',(0.818970186768649,-4.83232156164975,
379.771109389213));
#50505=CARTESIAN_POINT('Ctrl Pts',(-1.5849291934243,-4.63789211752843,379.691981513754));
#50506=CARTESIAN_POINT('Ctrl Pts',(-3.60506455052847,-3.32047487997185,
379.612853638294));
#50507=CARTESIAN_POINT('Ctrl Pts',(-4.75229398783147,-1.19906033844088,
379.533725762834));
#50508=CARTESIAN_POINT('Ctrl Pts',(-4.74883513745721,1.21268655441244,379.454597887374));
#50509=CARTESIAN_POINT('Ctrl Pts',(-3.59552550201493,3.33080173627333,379.375470011914));
#50510=CARTESIAN_POINT('Ctrl Pts',(-1.57161966738812,4.64241913909978,379.296342136455));
#50511=CARTESIAN_POINT('Ctrl Pts',(0.832827511814025,4.82995260614083,379.217214260995));
#50512=CARTESIAN_POINT('Ctrl Pts',(3.03561947651265,3.84799405350607,379.138086385535));
#50513=CARTESIAN_POINT('Ctrl Pts',(4.50338709582942,1.93430827613337,379.058958510075));
#50514=CARTESIAN_POINT('Ctrl Pts',(4.88073505691033,-0.447737809714184,
378.979830634616));
#50515=CARTESIAN_POINT('Ctrl Pts',(4.07629487954206,-2.72137169402128,378.900702759156));
#50516=CARTESIAN_POINT('Ctrl Pts',(2.28484826128058,-4.33607106317736,378.821574883696));
#50517=CARTESIAN_POINT('Ctrl Pts',(-0.0598360438974424,-4.90086354532054,
378.742447008237));
#50518=CARTESIAN_POINT('Ctrl Pts',(-2.39003205456549,-4.27899411312408,
378.663319132776));
#50519=CARTESIAN_POINT('Ctrl Pts',(-4.14152188682712,-2.62103802012351,
378.584191257317));
#50520=CARTESIAN_POINT('Ctrl Pts',(-4.89021165231393,-0.328441528394388,
378.505063381857));
#50521=CARTESIAN_POINT('Ctrl Pts',(-4.45481868070814,2.04368157109047,378.425935506397));
#50522=CARTESIAN_POINT('Ctrl Pts',(-2.94076607803947,3.92096145304356,378.346807630937));
#50523=CARTESIAN_POINT('Ctrl Pts',(-0.714656289627798,4.84884627820851,
378.267679755477));
#50524=CARTESIAN_POINT('Ctrl Pts',(1.68449553370326,4.60266429787517,378.188551880018));
#50525=CARTESIAN_POINT('Ctrl Pts',(3.67577501448982,3.24202434982427,378.109424004558));
#50526=CARTESIAN_POINT('Ctrl Pts',(4.77702722252339,1.09638257796792,378.030296129098));
#50527=CARTESIAN_POINT('Ctrl Pts',(4.72160240490404,-1.31472984753725,377.951168253638));
#50528=CARTESIAN_POINT('Ctrl Pts',(3.52292075167996,-3.40750249000403,377.872040378179));
#50529=CARTESIAN_POINT('Ctrl Pts',(1.47122292189925,-4.67520555228101,377.792912502719));
#50530=CARTESIAN_POINT('Ctrl Pts',(-0.936706864306466,-4.81088599868696,
377.713784627259));
#50531=CARTESIAN_POINT('Ctrl Pts',(-3.11782879297974,-3.78169108464289,
377.634656751799));
#50532=CARTESIAN_POINT('Ctrl Pts',(-4.54402076903412,-1.83682309779347,
377.555528876339));
#50533=CARTESIAN_POINT('Ctrl Pts',(-4.86995432435985,0.552800796535157,
377.47640100088));
#50534=CARTESIAN_POINT('Ctrl Pts',(-4.01671011481814,2.80857324909262,377.39727312542));
#50535=CARTESIAN_POINT('Ctrl Pts',(-2.19088691585556,4.3842967924097,377.31814524996));
#50536=CARTESIAN_POINT('Ctrl Pts',(0.165422806069439,4.89843639718154,377.2390173745));
#50537=CARTESIAN_POINT('Ctrl Pts',(2.48167816983692,4.22650178082969,377.159889499041));
#50538=CARTESIAN_POINT('Ctrl Pts',(4.19703678539643,2.53119064158134,377.080761623581));
#50539=CARTESIAN_POINT('Ctrl Pts',(4.89615333254211,0.222994139474255,377.001633748121));
#50540=CARTESIAN_POINT('Ctrl Pts',(4.40974846437591,-2.13919665363753,376.922505872661));
#50541=CARTESIAN_POINT('Ctrl Pts',(2.85559696215369,-3.98341685387501,376.843377997201));
#50542=CARTESIAN_POINT('Ctrl Pts',(0.610010547211784,-4.86311946946737,
376.764250121742));
#50543=CARTESIAN_POINT('Ctrl Pts',(-1.78327969114604,-4.56529926566563,
376.685122246282));
#50544=CARTESIAN_POINT('Ctrl Pts',(-3.74477865997579,-3.16206841006309,
376.605994370822));
#50545=CARTESIAN_POINT('Ctrl Pts',(-4.79954228053442,-0.99319572046786,
376.526866495362));
#50546=CARTESIAN_POINT('Ctrl Pts',(-4.69217723182007,1.41616265569688,376.447738619902));
#50547=CARTESIAN_POINT('Ctrl Pts',(-3.44868015951322,3.48262099568224,376.368610744443));
#50548=CARTESIAN_POINT('Ctrl Pts',(-1.37014302527182,4.70582106870975,376.289482868983));
#50549=CARTESIAN_POINT('Ctrl Pts',(1.04015126435086,4.78958549295691,376.210354993523));
#50550=CARTESIAN_POINT('Ctrl Pts',(3.1985903683765,3.71363211500125,376.131227118063));
#50551=CARTESIAN_POINT('Ctrl Pts',(4.58254446188996,1.73848500650345,376.052099242604));
#50552=CARTESIAN_POINT('Ctrl Pts',(4.85691226192656,-0.657607098782336,
375.972971367144));
#50553=CARTESIAN_POINT('Ctrl Pts',(3.95526022777064,-2.89447065515981,375.893843491684));
#50554=CARTESIAN_POINT('Ctrl Pts',(2.09590823415934,-4.43048672573689,375.814715616224));
#50555=CARTESIAN_POINT('Ctrl Pts',(-0.270932724915457,-4.89373465602332,
375.735587740765));
#50556=CARTESIAN_POINT('Ctrl Pts',(-2.57217200103202,-4.17204699080374,
375.656459865305));
#50557=CARTESIAN_POINT('Ctrl Pts',(-4.25060268497819,-2.44016774048634,
375.577331989845));
#50558=CARTESIAN_POINT('Ctrl Pts',(-4.8998218096771,-0.117443592583374,
375.498204114385));
#50559=CARTESIAN_POINT('Ctrl Pts',(-4.36263000323237,2.23371923670199,375.419076238926));
#50560=CARTESIAN_POINT('Ctrl Pts',(-2.76910316484765,4.04402084944263,375.339948363465));
#50561=CARTESIAN_POINT('Ctrl Pts',(-0.505078814327535,4.87513818307261,
375.260820488006));
#50562=CARTESIAN_POINT('Ctrl Pts',(1.88123000134211,4.52580661359865,375.181692612546));
#50563=CARTESIAN_POINT('Ctrl Pts',(3.81205567946445,3.08066074485737,375.102564737086));
#50564=CARTESIAN_POINT('Ctrl Pts',(4.81980261485754,0.889513660705449,375.023436861627));
#50565=CARTESIAN_POINT('Ctrl Pts',(4.6606270588275,-1.51685826939215,374.944308986167));
#50566=CARTESIAN_POINT('Ctrl Pts',(3.37271297305025,-3.55624114494146,374.865181110707));
#50567=CARTESIAN_POINT('Ctrl Pts',(1.96999142168877,-4.34109857602843,374.812429193734));
#50568=CARTESIAN_POINT('Ctrl Pts',(1.21713437249897,-4.54280821229842,374.786053235247));
#50569=CARTESIAN_POINT('Ctrl Pts',(3.71544298812251,3.17665283523749,400.213946764753));
#50570=CARTESIAN_POINT('Ctrl Pts',(4.24189388987153,2.56091091663784,400.187570806266));
#50571=CARTESIAN_POINT('Ctrl Pts',(4.98214581433909,1.06316653552657,400.134818889293));
#50572=CARTESIAN_POINT('Ctrl Pts',(4.88599424296224,-1.44202664096201,400.055691013833));
#50573=CARTESIAN_POINT('Ctrl Pts',(3.60674265589465,-3.5976617763163,399.976563138373));
#50574=CARTESIAN_POINT('Ctrl Pts',(1.45418293597717,-4.88238291434578,399.897435262914));
#50575=CARTESIAN_POINT('Ctrl Pts',(-1.05048684560331,-4.98482476427098,
399.818307387454));
#50576=CARTESIAN_POINT('Ctrl Pts',(-3.30079722370572,-3.88031872051941,
399.739179511994));
#50577=CARTESIAN_POINT('Ctrl Pts',(-4.75187572291575,-1.83623790534267,
399.660051636534));
#50578=CARTESIAN_POINT('Ctrl Pts',(-5.05236683263146,0.652447348843657,
399.580923761074));
#50579=CARTESIAN_POINT('Ctrl Pts',(-4.12951222709533,2.98315803806871,399.501795885615));
#50580=CARTESIAN_POINT('Ctrl Pts',(-2.20676540787796,4.59154485677586,399.422668010155));
#50581=CARTESIAN_POINT('Ctrl Pts',(0.250312604852073,5.08816712539591,399.343540134695));
#50582=CARTESIAN_POINT('Ctrl Pts',(2.64678163724731,4.35277457160906,399.264412259235));
#50583=CARTESIAN_POINT('Ctrl Pts',(4.40237687684668,2.5634308867403,399.185284383776));
#50584=CARTESIAN_POINT('Ctrl Pts',(5.09201039289903,0.153395295488701,399.106156508315));
#50585=CARTESIAN_POINT('Ctrl Pts',(4.54869898923014,-2.29378234250105,399.027028632856));
#50586=CARTESIAN_POINT('Ctrl Pts',(2.90399641321393,-4.1855590799549,398.947900757396));
#50587=CARTESIAN_POINT('Ctrl Pts',(0.556139808676901,-5.06387287138275,
398.868772881936));
#50588=CARTESIAN_POINT('Ctrl Pts',(-1.92637672321179,-4.7160547794503,398.789645006477));
#50589=CARTESIAN_POINT('Ctrl Pts',(-3.94245343924376,-3.22632311381047,
398.710517131017));
#50590=CARTESIAN_POINT('Ctrl Pts',(-5.00393117442772,-0.955391416550765,
398.631389255557));
#50591=CARTESIAN_POINT('Ctrl Pts',(-4.85379089746955,1.54687228977885,398.552261380098));
#50592=CARTESIAN_POINT('Ctrl Pts',(-3.52838655837555,3.67458681370817,398.473133504638));
#50593=CARTESIAN_POINT('Ctrl Pts',(-1.34864258930642,4.91256176790427,398.394005629178));
#50594=CARTESIAN_POINT('Ctrl Pts',(1.15765256446685,4.96104227929438,398.314877753718));
#50595=CARTESIAN_POINT('Ctrl Pts',(3.38364156492812,3.80828960520879,398.235749878258));
#50596=CARTESIAN_POINT('Ctrl Pts',(4.79033850803188,1.73342347263734,398.156622002798));
#50597=CARTESIAN_POINT('Ctrl Pts',(5.03713532094231,-0.761162082306909,
398.077494127339));
#50598=CARTESIAN_POINT('Ctrl Pts',(4.064274294482,-3.07144500459355,397.998366251879));
#50599=CARTESIAN_POINT('Ctrl Pts',(2.10731741020158,-4.63802903070772,397.919238376419));
#50600=CARTESIAN_POINT('Ctrl Pts',(-0.359891042804634,-5.08159211215712,
397.840110500959));
#50601=CARTESIAN_POINT('Ctrl Pts',(-2.73995791558548,-4.29473288783458,
397.7609826255));
#50602=CARTESIAN_POINT('Ctrl Pts',(-4.45658993137603,-2.46797612236942,
397.68185475004));
#50603=CARTESIAN_POINT('Ctrl Pts',(-5.0941334374604,-0.0436403296913884,
397.60272687458));
#50604=CARTESIAN_POINT('Ctrl Pts',(-4.49821796618352,2.39126223692249,397.52359899912));
#50605=CARTESIAN_POINT('Ctrl Pts',(-2.81313445472219,4.24716075710381,397.44447112366));
#50606=CARTESIAN_POINT('Ctrl Pts',(-0.446897614573966,5.07468052975907,
397.365343248201));
#50607=CARTESIAN_POINT('Ctrl Pts',(2.02754798795257,4.67345152040515,397.286215372741));
#50608=CARTESIAN_POINT('Ctrl Pts',(4.01105684952524,3.14062460458175,397.207087497281));
#50609=CARTESIAN_POINT('Ctrl Pts',(5.02335556505595,0.847348112672217,397.127959621822));
#50610=CARTESIAN_POINT('Ctrl Pts',(4.8193329780012,-1.65109951371132,397.048831746361));
#50611=CARTESIAN_POINT('Ctrl Pts',(3.44838973612117,-3.74976108370145,396.969703870902));
#50612=CARTESIAN_POINT('Ctrl Pts',(1.24247675313054,-4.94048089511111,396.890575995442));
#50613=CARTESIAN_POINT('Ctrl Pts',(-1.26428113785597,-4.93494611535824,
396.811448119982));
#50614=CARTESIAN_POINT('Ctrl Pts',(-3.46491455477013,-3.73449689853531,
396.732320244522));
#50615=CARTESIAN_POINT('Ctrl Pts',(-4.82657702287821,-1.62980188957181,
396.653192369063));
#50616=CARTESIAN_POINT('Ctrl Pts',(-5.01956481218505,0.869522313285533,
396.574064493603));
#50617=CARTESIAN_POINT('Ctrl Pts',(-3.99714916613881,3.15830627087741,396.494936618143));
#50618=CARTESIAN_POINT('Ctrl Pts',(-2.00689088633465,4.68235933343167,396.415808742683));
#50619=CARTESIAN_POINT('Ctrl Pts',(0.469302363710116,5.07265761198643,396.336680867223));
#50620=CARTESIAN_POINT('Ctrl Pts',(2.83186191712685,4.23469692414397,396.257552991764));
#50621=CARTESIAN_POINT('Ctrl Pts',(4.50873360091663,2.37137539689376,396.178425116304));
#50622=CARTESIAN_POINT('Ctrl Pts',(5.09389105993074,-0.066134912001412,
396.099297240844));
#50623=CARTESIAN_POINT('Ctrl Pts',(4.44564822923743,-2.48763176111453,396.020169365385));
#50624=CARTESIAN_POINT('Ctrl Pts',(2.72096623850579,-4.30679029974057,395.941041489925));
#50625=CARTESIAN_POINT('Ctrl Pts',(0.337447906876279,-5.08313179714755,
395.861913614465));
#50626=CARTESIAN_POINT('Ctrl Pts',(-2.12777777601096,-4.6286781798848,395.782785739005));
#50627=CARTESIAN_POINT('Ctrl Pts',(-4.07779775573568,-3.05346776965875,
395.703657863545));
#50628=CARTESIAN_POINT('Ctrl Pts',(-5.04044739830187,-0.738911349202079,
395.624529988086));
#50629=CARTESIAN_POINT('Ctrl Pts',(-4.78263723751197,1.75456006206446,395.545402112625));
#50630=CARTESIAN_POINT('Ctrl Pts',(-3.36679168002614,3.82319418030715,395.466274237166));
#50631=CARTESIAN_POINT('Ctrl Pts',(-1.13573398221921,4.9661059471844,395.387146361706));
#50632=CARTESIAN_POINT('Ctrl Pts',(1.37032265180738,4.90655844630137,395.308018486247));
#50633=CARTESIAN_POINT('Ctrl Pts',(3.54457863759732,3.65897010631632,395.228890610786));
#50634=CARTESIAN_POINT('Ctrl Pts',(4.86057435298355,1.52542352025471,395.149762735327));
#50635=CARTESIAN_POINT('Ctrl Pts',(4.99966350625814,-0.977478788116796,
395.070634859867));
#50636=CARTESIAN_POINT('Ctrl Pts',(3.9281679916419,-3.24370100139759,394.991506984407));
#50637=CARTESIAN_POINT('Ctrl Pts',(1.90553247777794,-4.72451541781389,394.912379108947));
#50638=CARTESIAN_POINT('Ctrl Pts',(-0.578495767592555,-5.0613676614039,
394.833251233488));
#50639=CARTESIAN_POINT('Ctrl Pts',(-2.92245096488478,-4.17269461078471,
394.754123358028));
#50640=CARTESIAN_POINT('Ctrl Pts',(-4.55878367391877,-2.27367354108707,
394.674995482568));
#50641=CARTESIAN_POINT('Ctrl Pts',(-5.09128337239731,0.175879444445247,
394.595867607109));
#50642=CARTESIAN_POINT('Ctrl Pts',(-4.39101418897073,2.58284617220721,394.516739731648));
#50643=CARTESIAN_POINT('Ctrl Pts',(-2.62753456208024,4.36442001669197,394.437611856189));
#50644=CARTESIAN_POINT('Ctrl Pts',(-0.227841507780872,5.08922275051504,
394.358483980729));
#50645=CARTESIAN_POINT('Ctrl Pts',(2.22701954646155,4.58175554746277,394.279356105269));
#50646=CARTESIAN_POINT('Ctrl Pts',(4.14264516722633,2.96489307994134,394.200228229809));
#50647=CARTESIAN_POINT('Ctrl Pts',(5.05519873770637,0.630131477804167,394.12110035435));
#50648=CARTESIAN_POINT('Ctrl Pts',(4.74372071539057,-1.85720589364835,394.04197247889));
#50649=CARTESIAN_POINT('Ctrl Pts',(3.28363027953537,-3.89485200544849,393.96284460343));
#50650=CARTESIAN_POINT('Ctrl Pts',(1.02846384177488,-4.98942502530997,393.883716727971));
#50651=CARTESIAN_POINT('Ctrl Pts',(-1.47572786674121,-4.87589245373102,
393.80458885251));
#50652=CARTESIAN_POINT('Ctrl Pts',(-3.62259682199201,-3.58174429884674,
393.725460977051));
#50653=CARTESIAN_POINT('Ctrl Pts',(-4.89231471194326,-1.42033683199839,
393.646333101591));
#50654=CARTESIAN_POINT('Ctrl Pts',(-4.97744064418338,1.0849813780241,393.567205226131));
#50655=CARTESIAN_POINT('Ctrl Pts',(-3.85736280188092,3.32758954375282,393.488077350671));
#50656=CARTESIAN_POINT('Ctrl Pts',(-1.8032892495463,4.76447770899377,393.408949475212));
#50657=CARTESIAN_POINT('Ctrl Pts',(0.687420551315965,5.04772750281314,393.329821599752));
#50658=CARTESIAN_POINT('Ctrl Pts',(3.01168299451616,4.1087547380648,393.250693724292));
#50659=CARTESIAN_POINT('Ctrl Pts',(4.60671691000739,2.1749159220714,393.171565848832));
#50660=CARTESIAN_POINT('Ctrl Pts',(5.08631158572023,-0.285542308591735,
393.092437973373));
#50661=CARTESIAN_POINT('Ctrl Pts',(4.33434121428917,-2.67686125810472,393.013310097913));
#50662=CARTESIAN_POINT('Ctrl Pts',(2.5328828097419,-4.42002314803234,392.934182222453));
#50663=CARTESIAN_POINT('Ctrl Pts',(0.118129312194917,-5.09295056157313,
392.855054346993));
#50664=CARTESIAN_POINT('Ctrl Pts',(-2.32522721713463,-4.53270541131057,
392.775926471534));
#50665=CARTESIAN_POINT('Ctrl Pts',(-4.20556897258945,-2.87494166442045,
392.696798596073));
#50666=CARTESIAN_POINT('Ctrl Pts',(-5.06760273359595,-0.521059009593531,
392.617670720614));
#50667=CARTESIAN_POINT('Ctrl Pts',(-4.70260148223132,1.95898934564318,392.538542845154));
#50668=CARTESIAN_POINT('Ctrl Pts',(-3.19894415001964,3.96470128535339,392.459414969695));
#50669=CARTESIAN_POINT('Ctrl Pts',(-0.920716141880372,5.01042730144931,
392.380287094234));
#50670=CARTESIAN_POINT('Ctrl Pts',(1.58044783853879,4.84296237717018,392.301159218775));
#50671=CARTESIAN_POINT('Ctrl Pts',(3.69893288079714,3.50285533534937,392.222031343315));
#50672=CARTESIAN_POINT('Ctrl Pts',(4.92178336136043,1.31459062101607,392.142903467856));
#50673=CARTESIAN_POINT('Ctrl Pts',(4.9529065449796,-1.19198016498848,392.063775592395));
#50674=CARTESIAN_POINT('Ctrl Pts',(3.78476647471314,-3.40993294492945,391.984647716936));
#50675=CARTESIAN_POINT('Ctrl Pts',(1.70020867751367,-4.80222765078197,391.905519841476));
#50676=CARTESIAN_POINT('Ctrl Pts',(-0.796026136476369,-5.03174346991918,
391.826391966016));
#50677=CARTESIAN_POINT('Ctrl Pts',(-3.09951657179924,-4.04290699598317,
391.747264090556));
#50678=CARTESIAN_POINT('Ctrl Pts',(-4.65251105174488,-2.07514839720426,
391.668136215097));
#50679=CARTESIAN_POINT('Ctrl Pts',(-5.07897800851123,0.395072583314779,
391.589008339637));
#50680=CARTESIAN_POINT('Ctrl Pts',(-4.27565562086226,2.76963336360912,391.509880464177));
#50681=CARTESIAN_POINT('Ctrl Pts',(-2.43705493231998,4.47357387486589,391.430752588717));
#50682=CARTESIAN_POINT('Ctrl Pts',(-0.00836226415120685,5.0943134993408,
391.351624713257));
#50683=CARTESIAN_POINT('Ctrl Pts',(2.42235518603692,4.48155054748998,391.272496837798));
#50684=CARTESIAN_POINT('Ctrl Pts',(4.26653995362923,2.78365529135943,391.193368962338));
#50685=CARTESIAN_POINT('Ctrl Pts',(5.0776536262684,0.411744591550536,391.114241086878));
#50686=CARTESIAN_POINT('Ctrl Pts',(4.65929863144093,-2.05986315566845,391.035113211418));
#50687=CARTESIAN_POINT('Ctrl Pts',(3.11277261484635,-4.03270958603397,390.955985335959));
#50688=CARTESIAN_POINT('Ctrl Pts',(0.812540914369942,-5.02910302335342,
390.876857460499));
#50689=CARTESIAN_POINT('Ctrl Pts',(-1.68443394126863,-4.80778350745226,
390.797729585039));
#50690=CARTESIAN_POINT('Ctrl Pts',(-3.7735513679378,-3.42233984732121,390.718601709579));
#50691=CARTESIAN_POINT('Ctrl Pts',(-4.94896661768926,-1.20823398976565,
390.639473834119));
#50692=CARTESIAN_POINT('Ctrl Pts',(-4.92607260087128,1.29842546492777,390.56034595866));
#50693=CARTESIAN_POINT('Ctrl Pts',(-3.71041271969718,3.49069296938833,390.4812180832));
#50694=CARTESIAN_POINT('Ctrl Pts',(-1.59633862636855,4.83774771427692,390.40209020774));
#50695=CARTESIAN_POINT('Ctrl Pts',(0.904262092886961,5.01342298478748,390.32296233228));
#50696=CARTESIAN_POINT('Ctrl Pts',(3.18591091187283,3.97518196044373,390.243834456821));
#50697=CARTESIAN_POINT('Ctrl Pts',(4.69614483496588,1.97441729278565,390.164706581361));
#50698=CARTESIAN_POINT('Ctrl Pts',(5.06928604606176,-0.504419409054961,
390.085578705901));
#50699=CARTESIAN_POINT('Ctrl Pts',(4.21498465890399,-2.86111941069082,390.006450830441));
#50700=CARTESIAN_POINT('Ctrl Pts',(2.34009542676882,-4.52504733131526,389.927322954981));
#50701=CARTESIAN_POINT('Ctrl Pts',(-0.101408666846889,-5.09331093094817,
389.848195079522));
#50702=CARTESIAN_POINT('Ctrl Pts',(-2.51835835252648,-4.42831470937736,
389.769067204062));
#50703=CARTESIAN_POINT('Ctrl Pts',(-4.3255297989291,-2.6910763488991,389.689939328602));
#50704=CARTESIAN_POINT('Ctrl Pts',(-5.08534674866728,-0.302238983003182,
389.610811453142));
#50705=CARTESIAN_POINT('Ctrl Pts',(-4.61383227037253,2.15978048372904,389.531683577683));
#50706=CARTESIAN_POINT('Ctrl Pts',(-3.02515568711978,4.09884532834732,389.452555702223));
#50707=CARTESIAN_POINT('Ctrl Pts',(-0.703988389596766,5.04544351909133,
389.373427826763));
#50708=CARTESIAN_POINT('Ctrl Pts',(1.78763788976615,4.7703721796208,389.294299951303));
#50709=CARTESIAN_POINT('Ctrl Pts',(3.84641763488075,3.34023522152349,389.215172075843));
#50710=CARTESIAN_POINT('Ctrl Pts',(4.97385185858917,1.10131632414888,389.136044200384));
#50711=CARTESIAN_POINT('Ctrl Pts',(4.89695127199855,-1.40426785076764,389.056916324924));
#50712=CARTESIAN_POINT('Ctrl Pts',(3.63433606243988,-3.56983211681959,388.977788449464));
#50713=CARTESIAN_POINT('Ctrl Pts',(1.4917273273879,-4.87102140600428,388.898660574004));
#50714=CARTESIAN_POINT('Ctrl Pts',(-1.0120781619955,-4.99277455439754,388.819532698545));
#50715=CARTESIAN_POINT('Ctrl Pts',(-3.27082589817505,-3.9056110790573,388.740404823085));
#50716=CARTESIAN_POINT('Ctrl Pts',(-4.73759799865136,-1.87276938254615,
388.661276947625));
#50717=CARTESIAN_POINT('Ctrl Pts',(-5.05724019876165,0.613532011436209,
388.582149072166));
#50718=CARTESIAN_POINT('Ctrl Pts',(-4.15235650051922,2.95127691849197,388.503021196705));
#50719=CARTESIAN_POINT('Ctrl Pts',(-2.24204931550549,4.57441961606814,388.423893321246));
#50720=CARTESIAN_POINT('Ctrl Pts',(0.211132509493252,5.0899433219303,388.344765445786));
#50721=CARTESIAN_POINT('Ctrl Pts',(2.613192138255,4.37302261663371,388.265637570326));
#50722=CARTESIAN_POINT('Ctrl Pts',(4.3825111169981,2.59724782537512,388.186509694867));
#50723=CARTESIAN_POINT('Ctrl Pts',(5.09067852854909,0.192593032057139,388.107381819407));
#50724=CARTESIAN_POINT('Ctrl Pts',(4.56622351098889,-2.25869493396522,388.028253943947));
#50725=CARTESIAN_POINT('Ctrl Pts',(2.93613405110136,-4.16307780265885,387.949126068487));
#50726=CARTESIAN_POINT('Ctrl Pts',(0.595108973109503,-5.05944120107668,
387.869998193027));
#50727=CARTESIAN_POINT('Ctrl Pts',(-1.89001176205386,-4.73074576534459,
387.790870317568));
#50728=CARTESIAN_POINT('Ctrl Pts',(-3.91749784672291,-3.2565795826218,387.711742442108));
#50729=CARTESIAN_POINT('Ctrl Pts',(-4.99642752878567,-0.993887270579772,
387.632614566648));
#50730=CARTESIAN_POINT('Ctrl Pts',(-4.86555608063145,1.50945817539208,387.553486691188));
#50731=CARTESIAN_POINT('Ctrl Pts',(-3.55657182856503,3.6473136395552,387.474358815728));
#50732=CARTESIAN_POINT('Ctrl Pts',(-1.38642335604174,4.90203327557553,387.395230940269));
#50733=CARTESIAN_POINT('Ctrl Pts',(1.11942428022107,4.96980776669272,387.316103064809));
#50734=CARTESIAN_POINT('Ctrl Pts',(3.35422210107046,3.83422665653951,387.236975189349));
#50735=CARTESIAN_POINT('Ctrl Pts',(4.77685129433647,1.77025186592861,387.157847313889));
#50736=CARTESIAN_POINT('Ctrl Pts',(5.04284606000954,-0.72235972484213,387.07871943843));
#50737=CARTESIAN_POINT('Ctrl Pts',(4.08780022662232,-3.04006402305186,386.99959156297));
#50738=CARTESIAN_POINT('Ctrl Pts',(2.14296212550442,-4.62166780347541,386.92046368751));
#50739=CARTESIAN_POINT('Ctrl Pts',(-0.320758314346703,-5.08421223601112,
386.84133581205));
#50740=CARTESIAN_POINT('Ctrl Pts',(-2.70681250786736,-4.31569994372646,
386.76220793659));
#50741=CARTESIAN_POINT('Ctrl Pts',(-4.43745744898977,-2.50221328935662,
386.683080061131));
#50742=CARTESIAN_POINT('Ctrl Pts',(-5.09364649014193,-0.082857651985011,
386.603952185671));
#50743=CARTESIAN_POINT('Ctrl Pts',(-4.51649446005934,2.35656057619595,386.524824310211));
#50744=CARTESIAN_POINT('Ctrl Pts',(-2.84574904331825,4.22537718310224,386.445696434751));
#50745=CARTESIAN_POINT('Ctrl Pts',(-0.485953222246148,5.07108956959117,
386.366568559292));
#50746=CARTESIAN_POINT('Ctrl Pts',(1.99150802159427,4.68892266485099,386.287440683832));
#50747=CARTESIAN_POINT('Ctrl Pts',(3.98675899790251,3.17141177548282,386.208312808372));
#50748=CARTESIAN_POINT('Ctrl Pts',(5.01668314543611,0.885996712931309,386.129184932912));
#50749=CARTESIAN_POINT('Ctrl Pts',(4.83190160489097,-1.61394759446514,386.050057057452));
#50750=CARTESIAN_POINT('Ctrl Pts',(3.47715612730962,-3.72310155963289,385.970929181992));
#50751=CARTESIAN_POINT('Ctrl Pts',(1.28047560943712,-4.93076892286227,385.891801306533));
#50752=CARTESIAN_POINT('Ctrl Pts',(-1.22625060220108,-4.94453328612815,
385.812673431073));
#50753=CARTESIAN_POINT('Ctrl Pts',(-3.43606079615961,-3.76106183970999,
385.733545555613));
#50754=CARTESIAN_POINT('Ctrl Pts',(-4.81388649504862,-1.66691234617067,
385.654417680153));
#50755=CARTESIAN_POINT('Ctrl Pts',(-5.02611031361548,0.830852015942555,
385.575289804694));
#50756=CARTESIAN_POINT('Ctrl Pts',(-4.02134581343353,3.12743949674625,385.496161929234));
#50757=CARTESIAN_POINT('Ctrl Pts',(-2.04287986715703,4.66676995419661,385.417034053774));
#50758=CARTESIAN_POINT('Ctrl Pts',(0.430235177489289,5.07612033437727,385.337906178314));
#50759=CARTESIAN_POINT('Ctrl Pts',(2.79917598944896,4.25637330800767,385.258778302855));
#50760=CARTESIAN_POINT('Ctrl Pts',(4.49034328098805,2.40601686941577,385.179650427394));
#50761=CARTESIAN_POINT('Ctrl Pts',(5.09424925529516,-0.0269162024146704,
385.100522551935));
#50762=CARTESIAN_POINT('Ctrl Pts',(4.46466820889472,-2.45333196724627,385.021394676475));
#50763=CARTESIAN_POINT('Ctrl Pts',(2.75404263336906,-4.28571454142868,384.942266801016));
#50764=CARTESIAN_POINT('Ctrl Pts',(0.376571822658881,-5.08038321580243,
384.863138925555));
#50765=CARTESIAN_POINT('Ctrl Pts',(-2.09207953936242,-4.64492229838228,
384.784011050096));
#50766=CARTESIAN_POINT('Ctrl Pts',(-4.05416892752487,-3.08477134713736,
384.704883174636));
#50767=CARTESIAN_POINT('Ctrl Pts',(-5.03460930299721,-0.777694749372607,
384.625755299176));
#50768=CARTESIAN_POINT('Ctrl Pts',(-4.79600347197984,1.71768758911072,384.546627423717));
#50769=CARTESIAN_POINT('Ctrl Pts',(-3.39612583475742,3.79716068550186,384.467499548257));
#50770=CARTESIAN_POINT('Ctrl Pts',(-1.17393328361345,4.9572150046828,384.388371672797));
#50771=CARTESIAN_POINT('Ctrl Pts',(1.33250752393625,4.91696284871881,384.309243797337));
#50772=CARTESIAN_POINT('Ctrl Pts',(3.51630398225976,3.6861506021013,384.230115921877));
#50773=CARTESIAN_POINT('Ctrl Pts',(4.84868640377085,1.56279880820132,384.150988046418));
#50774=CARTESIAN_POINT('Ctrl Pts',(5.00704073069747,-0.938958507157973,
384.071860170958));
#50775=CARTESIAN_POINT('Ctrl Pts',(3.95302411855986,-3.213362767431,383.992732295498));
#50776=CARTESIAN_POINT('Ctrl Pts',(1.94184901290741,-4.70970512538717,383.913604420038));
#50777=CARTESIAN_POINT('Ctrl Pts',(-0.539512264162803,-5.06567137444245,
383.834476544579));
#50778=CARTESIAN_POINT('Ctrl Pts',(-2.89023969471176,-4.19507025735449,
383.755348669118));
#50779=CARTESIAN_POINT('Ctrl Pts',(-4.54114405585455,-2.30870323363671,
383.676220793659));
#50780=CARTESIAN_POINT('Ctrl Pts',(-5.0924865441193,0.136677558478088,383.597092918199));
#50781=CARTESIAN_POINT('Ctrl Pts',(-4.41076882262505,2.54896417204843,383.51796504274));
#50782=CARTESIAN_POINT('Ctrl Pts',(-2.66105740443557,4.34406186043965,383.43883716728));
#50783=CARTESIAN_POINT('Ctrl Pts',(-0.267015564777766,5.08731782427579,
383.35970929182));
#50784=CARTESIAN_POINT('Ctrl Pts',(2.19167961573057,4.59876509717759,383.28058141636));
#50785=CARTESIAN_POINT('Ctrl Pts',(4.11969633429617,2.99669852841663,383.201453540901));
#50786=CARTESIAN_POINT('Ctrl Pts',(5.05019767759256,0.669031669105843,383.12232566544));
#50787=CARTESIAN_POINT('Ctrl Pts',(4.75787835092606,-1.8206299884427,383.043197789981));
#50788=CARTESIAN_POINT('Ctrl Pts',(3.31351857671521,-3.8694566283641,382.964069914521));
#50789=CARTESIAN_POINT('Ctrl Pts',(1.06684585069835,-4.98135924099793,382.884942039061));
#50790=CARTESIAN_POINT('Ctrl Pts',(-1.43814570582419,-4.88710925658996,
382.805814163602));
#50791=CARTESIAN_POINT('Ctrl Pts',(-3.59491439905111,-3.60952772818311,
382.726686288142));
#50792=CARTESIAN_POINT('Ctrl Pts',(-4.8812348614273,-1.45795959635872,382.647558412682));
#50793=CARTESIAN_POINT('Ctrl Pts',(-4.98564616607288,1.04662900005231,382.568430537222));
#50794=CARTESIAN_POINT('Ctrl Pts',(-3.88286686666645,3.29779393728166,382.489302661762));
#50795=CARTESIAN_POINT('Ctrl Pts',(-1.83991647567274,4.75045338042336,382.410174786303));
#50796=CARTESIAN_POINT('Ctrl Pts',(0.648538832374088,5.05287020810257,382.331046910843));
#50797=CARTESIAN_POINT('Ctrl Pts',(2.97996133890915,4.13181925737738,382.251919035383));
#50798=CARTESIAN_POINT('Ctrl Pts',(4.58983618463159,2.21031756887428,382.172791159923));
#50799=CARTESIAN_POINT('Ctrl Pts',(5.08835917511605,-0.246375449345246,
382.093663284464));
#50800=CARTESIAN_POINT('Ctrl Pts',(4.35482132902486,-2.64341278450753,382.014535409004));
#50801=CARTESIAN_POINT('Ctrl Pts',(2.56683653350947,-4.40039204699635,381.935407533544));
#50802=CARTESIAN_POINT('Ctrl Pts',(0.157335320227334,-5.09189017497793,
381.856279658084));
#50803=CARTESIAN_POINT('Ctrl Pts',(-2.29026200215225,-4.55047249398623,
381.777151782624));
#50804=CARTESIAN_POINT('Ctrl Pts',(-4.1833107910579,-2.90723421527166,381.698023907165));
#50805=CARTESIAN_POINT('Ctrl Pts',(-5.06344103087761,-0.560057929015174,
381.618896031705));
#50806=CARTESIAN_POINT('Ctrl Pts',(-4.71754394484289,1.92272699193202,381.539768156245));
#50807=CARTESIAN_POINT('Ctrl Pts',(-3.22937271124211,3.9399558181422,381.460640280785));
#50808=CARTESIAN_POINT('Ctrl Pts',(-0.959263035935946,5.0031904206131,381.381512405325));
#50809=CARTESIAN_POINT('Ctrl Pts',(1.54311609556955,4.85498637203256,381.302384529866));
#50810=CARTESIAN_POINT('Ctrl Pts',(3.67185554437766,3.53122879721078,381.223256654406));
#50811=CARTESIAN_POINT('Ctrl Pts',(4.91151675438643,1.35244339194259,381.144128778947));
#50812=CARTESIAN_POINT('Ctrl Pts',(4.96193655414693,-1.15381349864191,381.065000903486));
#50813=CARTESIAN_POINT('Ctrl Pts',(3.81090663474561,-3.38069380131942,380.985873028027));
#50814=CARTESIAN_POINT('Ctrl Pts',(1.73712958706021,-4.78899579815935,380.906745152567));
#50815=CARTESIAN_POINT('Ctrl Pts',(-0.757264256456047,-5.03772277948299,
380.827617277107));
#50816=CARTESIAN_POINT('Ctrl Pts',(-3.06829926047039,-4.0666496782025,380.748489401647));
#50817=CARTESIAN_POINT('Ctrl Pts',(-4.63639705749532,-2.11090555977201,
380.669361526187));
#50818=CARTESIAN_POINT('Ctrl Pts',(-5.08186906479814,0.355958937625331,
380.590233650728));
#50819=CARTESIAN_POINT('Ctrl Pts',(-4.29685170689215,2.73663394812055,380.511105775268));
#50820=CARTESIAN_POINT('Ctrl Pts',(-2.47142377134362,4.45467894460033,380.431977899808));
#50821=CARTESIAN_POINT('Ctrl Pts',(-0.0475820182042561,5.09409814477217,
380.352850024348));
#50822=CARTESIAN_POINT('Ctrl Pts',(2.38778092263769,4.50006691311533,380.273722148889));
#50823=CARTESIAN_POINT('Ctrl Pts',(4.24498275891546,2.81641994978345,380.194594273428));
#50824=CARTESIAN_POINT('Ctrl Pts',(5.07433321340091,0.450824130237162,380.115466397969));
#50825=CARTESIAN_POINT('Ctrl Pts',(4.67501898270842,-2.02393119160303,380.036338522509));
#50826=CARTESIAN_POINT('Ctrl Pts',(3.14372731083789,-4.00862551906755,379.957210647049));
#50827=CARTESIAN_POINT('Ctrl Pts',(0.851234794597309,-5.02269840638422,
379.87808277159));
#50828=CARTESIAN_POINT('Ctrl Pts',(-1.64736995096127,-4.82060911106652,
379.79895489613));
#50829=CARTESIAN_POINT('Ctrl Pts',(-3.74709169119734,-3.45129016670399,
379.71982702067));
#50830=CARTESIAN_POINT('Ctrl Pts',(-4.93951802147898,-1.2462991906088,379.64069914521));
#50831=CARTESIAN_POINT('Ctrl Pts',(-4.93592290429957,1.26046223261093,379.56157126975));
#50832=CARTESIAN_POINT('Ctrl Pts',(-3.73717683698987,3.46202386561592,379.482443394291));
#50833=CARTESIAN_POINT('Ctrl Pts',(-1.63353607538846,4.82531448171332,379.403315518831));
#50834=CARTESIAN_POINT('Ctrl Pts',(0.865638050575662,5.02023612217824,379.324187643371));
#50835=CARTESIAN_POINT('Ctrl Pts',(3.15521244034589,3.99959178083392,379.245059767911));
#50836=CARTESIAN_POINT('Ctrl Pts',(4.6808050542546,2.01051336754875,379.165931892452));
#50837=CARTESIAN_POINT('Ctrl Pts',(5.07301922679952,-0.465377139049836,
379.086804016992));
#50838=CARTESIAN_POINT('Ctrl Pts',(4.23688687398491,-2.82858437634132,379.007676141532));
#50839=CARTESIAN_POINT('Ctrl Pts',(2.37486342213654,-4.5068973455389,378.928548266072));
#50840=CARTESIAN_POINT('Ctrl Pts',(-0.0621933781710937,-5.0939407084044,
378.849420390613));
#50841=CARTESIAN_POINT('Ctrl Pts',(-2.48419109500962,-4.44757176001722,
378.770292515152));
#50842=CARTESIAN_POINT('Ctrl Pts',(-4.30468360095437,-2.72429790087321,
378.691164639693));
#50843=CARTESIAN_POINT('Ctrl Pts',(-5.08286916745938,-0.341380994664952,
378.612036764233));
#50844=CARTESIAN_POINT('Ctrl Pts',(-4.63032321066906,2.12419559404662,378.532908888774));
#50845=CARTESIAN_POINT('Ctrl Pts',(-3.05662214430013,4.07543384488105,378.453781013314));
#50846=CARTESIAN_POINT('Ctrl Pts',(-0.742811288783636,5.03987413992486,
378.374653137854));
#50847=CARTESIAN_POINT('Ctrl Pts',(1.75085886250587,4.78399343651434,378.295525262394));
#50848=CARTESIAN_POINT('Ctrl Pts',(3.82058790417125,3.36974895556452,378.216397386935));
#50849=CARTESIAN_POINT('Ctrl Pts',(4.9652256605272,1.13957627961887,378.137269511474));
#50850=CARTESIAN_POINT('Ctrl Pts',(4.90761729577347,-1.36652568042196,378.058141636015));
#50851=CARTESIAN_POINT('Ctrl Pts',(3.66171170927622,-3.54174636516749,377.979013760555));
#50852=CARTESIAN_POINT('Ctrl Pts',(1.52918404352555,-4.85939256677772,377.899885885095));
#50853=CARTESIAN_POINT('Ctrl Pts',(-0.973609892176757,-5.00041835598616,
377.820758009635));
#50854=CARTESIAN_POINT('Ctrl Pts',(-3.24066052105438,-3.93067670310182,
377.741630134176));
#50855=CARTESIAN_POINT('Ctrl Pts',(-4.72303955439021,-1.90918760856372,
377.662502258716));
#50856=CARTESIAN_POINT('Ctrl Pts',(-5.06181377047586,0.574579246099912,
377.583374383256));
#50857=CARTESIAN_POINT('Ctrl Pts',(-4.17495467452228,2.91922137268011,377.504246507796));
#50858=CARTESIAN_POINT('Ctrl Pts',(-2.27720032296007,4.55702300259043,377.425118632336));
#50859=CARTESIAN_POINT('Ctrl Pts',(0.171939895519064,5.09141793897891,377.345990756877));
#50860=CARTESIAN_POINT('Ctrl Pts',(2.5794477519296,4.39301141042152,377.266862881417));
#50861=CARTESIAN_POINT('Ctrl Pts',(4.36238559553759,2.63091084472138,377.187735005957));
#50862=CARTESIAN_POINT('Ctrl Pts',(5.08904492944719,0.231779341395482,377.108607130498));
#50863=CARTESIAN_POINT('Ctrl Pts',(4.58347738286989,-2.22347364224237,377.029479255037));
#50864=CARTESIAN_POINT('Ctrl Pts',(2.96809765825856,-4.14034977363789,376.950351379578));
#50865=CARTESIAN_POINT('Ctrl Pts',(0.634042864132613,-5.0547096458148,376.871223504118));
#50866=CARTESIAN_POINT('Ctrl Pts',(-1.85353477590152,-4.7451563505839,376.792095628658));
#50867=CARTESIAN_POINT('Ctrl Pts',(-3.89231005589385,-3.28664302685179,
376.712967753199));
#50868=CARTESIAN_POINT('Ctrl Pts',(-4.98862773436458,-1.03232421493045,
376.633839877739));
#50869=CARTESIAN_POINT('Ctrl Pts',(-4.87703287210239,1.47195459226046,376.554712002279));
#50870=CARTESIAN_POINT('Ctrl Pts',(-3.58454629319045,3.61982428153675,376.475584126819));
#50871=CARTESIAN_POINT('Ctrl Pts',(-1.42412194671949,4.89121422922617,376.39645625136));
#50872=CARTESIAN_POINT('Ctrl Pts',(1.08112964569973,4.97827868361118,376.3173283759));
#50873=CARTESIAN_POINT('Ctrl Pts',(3.32460382467506,3.85993644420179,376.23820050044));
#50874=CARTESIAN_POINT('Ctrl Pts',(4.76308094821025,1.80697533479263,376.15907262498));
#50875=CARTESIAN_POINT('Ctrl Pts',(5.04825789565173,-0.683514556087066,
376.07994474952));
#50876=CARTESIAN_POINT('Ctrl Pts',(4.11108387333318,-3.00850284103068,376.000816874061));
#50877=CARTESIAN_POINT('Ctrl Pts',(2.1784798079633,-4.60503266038196,375.921688998601));
#50878=CARTESIAN_POINT('Ctrl Pts',(-0.281606542178375,-5.08653096539461,
375.842561123141));
#50879=CARTESIAN_POINT('Ctrl Pts',(-2.67350672874489,-4.33641128901115,
375.763433247681));
#50880=CARTESIAN_POINT('Ctrl Pts',(-4.41806180727835,-2.5363019544723,375.684305372222));
#50881=CARTESIAN_POINT('Ctrl Pts',(-5.09285793196053,-0.12207046608611,
375.605177496761));
#50882=CARTESIAN_POINT('Ctrl Pts',(-4.53450261646048,2.32172008989041,375.526049621302));
#50883=CARTESIAN_POINT('Ctrl Pts',(-2.8781963029061,4.20334135813296,375.446921745842));
#50884=CARTESIAN_POINT('Ctrl Pts',(-0.524977181972811,5.06720185538771,
375.367793870382));
#50885=CARTESIAN_POINT('Ctrl Pts',(1.95534399133764,4.70410782389334,375.288665994923));
#50886=CARTESIAN_POINT('Ctrl Pts',(3.96223755849503,3.20202817970643,375.209538119463));
#50887=CARTESIAN_POINT('Ctrl Pts',(5.00968625615773,0.924557438714191,375.130410244003));
#50888=CARTESIAN_POINT('Ctrl Pts',(4.84423973083701,-1.5766172667089,375.051282368543));
#50889=CARTESIAN_POINT('Ctrl Pts',(3.50558626093324,-3.69634481139898,374.972154493084));
#50890=CARTESIAN_POINT('Ctrl Pts',(2.04760230627713,-4.51212292509998,374.91940257611));
#50891=CARTESIAN_POINT('Ctrl Pts',(1.26508527942809,-4.72177922709072,374.893026617624));
#50892=CARTESIAN_POINT('Ctrl Pts',(3.8562705385027,3.2970584607914,400.320920147129));
#50893=CARTESIAN_POINT('Ctrl Pts',(4.40267566673985,2.65797789150057,400.294544188642));
#50894=CARTESIAN_POINT('Ctrl Pts',(5.17098558200965,1.10346405572081,400.241792271669));
#50895=CARTESIAN_POINT('Ctrl Pts',(5.07118954877308,-1.49668420940778,400.162664396209));
#50896=CARTESIAN_POINT('Ctrl Pts',(3.74345010496737,-3.73402503008569,400.08353652075));
#50897=CARTESIAN_POINT('Ctrl Pts',(1.50930126812034,-5.0674413388845,400.00440864529));
#50898=CARTESIAN_POINT('Ctrl Pts',(-1.09030376370591,-5.17376607298461,
399.925280769831));
#50899=CARTESIAN_POINT('Ctrl Pts',(-3.42590833126468,-4.02739560525483,
399.84615289437));
#50900=CARTESIAN_POINT('Ctrl Pts',(-4.93198749421962,-1.90583738162352,
399.767025018911));
#50901=CARTESIAN_POINT('Ctrl Pts',(-5.24386820862784,0.677177256470671,
399.68789714345));
#50902=CARTESIAN_POINT('Ctrl Pts',(-4.28603436807985,3.09622957226831,399.608769267991));
#50903=CARTESIAN_POINT('Ctrl Pts',(-2.29040909926245,4.7655795591539,399.529641392531));
#50904=CARTESIAN_POINT('Ctrl Pts',(0.259800278618912,5.28102545063066,399.450513517072));
#50905=CARTESIAN_POINT('Ctrl Pts',(2.7471033957984,4.51775909222651,399.371385641611));
#50906=CARTESIAN_POINT('Ctrl Pts',(4.56924148852249,2.66059337678593,399.292257766152));
#50907=CARTESIAN_POINT('Ctrl Pts',(5.2850143906551,0.159209483399153,399.213129890692));
#50908=CARTESIAN_POINT('Ctrl Pts',(4.7211096918349,-2.38072426286758,399.134002015232));
#50909=CARTESIAN_POINT('Ctrl Pts',(3.01406746059458,-4.34420558161996,399.054874139772));
#50910=CARTESIAN_POINT('Ctrl Pts',(0.577219342712345,-5.25581036421826,
398.975746264313));
#50911=CARTESIAN_POINT('Ctrl Pts',(-1.99939275815206,-4.89480881878609,
398.896618388853));
#50912=CARTESIAN_POINT('Ctrl Pts',(-4.09188543486623,-3.34861140683646,
398.817490513394));
#50913=CARTESIAN_POINT('Ctrl Pts',(-5.19359667913832,-0.991603904073038,
398.738362637933));
#50914=CARTESIAN_POINT('Ctrl Pts',(-5.03776559021372,1.60550385431017,398.659234762474));
#50915=CARTESIAN_POINT('Ctrl Pts',(-3.66212405277363,3.81386578025083,398.580106887014));
#50916=CARTESIAN_POINT('Ctrl Pts',(-1.39976059402284,5.09876407058445,398.500979011554));
#50917=CARTESIAN_POINT('Ctrl Pts',(1.2015314169661,5.14908215334412,398.421851136094));
#50918=CARTESIAN_POINT('Ctrl Pts',(3.51189274640949,3.9526363487746,398.342723260634));
#50919=CARTESIAN_POINT('Ctrl Pts',(4.97190814582059,1.79912594262636,398.263595385175));
#50920=CARTESIAN_POINT('Ctrl Pts',(5.22805937238099,-0.790012637095727,
398.184467509715));
#50921=CARTESIAN_POINT('Ctrl Pts',(4.21832370253235,-3.18786290617544,398.105339634255));
#50922=CARTESIAN_POINT('Ctrl Pts',(2.18719169429123,-4.81382563667766,398.026211758795));
#50923=CARTESIAN_POINT('Ctrl Pts',(-0.37353210098369,-5.27420122269227,
397.947083883336));
#50924=CARTESIAN_POINT('Ctrl Pts',(-2.84381136257153,-4.45751743709679,
397.867956007876));
#50925=CARTESIAN_POINT('Ctrl Pts',(-4.62550939672404,-2.56152056184034,
397.788828132416));
#50926=CARTESIAN_POINT('Ctrl Pts',(-5.2872179056115,-0.0452944422017613,
397.709700256956));
#50927=CARTESIAN_POINT('Ctrl Pts',(-4.66871527142514,2.48189896697567,397.630572381496));
#50928=CARTESIAN_POINT('Ctrl Pts',(-2.91976153402742,4.40814216562114,397.551444506037));
#50929=CARTESIAN_POINT('Ctrl Pts',(-0.463836508948714,5.26702766851281,
397.472316630577));
#50930=CARTESIAN_POINT('Ctrl Pts',(2.10439874769627,4.85059075563045,397.393188755117));
#50931=CARTESIAN_POINT('Ctrl Pts',(4.16308914079174,3.25966464129901,397.314060879657));
#50932=CARTESIAN_POINT('Ctrl Pts',(5.21375731827273,0.87946540242969,397.234933004198));
#50933=CARTESIAN_POINT('Ctrl Pts',(5.00200160188481,-1.71368163398425,397.155805128738));
#50934=CARTESIAN_POINT('Ctrl Pts',(3.57909508696266,-3.89188940315535,397.076677253278));
#50935=CARTESIAN_POINT('Ctrl Pts',(1.28957072230382,-5.12774142484681,396.997549377819));
#50936=CARTESIAN_POINT('Ctrl Pts',(-1.31220156516579,-5.12199685867627,
396.918421502358));
#50937=CARTESIAN_POINT('Ctrl Pts',(-3.59624625077107,-3.87604665499891,
396.839293626899));
#50938=CARTESIAN_POINT('Ctrl Pts',(-5.00952021996834,-1.69157675960673,
396.760165751439));
#50939=CARTESIAN_POINT('Ctrl Pts',(-5.20982288335836,0.90248007842212,396.681037875979));
#50940=CARTESIAN_POINT('Ctrl Pts',(-4.14865431030898,3.27801650109757,396.601910000519));
#50941=CARTESIAN_POINT('Ctrl Pts',(-2.08295867375766,4.85983620416686,396.52278212506));
#50942=CARTESIAN_POINT('Ctrl Pts',(0.487090472013812,5.26492807548086,396.4436542496));
#50943=CARTESIAN_POINT('Ctrl Pts',(2.93919882905869,4.3952059122609,396.36452637414));
#50944=CARTESIAN_POINT('Ctrl Pts',(4.67962948341671,2.46125835008237,396.28539849868));
#50945=CARTESIAN_POINT('Ctrl Pts',(5.2869663411736,-0.0686416434144708,
396.206270623221));
#50946=CARTESIAN_POINT('Ctrl Pts',(4.61415296796628,-2.58192121415839,396.127142747761));
#50947=CARTESIAN_POINT('Ctrl Pts',(2.82409983825713,-4.47003186470401,396.048014872301));
#50948=CARTESIAN_POINT('Ctrl Pts',(0.350238296140284,-5.27579926682488,
395.968886996841));
#50949=CARTESIAN_POINT('Ctrl Pts',(-2.20842757548492,-4.80412035775031,
395.889759121382));
#50950=CARTESIAN_POINT('Ctrl Pts',(-4.23235974759556,-3.16920427471092,
395.810631245921));
#50951=CARTESIAN_POINT('Ctrl Pts',(-5.23149698840249,-0.766918527777797,
395.731503370462));
#50952=CARTESIAN_POINT('Ctrl Pts',(-4.96391497173342,1.82106367854447,395.652375495002));
#50953=CARTESIAN_POINT('Ctrl Pts',(-3.49440419526435,3.96810585645496,395.573247619542));
#50954=CARTESIAN_POINT('Ctrl Pts',(-1.17878204811896,5.1543377509575,395.494119744082));
#50955=CARTESIAN_POINT('Ctrl Pts',(1.42226240243777,5.09253320328156,395.414991868623));
#50956=CARTESIAN_POINT('Ctrl Pts',(3.67892986523249,3.79765714811298,395.335863993163));
#50957=CARTESIAN_POINT('Ctrl Pts',(5.0448061610774,1.58324210563915,395.256736117703));
#50958=CARTESIAN_POINT('Ctrl Pts',(5.18916725226161,-1.01452845991075,395.177608242243));
#50959=CARTESIAN_POINT('Ctrl Pts',(4.07705852165763,-3.36664797371096,395.098480366784));
#50960=CARTESIAN_POINT('Ctrl Pts',(1.97775844702931,-4.90359014326416,395.019352491324));
#50961=CARTESIAN_POINT('Ctrl Pts',(-0.60042266624658,-5.25321019851391,
394.940224615864));
#50962=CARTESIAN_POINT('Ctrl Pts',(-3.03322150067462,-4.33085350661488,
394.861096740404));
#50963=CARTESIAN_POINT('Ctrl Pts',(-4.73157661935314,-2.35985327152006,
394.781968864945));
#50964=CARTESIAN_POINT('Ctrl Pts',(-5.28425981367717,0.182545855799866,
394.702840989484));
#50965=CARTESIAN_POINT('Ctrl Pts',(-4.55744811727866,2.68074456564335,394.623713114025));
#50966=CARTESIAN_POINT('Ctrl Pts',(-2.72712679296628,4.52984593810856,394.544585238565));
#50967=CARTESIAN_POINT('Ctrl Pts',(-0.236477452813074,5.28212108742541,
394.465457363106));
#50968=CARTESIAN_POINT('Ctrl Pts',(2.31143093653793,4.75541920271268,394.386329487645));
#50969=CARTESIAN_POINT('Ctrl Pts',(4.29966508998112,3.07727231195273,394.307201612186));
#50970=CARTESIAN_POINT('Ctrl Pts',(5.2468074522505,0.654015540275394,394.228073736726));
#50971=CARTESIAN_POINT('Ctrl Pts',(4.92352338499734,-1.92760012588128,394.148945861266));
#50972=CARTESIAN_POINT('Ctrl Pts',(3.40809070325859,-4.04247974964323,394.069817985806));
#50973=CARTESIAN_POINT('Ctrl Pts',(1.06744601535546,-5.17854069909805,393.990690110347));
#50974=CARTESIAN_POINT('Ctrl Pts',(-1.53166282285958,-5.06070486839363,
393.911562234887));
#50975=CARTESIAN_POINT('Ctrl Pts',(-3.75990519627929,-3.71750422769163,
393.832434359427));
#50976=CARTESIAN_POINT('Ctrl Pts',(-5.07774958438631,-1.47417228510708,
393.753306483967));
#50977=CARTESIAN_POINT('Ctrl Pts',(-5.16610207037776,1.12610575273896,393.674178608508));
#50978=CARTESIAN_POINT('Ctrl Pts',(-4.00356958154437,3.45371616865744,393.595050733048));
#50979=CARTESIAN_POINT('Ctrl Pts',(-1.8716398630404,4.94506713715712,393.515922857588));
#50980=CARTESIAN_POINT('Ctrl Pts',(0.713476058729831,5.23905303289941,393.436794982128));
#50981=CARTESIAN_POINT('Ctrl Pts',(3.12583571869877,4.26449010171441,393.357667106669));
#50982=CARTESIAN_POINT('Ctrl Pts',(4.78132668327137,2.25735241283907,393.278539231209));
#50983=CARTESIAN_POINT('Ctrl Pts',(5.2790995798779,-0.296365304389928,393.199411355749));
#50984=CARTESIAN_POINT('Ctrl Pts',(4.49862704983328,-2.77832313355043,393.120283480289));
#50985=CARTESIAN_POINT('Ctrl Pts',(2.62888742685924,-4.58755661161959,393.041155604829));
#50986=CARTESIAN_POINT('Ctrl Pts',(0.122606802959192,-5.28599019482455,
392.96202772937));
#50987=CARTESIAN_POINT('Ctrl Pts',(-2.41336100201929,-4.70450990453263,
392.88289985391));
#50988=CARTESIAN_POINT('Ctrl Pts',(-4.3649739152189,-2.98391144093985,392.80377197845));
#50989=CARTESIAN_POINT('Ctrl Pts',(-5.25968160051806,-0.540808865575483,
392.724644102991));
#50990=CARTESIAN_POINT('Ctrl Pts',(-4.88084559720602,2.03324150659673,392.64551622753));
#50991=CARTESIAN_POINT('Ctrl Pts',(-3.32019468996614,4.11497654776232,392.566388352071));
#50992=CARTESIAN_POINT('Ctrl Pts',(-0.955614322062658,5.20033903081154,
392.487260476611));
#50993=CARTESIAN_POINT('Ctrl Pts',(1.64035202716895,5.02652663326038,392.408132601151));
#50994=CARTESIAN_POINT('Ctrl Pts',(3.83913464362559,3.63562511214056,392.329004725691));
#50995=CARTESIAN_POINT('Ctrl Pts',(5.10833519286426,1.36441794376124,392.249876850232));
#50996=CARTESIAN_POINT('Ctrl Pts',(5.14063804785052,-1.23716014683014,392.170748974772));
#50997=CARTESIAN_POINT('Ctrl Pts',(3.92822161400576,-3.53918065647562,392.091621099312));
#50998=CARTESIAN_POINT('Ctrl Pts',(1.76465219715718,-4.98424792631562,392.012493223852));
#50999=CARTESIAN_POINT('Ctrl Pts',(-0.826198153971171,-5.22246315241074,
391.933365348392));
#51000=CARTESIAN_POINT('Ctrl Pts',(-3.21699847841567,-4.19614651290735,
391.854237472933));
#51001=CARTESIAN_POINT('Ctrl Pts',(-4.82885657410346,-2.15380336954211,
391.775109597473));
#51002=CARTESIAN_POINT('Ctrl Pts',(-5.27148803589155,0.41004713797985,391.695981722013));
#51003=CARTESIAN_POINT('Ctrl Pts',(-4.43771707875037,2.8746116080056,391.616853846554));
#51004=CARTESIAN_POINT('Ctrl Pts',(-2.52942735664669,4.64313708771996,391.537725971094));
#51005=CARTESIAN_POINT('Ctrl Pts',(-0.00867922155838994,5.28740479243137,
391.458598095634));
#51006=CARTESIAN_POINT('Ctrl Pts',(2.51417044146968,4.65141610255989,391.379470220174));
#51007=CARTESIAN_POINT('Ctrl Pts',(4.42825589764708,2.88916501309064,391.300342344714));
#51008=CARTESIAN_POINT('Ctrl Pts',(5.27011345519119,0.427351070346123,391.221214469255));
#51009=CARTESIAN_POINT('Ctrl Pts',(4.8359014254693,-2.1379387669101,391.142086593795));
#51010=CARTESIAN_POINT('Ctrl Pts',(3.23075696923981,-4.18556258746916,391.062958718335));
#51011=CARTESIAN_POINT('Ctrl Pts',(0.843338896446427,-5.21972262420654,
390.983830842875));
#51012=CARTESIAN_POINT('Ctrl Pts',(-1.7482795463511,-4.99001436828829,390.904702967415));
#51013=CARTESIAN_POINT('Ctrl Pts',(-3.91658141767327,-3.55205782141137,
390.825575091956));
#51014=CARTESIAN_POINT('Ctrl Pts',(-5.13654878431394,-1.25403004520473,
390.746447216496));
#51015=CARTESIAN_POINT('Ctrl Pts',(-5.11278700870727,1.34764007491144,390.667319341036));
#51016=CARTESIAN_POINT('Ctrl Pts',(-3.85104960630393,3.62300175237324,390.588191465576));
#51017=CARTESIAN_POINT('Ctrl Pts',(-1.65684512829777,5.02111431743484,390.509063590116));
#51018=CARTESIAN_POINT('Ctrl Pts',(0.938536610313288,5.20344826043412,390.429935714657));
#51019=CARTESIAN_POINT('Ctrl Pts',(3.30666744908329,4.12585447502528,390.350807839197));
#51020=CARTESIAN_POINT('Ctrl Pts',(4.874144221702,2.04925422384882,390.271679963737));
#51021=CARTESIAN_POINT('Ctrl Pts',(5.26142871608132,-0.523538569265068,
390.192552088277));
#51022=CARTESIAN_POINT('Ctrl Pts',(4.37474648711696,-2.96956527817979,390.113424212818));
#51023=CARTESIAN_POINT('Ctrl Pts',(2.42879276586438,-4.69656155803349,390.034296337358));
#51024=CARTESIAN_POINT('Ctrl Pts',(-0.105252389973582,-5.28636422338813,
389.955168461898));
#51025=CARTESIAN_POINT('Ctrl Pts',(-2.61381244478399,-4.59616245050211,
389.876040586438));
#51026=CARTESIAN_POINT('Ctrl Pts',(-4.48948165275299,-2.79307702319636,
389.796912710979));
#51027=CARTESIAN_POINT('Ctrl Pts',(-5.27809817231664,-0.313694837861352,
389.717784835519));
#51028=CARTESIAN_POINT('Ctrl Pts',(-4.78871173927535,2.2416432914359,389.638656960059));
#51029=CARTESIAN_POINT('Ctrl Pts',(-3.13981907081257,4.25420509266713,389.559529084599));
#51030=CARTESIAN_POINT('Ctrl Pts',(-0.730671872756092,5.23668247865729,
389.48040120914));
#51031=CARTESIAN_POINT('Ctrl Pts',(1.85539526507438,4.95118502767294,389.401273333679));
#51032=CARTESIAN_POINT('Ctrl Pts',(3.99220955659535,3.46684115934693,389.32214545822));
#51033=CARTESIAN_POINT('Ctrl Pts',(5.16237725796638,1.14305984722794,389.24301758276));
#51034=CARTESIAN_POINT('Ctrl Pts',(5.08256188536855,-1.45749423645932,389.1638897073));
#51035=CARTESIAN_POINT('Ctrl Pts',(3.77208939268016,-3.70514053465492,389.08476183184));
#51036=CARTESIAN_POINT('Ctrl Pts',(1.54826871586373,-5.05564919188336,389.005633956381));
#51037=CARTESIAN_POINT('Ctrl Pts',(-1.05043926423896,-5.18201718639165,
388.926506080921));
#51038=CARTESIAN_POINT('Ctrl Pts',(-3.39480099358967,-4.05364662764723,
388.847378205461));
#51039=CARTESIAN_POINT('Ctrl Pts',(-4.91716859708847,-1.94375352236854,
388.768250330001));
#51040=CARTESIAN_POINT('Ctrl Pts',(-5.2489262914167,0.636786899353102,388.689122454542));
#51041=CARTESIAN_POINT('Ctrl Pts',(-4.30974451485365,3.06314005305047,388.609994579082));
#51042=CARTESIAN_POINT('Ctrl Pts',(-2.32703038342756,4.74780521530929,388.530866703622));
#51043=CARTESIAN_POINT('Ctrl Pts',(0.2191351283499,5.28286897087523,388.451738828163));
#51044=CARTESIAN_POINT('Ctrl Pts',(2.71224074394742,4.53877460497707,388.372610952702));
#51045=CARTESIAN_POINT('Ctrl Pts',(4.54862275081774,2.69569208899244,388.293483077243));
#51046=CARTESIAN_POINT('Ctrl Pts',(5.28363204425109,0.199892943537846,388.214355201783));
#51047=CARTESIAN_POINT('Ctrl Pts',(4.73929845080001,-2.34430692575821,388.135227326323));
#51048=CARTESIAN_POINT('Ctrl Pts',(3.04742322101362,-4.32087218972514,388.056099450863));
#51049=CARTESIAN_POINT('Ctrl Pts',(0.617665567076949,-5.25121071898288,
387.976971575404));
#51050=CARTESIAN_POINT('Ctrl Pts',(-1.96164944496022,-4.9100566415267,387.897843699944));
#51051=CARTESIAN_POINT('Ctrl Pts',(-4.06598394303424,-3.38001469566346,
387.818715824484));
#51052=CARTESIAN_POINT('Ctrl Pts',(-5.18580862056406,-1.03155887800781,
387.739587949024));
#51053=CARTESIAN_POINT('Ctrl Pts',(-5.04997671264308,1.56667162151986,387.660460073564));
#51054=CARTESIAN_POINT('Ctrl Pts',(-3.69137763771595,3.78555886279474,387.581332198105));
#51055=CARTESIAN_POINT('Ctrl Pts',(-1.43897337649567,5.08783651365194,387.502204322645));
#51056=CARTESIAN_POINT('Ctrl Pts',(1.16185415459233,5.15817988164137,387.423076447186));
#51057=CARTESIAN_POINT('Ctrl Pts',(3.48135818778607,3.97955649994419,387.343948571725));
#51058=CARTESIAN_POINT('Ctrl Pts',(4.95790972221771,1.83735025355874,387.264820696266));
#51059=CARTESIAN_POINT('Ctrl Pts',(5.23398656730458,-0.749739542233496,
387.185692820806));
#51060=CARTESIAN_POINT('Ctrl Pts',(4.24274134513742,-3.15529248187465,387.106564945346));
#51061=CARTESIAN_POINT('Ctrl Pts',(2.22418746193322,-4.79684426494046,387.027437069886));
#51062=CARTESIAN_POINT('Ctrl Pts',(-0.332916112977428,-5.27692065788687,
386.948309194427));
#51063=CARTESIAN_POINT('Ctrl Pts',(-2.80940963451955,-4.47927921359921,
386.869181318967));
#51064=CARTESIAN_POINT('Ctrl Pts',(-4.6056517301173,-2.59705543044056,386.790053443507));
#51065=CARTESIAN_POINT('Ctrl Pts',(-5.2867125013827,-0.0859982304292488,
386.710925568047));
#51066=CARTESIAN_POINT('Ctrl Pts',(-4.68768450473212,2.44588199879054,386.631797692588));
#51067=CARTESIAN_POINT('Ctrl Pts',(-2.95361232316089,4.38553292227813,386.552669817127));
#51068=CARTESIAN_POINT('Ctrl Pts',(-0.504372453036948,5.26330059910421,
386.473541941668));
#51069=CARTESIAN_POINT('Ctrl Pts',(2.06699274767947,4.86664830750627,386.394414066208));
#51070=CARTESIAN_POINT('Ctrl Pts',(4.1378703204085,3.29161874757629,386.315286190749));
#51071=CARTESIAN_POINT('Ctrl Pts',(5.20683199193,0.919578912180737,386.236158315288));
#51072=CARTESIAN_POINT('Ctrl Pts',(5.01504662121074,-1.67512153439562,386.157030439829));
#51073=CARTESIAN_POINT('Ctrl Pts',(3.60895181930755,-3.86421939514695,386.077902564369));
#51074=CARTESIAN_POINT('Ctrl Pts',(1.32900986066236,-5.11766133679979,385.998774688909));
#51075=CARTESIAN_POINT('Ctrl Pts',(-1.2727295467071,-5.13194741485647,385.91964681345));
#51076=CARTESIAN_POINT('Ctrl Pts',(-3.5662988394905,-3.90361849510962,385.84051893799));
#51077=CARTESIAN_POINT('Ctrl Pts',(-4.99634867925468,-1.73009382497687,
385.76139106253));
#51078=CARTESIAN_POINT('Ctrl Pts',(-5.21661648089346,0.862344049196109,
385.68226318707));
#51079=CARTESIAN_POINT('Ctrl Pts',(-4.1737680903862,3.24597977436508,385.60313531161));
#51080=CARTESIAN_POINT('Ctrl Pts',(-2.12031175571847,4.84365593601313,385.524007436151));
#51081=CARTESIAN_POINT('Ctrl Pts',(0.446542510511727,5.26852204647746,385.44487956069));
#51082=CARTESIAN_POINT('Ctrl Pts',(2.90527399685678,4.41770390260608,385.365751685231));
#51083=CARTESIAN_POINT('Ctrl Pts',(4.66054210967394,2.4972128487314,385.286623809771));
#51084=CARTESIAN_POINT('Ctrl Pts',(5.2873381133244,-0.0279364153108744,
385.207495934311));
#51085=CARTESIAN_POINT('Ctrl Pts',(4.63389386761938,-2.54632134491165,385.128368058852));
#51086=CARTESIAN_POINT('Ctrl Pts',(2.85842993763932,-4.44815726560116,385.049240183392));
#51087=CARTESIAN_POINT('Ctrl Pts',(0.390845137441743,-5.27294650517633,
384.970112307932));
#51088=CARTESIAN_POINT('Ctrl Pts',(-2.1713762578616,-4.82098018194518,384.890984432472));
#51089=CARTESIAN_POINT('Ctrl Pts',(-4.20783530881936,-3.2016943610792,384.811856557012));
#51090=CARTESIAN_POINT('Ctrl Pts',(-5.2254376100198,-0.807171946801767,
384.732728681553));
#51091=CARTESIAN_POINT('Ctrl Pts',(-4.97778783059681,1.78279361718495,384.653600806093));
#51092=CARTESIAN_POINT('Ctrl Pts',(-3.52485021126398,3.94108560628483,384.574472930633));
#51093=CARTESIAN_POINT('Ctrl Pts',(-1.21842922909547,5.14510981239459,384.495345055173));
#51094=CARTESIAN_POINT('Ctrl Pts',(1.38301395642869,5.10333196688562,384.416217179714));
#51095=CARTESIAN_POINT('Ctrl Pts',(3.64958350715001,3.82586787438508,384.337089304254));
#51096=CARTESIAN_POINT('Ctrl Pts',(5.03246761935876,1.62203404033908,384.257961428794));
#51097=CARTESIAN_POINT('Ctrl Pts',(5.19682409785237,-0.974548133184912,
384.178833553334));
#51098=CARTESIAN_POINT('Ctrl Pts',(4.10285677781212,-3.33515982055948,384.099705677875));
#51099=CARTESIAN_POINT('Ctrl Pts',(2.0154514986864,-4.88821849187982,384.020577802414));
#51100=CARTESIAN_POINT('Ctrl Pts',(-0.559961559389509,-5.25767703647906,
383.941449926955));
#51101=CARTESIAN_POINT('Ctrl Pts',(-2.99978931706339,-4.3540772640303,383.862322051495));
#51102=CARTESIAN_POINT('Ctrl Pts',(-4.71326840155275,-2.39621070501691,
383.783194176035));
#51103=CARTESIAN_POINT('Ctrl Pts',(-5.28550858957794,0.14185808898655,383.704066300575));
#51104=CARTESIAN_POINT('Ctrl Pts',(-4.57795151673967,2.64557832586642,383.624938425116));
#51105=CARTESIAN_POINT('Ctrl Pts',(-2.76192026167378,4.50871614055144,383.545810549656));
#51106=CARTESIAN_POINT('Ctrl Pts',(-0.277136335846315,5.28014395819535,
383.466682674197));
#51107=CARTESIAN_POINT('Ctrl Pts',(2.27475150580887,4.77307347049397,383.387554798736));
#51108=CARTESIAN_POINT('Ctrl Pts',(4.27584642055071,3.11028329188466,383.308426923277));
#51109=CARTESIAN_POINT('Ctrl Pts',(5.24161683545466,0.6943901771998,383.229299047817));
#51110=CARTESIAN_POINT('Ctrl Pts',(4.93821764164047,-1.8896378731662,383.150171172357));
#51111=CARTESIAN_POINT('Ctrl Pts',(3.43911186553428,-4.01612180396144,383.071043296897));
#51112=CARTESIAN_POINT('Ctrl Pts',(1.1072828290795,-5.17016919494313,382.991915421438));
#51113=CARTESIAN_POINT('Ctrl Pts',(-1.49265617402097,-5.07234682509687,
382.912787545978));
#51114=CARTESIAN_POINT('Ctrl Pts',(-3.73117351815568,-3.74634074068643,
382.833659670518));
#51115=CARTESIAN_POINT('Ctrl Pts',(-5.06624977097178,-1.5132210763935,382.754531795058));
#51116=CARTESIAN_POINT('Ctrl Pts',(-5.17461860862547,1.08629969307746,382.675403919598));
#51117=CARTESIAN_POINT('Ctrl Pts',(-4.03004033454984,3.42279121037416,382.596276044139));
#51118=CARTESIAN_POINT('Ctrl Pts',(-1.90965538190854,4.93051124025298,382.517148168679));
#51119=CARTESIAN_POINT('Ctrl Pts',(0.673120594328623,5.24439066369047,382.438020293219));
#51120=CARTESIAN_POINT('Ctrl Pts',(3.09291170766135,4.28842884242289,382.35889241776));
#51121=CARTESIAN_POINT('Ctrl Pts',(4.76380612269667,2.29409589888282,382.2797645423));
#51122=CARTESIAN_POINT('Ctrl Pts',(5.28122477966896,-0.255713891925586,
382.20063666684));
#51123=CARTESIAN_POINT('Ctrl Pts',(4.51988342850276,-2.74360685242242,382.12150879138));
#51124=CARTESIAN_POINT('Ctrl Pts',(2.66412810880644,-4.56718142707082,382.04238091592));
#51125=CARTESIAN_POINT('Ctrl Pts',(0.16329884807764,-5.28488961607806,381.96325304046));
#51126=CARTESIAN_POINT('Ctrl Pts',(-2.37707049000228,-4.72295041827389,
381.884125165001));
#51127=CARTESIAN_POINT('Ctrl Pts',(-4.3418720751543,-3.0174279860352,381.804997289541));
#51128=CARTESIAN_POINT('Ctrl Pts',(-5.25536215553288,-0.581285972741413,
381.725869414081));
#51129=CARTESIAN_POINT('Ctrl Pts',(-4.89635442846138,1.99560469001251,381.646741538622));
#51130=CARTESIAN_POINT('Ctrl Pts',(-3.35177659407457,4.08929314568265,381.567613663161));
#51131=CARTESIAN_POINT('Ctrl Pts',(-0.995622270609436,5.1928278483096,381.488485787702));
#51132=CARTESIAN_POINT('Ctrl Pts',(1.60160528794473,5.03900637720777,381.409357912242));
#51133=CARTESIAN_POINT('Ctrl Pts',(3.81103098679937,3.66507402184023,381.330230036782));
#51134=CARTESIAN_POINT('Ctrl Pts',(5.09767944760569,1.40370545962173,381.251102161322));
#51135=CARTESIAN_POINT('Ctrl Pts',(5.15001032416474,-1.1975468378773,381.171974285863));
#51136=CARTESIAN_POINT('Ctrl Pts',(3.95535257236717,-3.50883325283227,381.092846410403));
#51137=CARTESIAN_POINT('Ctrl Pts',(1.8029725310162,-4.97051454281288,381.013718534943));
#51138=CARTESIAN_POINT('Ctrl Pts',(-0.785967070782117,-5.22866909753901,
380.934590659483));
#51139=CARTESIAN_POINT('Ctrl Pts',(-3.18459792796892,-4.22078912113472,
380.855462784024));
#51140=CARTESIAN_POINT('Ctrl Pts',(-4.81213180629493,-2.19091584657144,
380.776334908564));
#51141=CARTESIAN_POINT('Ctrl Pts',(-5.27448867275235,0.369450956041967,
380.697207033104));
#51142=CARTESIAN_POINT('Ctrl Pts',(-4.45971656638884,2.84036140577044,380.618079157644));
#51143=CARTESIAN_POINT('Ctrl Pts',(-2.56509888808806,4.6235259772432,380.538951282184));
#51144=CARTESIAN_POINT('Ctrl Pts',(-0.0493855337170155,5.28718127521391,
380.459823406725));
#51145=CARTESIAN_POINT('Ctrl Pts',(2.47828569939099,4.67063429954727,380.380695531265));
#51146=CARTESIAN_POINT('Ctrl Pts',(4.40588161411396,2.92317156019379,380.301567655805));
#51147=CARTESIAN_POINT('Ctrl Pts',(5.26666718771851,0.467911852513223,380.222439780345));
#51148=CARTESIAN_POINT('Ctrl Pts',(4.8522176299277,-2.10064486282949,380.143311904886));
#51149=CARTESIAN_POINT('Ctrl Pts',(3.26288495036134,-4.1605656548862,380.064184029426));
#51150=CARTESIAN_POINT('Ctrl Pts',(0.883499402425967,-5.21307525111868,
379.985056153966));
#51151=CARTESIAN_POINT('Ctrl Pts',(-1.70981070849824,-5.0033261046046,379.905928278506));
#51152=CARTESIAN_POINT('Ctrl Pts',(-3.88911883186622,-3.58210545343612,
379.826800403046));
#51153=CARTESIAN_POINT('Ctrl Pts',(-5.1267420551265,-1.29353804277671,379.747672527587));
#51154=CARTESIAN_POINT('Ctrl Pts',(-5.12301067114194,1.3082379108094,379.668544652126));
#51155=CARTESIAN_POINT('Ctrl Pts',(-3.87882817196482,3.59324599495851,379.589416776668));
#51156=CARTESIAN_POINT('Ctrl Pts',(-1.69545248338881,5.00820982432685,379.510288901207));
#51157=CARTESIAN_POINT('Ctrl Pts',(0.898448589337301,5.21051963821565,379.431161025747));
#51158=CARTESIAN_POINT('Ctrl Pts',(3.27480540417913,4.15118950816177,379.352033150288));
#51159=CARTESIAN_POINT('Ctrl Pts',(4.85822301267979,2.08671845896413,379.272905274828));
#51160=CARTESIAN_POINT('Ctrl Pts',(5.26530339668872,-0.483016468385486,
379.193777399368));
#51161=CARTESIAN_POINT('Ctrl Pts',(4.39747886842774,-2.93579705866137,379.114649523908));
#51162=CARTESIAN_POINT('Ctrl Pts',(2.4648785829925,-4.67772362790043,379.035521648449));
#51163=CARTESIAN_POINT('Ctrl Pts',(-0.0645507124447473,-5.28701787148826,
378.956393772989));
#51164=CARTESIAN_POINT('Ctrl Pts',(-2.57835013545374,-4.61614940691036,
378.877265897529));
#51165=CARTESIAN_POINT('Ctrl Pts',(-4.46784531508162,-2.82755778162292,
378.798138022069));
#51166=CARTESIAN_POINT('Ctrl Pts',(-5.27552668260484,-0.354320460935515,
378.719010146609));
#51167=CARTESIAN_POINT('Ctrl Pts',(-4.80582774062997,2.20470961700277,378.63988227115));
#51168=CARTESIAN_POINT('Ctrl Pts',(-3.17247821056078,4.22990623671853,378.56075439569));
#51169=CARTESIAN_POINT('Ctrl Pts',(-0.770966287939471,5.23090200164121,
378.48162652023));
#51170=CARTESIAN_POINT('Ctrl Pts',(1.81722219130848,4.96532257515351,378.40249864477));
#51171=CARTESIAN_POINT('Ctrl Pts',(3.96540079385267,3.49747356130477,378.323370769311));
#51172=CARTESIAN_POINT('Ctrl Pts',(5.15342409853101,1.18276998126983,378.244242893851));
#51173=CARTESIAN_POINT('Ctrl Pts',(5.09363218664291,-1.41832151330666,378.165115018391));
#51174=CARTESIAN_POINT('Ctrl Pts',(3.80050266687247,-3.67599024033094,378.085987142931));
#51175=CARTESIAN_POINT('Ctrl Pts',(1.58714516515185,-5.04357958127442,378.006859267472));
#51176=CARTESIAN_POINT('Ctrl Pts',(-1.01051292004705,-5.18995071328536,
377.927731392012));
#51177=CARTESIAN_POINT('Ctrl Pts',(-3.36349224912901,-4.07966232156074,
377.848603516552));
#51178=CARTESIAN_POINT('Ctrl Pts',(-4.90205833974629,-1.98155211933397,
377.769475641092));
#51179=CARTESIAN_POINT('Ctrl Pts',(-5.25367321659188,0.596357695664665,
377.690347765633));
#51180=CARTESIAN_POINT('Ctrl Pts',(-4.33319923422642,3.02986949626759,377.611219890172));
#51181=CARTESIAN_POINT('Ctrl Pts',(-2.36351373006459,4.72974921277116,377.532092014713));
#51182=CARTESIAN_POINT('Ctrl Pts',(0.178456984968689,5.28439948077629,377.452964139253));
#51183=CARTESIAN_POINT('Ctrl Pts',(2.67721733402229,4.55952104001336,377.373836263793));
#51184=CARTESIAN_POINT('Ctrl Pts',(4.52773440567874,2.73063104786141,377.294708388334));
#51185=CARTESIAN_POINT('Ctrl Pts',(5.28193652635228,0.240564543316707,377.215580512874));
#51186=CARTESIAN_POINT('Ctrl Pts',(4.75720630136386,-2.3077506308472,377.136452637414));
#51187=CARTESIAN_POINT('Ctrl Pts',(3.08059835436342,-4.29728269340077,377.057324761954));
#51188=CARTESIAN_POINT('Ctrl Pts',(0.658075181053442,-5.24629982216222,
376.978196886494));
#51189=CARTESIAN_POINT('Ctrl Pts',(-1.923789860657,-4.92501343550216,376.899069011035));
#51190=CARTESIAN_POINT('Ctrl Pts',(-4.03984145181191,-3.4112176436405,376.819941135575));
#51191=CARTESIAN_POINT('Ctrl Pts',(-5.17771318819473,-1.07145270939303,
376.740813260115));
#51192=CARTESIAN_POINT('Ctrl Pts',(-5.0618885123847,1.52774652882403,376.661685384655));
#51193=CARTESIAN_POINT('Ctrl Pts',(-3.72041242686768,3.75702756739127,376.582557509196));
#51194=CARTESIAN_POINT('Ctrl Pts',(-1.47810086816716,5.0766073897426,376.503429633736));
#51195=CARTESIAN_POINT('Ctrl Pts',(1.12210802704861,5.16697187426544,376.424301758276));
#51196=CARTESIAN_POINT('Ctrl Pts',(3.45061728097363,4.00624077340234,376.345173882816));
#51197=CARTESIAN_POINT('Ctrl Pts',(4.94361743453053,1.87546566308182,376.266046007357));
#51198=CARTESIAN_POINT('Ctrl Pts',(5.23960352937691,-0.709422013391795,
376.186918131896));
#51199=CARTESIAN_POINT('Ctrl Pts',(4.2669075188957,-3.12253502690154,376.107790256437));
#51200=CARTESIAN_POINT('Ctrl Pts',(2.26105138176727,-4.77957859502704,376.028662380977));
#51201=CARTESIAN_POINT('Ctrl Pts',(-0.292280359441297,-5.27932727476591,
375.949534505517));
#51202=CARTESIAN_POINT('Ctrl Pts',(-2.77484145645776,-4.50077558721857,
375.870406630058));
#51203=CARTESIAN_POINT('Ctrl Pts',(-4.58552092957851,-2.63243616845826,
375.791278754598));
#51204=CARTESIAN_POINT('Ctrl Pts',(-5.28589405424394,-0.126697339588848,
375.712150879138));
#51205=CARTESIAN_POINT('Ctrl Pts',(-4.70637522968859,2.40972094307884,375.633023003678));
#51206=CARTESIAN_POINT('Ctrl Pts',(-2.98728944096456,4.36266186682328,375.553895128218));
#51207=CARTESIAN_POINT('Ctrl Pts',(-0.544875549618088,5.2592655277028,375.474767252759));
#51208=CARTESIAN_POINT('Ctrl Pts',(2.02945798133318,4.88240903418803,375.395639377299));
#51209=CARTESIAN_POINT('Ctrl Pts',(4.1124194375256,3.3233956145555,375.316511501839));
#51210=CARTESIAN_POINT('Ctrl Pts',(5.19956989745793,0.959601216722932,375.237383626379));
#51211=CARTESIAN_POINT('Ctrl Pts',(5.02785240284651,-1.63637626402564,375.15825575092));
#51212=CARTESIAN_POINT('Ctrl Pts',(3.63845954881624,-3.83644847785649,375.07912787546));
#51213=CARTESIAN_POINT('Ctrl Pts',(2.1252131908655,-4.68314727417153,375.026375958487));
#51214=CARTESIAN_POINT('Ctrl Pts',(1.3130361863572,-4.90075024188303,375.));
#51215=CARTESIAN_POINT('Ctrl Pts',(3.43378788736214,2.93584158412968,400.));
#51216=CARTESIAN_POINT('Ctrl Pts',(3.5274081047691,2.83896859117363,400.));
#51217=CARTESIAN_POINT('Ctrl Pts',(3.61639766139016,2.73803801067182,400.));
#51218=CARTESIAN_POINT('Ctrl Pts',(3.70064392711817,2.63347462098305,400.));
#51219=CARTESIAN_POINT('Ctrl Pts',(3.7863602040819,2.52708670700993,400.));
#51220=CARTESIAN_POINT('Ctrl Pts',(3.86716669541736,2.4169376104458,400.));
#51221=CARTESIAN_POINT('Ctrl Pts',(3.94291532865978,2.30342952486372,400.));
#51222=CARTESIAN_POINT('Ctrl Pts',(4.0194785589048,2.18870077902246,400.));
#51223=CARTESIAN_POINT('Ctrl Pts',(4.09087506217895,2.07053982333204,400.));
#51224=CARTESIAN_POINT('Ctrl Pts',(4.15691470252894,1.94932444936402,400.));
#51225=CARTESIAN_POINT('Ctrl Pts',(4.22265038067262,1.82866699624951,400.));
#51226=CARTESIAN_POINT('Ctrl Pts',(4.28307881326963,1.70498249960347,400.));
#51227=CARTESIAN_POINT('Ctrl Pts',(4.33796903578875,1.57861622186133,400.));
#51228=CARTESIAN_POINT('Ctrl Pts',(4.35514545623615,1.53907329021963,400.));
#51229=CARTESIAN_POINT('Ctrl Pts',(4.37177922400871,1.4992675947038,400.));
#51230=CARTESIAN_POINT('Ctrl Pts',(4.38786228046478,1.45920932342454,400.));
#51231=CARTESIAN_POINT('Ctrl Pts',(4.39466658849891,1.44226174770453,400.));
#51232=CARTESIAN_POINT('Ctrl Pts',(4.40137035215038,1.4252737748662,400.));
#51233=CARTESIAN_POINT('Ctrl Pts',(4.40797035684919,1.40825358562441,400.));
#51234=CARTESIAN_POINT('Ctrl Pts',(4.45876403554847,1.27726609952389,400.));
#51235=CARTESIAN_POINT('Ctrl Pts',(4.50346815482664,1.14424239282724,400.));
#51236=CARTESIAN_POINT('Ctrl Pts',(4.54192438339399,1.0095915875114,400.));
#51237=CARTESIAN_POINT('Ctrl Pts',(4.54556160496616,0.996856204140475,400.));
#51238=CARTESIAN_POINT('Ctrl Pts',(4.54914290628383,0.984106240915922,400.));
#51239=CARTESIAN_POINT('Ctrl Pts',(4.55266813447105,0.971342029205324,400.));
#51240=CARTESIAN_POINT('Ctrl Pts',(4.58957020263633,0.837726335240427,400.));
#51241=CARTESIAN_POINT('Ctrl Pts',(4.62033177525015,0.702551284224113,400.));
#51242=CARTESIAN_POINT('Ctrl Pts',(4.64501953741251,0.566245432199611,400.));
#51243=CARTESIAN_POINT('Ctrl Pts',(4.66997011124341,0.428488546737278,400.));
#51244=CARTESIAN_POINT('Ctrl Pts',(4.68871702492031,0.289575922051531,400.));
#51245=CARTESIAN_POINT('Ctrl Pts',(4.70127911966368,0.149931994443125,400.));
#51246=CARTESIAN_POINT('Ctrl Pts',(4.71259060845871,0.0241901691579915,
400.));
#51247=CARTESIAN_POINT('Ctrl Pts',(4.71888682786237,-0.102145233205809,
400.));
#51248=CARTESIAN_POINT('Ctrl Pts',(4.72014590598849,-0.228768981279396,
400.));
#51249=CARTESIAN_POINT('Ctrl Pts',(4.72038025896983,-0.252337536919386,
400.));
#51250=CARTESIAN_POINT('Ctrl Pts',(4.72044000678068,-0.275916082362071,
400.));
#51251=CARTESIAN_POINT('Ctrl Pts',(4.72032487691908,-0.299502644881673,
400.));
#51252=CARTESIAN_POINT('Ctrl Pts',(4.7202295663887,-0.319028836890583,400.));
#51253=CARTESIAN_POINT('Ctrl Pts',(4.72001432373552,-0.338562445738198,
400.));
#51254=CARTESIAN_POINT('Ctrl Pts',(4.71967941555818,-0.358084898519809,
400.));
#51255=CARTESIAN_POINT('Ctrl Pts',(4.71723826258667,-0.50038448044343,400.));
#51256=CARTESIAN_POINT('Ctrl Pts',(4.70844382065583,-0.642283037525432,
400.));
#51257=CARTESIAN_POINT('Ctrl Pts',(4.69336920270997,-0.783339178745919,
400.));
#51258=CARTESIAN_POINT('Ctrl Pts',(4.6781762779915,-0.925502339519639,400.));
#51259=CARTESIAN_POINT('Ctrl Pts',(4.65660432919034,-1.06681060067863,400.));
#51260=CARTESIAN_POINT('Ctrl Pts',(4.62867689090467,-1.20682343753469,400.));
#51261=CARTESIAN_POINT('Ctrl Pts',(4.61869343839589,-1.25687498515869,400.));
#51262=CARTESIAN_POINT('Ctrl Pts',(4.6078973313099,-1.30676103650428,400.));
#51263=CARTESIAN_POINT('Ctrl Pts',(4.59628802798414,-1.35646151489045,400.));
#51264=CARTESIAN_POINT('Ctrl Pts',(4.56393613692852,-1.49496288892161,400.));
#51265=CARTESIAN_POINT('Ctrl Pts',(4.5252728763513,-1.63202392528166,400.));
#51266=CARTESIAN_POINT('Ctrl Pts',(4.48051876179014,-1.76728613860278,400.));
#51267=CARTESIAN_POINT('Ctrl Pts',(4.45444111221125,-1.84610169857621,400.));
#51268=CARTESIAN_POINT('Ctrl Pts',(4.42629449108343,-1.92430635496666,400.));
#51269=CARTESIAN_POINT('Ctrl Pts',(4.3961147432142,-2.00182684735068,400.));
#51270=CARTESIAN_POINT('Ctrl Pts',(4.37905752655991,-2.04564046168142,400.));
#51271=CARTESIAN_POINT('Ctrl Pts',(4.36135075314648,-2.08923549081769,400.));
#51272=CARTESIAN_POINT('Ctrl Pts',(4.34300012999985,-2.13259835388101,400.));
#51273=CARTESIAN_POINT('Ctrl Pts',(4.33569114983399,-2.14986960965973,400.));
#51274=CARTESIAN_POINT('Ctrl Pts',(4.32828379731778,-2.1670950989908,400.));
#51275=CARTESIAN_POINT('Ctrl Pts',(4.32077934892109,-2.18427268326289,400.));
#51276=CARTESIAN_POINT('Ctrl Pts',(4.26291559960507,-2.31672204897711,400.));
#51277=CARTESIAN_POINT('Ctrl Pts',(4.19927220468674,-2.44635051906979,400.));
#51278=CARTESIAN_POINT('Ctrl Pts',(4.13013682131626,-2.57280699644751,400.));
#51279=CARTESIAN_POINT('Ctrl Pts',(4.06045781537672,-2.70025782131784,400.));
#51280=CARTESIAN_POINT('Ctrl Pts',(3.98519984558575,-2.82448729912954,400.));
#51281=CARTESIAN_POINT('Ctrl Pts',(3.90460511771477,-2.94512595263581,400.));
#51282=CARTESIAN_POINT('Ctrl Pts',(3.82424500701874,-3.06541341815719,400.));
#51283=CARTESIAN_POINT('Ctrl Pts',(3.73857881602801,-3.18213164834041,400.));
#51284=CARTESIAN_POINT('Ctrl Pts',(3.6477996177404,-3.29489368172134,400.));
#51285=CARTESIAN_POINT('Ctrl Pts',(3.5967838663573,-3.35826326383848,400.));
#51286=CARTESIAN_POINT('Ctrl Pts',(3.54415252096129,-3.42038297838046,400.));
#51287=CARTESIAN_POINT('Ctrl Pts',(3.48993392052895,-3.48117996717138,400.));
#51288=CARTESIAN_POINT('Ctrl Pts',(3.44896085489101,-3.52712432929906,400.));
#51289=CARTESIAN_POINT('Ctrl Pts',(3.40708123835602,-3.57231323683387,400.));
#51290=CARTESIAN_POINT('Ctrl Pts',(3.36432098798037,-3.61672891625407,400.));
#51291=CARTESIAN_POINT('Ctrl Pts',(3.33855500174508,-3.64349241212974,400.));
#51292=CARTESIAN_POINT('Ctrl Pts',(3.31246924398559,-3.66997513430726,400.));
#51293=CARTESIAN_POINT('Ctrl Pts',(3.28606918882681,-3.69617297251379,400.));
#51294=CARTESIAN_POINT('Ctrl Pts',(3.27036247014898,-3.71175938217099,400.));
#51295=CARTESIAN_POINT('Ctrl Pts',(3.25455092639766,-3.72723854435311,400.));
#51296=CARTESIAN_POINT('Ctrl Pts',(3.23863897351742,-3.74260697959096,400.));
#51297=CARTESIAN_POINT('Ctrl Pts',(3.1336340986207,-3.84402511673945,400.));
#51298=CARTESIAN_POINT('Ctrl Pts',(3.02421929001433,-3.94066423251855,400.));
#51299=CARTESIAN_POINT('Ctrl Pts',(2.9108005879282,-4.03233943093569,400.));
#51300=CARTESIAN_POINT('Ctrl Pts',(2.80145832608402,-4.12071968362393,400.));
#51301=CARTESIAN_POINT('Ctrl Pts',(2.6883940765038,-4.20448664484191,400.));
#51302=CARTESIAN_POINT('Ctrl Pts',(2.57193725133249,-4.28344581179871,400.));
#51303=CARTESIAN_POINT('Ctrl Pts',(2.52394060920348,-4.31598812843542,400.));
#51304=CARTESIAN_POINT('Ctrl Pts',(2.47536734937678,-4.34771342641671,400.));
#51305=CARTESIAN_POINT('Ctrl Pts',(2.4262391678432,-4.37860645542617,400.));
#51306=CARTESIAN_POINT('Ctrl Pts',(2.4057205129273,-4.39150909871084,400.));
#51307=CARTESIAN_POINT('Ctrl Pts',(2.38510290902907,-4.40426785187222,400.));
#51308=CARTESIAN_POINT('Ctrl Pts',(2.36439500508045,-4.41687723791363,400.));
#51309=CARTESIAN_POINT('Ctrl Pts',(2.23718127032588,-4.49433979014823,400.));
#51310=CARTESIAN_POINT('Ctrl Pts',(2.10670807231056,-4.56608151115334,400.));
#51311=CARTESIAN_POINT('Ctrl Pts',(1.97337536799814,-4.63189274468176,400.));
#51312=CARTESIAN_POINT('Ctrl Pts',(1.84010399988323,-4.69767370348621,400.));
#51313=CARTESIAN_POINT('Ctrl Pts',(1.70397511685538,-4.75753010362705,400.));
#51314=CARTESIAN_POINT('Ctrl Pts',(1.56535633801641,-4.81121182598771,400.));
#51315=CARTESIAN_POINT('Ctrl Pts',(1.52584133805609,-4.82651446589492,400.));
#51316=CARTESIAN_POINT('Ctrl Pts',(1.48612384295406,-4.84131506971587,400.));
#51317=CARTESIAN_POINT('Ctrl Pts',(1.44621200692229,-4.85560715259022,400.));
#51318=CARTESIAN_POINT('Ctrl Pts',(1.4021027224054,-4.87140230542011,400.));
#51319=CARTESIAN_POINT('Ctrl Pts',(1.35775607141996,-4.88657636029028,400.));
#51320=CARTESIAN_POINT('Ctrl Pts',(1.31318543090145,-4.90112867346808,400.));
#51321=CARTESIAN_POINT('Ctrl Pts',(-4.51746064445937,-7.62825515632226E-5,
398.387416697508));
#51322=CARTESIAN_POINT('Ctrl Pts',(-4.51763289072636,-0.284226777710601,
398.397425295273));
#51323=CARTESIAN_POINT('Ctrl Pts',(-4.49123863994107,-0.568345670691312,
398.407433893039));
#51324=CARTESIAN_POINT('Ctrl Pts',(-4.4379719366677,-0.847333855511198,
398.417442490804));
#51325=CARTESIAN_POINT('Ctrl Pts',(-4.29759659267063,-1.58255980359031,
398.443818449291));
#51326=CARTESIAN_POINT('Ctrl Pts',(-3.97059302033473,-2.2821531656744,398.470194407778));
#51327=CARTESIAN_POINT('Ctrl Pts',(-3.49655043505552,-2.86141654221982,
398.496570366264));
#51328=CARTESIAN_POINT('Ctrl Pts',(-3.0225078497763,-3.44067991876523,398.522946324751));
#51329=CARTESIAN_POINT('Ctrl Pts',(-2.40142625155378,-3.89961330977197,
398.549322283237));
#51330=CARTESIAN_POINT('Ctrl Pts',(-1.70849788678631,-4.18265520276417,
398.575698241724));
#51331=CARTESIAN_POINT('Ctrl Pts',(-1.01556952201883,-4.46569709575638,
398.60207420021));
#51332=CARTESIAN_POINT('Ctrl Pts',(-0.250794390706405,-4.57284749073406,
398.628450158697));
#51333=CARTESIAN_POINT('Ctrl Pts',(0.493238771257572,-4.49113405337507,
398.654826117184));
#51334=CARTESIAN_POINT('Ctrl Pts',(1.23727193322155,-4.40942061601609,398.68120207567));
#51335=CARTESIAN_POINT('Ctrl Pts',(1.96056312583708,-4.13884334632044,398.707578034157));
#51336=CARTESIAN_POINT('Ctrl Pts',(2.57554593307285,-3.71216011566315,398.733953992643));
#51337=CARTESIAN_POINT('Ctrl Pts',(3.19052874030862,-3.28547688500585,398.76032995113));
#51338=CARTESIAN_POINT('Ctrl Pts',(3.69720316216463,-2.70268769338692,398.786705909617));
#51339=CARTESIAN_POINT('Ctrl Pts',(4.03422784198701,-2.03434886067149,398.813081868103));
#51340=CARTESIAN_POINT('Ctrl Pts',(4.37125252180939,-1.36601002795605,398.83945782659));
#51341=CARTESIAN_POINT('Ctrl Pts',(4.53862745959814,-0.612121554144129,
398.865833785076));
#51342=CARTESIAN_POINT('Ctrl Pts',(4.51608913784387,0.136045847258709,398.892209743563));
#51343=CARTESIAN_POINT('Ctrl Pts',(4.49355081608961,0.884213248661547,398.91858570205));
#51344=CARTESIAN_POINT('Ctrl Pts',(4.28109923479233,1.6266595776553,398.944961660536));
#51345=CARTESIAN_POINT('Ctrl Pts',(3.90445518858537,2.27349934610636,398.971337619023));
#51346=CARTESIAN_POINT('Ctrl Pts',(3.5278111423784,2.92033911455742,398.997713577509));
#51347=CARTESIAN_POINT('Ctrl Pts',(2.98697463126176,3.47157232246578,399.024089535996));
#51348=CARTESIAN_POINT('Ctrl Pts',(2.34742289856565,3.86046308384535,399.050465494483));
#51349=CARTESIAN_POINT('Ctrl Pts',(1.70787116586954,4.24935384522491,399.076841452969));
#51350=CARTESIAN_POINT('Ctrl Pts',(0.969604211593966,4.47590216007566,399.103217411456));
#51351=CARTESIAN_POINT('Ctrl Pts',(0.222001520718283,4.51268048034993,399.129593369942));
#51352=CARTESIAN_POINT('Ctrl Pts',(-0.525601170157399,4.5494588006242,399.155969328429));
#51353=CARTESIAN_POINT('Ctrl Pts',(-1.28253959763319,4.39646712632199,399.182345286915));
#51354=CARTESIAN_POINT('Ctrl Pts',(-1.95717379804064,4.07222787544583,399.208721245402));
#51355=CARTESIAN_POINT('Ctrl Pts',(-2.63180799844808,3.74798862456968,399.235097203889));
#51356=CARTESIAN_POINT('Ctrl Pts',(-3.22413797178719,3.25250179711959,399.261473162375));
#51357=CARTESIAN_POINT('Ctrl Pts',(-3.66245231437547,2.64575381071457,399.287849120862));
#51358=CARTESIAN_POINT('Ctrl Pts',(-4.10076665696376,2.03900582430954,399.314225079348));
#51359=CARTESIAN_POINT('Ctrl Pts',(-4.38506536880122,1.32099667894959,399.340601037835));
#51360=CARTESIAN_POINT('Ctrl Pts',(-4.48092940799817,0.578654358541173,
399.366976996322));
#51361=CARTESIAN_POINT('Ctrl Pts',(-4.50569226564232,0.386898228114258,
399.37379023005));
#51362=CARTESIAN_POINT('Ctrl Pts',(-4.51788177656568,0.193518461005119,
399.380603463779));
#51363=CARTESIAN_POINT('Ctrl Pts',(-4.51769110620511,0.00011483889287206,
399.387416697508));
#51364=CARTESIAN_POINT('Ctrl Pts',(-1.31303618635555,-4.90075024188347,
400.));
#51365=CARTESIAN_POINT('Ctrl Pts',(-2.12521319086393,-4.68314727417224,
399.973624041513));
#51366=CARTESIAN_POINT('Ctrl Pts',(-3.63845957255092,-3.83644859241818,
399.92087212454));
#51367=CARTESIAN_POINT('Ctrl Pts',(-5.02785239518849,-1.63637624738159,
399.84174424908));
#51368=CARTESIAN_POINT('Ctrl Pts',(-5.19956989353463,0.959601198026513,
399.76261637362));
#51369=CARTESIAN_POINT('Ctrl Pts',(-4.11241943286933,3.32339561801255,399.683488498161));
#51370=CARTESIAN_POINT('Ctrl Pts',(-2.02945797892606,4.8824090247121,399.604360622701));
#51371=CARTESIAN_POINT('Ctrl Pts',(0.54487554882432,5.2592655238007,399.525232747241));
#51372=CARTESIAN_POINT('Ctrl Pts',(2.98728943775363,4.36266186092565,399.446104871781));
#51373=CARTESIAN_POINT('Ctrl Pts',(4.70637522433117,2.40972094089285,399.366976996322));
#51374=CARTESIAN_POINT('Ctrl Pts',(5.28589404837916,-0.126697339701679,
399.287849120862));
#51375=CARTESIAN_POINT('Ctrl Pts',(4.58552092441564,-2.6324361653814,399.208721245402));
#51376=CARTESIAN_POINT('Ctrl Pts',(2.77484145336967,-4.50077558224301,399.129593369943));
#51377=CARTESIAN_POINT('Ctrl Pts',(0.292280359106768,-5.27932726882375,
399.050465494482));
#51378=CARTESIAN_POINT('Ctrl Pts',(-2.26105137922953,-4.77957858969287,
398.971337619023));
#51379=CARTESIAN_POINT('Ctrl Pts',(-4.26690751412045,-3.12253502339944,
398.892209743563));
#51380=CARTESIAN_POINT('Ctrl Pts',(-5.23960352350959,-0.709422012603199,
398.813081868103));
#51381=CARTESIAN_POINT('Ctrl Pts',(-4.94361742899746,1.87546566098248,398.733953992643));
#51382=CARTESIAN_POINT('Ctrl Pts',(-3.45061727711166,4.00624076891526,398.654826117184));
#51383=CARTESIAN_POINT('Ctrl Pts',(-1.12210802579434,5.16697186848109,398.575698241724));
#51384=CARTESIAN_POINT('Ctrl Pts',(1.47810086651078,5.07660738405961,398.496570366264));
#51385=CARTESIAN_POINT('Ctrl Pts',(3.72041242270134,3.75702756318667,398.417442490805));
#51386=CARTESIAN_POINT('Ctrl Pts',(5.06188850671742,1.52774652711538,398.338314615344));
#51387=CARTESIAN_POINT('Ctrl Pts',(5.17771318239863,-1.0714527081918,398.259186739885));
#51388=CARTESIAN_POINT('Ctrl Pts',(4.03984144729043,-3.41121763982034,398.180058864425));
#51389=CARTESIAN_POINT('Ctrl Pts',(1.92378985850489,-4.92501342998799,398.100930988965));
#51390=CARTESIAN_POINT('Ctrl Pts',(-0.658075180315041,-5.24629981628919,
398.021803113506));
#51391=CARTESIAN_POINT('Ctrl Pts',(-3.08059835091328,-4.29728268859095,
397.942675238046));
#51392=CARTESIAN_POINT('Ctrl Pts',(-4.75720629603741,-2.30775062826524,
397.863547362586));
#51393=CARTESIAN_POINT('Ctrl Pts',(-5.28193652043922,0.240564543045645,
397.784419487126));
#51394=CARTESIAN_POINT('Ctrl Pts',(-4.52773440061085,2.73063104480294,397.705291611666));
#51395=CARTESIAN_POINT('Ctrl Pts',(-2.67721733102668,4.55952103490808,397.626163736206));
#51396=CARTESIAN_POINT('Ctrl Pts',(-0.178456984770649,5.28439947486034,
397.547035860747));
#51397=CARTESIAN_POINT('Ctrl Pts',(2.36351372741711,4.72974920747697,397.467907985287));
#51398=CARTESIAN_POINT('Ctrl Pts',(4.33319922937441,3.02986949287705,397.388780109827));
#51399=CARTESIAN_POINT('Ctrl Pts',(5.25367321071018,0.596357694998765,397.309652234368));
#51400=CARTESIAN_POINT('Ctrl Pts',(4.90205833425909,-1.98155211711401,397.230524358907));
#51401=CARTESIAN_POINT('Ctrl Pts',(3.36349224536493,-4.07966231699243,397.151396483448));
#51402=CARTESIAN_POINT('Ctrl Pts',(1.01051291891753,-5.18995070747486,397.072268607988));
#51403=CARTESIAN_POINT('Ctrl Pts',(-1.58714516337332,-5.04357957562867,
396.993140732529));
#51404=CARTESIAN_POINT('Ctrl Pts',(-3.80050266261658,-3.67599023621695,
396.914012857068));
#51405=CARTESIAN_POINT('Ctrl Pts',(-5.09363218094012,-1.41832151172053,
396.834884981609));
#51406=CARTESIAN_POINT('Ctrl Pts',(-5.15342409276215,1.182769979944,396.755757106149));
#51407=CARTESIAN_POINT('Ctrl Pts',(-3.96540078941456,3.49747355738801,396.676629230689));
#51408=CARTESIAN_POINT('Ctrl Pts',(-1.81722218927578,4.96532256959422,396.597501355229));
#51409=CARTESIAN_POINT('Ctrl Pts',(0.770966287074601,5.23090199578547,396.51837347977));
#51410=CARTESIAN_POINT('Ctrl Pts',(3.17247820700774,4.22990623198423,396.43924560431));
#51411=CARTESIAN_POINT('Ctrl Pts',(4.8058277352491,2.20470961453625,396.36011772885));
#51412=CARTESIAN_POINT('Ctrl Pts',(5.275526676699,-0.354320460537079,396.28098985339));
#51413=CARTESIAN_POINT('Ctrl Pts',(4.46784531008081,-2.82755777845599,396.201861977931));
#51414=CARTESIAN_POINT('Ctrl Pts',(2.57835013256881,-4.61614940174172,396.122734102471));
#51415=CARTESIAN_POINT('Ctrl Pts',(0.0645507123742531,-5.2870178655694,
396.043606227011));
#51416=CARTESIAN_POINT('Ctrl Pts',(-2.46487858023149,-4.67772362266456,
395.964478351551));
#51417=CARTESIAN_POINT('Ctrl Pts',(-4.39747886350376,-2.93579705537622,
395.885350476092));
#51418=CARTESIAN_POINT('Ctrl Pts',(-5.26530339079403,-0.48301646784655,
395.806222600631));
#51419=CARTESIAN_POINT('Ctrl Pts',(-4.85822300724173,2.08671845662638,395.727094725172));
#51420=CARTESIAN_POINT('Ctrl Pts',(-3.27480540051438,4.15118950351341,395.647966849712));
#51421=CARTESIAN_POINT('Ctrl Pts',(-0.898448588333209,5.21051963238218,
395.568838974252));
#51422=CARTESIAN_POINT('Ctrl Pts',(1.69545248148909,5.00820981872071,395.489711098793));
#51423=CARTESIAN_POINT('Ctrl Pts',(3.87882816762124,3.59324599093717,395.410583223333));
#51424=CARTESIAN_POINT('Ctrl Pts',(5.12301066540628,1.30823790934658,395.331455347873));
#51425=CARTESIAN_POINT('Ctrl Pts',(5.12674204938754,-1.29353804132683,395.252327472413));
#51426=CARTESIAN_POINT('Ctrl Pts',(3.88911882751359,-3.58210544942458,395.173199596953));
#51427=CARTESIAN_POINT('Ctrl Pts',(1.70981070658587,-5.00332609900278,395.094071721494));
#51428=CARTESIAN_POINT('Ctrl Pts',(-0.883499401435098,-5.21307524528295,
395.014943846034));
#51429=CARTESIAN_POINT('Ctrl Pts',(-3.26288494670713,-4.16056565022955,
394.935815970574));
#51430=CARTESIAN_POINT('Ctrl Pts',(-4.85221762449495,-2.10064486047942,
394.856688095114));
#51431=CARTESIAN_POINT('Ctrl Pts',(-5.26666718182262,0.467911851987696,
394.777560219655));
#51432=CARTESIAN_POINT('Ctrl Pts',(-4.40588160918252,2.92317155691987,394.698432344195));
#51433=CARTESIAN_POINT('Ctrl Pts',(-2.47828569661807,4.67063429431767,394.619304468735));
#51434=CARTESIAN_POINT('Ctrl Pts',(0.0493855336599835,5.28718126929493,
394.540176593275));
#51435=CARTESIAN_POINT('Ctrl Pts',(2.56509888521489,4.623525972068,394.461048717816));
#51436=CARTESIAN_POINT('Ctrl Pts',(4.45971656139522,2.84036140259214,394.381920842355));
#51437=CARTESIAN_POINT('Ctrl Pts',(5.27448866684743,0.369450955630144,394.302792966896));
#51438=CARTESIAN_POINT('Ctrl Pts',(4.81213180090847,-2.19091584411711,394.223665091436));
#51439=CARTESIAN_POINT('Ctrl Pts',(3.18459792440514,-4.2207891164085,394.144537215977));
#51440=CARTESIAN_POINT('Ctrl Pts',(0.785967069903959,-5.22866909168525,
394.065409340517));
#51441=CARTESIAN_POINT('Ctrl Pts',(-1.8029725289961,-4.97051453724898,393.986281465057));
#51442=CARTESIAN_POINT('Ctrl Pts',(-3.95535256793798,-3.50883324890547,
393.907153589597));
#51443=CARTESIAN_POINT('Ctrl Pts',(-5.15001031839888,-1.19754683653839,
393.828025714137));
#51444=CARTESIAN_POINT('Ctrl Pts',(-5.0976794418993,1.40370545804854,393.748897838677));
#51445=CARTESIAN_POINT('Ctrl Pts',(-3.81103098253419,3.66507401773587,393.669769963218));
#51446=CARTESIAN_POINT('Ctrl Pts',(-1.60160528615343,5.03900637156607,393.590642087758));
#51447=CARTESIAN_POINT('Ctrl Pts',(0.995622269493122,5.19282784249655,393.511514212298));
#51448=CARTESIAN_POINT('Ctrl Pts',(3.3517765903209,4.08929314110579,393.432386336838));
#51449=CARTESIAN_POINT('Ctrl Pts',(4.89635442297923,1.99560468778007,393.353258461378));
#51450=CARTESIAN_POINT('Ctrl Pts',(5.2553621496497,-0.581285972088894,393.274130585919));
#51451=CARTESIAN_POINT('Ctrl Pts',(4.34187207029457,-3.01742798265574,393.195002710459));
#51452=CARTESIAN_POINT('Ctrl Pts',(2.37707048734272,-4.72295041298575,393.115874834999));
#51453=CARTESIAN_POINT('Ctrl Pts',(-0.163298847893048,-5.28488961016167,
393.03674695954));
#51454=CARTESIAN_POINT('Ctrl Pts',(-2.66412810582239,-4.56718142195876,
392.957619084079));
#51455=CARTESIAN_POINT('Ctrl Pts',(-4.51988342344183,-2.74360684935247,
392.87849120862));
#51456=CARTESIAN_POINT('Ctrl Pts',(-5.28122477375654,-0.255713891641081,
392.79936333316));
#51457=CARTESIAN_POINT('Ctrl Pts',(-4.76380611736435,2.29409589631297,392.7202354577));
#51458=CARTESIAN_POINT('Ctrl Pts',(-3.09291170420029,4.28842883762094,392.64110758224));
#51459=CARTESIAN_POINT('Ctrl Pts',(-0.67312059357683,5.24439065781915,392.561979706781));
#51460=CARTESIAN_POINT('Ctrl Pts',(1.90965537976903,4.9305112347339,392.482851831321));
#51461=CARTESIAN_POINT('Ctrl Pts',(4.03004033003705,3.4227912065437,392.403723955861));
#51462=CARTESIAN_POINT('Ctrl Pts',(5.17461860283211,1.0862996918631,392.324596080401));
#51463=CARTESIAN_POINT('Ctrl Pts',(5.06624976530063,-1.51322107469774,392.245468204942));
#51464=CARTESIAN_POINT('Ctrl Pts',(3.73117351397988,-3.74634073649114,392.166340329482));
#51465=CARTESIAN_POINT('Ctrl Pts',(1.49265617235166,-5.07234681941786,392.087212454022));
#51466=CARTESIAN_POINT('Ctrl Pts',(-1.10728282783815,-5.1701691891555,392.008084578562));
#51467=CARTESIAN_POINT('Ctrl Pts',(-3.43911186168285,-4.01612179946654,
391.928956703103));
#51468=CARTESIAN_POINT('Ctrl Pts',(-4.93821763611149,-1.8896378710524,391.849828827643));
#51469=CARTESIAN_POINT('Ctrl Pts',(-5.24161682958689,0.694390176420624,
391.770700952183));
#51470=CARTESIAN_POINT('Ctrl Pts',(-4.27584641576499,3.1102832884012,391.691573076723));
#51471=CARTESIAN_POINT('Ctrl Pts',(-2.27475150326393,4.77307346514974,391.612445201264));
#51472=CARTESIAN_POINT('Ctrl Pts',(0.277136335534271,5.28014395228432,391.533317325804));
#51473=CARTESIAN_POINT('Ctrl Pts',(2.76192025858026,4.50871613550486,391.454189450344));
#51474=CARTESIAN_POINT('Ctrl Pts',(4.57795151161372,2.64557832290629,391.375061574885));
#51475=CARTESIAN_POINT('Ctrl Pts',(5.28550858366077,0.141858088829558,391.295933699424));
#51476=CARTESIAN_POINT('Ctrl Pts',(4.71326839627705,-2.39621070233275,391.216805823965));
#51477=CARTESIAN_POINT('Ctrl Pts',(2.99978931370662,-4.35407725915487,391.137677948505));
#51478=CARTESIAN_POINT('Ctrl Pts',(0.559961558764467,-5.2576770305929,391.058550073045));
#51479=CARTESIAN_POINT('Ctrl Pts',(-2.01545149642842,-4.88821848640817,
390.979422197585));
#51480=CARTESIAN_POINT('Ctrl Pts',(-4.10285677321784,-3.33515981682715,
390.900294322126));
#51481=CARTESIAN_POINT('Ctrl Pts',(-5.19682409203417,-0.974548132095691,
390.821166446665));
#51482=CARTESIAN_POINT('Ctrl Pts',(-5.03246761372548,1.62203403852146,390.742038571206));
#51483=CARTESIAN_POINT('Ctrl Pts',(-3.64958350306562,3.82586787010077,390.662910695746));
#51484=CARTESIAN_POINT('Ctrl Pts',(-1.38301395488213,5.10333196117197,390.583782820286));
#51485=CARTESIAN_POINT('Ctrl Pts',(1.21842922772966,5.14510980663504,390.504654944826));
#51486=CARTESIAN_POINT('Ctrl Pts',(3.52485020731651,3.94108560187402,390.425527069367));
#51487=CARTESIAN_POINT('Ctrl Pts',(4.97778782502355,1.78279361519087,390.346399193907));
#51488=CARTESIAN_POINT('Ctrl Pts',(5.2254376041702,-0.807171945896316,390.267271318447));
#51489=CARTESIAN_POINT('Ctrl Pts',(4.2078353041098,-3.20169435749343,390.188143442988));
#51490=CARTESIAN_POINT('Ctrl Pts',(2.17137625543244,-4.82098017654731,390.109015567527));
#51491=CARTESIAN_POINT('Ctrl Pts',(-0.390845137002325,-5.27294649927341,
390.029887692068));
#51492=CARTESIAN_POINT('Ctrl Pts',(-2.85842993443779,-4.44815726062243,
389.950759816608));
#51493=CARTESIAN_POINT('Ctrl Pts',(-4.63389386243089,-2.54632134206259,
389.871631941148));
#51494=CARTESIAN_POINT('Ctrl Pts',(-5.2873381074052,-0.0279364152813674,
389.792504065688));
#51495=CARTESIAN_POINT('Ctrl Pts',(-4.66054210445731,2.49721284593419,389.713376190229));
#51496=CARTESIAN_POINT('Ctrl Pts',(-2.90527399360582,4.41770389765948,389.634248314769));
#51497=CARTESIAN_POINT('Ctrl Pts',(-0.446542510013585,5.2685220405792,389.55512043931));
#51498=CARTESIAN_POINT('Ctrl Pts',(2.12031175334316,4.84365593059135,389.475992563849));
#51499=CARTESIAN_POINT('Ctrl Pts',(4.17376808571255,3.24597977073262,389.39686468839));
#51500=CARTESIAN_POINT('Ctrl Pts',(5.21661647505316,0.862344048232485,389.31773681293));
#51501=CARTESIAN_POINT('Ctrl Pts',(4.99634867366186,-1.73009382303836,389.23860893747));
#51502=CARTESIAN_POINT('Ctrl Pts',(3.56629883549932,-3.90361849073832,389.15948106201));
#51503=CARTESIAN_POINT('Ctrl Pts',(1.27272954528402,-5.13194740911081,389.08035318655));
#51504=CARTESIAN_POINT('Ctrl Pts',(-1.3290098591728,-5.11766133107102,389.001225311091));
#51505=CARTESIAN_POINT('Ctrl Pts',(-3.60895181526604,-3.86421939082217,
388.922097435631));
#51506=CARTESIAN_POINT('Ctrl Pts',(-5.01504661559582,-1.67512153252199,
388.842969560171));
#51507=CARTESIAN_POINT('Ctrl Pts',(-5.20683198610126,0.919578911149497,
388.763841684712));
#51508=CARTESIAN_POINT('Ctrl Pts',(-4.13787031577727,3.29161874388992,388.684713809251));
#51509=CARTESIAN_POINT('Ctrl Pts',(-2.0669927453671,4.86664830205737,388.605585933792));
#51510=CARTESIAN_POINT('Ctrl Pts',(0.504372452470541,5.2633005932121,388.526458058332));
#51511=CARTESIAN_POINT('Ctrl Pts',(2.95361231985281,4.38553291736953,388.447330182872));
#51512=CARTESIAN_POINT('Ctrl Pts',(4.68768449948338,2.44588199605403,388.368202307412));
#51513=CARTESIAN_POINT('Ctrl Pts',(5.28671249546426,-0.0859982303311033,
388.289074431953));
#51514=CARTESIAN_POINT('Ctrl Pts',(4.60565172496217,-2.59705542753155,388.209946556493));
#51515=CARTESIAN_POINT('Ctrl Pts',(2.80940963137597,-4.47927920858367,388.130818681033));
#51516=CARTESIAN_POINT('Ctrl Pts',(0.332916112606594,-5.27692065197923,
388.051690805573));
#51517=CARTESIAN_POINT('Ctrl Pts',(-2.22418745944155,-4.79684425957118,
387.972562930114));
#51518=CARTESIAN_POINT('Ctrl Pts',(-4.24274134038657,-3.15529247834378,
387.893435054654));
#51519=CARTESIAN_POINT('Ctrl Pts',(-5.23398656144486,-0.749739541395986,
387.814307179194));
#51520=CARTESIAN_POINT('Ctrl Pts',(-4.95790971666796,1.83735025150007,387.735179303734));
#51521=CARTESIAN_POINT('Ctrl Pts',(-3.48135818389009,3.97955649548785,387.656051428275));
#51522=CARTESIAN_POINT('Ctrl Pts',(-1.16185415329344,5.15817987586638,387.576923552815));
#51523=CARTESIAN_POINT('Ctrl Pts',(1.43897337488296,5.0878365079566,387.497795677355));
#51524=CARTESIAN_POINT('Ctrl Pts',(3.69137763358211,3.7855588585581,387.418667801895));
#51525=CARTESIAN_POINT('Ctrl Pts',(5.04997670698908,1.56667161976776,387.339539926436));
#51526=CARTESIAN_POINT('Ctrl Pts',(5.1858086147589,-1.03155887685117,387.260412050976));
#51527=CARTESIAN_POINT('Ctrl Pts',(4.06598393848355,-3.38001469187811,387.181284175516));
#51528=CARTESIAN_POINT('Ctrl Pts',(1.96164944276588,-4.91005663602919,387.102156300056));
#51529=CARTESIAN_POINT('Ctrl Pts',(-0.617665566383616,-5.25121071310437,
387.023028424596));
#51530=CARTESIAN_POINT('Ctrl Pts',(-3.04742321760052,-4.32087218488899,
386.943900549136));
#51531=CARTESIAN_POINT('Ctrl Pts',(-4.73929844549354,-2.34430692313541,
386.864772673677));
#51532=CARTESIAN_POINT('Ctrl Pts',(-5.28363203833613,0.199892943312196,
386.785644798217));
#51533=CARTESIAN_POINT('Ctrl Pts',(-4.54862274572651,2.695692085973,386.706516922757));
#51534=CARTESIAN_POINT('Ctrl Pts',(-2.71224074091265,4.53877459989496,386.627389047297));
#51535=CARTESIAN_POINT('Ctrl Pts',(-0.219135128106394,5.28286896496098,
386.548261171838));
#51536=CARTESIAN_POINT('Ctrl Pts',(2.32703038082081,4.74780520999492,386.469133296378));
#51537=CARTESIAN_POINT('Ctrl Pts',(4.30974451002784,3.06314004962277,386.390005420918));
#51538=CARTESIAN_POINT('Ctrl Pts',(5.24892628554031,0.636786898642001,386.310877545458));
#51539=CARTESIAN_POINT('Ctrl Pts',(4.91716859158436,-1.94375352019086,386.231749669999));
#51540=CARTESIAN_POINT('Ctrl Pts',(3.39480098979053,-4.05364662310803,386.152621794539));
#51541=CARTESIAN_POINT('Ctrl Pts',(1.05043926306477,-5.18201718059,386.073493919079));
#51542=CARTESIAN_POINT('Ctrl Pts',(-1.54826871412865,-5.0556491862241,385.994366043619));
#51543=CARTESIAN_POINT('Ctrl Pts',(-3.772089388456,-3.70514053050835,385.91523816816));
#51544=CARTESIAN_POINT('Ctrl Pts',(-5.08256187967811,-1.45749423482943,
385.836110292699));
#51545=CARTESIAN_POINT('Ctrl Pts',(-5.16237725218749,1.14305984594648,385.75698241724));
#51546=CARTESIAN_POINT('Ctrl Pts',(-3.99220955212729,3.46684115546438,385.67785454178));
#51547=CARTESIAN_POINT('Ctrl Pts',(-1.85539526299902,4.95118502212943,385.59872666632));
#51548=CARTESIAN_POINT('Ctrl Pts',(0.73067187193628,5.23668247279509,385.51959879086));
#51549=CARTESIAN_POINT('Ctrl Pts',(3.13981906729605,4.25420508790564,385.440470915401));
#51550=CARTESIAN_POINT('Ctrl Pts',(4.78871173391359,2.24164328892807,385.361343039941));
#51551=CARTESIAN_POINT('Ctrl Pts',(5.27809816640793,-0.313694837508304,
385.282215164481));
#51552=CARTESIAN_POINT('Ctrl Pts',(4.48948164772799,-2.79307702006795,385.203087289022));
#51553=CARTESIAN_POINT('Ctrl Pts',(2.61381244185943,-4.59616244535579,385.123959413562));
#51554=CARTESIAN_POINT('Ctrl Pts',(0.105252389857621,-5.28636421747,385.044831538102));
#51555=CARTESIAN_POINT('Ctrl Pts',(-2.42879276314368,-4.69656155277656,
384.965703662642));
#51556=CARTESIAN_POINT('Ctrl Pts',(-4.3747464822184,-2.96956527485689,384.886575787182));
#51557=CARTESIAN_POINT('Ctrl Pts',(-5.26142871019096,-0.5235385686808,384.807447911723));
#51558=CARTESIAN_POINT('Ctrl Pts',(-4.87414421624611,2.04925422155296,384.728320036263));
#51559=CARTESIAN_POINT('Ctrl Pts',(-3.30666744538294,4.12585447040522,384.649192160803));
#51560=CARTESIAN_POINT('Ctrl Pts',(-0.93853660926441,5.20344825460853,384.570064285343));
#51561=CARTESIAN_POINT('Ctrl Pts',(1.65684512644118,5.02111431181428,384.490936409884));
#51562=CARTESIAN_POINT('Ctrl Pts',(3.85104960199139,3.62300174831864,384.411808534424));
#51563=CARTESIAN_POINT('Ctrl Pts',(5.11278700298303,1.34764007340457,384.332680658964));
#51564=CARTESIAN_POINT('Ctrl Pts',(5.13654877856401,-1.25403004379905,384.253552783504));
#51565=CARTESIAN_POINT('Ctrl Pts',(3.91658141328989,-3.55205781743347,384.174424908044));
#51566=CARTESIAN_POINT('Ctrl Pts',(1.74827954439566,-4.99001436270134,384.095297032584));
#51567=CARTESIAN_POINT('Ctrl Pts',(-0.843338895500463,-5.21972261836337,
384.016169157125));
#51568=CARTESIAN_POINT('Ctrl Pts',(-3.23075696562154,-4.18556258278454,
383.937041281665));
#51569=CARTESIAN_POINT('Ctrl Pts',(-4.8359014200548,-2.1379387645183,383.857913406205));
#51570=CARTESIAN_POINT('Ctrl Pts',(-5.27011344929143,0.427351069865941,
383.778785530745));
#51571=CARTESIAN_POINT('Ctrl Pts',(-4.42825589269063,2.88916500985471,383.699657655286));
#51572=CARTESIAN_POINT('Ctrl Pts',(-2.51417043865664,4.65141609735177,383.620529779826));
#51573=CARTESIAN_POINT('Ctrl Pts',(0.00867922154690349,5.28740478651213,
383.541401904366));
#51574=CARTESIAN_POINT('Ctrl Pts',(2.52942735381344,4.6431370825228,383.462274028906));
#51575=CARTESIAN_POINT('Ctrl Pts',(4.43771707378134,2.87461160478899,383.383146153446));
#51576=CARTESIAN_POINT('Ctrl Pts',(5.27148802998996,0.410047137522666,383.304018277987));
#51577=CARTESIAN_POINT('Ctrl Pts',(4.82885656869832,-2.15380336712922,383.224890402527));
#51578=CARTESIAN_POINT('Ctrl Pts',(3.2169984748157,-4.19614650820864,383.145762527067));
#51579=CARTESIAN_POINT('Ctrl Pts',(0.82619815304806,-5.22246314656389,383.066634651607));
#51580=CARTESIAN_POINT('Ctrl Pts',(-1.76465219517988,-4.98424792073636,
382.987506776148));
#51581=CARTESIAN_POINT('Ctrl Pts',(-3.92822160960685,-3.5391806525149,382.908378900688));
#51582=CARTESIAN_POINT('Ctrl Pts',(-5.14063804209515,-1.23716014544694,
382.829251025228));
#51583=CARTESIAN_POINT('Ctrl Pts',(-5.10833518714595,1.36441794223199,382.750123149768));
#51584=CARTESIAN_POINT('Ctrl Pts',(-3.83913463932894,3.63562510806912,382.670995274309));
#51585=CARTESIAN_POINT('Ctrl Pts',(-1.64035202533435,5.0265266276326,382.591867398849));
#51586=CARTESIAN_POINT('Ctrl Pts',(0.955614320991023,5.2003390249901,382.512739523389));
#51587=CARTESIAN_POINT('Ctrl Pts',(3.32019468624774,4.11497654315675,382.433611647929));
#51588=CARTESIAN_POINT('Ctrl Pts',(4.8808455917412,2.03324150432223,382.354483772469));
#51589=CARTESIAN_POINT('Ctrl Pts',(5.25968159463003,-0.540808864968189,
382.27535589701));
#51590=CARTESIAN_POINT('Ctrl Pts',(4.36497391033337,-2.98391143759783,382.19622802155));
#51591=CARTESIAN_POINT('Ctrl Pts',(2.41336099931917,-4.70450989926509,382.11710014609));
#51592=CARTESIAN_POINT('Ctrl Pts',(-0.122606802820077,-5.28599018890692,
382.03797227063));
#51593=CARTESIAN_POINT('Ctrl Pts',(-2.6288874239146,-4.58755660648474,381.958844395171));
#51594=CARTESIAN_POINT('Ctrl Pts',(-4.49862704479611,-2.77832313044165,
381.879716519711));
#51595=CARTESIAN_POINT('Ctrl Pts',(-5.27909957396784,-0.296365304059962,
381.800588644251));
#51596=CARTESIAN_POINT('Ctrl Pts',(-4.78132667791946,2.25735241031028,381.721460768791));
#51597=CARTESIAN_POINT('Ctrl Pts',(-3.12583571520092,4.26449009693918,381.642332893332));
#51598=CARTESIAN_POINT('Ctrl Pts',(-0.713476057932961,5.23905302703404,
381.563205017871));
#51599=CARTESIAN_POINT('Ctrl Pts',(1.87163986094335,4.94506713162178,381.484077142412));
#51600=CARTESIAN_POINT('Ctrl Pts',(4.00356957706116,3.45371616479241,381.404949266952));
#51601=CARTESIAN_POINT('Ctrl Pts',(5.16610206459392,1.12610575148009,381.325821391492));
#51602=CARTESIAN_POINT('Ctrl Pts',(5.07774957870228,-1.47417228345499,381.246693516033));
#51603=CARTESIAN_POINT('Ctrl Pts',(3.75990519207135,-3.71750422352859,381.167565640573));
#51604=CARTESIAN_POINT('Ctrl Pts',(1.53166282114666,-5.06070486272762,381.088437765113));
#51605=CARTESIAN_POINT('Ctrl Pts',(-1.0674460141586,-5.17854069330105,381.009309889653));
#51606=CARTESIAN_POINT('Ctrl Pts',(-3.40809069944175,-4.04247974511891,
380.930182014193));
#51607=CARTESIAN_POINT('Ctrl Pts',(-4.92352337948473,-1.92760012372517,
380.851054138734));
#51608=CARTESIAN_POINT('Ctrl Pts',(-5.24680744637695,0.654015539541282,
380.771926263274));
#51609=CARTESIAN_POINT('Ctrl Pts',(-4.29966508516876,3.07727230850615,380.692798387814));
#51610=CARTESIAN_POINT('Ctrl Pts',(-2.31143093395199,4.75541919738815,380.613670512354));
#51611=CARTESIAN_POINT('Ctrl Pts',(0.236477452546483,5.28212108151216,380.534542636895));
#51612=CARTESIAN_POINT('Ctrl Pts',(2.7271267899117,4.52984593303835,380.455414761435));
#51613=CARTESIAN_POINT('Ctrl Pts',(4.55744811217567,2.68074456264382,380.376286885975));
#51614=CARTESIAN_POINT('Ctrl Pts',(5.28425980776137,0.182545855597361,380.297159010515));
#51615=CARTESIAN_POINT('Ctrl Pts',(4.73157661405697,-2.35985326887651,380.218031135055));
#51616=CARTESIAN_POINT('Ctrl Pts',(3.03322149728047,-4.33085350176541,380.138903259596));
#51617=CARTESIAN_POINT('Ctrl Pts',(0.600422665576261,-5.25321019263273,
380.059775384136));
#51618=CARTESIAN_POINT('Ctrl Pts',(-1.97775844481349,-4.90359013777528,
379.980647508676));
#51619=CARTESIAN_POINT('Ctrl Pts',(-4.07705851709219,-3.36664796994342,
379.901519633216));
#51620=CARTESIAN_POINT('Ctrl Pts',(-5.18916724645199,-1.01452845877678,
379.822391757756));
#51621=CARTESIAN_POINT('Ctrl Pts',(-5.04480615543027,1.58324210386498,379.743263882297));
#51622=CARTESIAN_POINT('Ctrl Pts',(-3.67892986111526,3.7976571438602,379.664136006837));
#51623=CARTESIAN_POINT('Ctrl Pts',(-1.42226240084736,5.09253319757995,379.585008131377));
#51624=CARTESIAN_POINT('Ctrl Pts',(1.17878204679748,5.15433774518764,379.505880255918));
#51625=CARTESIAN_POINT('Ctrl Pts',(3.49440419135096,3.9681058520139,379.426752380457));
#51626=CARTESIAN_POINT('Ctrl Pts',(4.96391496617568,1.82106367650753,379.347624504998));
#51627=CARTESIAN_POINT('Ctrl Pts',(5.2314969825461,-0.766918526917405,379.268496629538));
#51628=CARTESIAN_POINT('Ctrl Pts',(4.23235974285854,-3.16920427116154,379.189368754078));
#51629=CARTESIAN_POINT('Ctrl Pts',(2.20842757301423,-4.80412035237133,379.110240878619));
#51630=CARTESIAN_POINT('Ctrl Pts',(-0.350238295746339,-5.27579926091873,
379.031113003158));
#51631=CARTESIAN_POINT('Ctrl Pts',(-2.82409983509395,-4.47003185970082,
378.951985127699));
#51632=CARTESIAN_POINT('Ctrl Pts',(-4.61415296279982,-2.58192121126957,
378.872857252239));
#51633=CARTESIAN_POINT('Ctrl Pts',(-5.28696633525482,-0.0686416433394937,
378.793729376779));
#51634=CARTESIAN_POINT('Ctrl Pts',(-4.67962947817872,2.46125834732535,378.71460150132));
#51635=CARTESIAN_POINT('Ctrl Pts',(-2.9391988257698,4.39520590733944,378.63547362586));
#51636=CARTESIAN_POINT('Ctrl Pts',(-0.487090471470337,5.2649280695866,378.5563457504));
#51637=CARTESIAN_POINT('Ctrl Pts',(2.08295867142411,4.85983619872698,378.47721787494));
#51638=CARTESIAN_POINT('Ctrl Pts',(4.1486543056634,3.27801649742928,378.398089999481));
#51639=CARTESIAN_POINT('Ctrl Pts',(5.20982287752563,0.902480077413658,378.318962124021));
#51640=CARTESIAN_POINT('Ctrl Pts',(5.00952021436078,-1.69157675771122,378.239834248561));
#51641=CARTESIAN_POINT('Ctrl Pts',(3.59624624674644,-3.8760466506584,378.160706373101));
#51642=CARTESIAN_POINT('Ctrl Pts',(1.31220156369858,-5.12199685294173,378.081578497641));
#51643=CARTESIAN_POINT('Ctrl Pts',(-1.28957072085835,-5.12774141910675,
378.002450622182));
#51644=CARTESIAN_POINT('Ctrl Pts',(-3.57909508295452,-3.89188939879962,
377.923322746722));
#51645=CARTESIAN_POINT('Ctrl Pts',(-5.00200159628448,-1.71368163206748,
377.844194871262));
#51646=CARTESIAN_POINT('Ctrl Pts',(-5.21375731243622,0.879465401443313,
377.765066995802));
#51647=CARTESIAN_POINT('Ctrl Pts',(-4.16308913613231,3.25966463764834,377.685939120343));
#51648=CARTESIAN_POINT('Ctrl Pts',(-2.1043987453421,4.85059075019948,377.606811244883));
#51649=CARTESIAN_POINT('Ctrl Pts',(0.463836508427624,5.26702766261653,377.527683369423));
#51650=CARTESIAN_POINT('Ctrl Pts',(2.91976153075723,4.40814216068722,377.448555493963));
#51651=CARTESIAN_POINT('Ctrl Pts',(4.66871526619766,2.48189896419878,377.369427618503));
#51652=CARTESIAN_POINT('Ctrl Pts',(5.28721789969248,-0.0452944421492617,
377.290299743044));
#51653=CARTESIAN_POINT('Ctrl Pts',(4.62550939154664,-2.56152055897115,377.211171867584));
#51654=CARTESIAN_POINT('Ctrl Pts',(2.84381135938942,-4.45751743210561,377.132043992124));
#51655=CARTESIAN_POINT('Ctrl Pts',(0.373532100567371,-5.27420121678766,
377.052916116664));
#51656=CARTESIAN_POINT('Ctrl Pts',(-2.18719169184094,-4.81382563128935,
376.973788241204));
#51657=CARTESIAN_POINT('Ctrl Pts',(-4.21832369780876,-3.18786290260816,
376.894660365745));
#51658=CARTESIAN_POINT('Ctrl Pts',(-5.2280593665279,-0.790012636213206,
376.815532490285));
#51659=CARTESIAN_POINT('Ctrl Pts',(-4.97190814025518,1.79912594061044,376.736404614825));
#51660=CARTESIAN_POINT('Ctrl Pts',(-3.51189274247934,3.95263634434836,376.657276739365));
#51661=CARTESIAN_POINT('Ctrl Pts',(-1.20153141562281,5.1490821475793,376.578148863906));
#51662=CARTESIAN_POINT('Ctrl Pts',(1.39976059245402,5.09876406487689,376.499020988446));
#51663=CARTESIAN_POINT('Ctrl Pts',(3.66212404867255,3.81386577598244,376.419893112986));
#51664=CARTESIAN_POINT('Ctrl Pts',(5.03776558457334,1.60550385251465,376.340765237526));
#51665=CARTESIAN_POINT('Ctrl Pts',(5.19359667332446,-0.99160390296118,376.261637362067));
#51666=CARTESIAN_POINT('Ctrl Pts',(4.09188543028651,-3.34861140308599,376.182509486607));
#51667=CARTESIAN_POINT('Ctrl Pts',(1.99939275591558,-4.89480881330613,376.103381611147));
#51668=CARTESIAN_POINT('Ctrl Pts',(-0.577219342064538,-5.2558103583336,
376.024253735687));
#51669=CARTESIAN_POINT('Ctrl Pts',(-3.01406745721832,-4.34420557675964,
375.945125860227));
#51670=CARTESIAN_POINT('Ctrl Pts',(-4.72110968654987,-2.38072426020005,
375.865997984768));
#51671=CARTESIAN_POINT('Ctrl Pts',(-5.28501438473626,0.159209483211192,
375.786870109308));
#51672=CARTESIAN_POINT('Ctrl Pts',(-4.56924148341307,2.66059337382158,375.707742233848));
#51673=CARTESIAN_POINT('Ctrl Pts',(-2.74710339271414,4.51775908713646,375.628614358388));
#51674=CARTESIAN_POINT('Ctrl Pts',(-0.25980027835232,5.28102544478076,375.549486482929));
#51675=CARTESIAN_POINT('Ctrl Pts',(2.29040909674433,4.76557955369675,375.470358607468));
#51676=CARTESIAN_POINT('Ctrl Pts',(4.28603436317887,3.09622956904483,375.391230732009));
#51677=CARTESIAN_POINT('Ctrl Pts',(5.24386820297344,0.677177255244125,375.312102856549));
#51678=CARTESIAN_POINT('Ctrl Pts',(4.93198748823577,-1.90583737857549,375.232974981089));
#51679=CARTESIAN_POINT('Ctrl Pts',(3.42590832840442,-4.02739560248487,375.153847105629));
#51680=CARTESIAN_POINT('Ctrl Pts',(1.09030376033057,-5.1737660638094,375.07471923017));
#51681=CARTESIAN_POINT('Ctrl Pts',(-1.50930126232148,-5.06744133910014,
374.99559135471));
#51682=CARTESIAN_POINT('Ctrl Pts',(-3.74345011231245,-3.7340250124542,374.91646347925));
#51683=CARTESIAN_POINT('Ctrl Pts',(-5.07118953303831,-1.49668421879837,
374.83733560379));
#51684=CARTESIAN_POINT('Ctrl Pts',(-5.17098566641861,1.10346413672945,374.758207728331));
#51685=CARTESIAN_POINT('Ctrl Pts',(-4.40267566674078,2.65797789149901,374.705455811358));
#51686=CARTESIAN_POINT('Ctrl Pts',(-3.85627053850387,3.29705846079003,374.679079852871));
#51687=CARTESIAN_POINT('Ctrl Pts',(-1.2650852794265,-4.72177922709115,400.106973382376));
#51688=CARTESIAN_POINT('Ctrl Pts',(-2.04760230627562,-4.51212292510067,
400.08059742389));
#51689=CARTESIAN_POINT('Ctrl Pts',(-3.50558628380115,-3.69634492177698,
400.027845506916));
#51690=CARTESIAN_POINT('Ctrl Pts',(-4.84423972345866,-1.57661725067267,
399.948717631457));
#51691=CARTESIAN_POINT('Ctrl Pts',(-5.0096862523777,0.92455742070055,399.869589755997));
#51692=CARTESIAN_POINT('Ctrl Pts',(-3.9622375540088,3.20202818303723,399.790461880537));
#51693=CARTESIAN_POINT('Ctrl Pts',(-1.95534398901843,4.70410781476347,399.711334005077));
#51694=CARTESIAN_POINT('Ctrl Pts',(0.524977181208032,5.06720185162811,399.632206129618));
#51695=CARTESIAN_POINT('Ctrl Pts',(2.87819629981243,4.2033413524507,399.553078254158));
#51696=CARTESIAN_POINT('Ctrl Pts',(4.53450261129871,2.32172008778426,399.473950378698));
#51697=CARTESIAN_POINT('Ctrl Pts',(5.09285792630992,-0.122070466194823,
399.394822503238));
#51698=CARTESIAN_POINT('Ctrl Pts',(4.41806180230403,-2.5363019515078,399.315694627778));
#51699=CARTESIAN_POINT('Ctrl Pts',(2.67350672576957,-4.3364112842173,399.236566752319));
#51700=CARTESIAN_POINT('Ctrl Pts',(0.281606541856066,-5.08653095966945,
399.157438876859));
#51701=CARTESIAN_POINT('Ctrl Pts',(-2.17847980551824,-4.60503265524259,
399.078311001399));
#51702=CARTESIAN_POINT('Ctrl Pts',(-4.1110838687323,-3.00850283765647,398.999183125939));
#51703=CARTESIAN_POINT('Ctrl Pts',(-5.04825788999868,-0.683514555327269,
398.920055250479));
#51704=CARTESIAN_POINT('Ctrl Pts',(-4.76308094287924,1.80697533276996,398.84092737502));
#51705=CARTESIAN_POINT('Ctrl Pts',(-3.32460382095413,3.85993643987858,398.76179949956));
#51706=CARTESIAN_POINT('Ctrl Pts',(-1.08112964449127,4.97827867803806,398.6826716241));
#51707=CARTESIAN_POINT('Ctrl Pts',(1.4241219451236,4.89121422375072,398.603543748641));
#51708=CARTESIAN_POINT('Ctrl Pts',(3.58454628917626,3.6198242774857,398.52441587318));
#51709=CARTESIAN_POINT('Ctrl Pts',(4.87703286664207,1.4719545906142,398.445287997721));
#51710=CARTESIAN_POINT('Ctrl Pts',(4.98862772878014,-1.03232421377308,398.366160122261));
#51711=CARTESIAN_POINT('Ctrl Pts',(3.89231005153748,-3.28664302317114,398.287032246801));
#51712=CARTESIAN_POINT('Ctrl Pts',(1.853534773828,-4.7451563452711,398.207904371342));
#51713=CARTESIAN_POINT('Ctrl Pts',(-0.634042863421179,-5.05470964015625,
398.128776495882));
#51714=CARTESIAN_POINT('Ctrl Pts',(-2.96809765493441,-4.14034976900372,
398.049648620422));
#51715=CARTESIAN_POINT('Ctrl Pts',(-4.58347737773795,-2.22347363975469,
397.970520744962));
#51716=CARTESIAN_POINT('Ctrl Pts',(-5.08904492375008,0.231779341134317,
397.891392869503));
#51717=CARTESIAN_POINT('Ctrl Pts',(-4.36238559065476,2.6309108417746,397.812264994043));
#51718=CARTESIAN_POINT('Ctrl Pts',(-2.57944774904339,4.39301140550268,397.733137118583));
#51719=CARTESIAN_POINT('Ctrl Pts',(-0.171939895328258,5.09141793327901,
397.654009243123));
#51720=CARTESIAN_POINT('Ctrl Pts',(2.27720032040928,4.55702299748958,397.574881367663));
#51721=CARTESIAN_POINT('Ctrl Pts',(4.17495466984747,2.91922136941339,397.495753492203));
#51722=CARTESIAN_POINT('Ctrl Pts',(5.06181376480896,0.574579245458329,397.416625616744));
#51723=CARTESIAN_POINT('Ctrl Pts',(4.72303954910339,-1.90918760642483,397.337497741284));
#51724=CARTESIAN_POINT('Ctrl Pts',(3.24066051742776,-3.93067669870034,397.258369865824));
#51725=CARTESIAN_POINT('Ctrl Pts',(0.973609891088484,-5.00041835038785,
397.179241990364));
#51726=CARTESIAN_POINT('Ctrl Pts',(-1.52918404181197,-4.85939256133815,
397.100114114905));
#51727=CARTESIAN_POINT('Ctrl Pts',(-3.66171170517574,-3.54174636120374,
397.020986239445));
#51728=CARTESIAN_POINT('Ctrl Pts',(-4.90761729027895,-1.36652567889375,
396.941858363985));
#51729=CARTESIAN_POINT('Ctrl Pts',(-4.965225654969,1.13957627834147,396.862730488525));
#51730=CARTESIAN_POINT('Ctrl Pts',(-3.82058789989522,3.3697489517908,396.783602613066));
#51731=CARTESIAN_POINT('Ctrl Pts',(-1.7508588605474,4.78399343115808,396.704474737606));
#51732=CARTESIAN_POINT('Ctrl Pts',(0.742811287950349,5.03987413428296,396.625346862146));
#51733=CARTESIAN_POINT('Ctrl Pts',(3.05662214087683,4.07543384031964,396.546218986686));
#51734=CARTESIAN_POINT('Ctrl Pts',(4.63032320548468,2.12419559167018,396.467091111227));
#51735=CARTESIAN_POINT('Ctrl Pts',(5.08286916176923,-0.341380994281065,
396.387963235767));
#51736=CARTESIAN_POINT('Ctrl Pts',(4.30468359613617,-2.72429789782194,396.308835360307));
#51737=CARTESIAN_POINT('Ctrl Pts',(2.48419109223004,-4.44757175503734,396.229707484847));
#51738=CARTESIAN_POINT('Ctrl Pts',(0.0621933781031742,-5.09394070270169,
396.150579609387));
#51739=CARTESIAN_POINT('Ctrl Pts',(-2.37486341947636,-4.50689734049423,
396.071451733928));
#51740=CARTESIAN_POINT('Ctrl Pts',(-4.23688686924074,-2.82858437317615,
395.992323858468));
#51741=CARTESIAN_POINT('Ctrl Pts',(-5.07301922112011,-0.46537713853058,
395.913195983008));
#51742=CARTESIAN_POINT('Ctrl Pts',(-4.68080504901513,2.01051336529637,395.834068107548));
#51743=CARTESIAN_POINT('Ctrl Pts',(-3.15521243681498,3.99959177635531,395.754940232089));
#51744=CARTESIAN_POINT('Ctrl Pts',(-0.865638049608238,5.0202361165578,395.675812356629));
#51745=CARTESIAN_POINT('Ctrl Pts',(1.63353607355812,4.82531447631191,395.596684481169));
#51746=CARTESIAN_POINT('Ctrl Pts',(3.73717683280492,3.46202386174144,395.517556605709));
#51747=CARTESIAN_POINT('Ctrl Pts',(4.93592289877338,1.26046223120153,395.43842873025));
#51748=CARTESIAN_POINT('Ctrl Pts',(4.93951801594962,-1.24629918921186,395.35930085479));
#51749=CARTESIAN_POINT('Ctrl Pts',(3.74709168700367,-3.45129016283895,395.28017297933));
#51750=CARTESIAN_POINT('Ctrl Pts',(1.64736994911874,-4.82060910566927,395.20104510387));
#51751=CARTESIAN_POINT('Ctrl Pts',(-0.851234793642623,-5.0226984007616,
395.12191722841));
#51752=CARTESIAN_POINT('Ctrl Pts',(-3.14372730731715,-4.00862551458096,
395.04278935295));
#51753=CARTESIAN_POINT('Ctrl Pts',(-4.67501897747406,-2.02393118933878,
394.963661477491));
#51754=CARTESIAN_POINT('Ctrl Pts',(-5.07433320772034,0.450824129730827,
394.884533602031));
#51755=CARTESIAN_POINT('Ctrl Pts',(-4.24498275416411,2.81641994662909,394.805405726571));
#51756=CARTESIAN_POINT('Ctrl Pts',(-2.38778091996604,4.50006690807671,394.726277851111));
#51757=CARTESIAN_POINT('Ctrl Pts',(0.0475820181493076,5.09409813906934,
394.647149975652));
#51758=CARTESIAN_POINT('Ctrl Pts',(2.47142376857538,4.45467893961412,394.568022100192));
#51759=CARTESIAN_POINT('Ctrl Pts',(4.29685170208089,2.73663394505832,394.488894224732));
#51760=CARTESIAN_POINT('Ctrl Pts',(5.08186905910887,0.355958937228547,394.409766349272));
#51761=CARTESIAN_POINT('Ctrl Pts',(4.63639705230557,-2.11090555740732,394.330638473812));
#51762=CARTESIAN_POINT('Ctrl Pts',(3.06829925703676,-4.06664967364888,394.251510598353));
#51763=CARTESIAN_POINT('Ctrl Pts',(0.757264255609957,-5.037722773843,394.172382722893));
#51764=CARTESIAN_POINT('Ctrl Pts',(-1.73712958511388,-4.78899579279863,
394.093254847433));
#51765=CARTESIAN_POINT('Ctrl Pts',(-3.81090663047816,-3.38069379753602,
394.014126971973));
#51766=CARTESIAN_POINT('Ctrl Pts',(-4.96193654859164,-1.15381349735189,
393.934999096513));
#51767=CARTESIAN_POINT('Ctrl Pts',(-4.91151674888844,1.35244339042685,393.855871221054));
#51768=CARTESIAN_POINT('Ctrl Pts',(-3.67185554026823,3.53122879325631,393.776743345594));
#51769=CARTESIAN_POINT('Ctrl Pts',(-1.54311609384367,4.85498636659688,393.697615470134));
#51770=CARTESIAN_POINT('Ctrl Pts',(0.959263034860399,5.00319041501234,393.618487594674));
#51771=CARTESIAN_POINT('Ctrl Pts',(3.22937270762551,3.93995581373248,393.539359719215));
#51772=CARTESIAN_POINT('Ctrl Pts',(4.71754393956094,1.92272698978111,393.460231843755));
#51773=CARTESIAN_POINT('Ctrl Pts',(5.06344102520928,-0.560057928386485,
393.381103968295));
#51774=CARTESIAN_POINT('Ctrl Pts',(4.18331078637565,-2.90723421201562,393.301976092835));
#51775=CARTESIAN_POINT('Ctrl Pts',(2.29026199958981,-4.55047248889121,393.222848217376));
#51776=CARTESIAN_POINT('Ctrl Pts',(-0.157335320049481,-5.0918901692776,
393.143720341916));
#51777=CARTESIAN_POINT('Ctrl Pts',(-2.5668365306344,-4.40039204207098,393.064592466456));
#51778=CARTESIAN_POINT('Ctrl Pts',(-4.35482132414875,-2.6434127815497,392.985464590996));
#51779=CARTESIAN_POINT('Ctrl Pts',(-5.08835916941954,-0.24637544907113,
392.906336715536));
#51780=CARTESIAN_POINT('Ctrl Pts',(-4.58983617949401,2.21031756639828,392.827208840077));
#51781=CARTESIAN_POINT('Ctrl Pts',(-2.97996133557448,4.13181925275079,392.748080964617));
#51782=CARTESIAN_POINT('Ctrl Pts',(-0.648538831649752,5.05287020244567,
392.668953089157));
#51783=CARTESIAN_POINT('Ctrl Pts',(1.83991647361136,4.75045337510584,392.589825213697));
#51784=CARTESIAN_POINT('Ctrl Pts',(3.88286686231846,3.29779393359108,392.510697338238));
#51785=CARTESIAN_POINT('Ctrl Pts',(4.98564616049109,1.04662899888231,392.431569462778));
#51786=CARTESIAN_POINT('Ctrl Pts',(4.88123485596325,-1.45795959472489,392.352441587318));
#51787=CARTESIAN_POINT('Ctrl Pts',(3.59491439502781,-3.60952772414103,392.273313711858));
#51788=CARTESIAN_POINT('Ctrl Pts',(1.43814570421584,-4.88710925111834,392.194185836399));
#51789=CARTESIAN_POINT('Ctrl Pts',(-1.06684584950233,-4.98135923542166,
392.115057960939));
#51790=CARTESIAN_POINT('Ctrl Pts',(-3.31351857300444,-3.86945662403335,
392.035930085479));
#51791=CARTESIAN_POINT('Ctrl Pts',(-4.75787834559899,-1.82062998640609,
391.956802210019));
#51792=CARTESIAN_POINT('Ctrl Pts',(-5.05019767193907,0.669031668355122,
391.877674334559));
#51793=CARTESIAN_POINT('Ctrl Pts',(-4.11969632968522,2.99669852506039,391.7985464591));
#51794=CARTESIAN_POINT('Ctrl Pts',(-2.19167961327856,4.59876509202852,391.71941858364));
#51795=CARTESIAN_POINT('Ctrl Pts',(0.267015564477117,5.08731781858062,391.64029070818));
#51796=CARTESIAN_POINT('Ctrl Pts',(2.66105740145502,4.34406185557737,391.56116283272));
#51797=CARTESIAN_POINT('Ctrl Pts',(4.4107688176863,2.54896416919641,391.48203495726));
#51798=CARTESIAN_POINT('Ctrl Pts',(5.09248653841822,0.136677558326831,391.402907081801));
#51799=CARTESIAN_POINT('Ctrl Pts',(4.54114405077152,-2.30870323105058,391.323779206341));
#51800=CARTESIAN_POINT('Ctrl Pts',(2.89023969147757,-4.1950702526571,391.244651330881));
#51801=CARTESIAN_POINT('Ctrl Pts',(0.539512263560586,-5.06567136877124,
391.165523455421));
#51802=CARTESIAN_POINT('Ctrl Pts',(-1.94184901073189,-4.70970512011533,
391.086395579962));
#51803=CARTESIAN_POINT('Ctrl Pts',(-3.95302411413336,-3.21336276383497,
391.007267704502));
#51804=CARTESIAN_POINT('Ctrl Pts',(-5.00704072509175,-0.93895850610853,
390.928139829042));
#51805=CARTESIAN_POINT('Ctrl Pts',(-4.84868639834328,1.56279880645007,390.849011953582));
#51806=CARTESIAN_POINT('Ctrl Pts',(-3.51630397832454,3.68615059797345,390.769884078122));
#51807=CARTESIAN_POINT('Ctrl Pts',(-1.33250752244617,4.91696284321382,390.690756202663));
#51808=CARTESIAN_POINT('Ctrl Pts',(1.17393328229752,4.95721499913359,390.611628327203));
#51809=CARTESIAN_POINT('Ctrl Pts',(3.39612583095411,3.79716068125213,390.532500451743));
#51810=CARTESIAN_POINT('Ctrl Pts',(4.79600346661011,1.71768758718946,390.453372576283));
#51811=CARTESIAN_POINT('Ctrl Pts',(5.03460929736123,-0.777694748500222,
390.374244700824));
#51812=CARTESIAN_POINT('Ctrl Pts',(4.05416892298729,-3.08477134368254,390.295116825364));
#51813=CARTESIAN_POINT('Ctrl Pts',(2.09207953702197,-4.64492229318153,390.215988949904));
#51814=CARTESIAN_POINT('Ctrl Pts',(-0.376571822235509,-5.08038321011508,
390.136861074444));
#51815=CARTESIAN_POINT('Ctrl Pts',(-2.75404263028444,-4.28571453663178,
390.057733198984));
#51816=CARTESIAN_POINT('Ctrl Pts',(-4.46466820389571,-2.45333196450126,
389.978605323525));
#51817=CARTESIAN_POINT('Ctrl Pts',(-5.09424924959213,-0.0269162023862396,
389.899477448065));
#51818=CARTESIAN_POINT('Ctrl Pts',(-4.49034327596192,2.40601686672071,389.820349572605));
#51819=CARTESIAN_POINT('Ctrl Pts',(-2.79917598631673,4.25637330324171,389.741221697145));
#51820=CARTESIAN_POINT('Ctrl Pts',(-0.430235177009337,5.07612032869441,
389.662093821686));
#51821=CARTESIAN_POINT('Ctrl Pts',(2.04287986486846,4.66676994897283,389.582965946226));
#51822=CARTESIAN_POINT('Ctrl Pts',(4.02134580893056,3.12743949324644,389.503838070766));
#51823=CARTESIAN_POINT('Ctrl Pts',(5.02611030798847,0.830852015014124,389.424710195306));
#51824=CARTESIAN_POINT('Ctrl Pts',(4.81388648966003,-1.66691234430295,389.345582319847));
#51825=CARTESIAN_POINT('Ctrl Pts',(3.43606079231419,-3.76106183549833,389.266454444386));
#51826=CARTESIAN_POINT('Ctrl Pts',(1.22625060082997,-4.94453328059232,389.187326568927));
#51827=CARTESIAN_POINT('Ctrl Pts',(-1.28047560800195,-4.93076891734271,
389.108198693467));
#51828=CARTESIAN_POINT('Ctrl Pts',(-3.4771561234157,-3.72310155546604,389.029070818007));
#51829=CARTESIAN_POINT('Ctrl Pts',(-4.8319015994811,-1.61394759265993,388.949942942547));
#51830=CARTESIAN_POINT('Ctrl Pts',(-5.01668313982022,0.88599671193773,388.870815067088));
#51831=CARTESIAN_POINT('Ctrl Pts',(-3.98675899344041,3.17141177193107,388.791687191628));
#51832=CARTESIAN_POINT('Ctrl Pts',(-1.99150801936634,4.68892265960108,388.712559316169));
#51833=CARTESIAN_POINT('Ctrl Pts',(0.485953221700427,5.07108956391423,388.633431440708));
#51834=CARTESIAN_POINT('Ctrl Pts',(2.84574904013097,4.2253771783729,388.554303565249));
#51835=CARTESIAN_POINT('Ctrl Pts',(4.51649445500228,2.35656057355938,388.475175689789));
#51836=CARTESIAN_POINT('Ctrl Pts',(5.09364648443963,-0.0828576518904476,
388.396047814329));
#51837=CARTESIAN_POINT('Ctrl Pts',(4.43745744402291,-2.50221328655385,388.316919938869));
#51838=CARTESIAN_POINT('Ctrl Pts',(2.70681250483858,-4.31569993889408,388.23779206341));
#51839=CARTESIAN_POINT('Ctrl Pts',(0.320758313989414,-5.08421223031922,
388.15866418795));
#51840=CARTESIAN_POINT('Ctrl Pts',(-2.14296212310374,-4.62166779830222,
388.07953631249));
#51841=CARTESIAN_POINT('Ctrl Pts',(-4.08780022204497,-3.04006401964993,
388.00040843703));
#51842=CARTESIAN_POINT('Ctrl Pts',(-5.04284605436382,-0.722359724035205,
387.921280561571));
#51843=CARTESIAN_POINT('Ctrl Pts',(-4.7768512889894,1.77025186394512,387.842152686111));
#51844=CARTESIAN_POINT('Ctrl Pts',(-3.35422209731677,3.83422665224591,387.763024810651));
#51845=CARTESIAN_POINT('Ctrl Pts',(-1.11942427896961,4.96980776112863,387.683896935191));
#51846=CARTESIAN_POINT('Ctrl Pts',(1.38642335448793,4.90203327008818,387.604769059731));
#51847=CARTESIAN_POINT('Ctrl Pts',(3.55657182458215,3.64731363547327,387.525641184271));
#51848=CARTESIAN_POINT('Ctrl Pts',(4.86555607518393,1.50945817370396,387.446513308812));
#51849=CARTESIAN_POINT('Ctrl Pts',(4.99642752319251,-0.993887269465375,
387.367385433352));
#51850=CARTESIAN_POINT('Ctrl Pts',(3.9174978423384,-3.25657957897469,387.288257557892));
#51851=CARTESIAN_POINT('Ctrl Pts',(1.89001175993966,-4.73074576004784,387.209129682432));
#51852=CARTESIAN_POINT('Ctrl Pts',(-0.595108972441489,-5.05944119541285,
387.130001806973));
#51853=CARTESIAN_POINT('Ctrl Pts',(-2.93613404781291,-4.1630777979993,387.050873931513));
#51854=CARTESIAN_POINT('Ctrl Pts',(-4.5662235058762,-2.2586949314382,386.971746056053));
#51855=CARTESIAN_POINT('Ctrl Pts',(-5.09067852285014,0.192593031839733,
386.892618180593));
#51856=CARTESIAN_POINT('Ctrl Pts',(-4.38251111209279,2.59724782246595,386.813490305134));
#51857=CARTESIAN_POINT('Ctrl Pts',(-2.61319213533106,4.37302261173721,386.734362429674));
#51858=CARTESIAN_POINT('Ctrl Pts',(-0.211132509258637,5.08994331623203,
386.655234554214));
#51859=CARTESIAN_POINT('Ctrl Pts',(2.24204931299394,4.57441961094785,386.576106678754));
#51860=CARTESIAN_POINT('Ctrl Pts',(4.15235649586965,2.95127691518944,386.496978803295));
#51861=CARTESIAN_POINT('Ctrl Pts',(5.05724019309986,0.613532010751077,386.417850927834));
#51862=CARTESIAN_POINT('Ctrl Pts',(4.73759799334825,-1.872769380448,386.338723052375));
#51863=CARTESIAN_POINT('Ctrl Pts',(3.27082589451466,-3.90561107468386,386.259595176915));
#51864=CARTESIAN_POINT('Ctrl Pts',(1.01207816086419,-4.99277454880777,386.180467301455));
#51865=CARTESIAN_POINT('Ctrl Pts',(-1.49172732571618,-4.87102140055169,
386.101339425996));
#51866=CARTESIAN_POINT('Ctrl Pts',(-3.63433605836998,-3.56983211282445,
386.022211550536));
#51867=CARTESIAN_POINT('Ctrl Pts',(-4.89695126651592,-1.40426784919727,
385.943083675076));
#51868=CARTESIAN_POINT('Ctrl Pts',(-4.97385185302132,1.10131632291422,385.863955799616));
#51869=CARTESIAN_POINT('Ctrl Pts',(-3.84641763057586,3.34023521778273,385.784827924157));
#51870=CARTESIAN_POINT('Ctrl Pts',(-1.78763788776658,4.77037217427974,385.705700048697));
#51871=CARTESIAN_POINT('Ctrl Pts',(0.703988388806892,5.0454435134432,385.626572173237));
#51872=CARTESIAN_POINT('Ctrl Pts',(3.02515568373168,4.09884532375971,385.547444297777));
#51873=CARTESIAN_POINT('Ctrl Pts',(4.61383226520657,2.15978048131279,385.468316422317));
#51874=CARTESIAN_POINT('Ctrl Pts',(5.08534674297434,-0.302238982663029,
385.389188546858));
#51875=CARTESIAN_POINT('Ctrl Pts',(4.32552979408761,-2.69107634588493,385.310060671397));
#51876=CARTESIAN_POINT('Ctrl Pts',(2.51835834970871,-4.42831470441898,385.230932795938));
#51877=CARTESIAN_POINT('Ctrl Pts',(0.10140866673516,-5.09331092524616,385.151804920478));
#51878=CARTESIAN_POINT('Ctrl Pts',(-2.34009542414748,-4.5250473262503,385.072677045019));
#51879=CARTESIAN_POINT('Ctrl Pts',(-4.21498465418432,-2.86111940748926,
384.993549169558));
#51880=CARTESIAN_POINT('Ctrl Pts',(-5.06928604038651,-0.504419408492031,
384.914421294099));
#51881=CARTESIAN_POINT('Ctrl Pts',(-4.69614482970923,1.97441729057362,384.835293418639));
#51882=CARTESIAN_POINT('Ctrl Pts',(-3.18591090830761,3.97518195599239,384.756165543179));
#51883=CARTESIAN_POINT('Ctrl Pts',(-0.904262091876385,5.01342297917464,
384.677037667719));
#51884=CARTESIAN_POINT('Ctrl Pts',(1.59633862457976,4.83774770886161,384.59790979226));
#51885=CARTESIAN_POINT('Ctrl Pts',(3.71041271554213,3.4906929654818,384.5187819168));
#51886=CARTESIAN_POINT('Ctrl Pts',(4.92607259535609,1.29842546347592,384.43965404134));
#51887=CARTESIAN_POINT('Ctrl Pts',(4.94896661214932,-1.20823398841131,384.360526165881));
#51888=CARTESIAN_POINT('Ctrl Pts',(3.77355136371449,-3.42233984348858,384.281398290421));
#51889=CARTESIAN_POINT('Ctrl Pts',(1.6844339393846,-4.80778350206934,384.202270414961));
#51890=CARTESIAN_POINT('Ctrl Pts',(-0.812540913458525,-5.02910301772363,
384.123142539501));
#51891=CARTESIAN_POINT('Ctrl Pts',(-3.11277261136022,-4.03270958152043,
384.044014664041));
#51892=CARTESIAN_POINT('Ctrl Pts',(-4.65929862622416,-2.05986315336399,
383.964886788582));
#51893=CARTESIAN_POINT('Ctrl Pts',(-5.07765362058409,0.411744591087888,
383.885758913121));
#51894=CARTESIAN_POINT('Ctrl Pts',(-4.26653994885377,2.78365528824167,383.806631037662));
#51895=CARTESIAN_POINT('Ctrl Pts',(-2.42235518332661,4.48155054247207,383.727503162202));
#51896=CARTESIAN_POINT('Ctrl Pts',(0.00836226414014005,5.09431349363773,
383.648375286742));
#51897=CARTESIAN_POINT('Ctrl Pts',(2.43705492959019,4.47357386985853,383.569247411283));
#51898=CARTESIAN_POINT('Ctrl Pts',(4.27565561607469,2.76963336050998,383.490119535823));
#51899=CARTESIAN_POINT('Ctrl Pts',(5.07897800282517,0.39507258287429,383.410991660363));
#51900=CARTESIAN_POINT('Ctrl Pts',(4.65251104653713,-2.07514839487948,383.331863784903));
#51901=CARTESIAN_POINT('Ctrl Pts',(3.09951656833074,-4.04290699145606,383.252735909444));
#51902=CARTESIAN_POINT('Ctrl Pts',(0.79602613558697,-5.03174346428585,383.173608033984));
#51903=CARTESIAN_POINT('Ctrl Pts',(-1.70020867560859,-4.80222764540647,
383.094480158524));
#51904=CARTESIAN_POINT('Ctrl Pts',(-3.78476647047488,-3.40993294111337,
383.015352283064));
#51905=CARTESIAN_POINT('Ctrl Pts',(-4.9529065394344,-1.1919801636558,382.936224407604));
#51906=CARTESIAN_POINT('Ctrl Pts',(-4.92178335585094,1.31459061954267,382.857096532145));
#51907=CARTESIAN_POINT('Ctrl Pts',(-3.6989328766574,3.50285533142662,382.777968656685));
#51908=CARTESIAN_POINT('Ctrl Pts',(-1.58044783677119,4.84296237174792,382.698840781225));
#51909=CARTESIAN_POINT('Ctrl Pts',(0.920716140847871,5.01042729584046,382.619712905765));
#51910=CARTESIAN_POINT('Ctrl Pts',(3.19894414643704,3.96470128091602,382.540585030306));
#51911=CARTESIAN_POINT('Ctrl Pts',(4.70260147696606,1.95898934345174,382.461457154846));
#51912=CARTESIAN_POINT('Ctrl Pts',(5.06760272792295,-0.521059009008414,
382.382329279386));
#51913=CARTESIAN_POINT('Ctrl Pts',(4.20556896788232,-2.87494166120048,382.303201403926));
#51914=CARTESIAN_POINT('Ctrl Pts',(2.32522721453312,-4.53270540623539,382.224073528466));
#51915=CARTESIAN_POINT('Ctrl Pts',(-0.118129312060885,-5.0929505558716,
382.144945653006));
#51916=CARTESIAN_POINT('Ctrl Pts',(-2.53288280690479,-4.42002314308501,
382.065817777547));
#51917=CARTESIAN_POINT('Ctrl Pts',(-4.33434120943595,-2.67686125510947,
381.986689902087));
#51918=CARTESIAN_POINT('Ctrl Pts',(-5.08631158002599,-0.285542308273818,
381.907562026627));
#51919=CARTESIAN_POINT('Ctrl Pts',(-4.60671690485093,2.17491591963496,381.828434151168));
#51920=CARTESIAN_POINT('Ctrl Pts',(-3.01168299114604,4.10875473346396,381.749306275708));
#51921=CARTESIAN_POINT('Ctrl Pts',(-0.687420550548197,5.04772749716196,
381.670178400248));
#51922=CARTESIAN_POINT('Ctrl Pts',(1.80328924752583,4.76447770366057,381.591050524788));
#51923=CARTESIAN_POINT('Ctrl Pts',(3.85736279756143,3.32758954002893,381.511922649328));
#51924=CARTESIAN_POINT('Ctrl Pts',(4.97744063861076,1.0849813768112,381.432794773869));
#51925=CARTESIAN_POINT('Ctrl Pts',(4.89231470646681,-1.42033683040663,381.353666898409));
#51926=CARTESIAN_POINT('Ctrl Pts',(3.62259681793774,-3.58174429483572,381.274539022949));
#51927=CARTESIAN_POINT('Ctrl Pts',(1.47572786509085,-4.87589244827193,381.195411147489));
#51928=CARTESIAN_POINT('Ctrl Pts',(-1.02846384062172,-4.98942501972467,
381.11628327203));
#51929=CARTESIAN_POINT('Ctrl Pts',(-3.28363027585792,-3.89485200108939,
381.03715539657));
#51930=CARTESIAN_POINT('Ctrl Pts',(-4.74372071007927,-1.85720589157097,
380.95802752111));
#51931=CARTESIAN_POINT('Ctrl Pts',(-5.05519873204731,0.630131477096863,
380.87889964565));
#51932=CARTESIAN_POINT('Ctrl Pts',(-4.14264516258972,2.96489307662063,380.79977177019));
#51933=CARTESIAN_POINT('Ctrl Pts',(-2.22701954397005,4.58175554233269,380.720643894731));
#51934=CARTESIAN_POINT('Ctrl Pts',(0.227841507524015,5.08922274481773,380.641516019271));
#51935=CARTESIAN_POINT('Ctrl Pts',(2.6275345591372,4.36442001180692,380.562388143811));
#51936=CARTESIAN_POINT('Ctrl Pts',(4.39101418405409,2.58284616931722,380.483260268351));
#51937=CARTESIAN_POINT('Ctrl Pts',(5.09128336669755,0.175879444250141,380.404132392892));
#51938=CARTESIAN_POINT('Ctrl Pts',(4.55878366881602,-2.27367353854006,380.325004517432));
#51939=CARTESIAN_POINT('Ctrl Pts',(2.92245096161458,-4.17269460611234,380.245876641972));
#51940=CARTESIAN_POINT('Ctrl Pts',(0.578495766946718,-5.0613676557375,380.166748766512));
#51941=CARTESIAN_POINT('Ctrl Pts',(-1.90553247564304,-4.72451541252546,
380.087620891052));
#51942=CARTESIAN_POINT('Ctrl Pts',(-3.92816798724318,-3.24370099776764,
380.008493015593));
#51943=CARTESIAN_POINT('Ctrl Pts',(-4.99966350066068,-0.977478787024238,
379.929365140133));
#51944=CARTESIAN_POINT('Ctrl Pts',(-4.86057434754265,1.52542351854533,379.850237264673));
#51945=CARTESIAN_POINT('Ctrl Pts',(-3.54457863363044,3.65897010221885,379.771109389213));
#51946=CARTESIAN_POINT('Ctrl Pts',(-1.37032265027505,4.90655844080798,379.691981513754));
#51947=CARTESIAN_POINT('Ctrl Pts',(1.13573398094598,4.96610594162524,379.612853638294));
#51948=CARTESIAN_POINT('Ctrl Pts',(3.36679167625567,3.82319417602828,379.533725762834));
#51949=CARTESIAN_POINT('Ctrl Pts',(4.78263723215717,1.75456006010191,379.454597887374));
#51950=CARTESIAN_POINT('Ctrl Pts',(5.04044739265935,-0.738911348373108,
379.375470011914));
#51951=CARTESIAN_POINT('Ctrl Pts',(4.07779775117163,-3.05346776623899,379.296342136454));
#51952=CARTESIAN_POINT('Ctrl Pts',(2.1277777736305,-4.62867817470224,379.217214260995));
#51953=CARTESIAN_POINT('Ctrl Pts',(-0.337447906496721,-5.0831317914571,
379.138086385535));
#51954=CARTESIAN_POINT('Ctrl Pts',(-2.72096623545812,-4.30679029492008,
379.058958510076));
#51955=CARTESIAN_POINT('Ctrl Pts',(-4.44564822425965,-2.48763175833121,
378.979830634615));
#51956=CARTESIAN_POINT('Ctrl Pts',(-5.09389105422811,-0.0661349119291711,
378.900702759156));
#51957=CARTESIAN_POINT('Ctrl Pts',(-4.50873359586993,2.37137539423742,378.821574883696));
#51958=CARTESIAN_POINT('Ctrl Pts',(-2.83186191395806,4.23469691940223,378.742447008236));
#51959=CARTESIAN_POINT('Ctrl Pts',(-0.469302363186489,5.07265760630743,
378.663319132776));
#51960=CARTESIAN_POINT('Ctrl Pts',(2.00689088408632,4.68235932819045,378.584191257317));
#51961=CARTESIAN_POINT('Ctrl Pts',(3.99714916166288,3.15830626734308,378.505063381856));
#51962=CARTESIAN_POINT('Ctrl Pts',(5.01956480656533,0.869522312313901,378.425935506397));
#51963=CARTESIAN_POINT('Ctrl Pts',(4.82657701747544,-1.62980188774553,378.346807630937));
#51964=CARTESIAN_POINT('Ctrl Pts',(3.46491455089248,-3.73449689435332,378.267679755478));
#51965=CARTESIAN_POINT('Ctrl Pts',(1.26428113644233,-4.93494610983311,378.188551880018));
#51966=CARTESIAN_POINT('Ctrl Pts',(-1.24247675173787,-4.94048088958068,
378.109424004558));
#51967=CARTESIAN_POINT('Ctrl Pts',(-3.4483897322594,-3.74976107950479,378.030296129098));
#51968=CARTESIAN_POINT('Ctrl Pts',(-4.81933297260539,-1.65109951186456,
377.951168253638));
#51969=CARTESIAN_POINT('Ctrl Pts',(-5.02335555943258,0.847348111721862,
377.872040378178));
#51970=CARTESIAN_POINT('Ctrl Pts',(-4.01105684503597,3.1406246010644,377.792912502719));
#51971=CARTESIAN_POINT('Ctrl Pts',(-2.02754798568437,4.67345151517251,377.713784627259));
#51972=CARTESIAN_POINT('Ctrl Pts',(0.44689761407191,5.07468052407812,377.634656751799));
#51973=CARTESIAN_POINT('Ctrl Pts',(2.81313445157142,4.24716075235008,377.555528876339));
#51974=CARTESIAN_POINT('Ctrl Pts',(4.49821796114695,2.39126223424701,377.47640100088));
#51975=CARTESIAN_POINT('Ctrl Pts',(5.09413343175754,-0.043640329640808,
377.39727312542));
#51976=CARTESIAN_POINT('Ctrl Pts',(4.4565899263877,-2.46797611960502,377.31814524996));
#51977=CARTESIAN_POINT('Ctrl Pts',(2.73995791251956,-4.29473288302567,377.2390173745));
#51978=CARTESIAN_POINT('Ctrl Pts',(0.35989104240352,-5.08159210646814,377.159889499041));
#51979=CARTESIAN_POINT('Ctrl Pts',(-2.10731740784078,-4.63802902551619,
377.080761623581));
#51980=CARTESIAN_POINT('Ctrl Pts',(-4.06427428993092,-3.07144500115654,
377.001633748121));
#51981=CARTESIAN_POINT('Ctrl Pts',(-5.03713531530297,-0.761162081456616,
376.922505872661));
#51982=CARTESIAN_POINT('Ctrl Pts',(-4.79033850266972,1.73342347069504,376.843377997201));
#51983=CARTESIAN_POINT('Ctrl Pts',(-3.38364156114149,3.8082896009442,376.764250121742));
#51984=CARTESIAN_POINT('Ctrl Pts',(-1.15765256317261,4.96104227374008,376.685122246282));
#51985=CARTESIAN_POINT('Ctrl Pts',(1.3486425877949,4.91256176240515,376.605994370822));
#51986=CARTESIAN_POINT('Ctrl Pts',(3.52838655442424,3.67458680959566,376.526866495362));
#51987=CARTESIAN_POINT('Ctrl Pts',(4.85379089203517,1.5468722880489,376.447738619903));
#51988=CARTESIAN_POINT('Ctrl Pts',(5.00393116882618,-0.955391415479512,
376.368610744443));
#51989=CARTESIAN_POINT('Ctrl Pts',(3.94245343483129,-3.22632311019696,376.289482868983));
#51990=CARTESIAN_POINT('Ctrl Pts',(1.92637672105698,-4.71605477417046,376.210354993523));
#51991=CARTESIAN_POINT('Ctrl Pts',(-0.556139808052753,-5.06387286571299,
376.131227118063));
#51992=CARTESIAN_POINT('Ctrl Pts',(-2.90399640996096,-4.18555907527208,
376.052099242604));
#51993=CARTESIAN_POINT('Ctrl Pts',(-4.54869898413812,-2.29378233993093,
375.972971367144));
#51994=CARTESIAN_POINT('Ctrl Pts',(-5.09201038719634,0.153395295307603,
375.893843491684));
#51995=CARTESIAN_POINT('Ctrl Pts',(-4.40237687192385,2.56343088388421,375.814715616224));
#51996=CARTESIAN_POINT('Ctrl Pts',(-2.64678163427568,4.35277456670489,375.735587740765));
#51997=CARTESIAN_POINT('Ctrl Pts',(-0.250312604595216,5.08816711975964,
375.656459865305));
#51998=CARTESIAN_POINT('Ctrl Pts',(2.2067654054518,4.59154485151799,375.577331989845));
#51999=CARTESIAN_POINT('Ctrl Pts',(4.12951222237333,2.98315803496294,375.498204114385));
#52000=CARTESIAN_POINT('Ctrl Pts',(5.05236682718355,0.652447347661906,375.419076238925));
#52001=CARTESIAN_POINT('Ctrl Pts',(4.75187571715042,-1.83623790240596,375.339948363465));
#52002=CARTESIAN_POINT('Ctrl Pts',(3.30079722094991,-3.88031871785061,375.260820488006));
#52003=CARTESIAN_POINT('Ctrl Pts',(1.05048684235124,-4.98482475543083,375.181692612546));
#52004=CARTESIAN_POINT('Ctrl Pts',(-1.45418293039009,-4.88238291455355,
375.102564737087));
#52005=CARTESIAN_POINT('Ctrl Pts',(-3.60674266297149,-3.59766175932869,
375.023436861626));
#52006=CARTESIAN_POINT('Ctrl Pts',(-4.8859942278021,-1.44202665000967,374.944308986167));
#52007=CARTESIAN_POINT('Ctrl Pts',(-4.98214589566551,1.06316661357685,374.865181110707));
#52008=CARTESIAN_POINT('Ctrl Pts',(-4.24189388987242,2.56091091663634,374.812429193734));
#52009=CARTESIAN_POINT('Ctrl Pts',(-3.71544298812364,3.17665283523617,374.786053235247));
#52010=CARTESIAN_POINT('Ctrl Pts',(-1.21713437249744,-4.54280821229883,
400.213946764753));
#52011=CARTESIAN_POINT('Ctrl Pts',(-1.96999142168732,-4.34109857602909,
400.187570806266));
#52012=CARTESIAN_POINT('Ctrl Pts',(-3.37271299505139,-3.55624125113577,
400.134818889293));
#52013=CARTESIAN_POINT('Ctrl Pts',(-4.66062705172882,-1.51685825396376,
400.055691013833));
#52014=CARTESIAN_POINT('Ctrl Pts',(-4.81980261122079,0.889513643374588,
399.976563138373));
#52015=CARTESIAN_POINT('Ctrl Pts',(-3.81205567514826,3.08066074806192,399.897435262913));
#52016=CARTESIAN_POINT('Ctrl Pts',(-1.8812299991108,4.52580660481483,399.818307387454));
#52017=CARTESIAN_POINT('Ctrl Pts',(0.505078813591743,4.87513817945551,399.739179511994));
#52018=CARTESIAN_POINT('Ctrl Pts',(2.76910316187124,4.04402084397575,399.660051636534));
#52019=CARTESIAN_POINT('Ctrl Pts',(4.36262999826625,2.23371923467566,399.580923761074));
#52020=CARTESIAN_POINT('Ctrl Pts',(4.89982180424067,-0.117443592687962,
399.501795885615));
#52021=CARTESIAN_POINT('Ctrl Pts',(4.25060268019241,-2.44016773763421,399.422668010155));
#52022=CARTESIAN_POINT('Ctrl Pts',(2.57217199816948,-4.17204698619159,399.343540134695));
#52023=CARTESIAN_POINT('Ctrl Pts',(0.270932724605363,-4.89373465051516,
399.264412259235));
#52024=CARTESIAN_POINT('Ctrl Pts',(-2.09590823180696,-4.43048672079232,
399.185284383776));
#52025=CARTESIAN_POINT('Ctrl Pts',(-3.95526022334416,-2.89447065191351,
399.106156508316));
#52026=CARTESIAN_POINT('Ctrl Pts',(-4.85691225648777,-0.657607098051338,
399.027028632856));
#52027=CARTESIAN_POINT('Ctrl Pts',(-4.58254445676102,1.73848500455744,398.947900757396));
#52028=CARTESIAN_POINT('Ctrl Pts',(-3.1985903647966,3.71363211084189,398.868772881936));
#52029=CARTESIAN_POINT('Ctrl Pts',(-1.0401512631882,4.78958548759503,398.789645006477));
#52030=CARTESIAN_POINT('Ctrl Pts',(1.37014302373642,4.70582106344184,398.710517131017));
#52031=CARTESIAN_POINT('Ctrl Pts',(3.44868015565118,3.48262099178473,398.631389255557));
#52032=CARTESIAN_POINT('Ctrl Pts',(4.69217722656672,1.41616265411303,398.552261380097));
#52033=CARTESIAN_POINT('Ctrl Pts',(4.79954227516165,-0.993195719354361,
398.473133504638));
#52034=CARTESIAN_POINT('Ctrl Pts',(3.74477865578454,-3.16206840652194,398.394005629178));
#52035=CARTESIAN_POINT('Ctrl Pts',(1.78327968915111,-4.56529926055421,398.314877753718));
#52036=CARTESIAN_POINT('Ctrl Pts',(-0.610010546527312,-4.8631194640233,
398.235749878258));
#52037=CARTESIAN_POINT('Ctrl Pts',(-2.85559695895555,-3.9834168494165,398.156622002799));
#52038=CARTESIAN_POINT('Ctrl Pts',(-4.40974845943849,-2.13919665124415,
398.077494127339));
#52039=CARTESIAN_POINT('Ctrl Pts',(-4.89615332706093,0.22299413922299,397.998366251879));
#52040=CARTESIAN_POINT('Ctrl Pts',(-4.19703678069868,2.53119063874627,397.919238376419));
#52041=CARTESIAN_POINT('Ctrl Pts',(-2.48167816706011,4.22650177609728,397.840110500959));
#52042=CARTESIAN_POINT('Ctrl Pts',(-0.165422805885864,4.89843639169769,
397.7609826255));
#52043=CARTESIAN_POINT('Ctrl Pts',(2.19088691340144,4.38429678750219,397.68185475004));
#52044=CARTESIAN_POINT('Ctrl Pts',(4.01671011032052,2.80857324594973,397.60272687458));
#52045=CARTESIAN_POINT('Ctrl Pts',(4.86995431890775,0.55280079591789,397.52359899912));
#52046=CARTESIAN_POINT('Ctrl Pts',(4.54402076394769,-1.83682309573565,397.444471123661));
#52047=CARTESIAN_POINT('Ctrl Pts',(3.11782878949058,-3.78169108040825,397.365343248201));
#52048=CARTESIAN_POINT('Ctrl Pts',(0.93670686325944,-4.81088599330085,397.286215372741));
#52049=CARTESIAN_POINT('Ctrl Pts',(-1.47122292025061,-4.67520554704762,
397.207087497281));
#52050=CARTESIAN_POINT('Ctrl Pts',(-3.52292074773491,-3.40750248619052,
397.127959621821));
#52051=CARTESIAN_POINT('Ctrl Pts',(-4.72160239961778,-1.31472984606697,
397.048831746362));
#52052=CARTESIAN_POINT('Ctrl Pts',(-4.77702721717586,1.09638257673893,396.969703870902));
#52053=CARTESIAN_POINT('Ctrl Pts',(-3.67577501037587,3.24202434619358,396.890575995442));
#52054=CARTESIAN_POINT('Ctrl Pts',(-1.68449553181902,4.60266429272193,396.811448119982));
#52055=CARTESIAN_POINT('Ctrl Pts',(0.714656288826095,4.84884627278046,396.732320244522));
#52056=CARTESIAN_POINT('Ctrl Pts',(2.94076607474594,3.92096144865504,396.653192369063));
#52057=CARTESIAN_POINT('Ctrl Pts',(4.45481867572026,2.0436815688041,396.574064493603));
#52058=CARTESIAN_POINT('Ctrl Pts',(4.89021164683945,-0.328441528025053,
396.494936618143));
#52059=CARTESIAN_POINT('Ctrl Pts',(4.14152188219155,-2.62103801718789,396.415808742683));
#52060=CARTESIAN_POINT('Ctrl Pts',(2.39003205189126,-4.27899410833295,396.336680867224));
#52061=CARTESIAN_POINT('Ctrl Pts',(0.0598360438320979,-4.90086353983399,
396.257552991764));
#52062=CARTESIAN_POINT('Ctrl Pts',(-2.28484825872123,-4.33607105832391,
396.178425116304));
#52063=CARTESIAN_POINT('Ctrl Pts',(-4.07629487497772,-2.72137169097608,
396.099297240844));
#52064=CARTESIAN_POINT('Ctrl Pts',(-4.88073505144618,-0.447737809214611,
396.020169365385));
#52065=CARTESIAN_POINT('Ctrl Pts',(-4.50338709078854,1.93430827396637,395.941041489924));
#52066=CARTESIAN_POINT('Ctrl Pts',(-3.03561947311557,3.84799404919722,395.861913614465));
#52067=CARTESIAN_POINT('Ctrl Pts',(-0.832827510883269,4.82995260073343,
395.782785739005));
#52068=CARTESIAN_POINT('Ctrl Pts',(1.57161966562715,4.64241913390311,395.703657863545));
#52069=CARTESIAN_POINT('Ctrl Pts',(3.5955254979886,3.3308017325457,395.624529988085));
#52070=CARTESIAN_POINT('Ctrl Pts',(4.74883513214048,1.21268655305647,395.545402112626));
#52071=CARTESIAN_POINT('Ctrl Pts',(4.75229398251168,-1.19906033709689,395.466274237166));
#52072=CARTESIAN_POINT('Ctrl Pts',(3.60506454649375,-3.32047487625331,395.387146361706));
#52073=CARTESIAN_POINT('Ctrl Pts',(1.5849291916516,-4.63789211233576,395.308018486247));
#52074=CARTESIAN_POINT('Ctrl Pts',(-0.818970185850148,-4.83232155624025,
395.228890610786));
#52075=CARTESIAN_POINT('Ctrl Pts',(-3.02456966792716,-3.85668537893236,
395.149762735327));
#52076=CARTESIAN_POINT('Ctrl Pts',(-4.49782033045318,-1.94721751819814,
395.070634859867));
#52077=CARTESIAN_POINT('Ctrl Pts',(-4.88199923361805,0.433736407473957,
394.991506984407));
#52078=CARTESIAN_POINT('Ctrl Pts',(-4.08408389914571,2.70966833633831,394.912379108948));
#52079=CARTESIAN_POINT('Ctrl Pts',(-2.29727614331402,4.32949952183574,394.833251233488));
#52080=CARTESIAN_POINT('Ctrl Pts',(0.04577850263863,4.90101500884376,394.754123358028));
#52081=CARTESIAN_POINT('Ctrl Pts',(2.37774865193587,4.28583190716024,394.674995482568));
#52082=CARTESIAN_POINT('Ctrl Pts',(4.13398684276656,2.63290648752449,394.595867607109));
#52083=CARTESIAN_POINT('Ctrl Pts',(4.8892494513703,0.34246691882695,394.516739731649));
#52084=CARTESIAN_POINT('Ctrl Pts',(4.46066230370267,-2.03089527069752,394.437611856189));
#52085=CARTESIAN_POINT('Ctrl Pts',(2.95200058966839,-3.91251023088926,394.358483980729));
#52086=CARTESIAN_POINT('Ctrl Pts',(0.728561441315958,-4.84677645600076,
394.279356105269));
#52087=CARTESIAN_POINT('Ctrl Pts',(-1.67128664123166,-4.60747704834829,
394.200228229809));
#52088=CARTESIAN_POINT('Ctrl Pts',(-3.66646069301835,-3.25255434616657,
394.12110035435));
#52089=CARTESIAN_POINT('Ctrl Pts',(-4.7738627787844,-1.11008015816539,394.04197247889));
#52090=CARTESIAN_POINT('Ctrl Pts',(-4.72535405587758,1.30118132280515,393.96284460343));
#52091=CARTESIAN_POINT('Ctrl Pts',(-3.53268009800228,3.39738356877675,393.88371672797));
#52092=CARTESIAN_POINT('Ctrl Pts',(-1.48462690153391,4.6709663616277,393.804588852511));
#52093=CARTESIAN_POINT('Ctrl Pts',(0.922903800227676,4.81355298752812,393.725460977051));
#52094=CARTESIAN_POINT('Ctrl Pts',(3.10696882493013,3.79061848635918,393.646333101591));
#52095=CARTESIAN_POINT('Ctrl Pts',(4.53873345614266,1.84984929178215,393.567205226131));
#52096=CARTESIAN_POINT('Ctrl Pts',(4.87151990076886,-0.538829884684078,
393.488077350672));
#52097=CARTESIAN_POINT('Ctrl Pts',(4.02474950245672,-2.79704044137549,393.408949475212));
#52098=CARTESIAN_POINT('Ctrl Pts',(2.2034535118369,-4.37799456479668,393.329821599752));
#52099=CARTESIAN_POINT('Ctrl Pts',(-0.151371792205916,-4.89889072839352,
393.250693724292));
#52100=CARTESIAN_POINT('Ctrl Pts',(-2.46954495544641,-4.23360266218321,
393.171565848832));
#52101=CARTESIAN_POINT('Ctrl Pts',(-4.18975922485567,-2.54321871374691,
393.092437973373));
#52102=CARTESIAN_POINT('Ctrl Pts',(-4.89549356508254,-0.23703700650118,
393.013310097913));
#52103=CARTESIAN_POINT('Ctrl Pts',(-4.41586624162366,2.12653923648359,392.934182222453));
#52104=CARTESIAN_POINT('Ctrl Pts',(-2.86701096694867,3.97520966788064,392.855054346993));
#52105=CARTESIAN_POINT('Ctrl Pts',(-0.623957069722673,4.86134974707218,
392.775926471534));
#52106=CARTESIAN_POINT('Ctrl Pts',(1.7701775674537,4.57039551547777,392.696798596074));
#52107=CARTESIAN_POINT('Ctrl Pts',(3.73569339459987,3.17279666063845,392.617670720614));
#52108=CARTESIAN_POINT('Ctrl Pts',(4.79667371815007,1.00695830590151,392.538542845154));
#52109=CARTESIAN_POINT('Ctrl Pts',(4.69621994662587,-1.40269811475204,392.459414969694));
#52110=CARTESIAN_POINT('Ctrl Pts',(3.45865527607574,-3.47271471179091,392.380287094234));
#52111=CARTESIAN_POINT('Ctrl Pts',(1.38363523608003,-4.70187168281881,392.301159218775));
#52112=CARTESIAN_POINT('Ctrl Pts',(-1.02640887116651,-4.79254928168782,
392.222031343315));
#52113=CARTESIAN_POINT('Ctrl Pts',(-3.18792528432602,-3.72279144860016,
392.142903467855));
#52114=CARTESIAN_POINT('Ctrl Pts',(-4.5775390550865,-1.75162210175979,392.063775592395));
#52115=CARTESIAN_POINT('Ctrl Pts',(-4.85877851429126,0.64367316028962,391.984647716936));
#52116=CARTESIAN_POINT('Ctrl Pts',(-3.96354624360545,2.88311376171958,391.905519841476));
#52117=CARTESIAN_POINT('Ctrl Pts',(-2.1086077232932,4.4244567189073,391.826391966016));
#52118=CARTESIAN_POINT('Ctrl Pts',(0.256894793419963,4.89449168487693,391.747264090557));
#52119=CARTESIAN_POINT('Ctrl Pts',(2.56019454432978,4.17940757564988,391.668136215096));
#52120=CARTESIAN_POINT('Ctrl Pts',(4.24358612375888,2.45235001548652,391.589008339637));
#52121=CARTESIAN_POINT('Ctrl Pts',(4.89946449317567,0.131497027824103,391.509880464177));
#52122=CARTESIAN_POINT('Ctrl Pts',(4.36901970526599,-2.22119575976841,391.430752588718));
#52123=CARTESIAN_POINT('Ctrl Pts',(2.78069006924853,-4.03606324615933,391.351624713257));
#52124=CARTESIAN_POINT('Ctrl Pts',(0.519062968356706,-4.87366570694958,
391.272496837798));
#52125=CARTESIAN_POINT('Ctrl Pts',(-1.86824652503536,-4.5311917538225,391.193368962338));
#52126=CARTESIAN_POINT('Ctrl Pts',(-3.80319145504887,-3.09156571084279,
391.114241086878));
#52127=CARTESIAN_POINT('Ctrl Pts',(-4.81725735814933,-0.903368880121367,
391.035113211418));
#52128=CARTESIAN_POINT('Ctrl Pts',(-4.66490518296109,1.50356357437869,390.955985335959));
#52129=CARTESIAN_POINT('Ctrl Pts',(-3.38302445358346,3.54643332584613,390.876857460499));
#52130=CARTESIAN_POINT('Ctrl Pts',(-1.28200109001022,4.73059372525567,390.797729585039));
#52131=CARTESIAN_POINT('Ctrl Pts',(1.12943733686538,4.76932019163214,390.718601709579));
#52132=CARTESIAN_POINT('Ctrl Pts',(3.2674014545917,3.65323576063024,390.639473834119));
#52133=CARTESIAN_POINT('Ctrl Pts',(4.61421910819667,1.65258155918805,390.56034595866));
#52134=CARTESIAN_POINT('Ctrl Pts',(4.84378099055226,-0.74821755110413,390.4812180832));
#52135=CARTESIAN_POINT('Ctrl Pts',(3.90050254186479,-2.96784832987165,390.40209020774));
#52136=CARTESIAN_POINT('Ctrl Pts',(2.01278281861149,-4.46886440981576,390.32296233228));
#52137=CARTESIAN_POINT('Ctrl Pts',(-0.362298507468694,-4.88781992095675,
390.243834456821));
#52138=CARTESIAN_POINT('Ctrl Pts',(-2.6496553261311,-4.12327181264112,390.164706581361));
#52139=CARTESIAN_POINT('Ctrl Pts',(-4.29544254536053,-2.36034258693993,
390.085578705901));
#52140=CARTESIAN_POINT('Ctrl Pts',(-4.90116039177906,-0.0258959894911138,
390.006450830441));
#52141=CARTESIAN_POINT('Ctrl Pts',(-4.32014444746653,2.31482088750723,389.927322954982));
#52142=CARTESIAN_POINT('Ctrl Pts',(-2.69307797902764,4.09504270882394,389.848195079522));
#52143=CARTESIAN_POINT('Ctrl Pts',(-0.41392784400509,4.88371861680963,389.769067204062));
#52144=CARTESIAN_POINT('Ctrl Pts',(1.96544797639375,4.48988396735431,389.689939328602));
#52145=CARTESIAN_POINT('Ctrl Pts',(3.86892353214857,3.00889921576025,389.610811453142));
#52146=CARTESIAN_POINT('Ctrl Pts',(4.83560414092378,0.799359981795764,389.531683577683));
#52147=CARTESIAN_POINT('Ctrl Pts',(4.63142430565821,-1.60373086556754,389.452555702223));
#52148=CARTESIAN_POINT('Ctrl Pts',(3.30582274912905,-3.61850518025834,389.373427826763));
#52149=CARTESIAN_POINT('Ctrl Pts',(1.17977165637593,-4.75711915207383,389.294299951303));
#52150=CARTESIAN_POINT('Ctrl Pts',(-1.23194135683111,-4.74387650361441,
389.215172075843));
#52151=CARTESIAN_POINT('Ctrl Pts',(-3.34536043156536,-3.58198372010992,
389.136044200384));
#52152=CARTESIAN_POINT('Ctrl Pts',(-4.64875658336638,-1.55277365279788,
389.056916324924));
#52153=CARTESIAN_POINT('Ctrl Pts',(-4.82653429353919,0.852414512725966,
388.977788449464));
#52154=CARTESIAN_POINT('Ctrl Pts',(-3.83564767110356,3.05120479997222,388.898660574004));
#52155=CARTESIAN_POINT('Ctrl Pts',(-1.91602329336559,4.5111970171448,388.819532698545));
#52156=CARTESIAN_POINT('Ctrl Pts',(0.467533990930312,4.87887853461636,388.740404823085));
#52157=CARTESIAN_POINT('Ctrl Pts',(2.73788576040913,4.06522143937628,388.661276947625));
#52158=CARTESIAN_POINT('Ctrl Pts',(4.34530441052119,2.26723915106472,388.582149072165));
#52159=CARTESIAN_POINT('Ctrl Pts',(4.90058047341499,-0.0797170734497908,
388.503021196706));
#52160=CARTESIAN_POINT('Ctrl Pts',(4.26926316308366,-2.40737114557615,388.423893321245));
#52161=CARTESIAN_POINT('Ctrl Pts',(2.60421537830119,-4.1521206692045,388.344765445786));
#52162=CARTESIAN_POINT('Ctrl Pts',(0.308600515372232,-4.89150380865921,
388.265637570326));
#52163=CARTESIAN_POINT('Ctrl Pts',(-2.06173678676592,-4.44649133703325,
388.186509694866));
#52164=CARTESIAN_POINT('Ctrl Pts',(-3.93285910370337,-2.92483556095608,
388.107381819407));
#52165=CARTESIAN_POINT('Ctrl Pts',(-4.85170554728278,-0.694979906674425,
388.028253943947));
#52166=CARTESIAN_POINT('Ctrl Pts',(-4.59579286131083,1.70315347639018,387.949126068487));
#52167=CARTESIAN_POINT('Ctrl Pts',(-3.22708601074344,3.68889680900396,387.869998193027));
#52168=CARTESIAN_POINT('Ctrl Pts',(-1.07699440464578,4.78143564639088,387.790870317567));
#52169=CARTESIAN_POINT('Ctrl Pts',(1.3338733340929,4.71623003221975,387.711742442108));
#52170=CARTESIAN_POINT('Ctrl Pts',(3.42176601558219,3.50906841238845,387.632614566648));
#52171=CARTESIAN_POINT('Ctrl Pts',(4.68113544337878,1.45224472764016,387.553486691188));
#52172=CARTESIAN_POINT('Ctrl Pts',(4.80704643162612,-0.956215662079578,
387.474358815728));
#52173=CARTESIAN_POINT('Ctrl Pts',(3.76901174619325,-3.13314446607126,387.395230940269));
#52174=CARTESIAN_POINT('Ctrl Pts',(1.81837407711343,-4.5514348840665,387.316103064809));
#52175=CARTESIAN_POINT('Ctrl Pts',(-0.572552378499359,-4.86767167772133,
387.236975189349));
#52176=CARTESIAN_POINT('Ctrl Pts',(-2.82484487802531,-4.00528341110962,
387.157847313889));
#52177=CARTESIAN_POINT('Ctrl Pts',(-4.39314856625886,-2.173082939741,387.07871943843));
#52178=CARTESIAN_POINT('Ctrl Pts',(-4.89772500736415,0.185293120367267,
386.99959156297));
#52179=CARTESIAN_POINT('Ctrl Pts',(-4.21639947845907,2.4988035589589,386.92046368751));
#52180=CARTESIAN_POINT('Ctrl Pts',(-2.51414352974947,4.20727062357945,386.84133581205));
#52181=CARTESIAN_POINT('Ctrl Pts',(-0.203129890410879,4.89701766750308,
386.762207936591));
#52182=CARTESIAN_POINT('Ctrl Pts',(2.15706824516707,4.40103401190078,386.68308006113));
#52183=CARTESIAN_POINT('Ctrl Pts',(3.99496848171146,2.83941378075611,386.603952185671));
#52184=CARTESIAN_POINT('Ctrl Pts',(4.86555410065941,0.590277122860157,386.524824310211));
#52185=CARTESIAN_POINT('Ctrl Pts',(4.55802739511214,-1.80178524070515,386.445696434751));
#52186=CARTESIAN_POINT('Ctrl Pts',(3.14685079923878,-3.75757552625969,386.366568559291));
#52187=CARTESIAN_POINT('Ctrl Pts',(0.973717058663619,-4.80353191702554,
386.287440683832));
#52188=CARTESIAN_POINT('Ctrl Pts',(-1.43518593730373,-4.68639361487927,
386.208312808372));
#52189=CARTESIAN_POINT('Ctrl Pts',(-3.49658272828396,-3.43452369514056,
386.129184932912));
#52190=CARTESIAN_POINT('Ctrl Pts',(-4.71134065335373,-1.35104146356512,
386.050057057452));
#52191=CARTESIAN_POINT('Ctrl Pts',(-4.78532645385515,1.05957279988197,385.970929181993));
#52192=CARTESIAN_POINT('Ctrl Pts',(-3.70062570902444,3.21362928010108,385.891801306533));
#52193=CARTESIAN_POINT('Ctrl Pts',(-1.71988051253413,4.58955932643004,385.812673431073));
#52194=CARTESIAN_POINT('Ctrl Pts',(0.677304905677504,4.85420455409132,385.733545555613));
#52195=CARTESIAN_POINT('Ctrl Pts',(2.91049230016732,3.94348555961378,385.654417680154));
#52196=CARTESIAN_POINT('Ctrl Pts',(4.43895279649954,2.07791767369751,385.575289804694));
#52197=CARTESIAN_POINT('Ctrl Pts',(4.89259531954076,-0.29078312781775,385.496161929234));
#52198=CARTESIAN_POINT('Ctrl Pts',(4.16157794044722,-2.58907567170192,385.417034053774));
#52199=CARTESIAN_POINT('Ctrl Pts',(2.42290425755801,-4.26046696348217,385.337906178315));
#52200=CARTESIAN_POINT('Ctrl Pts',(0.0975649436126985,-4.90025763302231,
385.258778302854));
#52201=CARTESIAN_POINT('Ctrl Pts',(-2.25139808515128,-4.35353309972404,
385.179650427395));
#52202=CARTESIAN_POINT('Ctrl Pts',(-4.05522282615024,-2.75267354012164,
385.100522551935));
#52203=CARTESIAN_POINT('Ctrl Pts',(-4.87714337058205,-0.485300248303261,
385.021394676475));
#52204=CARTESIAN_POINT('Ctrl Pts',(-4.51814544317236,1.89958035959429,384.942266801015));
#52205=CARTESIAN_POINT('Ctrl Pts',(-3.06515437123229,3.82450944157957,384.863138925556));
#52206=CARTESIAN_POINT('Ctrl Pts',(-0.869987574488363,4.82339770374075,
384.784011050096));
#52207=CARTESIAN_POINT('Ctrl Pts',(1.53583212271834,4.65438110590894,384.704883174636));
#52208=CARTESIAN_POINT('Ctrl Pts',(3.56977582909287,3.35838418264497,384.625755299176));
#52209=CARTESIAN_POINT('Ctrl Pts',(4.73935818772915,1.24921085354728,384.546627423716));
#52210=CARTESIAN_POINT('Ctrl Pts',(4.76138444573462,-1.16243793302357,384.467499548257));
#52211=CARTESIAN_POINT('Ctrl Pts',(3.6305213141391,-3.29262186954369,384.388371672797));
#52212=CARTESIAN_POINT('Ctrl Pts',(1.62058833437354,-4.62555264143734,384.309243797337));
#52213=CARTESIAN_POINT('Ctrl Pts',(-0.781742931416587,-4.83848341708389,
384.230115921878));
#52214=CARTESIAN_POINT('Ctrl Pts',(-2.9947882570989,-3.87985658025632,384.150988046417));
#52215=CARTESIAN_POINT('Ctrl Pts',(-4.48269583239351,-1.98178754220968,
384.071860170958));
#52216=CARTESIAN_POINT('Ctrl Pts',(-4.88519379187676,0.396138112309837,
383.992732295498));
#52217=CARTESIAN_POINT('Ctrl Pts',(-4.10482400501691,2.67814556662863,383.913604420039));
#52218=CARTESIAN_POINT('Ctrl Pts',(-2.33053992799659,4.31168498759236,383.834476544578));
#52219=CARTESIAN_POINT('Ctrl Pts',(0.00804530673338092,4.90122220076332,
383.755348669119));
#52220=CARTESIAN_POINT('Ctrl Pts',(2.34468250536694,4.30401065719426,383.676220793659));
#52221=CARTESIAN_POINT('Ctrl Pts',(4.11359415836805,2.66465511623097,383.5970929182));
#52222=CARTESIAN_POINT('Ctrl Pts',(4.88646797566037,0.380098028225917,383.517965042739));
#52223=CARTESIAN_POINT('Ctrl Pts',(4.47616552437595,-1.99649342262975,383.43883716728));
#52224=CARTESIAN_POINT('Ctrl Pts',(2.98203466184577,-3.88966747470347,383.35970929182));
#52225=CARTESIAN_POINT('Ctrl Pts',(0.765854118125881,-4.84102378200782,
383.28058141636));
#52226=CARTESIAN_POINT('Ctrl Pts',(-1.6357651560373,-4.62020737007657,383.2014535409));
#52227=CARTESIAN_POINT('Ctrl Pts',(-3.6413113313429,-3.28068522971184,383.122325665441));
#52228=CARTESIAN_POINT('Ctrl Pts',(-4.76517503677366,-1.14680018186465,
383.043197789981));
#52229=CARTESIAN_POINT('Ctrl Pts',(-4.73523152455593,1.26476329685335,382.964069914521));
#52230=CARTESIAN_POINT('Ctrl Pts',(-3.55873111398586,3.37008555478411,382.884942039061));
#52231=CARTESIAN_POINT('Ctrl Pts',(-1.52054364820804,4.65939811586324,382.805814163601));
#52232=CARTESIAN_POINT('Ctrl Pts',(0.885817960704724,4.82051556669083,382.726686288142));
#52233=CARTESIAN_POINT('Ctrl Pts',(3.07769360662633,3.8144260186753,382.647558412682));
#52234=CARTESIAN_POINT('Ctrl Pts',(4.52435736219093,1.88473718258125,382.568430537222));
#52235=CARTESIAN_POINT('Ctrl Pts',(4.87552386121587,-0.501309153048634,
382.489302661763));
#52236=CARTESIAN_POINT('Ctrl Pts',(4.04616402543129,-2.76597188480314,382.410174786302));
#52237=CARTESIAN_POINT('Ctrl Pts',(2.23709342974706,-4.36090091320568,382.331046910843));
#52238=CARTESIAN_POINT('Ctrl Pts',(-0.113651821301689,-4.89991092283629,
382.251919035383));
#52239=CARTESIAN_POINT('Ctrl Pts',(-2.43687818989498,-4.25248967968529,
382.172791159923));
#52240=CARTESIAN_POINT('Ctrl Pts',(-4.17005537407579,-2.5753993797773,382.093663284464));
#52241=CARTESIAN_POINT('Ctrl Pts',(-4.89352358608415,-0.274719312487676,
382.014535409004));
#52242=CARTESIAN_POINT('Ctrl Pts',(-4.43210713178239,2.09247942895964,381.935407533544));
#52243=CARTESIAN_POINT('Ctrl Pts',(-2.89753026709117,3.95301936998874,381.856279658084));
#52244=CARTESIAN_POINT('Ctrl Pts',(-0.661365043163431,4.85640196728989,
381.777151782624));
#52245=CARTESIAN_POINT('Ctrl Pts',(1.73493863410831,4.58388827569936,381.698023907165));
#52246=CARTESIAN_POINT('Ctrl Pts',(3.7111560180617,3.20146291526546,381.618896031705));
#52247=CARTESIAN_POINT('Ctrl Pts',(4.78877921262759,1.04385700214232,381.539768156245));
#52248=CARTESIAN_POINT('Ctrl Pts',(4.70687983423134,-1.36650137735827,381.460640280785));
#52249=CARTESIAN_POINT('Ctrl Pts',(3.48528844380413,-3.44598436614286,381.381512405325));
#52250=CARTESIAN_POINT('Ctrl Pts',(1.41979290903503,-4.69108003381625,381.302384529866));
#52251=CARTESIAN_POINT('Ctrl Pts',(-0.989481667084847,-4.80030934614829,
381.223256654406));
#52252=CARTESIAN_POINT('Ctrl Pts',(-3.1591698522741,-3.74722425705989,381.144128778946));
#52253=CARTESIAN_POINT('Ctrl Pts',(-4.56391804067381,-1.78681165941677,
381.065000903487));
#52254=CARTESIAN_POINT('Ctrl Pts',(-4.86359001771767,0.606247414652442,
380.985873028026));
#52255=CARTESIAN_POINT('Ctrl Pts',(-3.98562524001068,2.85251384473511,380.906745152567));
#52256=CARTESIAN_POINT('Ctrl Pts',(-2.1426081539881,4.40809188727722,380.827617277107));
#52257=CARTESIAN_POINT('Ctrl Pts',(0.219205562501549,4.89632440812331,380.748489401647));
#52258=CARTESIAN_POINT('Ctrl Pts',(2.52794232836271,4.19899409057548,380.669361526187));
#52259=CARTESIAN_POINT('Ctrl Pts',(4.22458025593252,2.48494777599062,380.590233650728));
#52260=CARTESIAN_POINT('Ctrl Pts',(4.89830692563373,0.169213032902914,380.511105775268));
#52261=CARTESIAN_POINT('Ctrl Pts',(4.38599072357506,-2.18749380820361,380.431977899808));
#52262=CARTESIAN_POINT('Ctrl Pts',(2.81168042594869,-4.01453571045926,380.352850024348));
#52263=CARTESIAN_POINT('Ctrl Pts',(0.556568868317172,-4.86952511884227,
380.273722148889));
#52264=CARTESIAN_POINT('Ctrl Pts',(-1.83330650647258,-4.54544068727564,
380.194594273429));
#52265=CARTESIAN_POINT('Ctrl Pts',(-3.77927745739419,-3.12075402559187,
380.115466397969));
#52266=CARTESIAN_POINT('Ctrl Pts',(-4.81015975486937,-0.940429115271696,
380.036338522509));
#52267=CARTESIAN_POINT('Ctrl Pts',(-4.67634253965503,1.46760493322567,379.95721064705));
#52268=CARTESIAN_POINT('Ctrl Pts',(-3.41022740614562,3.5202830605775,379.878082771589));
#52269=CARTESIAN_POINT('Ctrl Pts',(-1.31838289970275,4.72058368403601,379.79895489613));
#52270=CARTESIAN_POINT('Ctrl Pts',(1.09268591509449,4.77787413806285,379.71982702067));
#52271=CARTESIAN_POINT('Ctrl Pts',(3.23917916116038,3.67828250004266,379.64069914521));
#52272=CARTESIAN_POINT('Ctrl Pts',(4.60135949813868,1.68805644369628,379.56157126975));
#52273=CARTESIAN_POINT('Ctrl Pts',(4.8493978027726,-0.71090416982881,379.482443394291));
#52274=CARTESIAN_POINT('Ctrl Pts',(3.92323575948474,-2.93773126131644,379.403315518831));
#52275=CARTESIAN_POINT('Ctrl Pts',(2.04712797424676,-4.45323599703316,379.324187643371));
#52276=CARTESIAN_POINT('Ctrl Pts',(-0.324657517247101,-4.89046432199546,
379.245059767911));
#52277=CARTESIAN_POINT('Ctrl Pts',(-2.61783263582229,-4.14354873013934,
379.165931892452));
#52278=CARTESIAN_POINT('Ctrl Pts',(-4.27714348571947,-2.39334230539285,
379.086804016992));
#52279=CARTESIAN_POINT('Ctrl Pts',(-4.90081577320139,-0.0636281805188475,
379.007676141532));
#52280=CARTESIAN_POINT('Ctrl Pts',(-4.33783771356114,2.28149244114949,378.928548266072));
#52281=CARTESIAN_POINT('Ctrl Pts',(-2.72452500214632,4.07418793146503,378.849420390613));
#52282=CARTESIAN_POINT('Ctrl Pts',(-0.451514254902642,4.88038714302825,
378.770292515153));
#52283=CARTESIAN_POINT('Ctrl Pts',(1.93082309674852,4.50488245765392,378.691164639693));
#52284=CARTESIAN_POINT('Ctrl Pts',(3.84564401766237,3.03859603725688,378.612036764233));
#52285=CARTESIAN_POINT('Ctrl Pts',(4.82930673560502,0.836564547214143,378.532908888774));
#52286=CARTESIAN_POINT('Ctrl Pts',(4.64363382059009,-1.56802701777984,378.453781013314));
#52287=CARTESIAN_POINT('Ctrl Pts',(3.33358285503851,-3.59294713804823,378.374653137854));
#52288=CARTESIAN_POINT('Ctrl Pts',(1.21636070918609,-4.74789536672449,378.295525262394));
#52289=CARTESIAN_POINT('Ctrl Pts',(-1.19538278261738,-4.7532203600546,378.216397386934));
#52290=CARTESIAN_POINT('Ctrl Pts',(-3.31768438156428,-3.60763276020996,
378.137269511475));
#52291=CARTESIAN_POINT('Ctrl Pts',(-4.6366643489263,-1.58851739166163,378.058141636015));
#52292=CARTESIAN_POINT('Ctrl Pts',(-4.83295380642895,0.815230822000412,
377.979013760555));
#52293=CARTESIAN_POINT('Ctrl Pts',(-3.85902455393964,3.02158456448046,377.899885885095));
#52294=CARTESIAN_POINT('Ctrl Pts',(-1.95069722602663,4.49631228014555,377.820758009635));
#52295=CARTESIAN_POINT('Ctrl Pts',(0.429958719716191,4.88233338553971,377.741630134176));
#52296=CARTESIAN_POINT('Ctrl Pts',(2.70650737238561,4.08617934401293,377.662502258716));
#52297=CARTESIAN_POINT('Ctrl Pts',(4.32772065609622,2.30062550429524,377.583374383256));
#52298=CARTESIAN_POINT('Ctrl Pts',(4.9010489638226,-0.0419862171323538,
377.504246507796));
#52299=CARTESIAN_POINT('Ctrl Pts',(4.28767046122876,-2.37443168023888,377.425118632336));
#52300=CARTESIAN_POINT('Ctrl Pts',(2.63610446564972,-4.13194833394574,377.345990756877));
#52301=CARTESIAN_POINT('Ctrl Pts',(0.346249984239667,-4.88898299614862,
377.266862881417));
#52302=CARTESIAN_POINT('Ctrl Pts',(-2.0274431238406,-4.46223241974302,377.187735005957));
#52303=CARTESIAN_POINT('Ctrl Pts',(-3.91022488205308,-2.95502709970493,
377.108607130498));
#52304=CARTESIAN_POINT('Ctrl Pts',(-4.84621126407803,-0.732311526700024,
377.029479255038));
#52305=CARTESIAN_POINT('Ctrl Pts',(-4.60876886508425,1.66772100077964,376.950351379578));
#52306=CARTESIAN_POINT('Ctrl Pts',(-3.25539037980364,3.66394285754004,376.871223504118));
#52307=CARTESIAN_POINT('Ctrl Pts',(-1.11377371072242,4.77300239990086,376.792095628659));
#52308=CARTESIAN_POINT('Ctrl Pts',(1.29752458313577,4.72635945993341,376.712967753198));
#52309=CARTESIAN_POINT('Ctrl Pts',(3.39464906017594,3.53530784320889,376.633839877739));
#52310=CARTESIAN_POINT('Ctrl Pts',(4.66981619949699,1.48824072358315,376.554712002279));
#52311=CARTESIAN_POINT('Ctrl Pts',(4.8142656643279,-0.919178927997845,376.475584126819));
#52312=CARTESIAN_POINT('Ctrl Pts',(3.79302143937608,-3.10403481730793,376.396456251359));
#52313=CARTESIAN_POINT('Ctrl Pts',(1.85336068619839,-4.53730073503479,376.3173283759));
#52314=CARTESIAN_POINT('Ctrl Pts',(-0.535060274040971,-4.87193537309239,
376.23820050044));
#52315=CARTESIAN_POINT('Ctrl Pts',(-2.7939253627036,-4.02691257378452,376.15907262498));
#52316=CARTESIAN_POINT('Ctrl Pts',(-4.37628828172638,-2.20684041966181,
376.07994474952));
#52317=CARTESIAN_POINT('Ctrl Pts',(-4.89900638965642,0.147581107404016,
376.000816874061));
#52318=CARTESIAN_POINT('Ctrl Pts',(-4.23551226043463,2.46626839394683,375.921688998601));
#52319=CARTESIAN_POINT('Ctrl Pts',(-2.54645987583722,4.18779004627332,375.842561123141));
#52320=CARTESIAN_POINT('Ctrl Pts',(-0.24082493083811,4.89530879473852,375.763433247681));
#52321=CARTESIAN_POINT('Ctrl Pts',(2.12312171415927,4.41751014933925,375.684305372222));
#52322=CARTESIAN_POINT('Ctrl Pts',(3.97299008156779,2.87008650088106,375.605177496762));
#52323=CARTESIAN_POINT('Ctrl Pts',(4.86086545139366,0.627717440079687,375.526049621302));
#52324=CARTESIAN_POINT('Ctrl Pts',(4.57176394606508,-1.76663842623643,375.446921745842));
#52325=CARTESIAN_POINT('Ctrl Pts',(3.1756861134954,-3.73324183321634,375.367793870382));
#52326=CARTESIAN_POINT('Ctrl Pts',(1.01066992437191,-4.79588344705227,375.288665994922));
#52327=CARTESIAN_POINT('Ctrl Pts',(-1.39906459845869,-4.69732449000695,
375.209538119463));
#52328=CARTESIAN_POINT('Ctrl Pts',(-3.47003521363053,-3.46129850620319,
375.130410244003));
#52329=CARTESIAN_POINT('Ctrl Pts',(-4.70079892256589,-1.38736908122097,
375.051282368543));
#52330=CARTESIAN_POINT('Ctrl Pts',(-4.79330612491241,1.02286909042425,374.972154493083));
#52331=CARTESIAN_POINT('Ctrl Pts',(-4.08111211300407,2.46384394177367,374.91940257611));
#52332=CARTESIAN_POINT('Ctrl Pts',(-3.57461543774341,3.05624720968232,374.893026617624));
#52333=CARTESIAN_POINT('Ctrl Pts',(-1.16918346556839,-4.36383719750651,
400.320920147129));
#52334=CARTESIAN_POINT('Ctrl Pts',(-1.89238053709901,-4.17007422695751,
400.294544188642));
#52335=CARTESIAN_POINT('Ctrl Pts',(-3.23983970630162,-3.41613758049457,
400.241792271669));
#52336=CARTESIAN_POINT('Ctrl Pts',(-4.47701437999898,-1.45709925725484,
400.162664396209));
#52337=CARTESIAN_POINT('Ctrl Pts',(-4.62991897006387,0.854469866048622,
400.08353652075));
#52338=CARTESIAN_POINT('Ctrl Pts',(-3.66187379628773,2.9592933130866,400.00440864529));
#52339=CARTESIAN_POINT('Ctrl Pts',(-1.80711600920317,4.34750539486619,399.92528076983));
#52340=CARTESIAN_POINT('Ctrl Pts',(0.485180445975455,4.68307450728292,399.84615289437));
#52341=CARTESIAN_POINT('Ctrl Pts',(2.66001002393004,3.8847003355008,399.767025018911));
#52342=CARTESIAN_POINT('Ctrl Pts',(4.19075738523379,2.14571838156707,399.687897143451));
#52343=CARTESIAN_POINT('Ctrl Pts',(4.70678568217143,-0.112816719181106,
399.608769267991));
#52344=CARTESIAN_POINT('Ctrl Pts',(4.0831435580808,-2.34403352376061,399.529641392531));
#52345=CARTESIAN_POINT('Ctrl Pts',(2.47083727056938,-4.00768268816587,399.450513517072));
#52346=CARTESIAN_POINT('Ctrl Pts',(0.26025890735466,-4.70093834136087,399.371385641611));
#52347=CARTESIAN_POINT('Ctrl Pts',(-2.01333665809567,-4.25594078634204,
399.292257766152));
#52348=CARTESIAN_POINT('Ctrl Pts',(-3.79943657795602,-2.78043846617054,
399.213129890692));
#52349=CARTESIAN_POINT('Ctrl Pts',(-4.66556662297687,-0.631699640775407,
399.134002015232));
#52350=CARTESIAN_POINT('Ctrl Pts',(-4.40200797064279,1.66999467634492,399.054874139773));
#52351=CARTESIAN_POINT('Ctrl Pts',(-3.07257690863908,3.56732778180521,398.975746264313));
#52352=CARTESIAN_POINT('Ctrl Pts',(-0.999172881885126,4.60089229715201,
398.896618388853));
#52353=CARTESIAN_POINT('Ctrl Pts',(1.31616410234924,4.52042790313295,398.817490513393));
#52354=CARTESIAN_POINT('Ctrl Pts',(3.3128140221261,3.34541770608376,398.738362637933));
#52355=CARTESIAN_POINT('Ctrl Pts',(4.50732158649137,1.36037071761185,398.659234762474));
#52356=CARTESIAN_POINT('Ctrl Pts',(4.61045682154316,-0.954067224935643,
398.580106887014));
#52357=CARTESIAN_POINT('Ctrl Pts',(3.5972472600316,-3.03749378987274,398.500979011554));
#52358=CARTESIAN_POINT('Ctrl Pts',(1.71302460447423,-4.38544217583732,398.421851136094));
#52359=CARTESIAN_POINT('Ctrl Pts',(-0.58597822963345,-4.67152928789035,
398.342723260635));
#52360=CARTESIAN_POINT('Ctrl Pts',(-2.74309626297668,-3.82648392982927,
398.263595385175));
#52361=CARTESIAN_POINT('Ctrl Pts',(-4.23601954113904,-2.05491966273361,
398.184467509715));
#52362=CARTESIAN_POINT('Ctrl Pts',(-4.70326173037178,0.214208937311664,
398.105339634255));
#52363=CARTESIAN_POINT('Ctrl Pts',(-4.0316879707426,2.43147043571793,398.026211758796));
#52364=CARTESIAN_POINT('Ctrl Pts',(-2.38390858507682,4.05999214669189,397.947083883336));
#52365=CARTESIAN_POINT('Ctrl Pts',(-0.158905716443472,4.70545485011635,
397.867956007876));
#52366=CARTESIAN_POINT('Ctrl Pts',(2.10457350639361,4.2115705775148,397.788828132416));
#52367=CARTESIAN_POINT('Ctrl Pts',(3.85846555079357,2.69792512248606,397.709700256956));
#52368=CARTESIAN_POINT('Ctrl Pts',(4.67809487300653,0.531022346377457,397.630572381497));
#52369=CARTESIAN_POINT('Ctrl Pts',(4.36500197879199,-1.76445858504648,397.551444506037));
#52370=CARTESIAN_POINT('Ctrl Pts',(2.99499706155341,-3.63270546211616,397.472316630577));
#52371=CARTESIAN_POINT('Ctrl Pts',(0.899803835430396,-4.62135363621384,
397.393188755117));
#52372=CARTESIAN_POINT('Ctrl Pts',(-1.41326179868926,-4.4910185327571,397.314060879658));
#52373=CARTESIAN_POINT('Ctrl Pts',(-3.38412979029408,-3.2732586111773,397.234933004198));
#52374=CARTESIAN_POINT('Ctrl Pts',(-4.53558750895661,-1.26293401324019,
397.155805128738));
#52375=CARTESIAN_POINT('Ctrl Pts',(-4.58882877938272,1.0531888751364,397.076677253278));
#52376=CARTESIAN_POINT('Ctrl Pts',(-3.53096212085652,3.11429974059636,396.997549377818));
#52377=CARTESIAN_POINT('Ctrl Pts',(-1.61813220309064,4.42133515428577,396.918421502359));
#52378=CARTESIAN_POINT('Ctrl Pts',(0.686501289701844,4.65781841127795,396.839293626899));
#52379=CARTESIAN_POINT('Ctrl Pts',(2.82491000861503,3.76648905699045,396.760165751439));
#52380=CARTESIAN_POINT('Ctrl Pts',(4.27931414595585,1.96316754593802,396.681037875979));
#52381=CARTESIAN_POINT('Ctrl Pts',(4.69755413190968,-0.315502061769038,
396.601910000519));
#52382=CARTESIAN_POINT('Ctrl Pts',(3.97836016824692,-2.51777813655384,396.52278212506));
#52383=CARTESIAN_POINT('Ctrl Pts',(2.29587301155249,-4.11041646162856,396.4436542496));
#52384=CARTESIAN_POINT('Ctrl Pts',(0.0574787095610184,-4.70778637696628,
396.36452637414));
#52385=CARTESIAN_POINT('Ctrl Pts',(-2.1948330979661,-4.16524477615358,396.28539849868));
#52386=CARTESIAN_POINT('Ctrl Pts',(-3.9157028807147,-2.614159008776,396.206270623221));
#52387=CARTESIAN_POINT('Ctrl Pts',(-4.68845088177226,-0.430098479898641,
396.127142747761));
#52388=CARTESIAN_POINT('Ctrl Pts',(-4.32596913256195,1.85810318263636,396.048014872301));
#52389=CARTESIAN_POINT('Ctrl Pts',(-2.91602650941616,3.69639632203913,395.968886996841));
#52390=CARTESIAN_POINT('Ctrl Pts',(-0.8000169721583,4.63966908490906,395.889759121381));
#52391=CARTESIAN_POINT('Ctrl Pts',(1.50970325769618,4.4595237914943,395.810631245922));
#52392=CARTESIAN_POINT('Ctrl Pts',(3.45387416317228,3.19957960334997,395.731503370462));
#52393=CARTESIAN_POINT('Ctrl Pts',(4.56174736550757,1.16491087491141,395.652375495002));
#52394=CARTESIAN_POINT('Ctrl Pts',(4.56506994907375,-1.15182148498192,395.573247619542));
#52395=CARTESIAN_POINT('Ctrl Pts',(3.46303740598383,-3.18965958966768,395.494119744083));
#52396=CARTESIAN_POINT('Ctrl Pts',(1.52248843418447,-4.45517511900225,395.414991868623));
#52397=CARTESIAN_POINT('Ctrl Pts',(-0.786705578057672,-4.64194471171891,
395.335863993163));
#52398=CARTESIAN_POINT('Ctrl Pts',(-2.90541202853717,-3.70474524328377,
395.256736117703));
#52399=CARTESIAN_POINT('Ctrl Pts',(-4.32062168343229,-1.87050384705749,
395.177608242243));
#52400=CARTESIAN_POINT('Ctrl Pts',(-4.68966525951576,0.416648685217087,
395.098480366784));
#52401=CARTESIAN_POINT('Ctrl Pts',(-3.92318504412731,2.60291672604753,395.019352491324));
#52402=CARTESIAN_POINT('Ctrl Pts',(-2.20677136666199,4.15893213559478,394.940224615864));
#52403=CARTESIAN_POINT('Ctrl Pts',(0.0439749871279553,4.70793187861818,
394.861096740404));
#52404=CARTESIAN_POINT('Ctrl Pts',(2.28407353529635,4.11698487470637,394.781968864944));
#52405=CARTESIAN_POINT('Ctrl Pts',(3.97112198345224,2.52917902999067,394.702840989485));
#52406=CARTESIAN_POINT('Ctrl Pts',(4.69662984363174,0.328974900425354,394.623713114025));
#52407=CARTESIAN_POINT('Ctrl Pts',(4.28492755509978,-1.95088498398772,394.544585238566));
#52408=CARTESIAN_POINT('Ctrl Pts',(2.83570192230001,-3.75837078812964,394.465457363105));
#52409=CARTESIAN_POINT('Ctrl Pts',(0.699858627021958,-4.65583013815851,
394.386329487646));
#52410=CARTESIAN_POINT('Ctrl Pts',(-1.60544369734944,-4.42595830389794,
394.307201612186));
#52411=CARTESIAN_POINT('Ctrl Pts',(-3.52201475555854,-3.12441489479712,
394.228073736726));
#52412=CARTESIAN_POINT('Ctrl Pts',(-4.58578900897716,-1.06634681897889,
394.148945861266));
#52413=CARTESIAN_POINT('Ctrl Pts',(-4.53919136286672,1.24991925518346,394.069817985807));
#52414=CARTESIAN_POINT('Ctrl Pts',(-3.39350465573632,3.26353834429719,393.990690110347));
#52415=CARTESIAN_POINT('Ctrl Pts',(-1.42613770922415,4.48694635665851,393.911562234887));
#52416=CARTESIAN_POINT('Ctrl Pts',(0.886544565594953,4.62391556004391,393.832434359427));
#52417=CARTESIAN_POINT('Ctrl Pts',(2.98456494223475,3.64128115898587,393.753306483967));
#52418=CARTESIAN_POINT('Ctrl Pts',(4.35992297272438,1.77697159378319,393.674178608508));
#52419=CARTESIAN_POINT('Ctrl Pts',(4.67959877632843,-0.51760184098167,393.595050733048));
#52420=CARTESIAN_POINT('Ctrl Pts',(3.86618821853779,-2.68684667073537,393.515922857588));
#52421=CARTESIAN_POINT('Ctrl Pts',(2.116645024084,-4.20551664070214,393.436794982129));
#52422=CARTESIAN_POINT('Ctrl Pts',(-0.14540826436235,-4.70589128750945,
393.357667106668));
#52423=CARTESIAN_POINT('Ctrl Pts',(-2.37225338025842,-4.06681328229544,
393.278539231209));
#52424=CARTESIAN_POINT('Ctrl Pts',(-4.02469712556258,-2.44302464594413,
393.199411355749));
#52425=CARTESIAN_POINT('Ctrl Pts',(-4.70262796074555,-0.227698563931231,
393.120283480289));
#52426=CARTESIAN_POINT('Ctrl Pts',(-4.24189630375331,2.04276090656889,393.04115560483));
#52427=CARTESIAN_POINT('Ctrl Pts',(-2.75406059832286,3.81860008301049,392.962027729369));
#52428=CARTESIAN_POINT('Ctrl Pts',(-0.599375307795595,4.66982929169869,
392.88289985391));
#52429=CARTESIAN_POINT('Ctrl Pts',(1.70043866129603,4.39033765584971,392.80377197845));
#52430=CARTESIAN_POINT('Ctrl Pts',(3.58851992688128,3.04779938768583,392.72464410299));
#52431=CARTESIAN_POINT('Ctrl Pts',(4.60770127580904,0.967287612920714,392.64551622753));
#52432=CARTESIAN_POINT('Ctrl Pts',(4.51120503728849,-1.34743663477919,392.566388352071));
#52433=CARTESIAN_POINT('Ctrl Pts',(3.32239615712367,-3.3359016994408,392.487260476611));
#52434=CARTESIAN_POINT('Ctrl Pts',(1.32912476794421,-4.51663411451929,392.408132601151));
#52435=CARTESIAN_POINT('Ctrl Pts',(-0.985971892830688,-4.60373932795397,
392.329004725692));
#52436=CARTESIAN_POINT('Ctrl Pts',(-3.06233199564761,-3.57612627316698,
392.249876850231));
#52437=CARTESIAN_POINT('Ctrl Pts',(-4.397199764574,-1.68261421711348,392.170748974772));
#52438=CARTESIAN_POINT('Ctrl Pts',(-4.66735935664344,0.618314652224117,
392.091621099312));
#52439=CARTESIAN_POINT('Ctrl Pts',(-3.80739615752567,2.76952899837877,392.012493223852));
#52440=CARTESIAN_POINT('Ctrl Pts',(-2.02553583330784,4.25014834578608,391.933365348393));
#52441=CARTESIAN_POINT('Ctrl Pts',(0.24677402236281,4.70166555117323,391.854237472933));
#52442=CARTESIAN_POINT('Ctrl Pts',(2.45933168720454,4.01475329572239,391.775109597473));
#52443=CARTESIAN_POINT('Ctrl Pts',(4.07640342983146,2.35573586177663,391.695981722014));
#52444=CARTESIAN_POINT('Ctrl Pts',(4.70644244793312,0.126316497321376,391.616853846553));
#52445=CARTESIAN_POINT('Ctrl Pts',(4.19689535976046,-2.13368828848624,391.537725971094));
#52446=CARTESIAN_POINT('Ctrl Pts',(2.67114044701949,-3.87705623966156,391.458598095634));
#52447=CARTESIAN_POINT('Ctrl Pts',(0.498613673152825,-4.68166004512793,
391.379470220174));
#52448=CARTESIAN_POINT('Ctrl Pts',(-1.79464403933883,-4.35267838752966,
391.300342344714));
#52449=CARTESIAN_POINT('Ctrl Pts',(-3.65335879596438,-2.96976865785062,
391.221214469255));
#52450=CARTESIAN_POINT('Ctrl Pts',(-4.62747399120691,-0.867779254134205,
391.142086593794));
#52451=CARTESIAN_POINT('Ctrl Pts',(-4.4811239675789,1.4443283423073,391.062958718335));
#52452=CARTESIAN_POINT('Ctrl Pts',(-3.24974492884238,3.40671605371881,390.983830842875));
#52453=CARTESIAN_POINT('Ctrl Pts',(-1.23149465757426,4.54422460729751,390.904702967416));
#52454=CARTESIAN_POINT('Ctrl Pts',(1.08494139143324,4.58142538413069,390.825575091955));
#52455=CARTESIAN_POINT('Ctrl Pts',(3.1386770782293,3.50931084000835,390.746447216496));
#52456=CARTESIAN_POINT('Ctrl Pts',(4.43243474978322,1.58747553118664,390.667319341036));
#52457=CARTESIAN_POINT('Ctrl Pts',(4.65295268374329,-0.718740353708034,
390.588191465577));
#52458=CARTESIAN_POINT('Ctrl Pts',(3.74683616074228,-2.85092531606077,390.509063590117));
#52459=CARTESIAN_POINT('Ctrl Pts',(1.93348610020102,-4.29280652644998,390.429935714657));
#52460=CARTESIAN_POINT('Ctrl Pts',(-0.348025192701879,-4.69525663179842,
390.350807839197));
#52461=CARTESIAN_POINT('Ctrl Pts',(-2.54526802197775,-3.96082908865047,
390.271679963737));
#52462=CARTESIAN_POINT('Ctrl Pts',(-4.12621688682536,-2.2673532093786,390.192552088278));
#52463=CARTESIAN_POINT('Ctrl Pts',(-4.70807153396599,-0.0248757765959869,
390.113424212818));
#52464=CARTESIAN_POINT('Ctrl Pts',(-4.14994561897114,2.22362490829375,390.034296337358));
#52465=CARTESIAN_POINT('Ctrl Pts',(-2.58697997173855,3.93371211440616,389.955168461898));
#52466=CARTESIAN_POINT('Ctrl Pts',(-0.397620511000842,4.69131690492484,
389.876040586439));
#52467=CARTESIAN_POINT('Ctrl Pts',(1.88801608791904,4.31299798573579,389.796912710978));
#52468=CARTESIAN_POINT('Ctrl Pts',(3.71650125536658,2.89035893827407,389.717784835519));
#52469=CARTESIAN_POINT('Ctrl Pts',(4.64509797385908,0.767867948577403,389.638656960059));
#52470=CARTESIAN_POINT('Ctrl Pts',(4.44896212165639,-1.54054938683214,389.559529084599));
#52471=CARTESIAN_POINT('Ctrl Pts',(3.17558470594392,-3.47594852501834,389.480401209139));
#52472=CARTESIAN_POINT('Ctrl Pts',(1.13329271192188,-4.56970502355534,389.40127333368));
#52473=CARTESIAN_POINT('Ctrl Pts',(-1.18340710566026,-4.55698408988609,
389.32214545822));
#52474=CARTESIAN_POINT('Ctrl Pts',(-3.21356473971502,-3.44086588475379,
389.24301758276));
#52475=CARTESIAN_POINT('Ctrl Pts',(-4.46561156725167,-1.49159971293583,
389.1638897073));
#52476=CARTESIAN_POINT('Ctrl Pts',(-4.63638544725815,0.818832313514199,
389.084761831841));
#52477=CARTESIAN_POINT('Ctrl Pts',(-3.6845363487667,2.93099782801338,389.00563395638));
#52478=CARTESIAN_POINT('Ctrl Pts',(-1.84053856736483,4.33347137468852,388.926506080921));
#52479=CARTESIAN_POINT('Ctrl Pts',(0.449114760160199,4.6866675053185,388.847378205461));
#52480=CARTESIAN_POINT('Ctrl Pts',(2.63002248068729,3.90506570037965,388.768250330001));
#52481=CARTESIAN_POINT('Ctrl Pts',(4.1741143660401,2.17791772857007,388.689122454542));
#52482=CARTESIAN_POINT('Ctrl Pts',(4.70751446239035,-0.0765764950091339,
388.609994579082));
#52483=CARTESIAN_POINT('Ctrl Pts',(4.10106888214441,-2.31252900459844,388.530866703622));
#52484=CARTESIAN_POINT('Ctrl Pts',(2.5016182517638,-3.98854139951492,388.451738828162));
#52485=CARTESIAN_POINT('Ctrl Pts',(0.296442716755053,-4.6987953869992,388.372610952703));
#52486=CARTESIAN_POINT('Ctrl Pts',(-1.98051145042811,-4.27131487576429,
388.293483077243));
#52487=CARTESIAN_POINT('Ctrl Pts',(-3.77791798536176,-2.80960710226223,
388.214355201783));
#52488=CARTESIAN_POINT('Ctrl Pts',(-4.66056504020173,-0.667600089313645,
388.135227326323));
#52489=CARTESIAN_POINT('Ctrl Pts',(-4.41473443363227,1.63605508883523,388.056099450863));
#52490=CARTESIAN_POINT('Ctrl Pts',(-3.09994992417011,3.54356696576203,387.976971575404));
#52491=CARTESIAN_POINT('Ctrl Pts',(-1.03456453032195,4.59306353165313,387.897843699944));
#52492=CARTESIAN_POINT('Ctrl Pts',(1.28132331369787,4.53042679435133,387.818715824484));
#52493=CARTESIAN_POINT('Ctrl Pts',(3.28696020658222,3.37082318930362,387.739587949024));
#52494=CARTESIAN_POINT('Ctrl Pts',(4.49671481157362,1.39503128157636,387.660460073565));
#52495=CARTESIAN_POINT('Ctrl Pts',(4.61766534005973,-0.918544054693783,
387.581332198105));
#52496=CARTESIAN_POINT('Ctrl Pts',(3.6205256500481,-3.00970935316784,387.502204322645));
#52497=CARTESIAN_POINT('Ctrl Pts',(1.74673639428721,-4.37212400808516,387.423076447185));
#52498=CARTESIAN_POINT('Ctrl Pts',(-0.549995784557234,-4.67590216002981,
387.343948571725));
#52499=CARTESIAN_POINT('Ctrl Pts',(-2.71355570823769,-3.84748902421993,
387.264820696266));
#52500=CARTESIAN_POINT('Ctrl Pts',(-4.22007362664152,-2.08747094804379,
387.185692820806));
#52501=CARTESIAN_POINT('Ctrl Pts',(-4.70477149187816,0.177993208894804,
387.106564945346));
#52502=CARTESIAN_POINT('Ctrl Pts',(-4.05028784482536,2.40035929545185,387.027437069887));
#52503=CARTESIAN_POINT('Ctrl Pts',(-2.41509492416788,4.04151863542169,386.948309194426));
#52504=CARTESIAN_POINT('Ctrl Pts',(-0.195127271563123,4.70409201877413,
386.869181318967));
#52505=CARTESIAN_POINT('Ctrl Pts',(2.0720871773402,4.22764841285371,386.790053443507));
#52506=CARTESIAN_POINT('Ctrl Pts',(3.83758046755327,2.72755064632278,386.710925568048));
#52507=CARTESIAN_POINT('Ctrl Pts',(4.67386800821896,0.567022234969233,386.631797692587));
#52508=CARTESIAN_POINT('Ctrl Pts',(4.37845679687603,-1.73080110096229,386.552669817128));
#52509=CARTESIAN_POINT('Ctrl Pts',(3.02287570396291,-3.60953997783552,386.473541941668));
#52510=CARTESIAN_POINT('Ctrl Pts',(0.935355956463039,-4.61428928524331,
386.394414066208));
#52511=CARTESIAN_POINT('Ctrl Pts',(-1.37864454889126,-4.50176582920686,
386.315286190748));
#52512=CARTESIAN_POINT('Ctrl Pts',(-3.35882939819794,-3.29921527745666,
386.236158315289));
#52513=CARTESIAN_POINT('Ctrl Pts',(-4.52573004019154,-1.29781507793296,
386.157030439828));
#52514=CARTESIAN_POINT('Ctrl Pts',(-4.59680105468898,1.01782927684972,386.077902564369));
#52515=CARTESIAN_POINT('Ctrl Pts',(-3.55483378747301,3.08702334241943,385.998774688909));
#52516=CARTESIAN_POINT('Ctrl Pts',(-1.65212313730168,4.40874647858035,385.91964681345));
#52517=CARTESIAN_POINT('Ctrl Pts',(0.650621422548117,4.66296559473944,385.84051893799));
#52518=CARTESIAN_POINT('Ctrl Pts',(2.79582891660295,3.78812579546785,385.76139106253));
#52519=CARTESIAN_POINT('Ctrl Pts',(4.26407332779252,1.99605486608223,385.68226318707));
#52520=CARTESIAN_POINT('Ctrl Pts',(4.69984389610718,-0.279327272972474,
385.603135311611));
#52521=CARTESIAN_POINT('Ctrl Pts',(3.99762608680683,-2.48707499751891,385.52400743615));
#52522=CARTESIAN_POINT('Ctrl Pts',(2.32745016540729,-4.09261922254535,385.444879560691));
#52523=CARTESIAN_POINT('Ctrl Pts',(0.0937212204902381,-4.70720434079847,
385.365751685231));
#52524=CARTESIAN_POINT('Ctrl Pts',(-2.16270074615507,-4.18201887319778,
385.286623809771));
#52525=CARTESIAN_POINT('Ctrl Pts',(-3.89546099811616,-2.64422767275401,
385.207495934311));
#52526=CARTESIAN_POINT('Ctrl Pts',(-4.6850007007776,-0.466181088114491,
385.128368058852));
#52527=CARTESIAN_POINT('Ctrl Pts',(-4.34014605663549,1.82474342861496,385.049240183392));
#52528=CARTESIAN_POINT('Ctrl Pts',(-2.94439783415696,3.67383692716674,384.970112307932));
#52529=CARTESIAN_POINT('Ctrl Pts',(-0.83571305710034,4.63337242830686,384.890984432472));
#52530=CARTESIAN_POINT('Ctrl Pts',(1.47532562085691,4.47101450295627,384.811856557013));
#52531=CARTESIAN_POINT('Ctrl Pts',(3.42913894264361,3.22607539980813,384.732728681553));
#52532=CARTESIAN_POINT('Ctrl Pts',(4.55264378010221,1.19999624361863,384.653600806093));
#52533=CARTESIAN_POINT('Ctrl Pts',(4.57380227931992,-1.11664187763583,384.574472930633));
#52534=CARTESIAN_POINT('Ctrl Pts',(3.4874912645637,-3.1629038955988,384.495345055174));
#52535=CARTESIAN_POINT('Ctrl Pts',(1.55674272936248,-4.44332178080534,384.416217179713));
#52536=CARTESIAN_POINT('Ctrl Pts',(-0.750944949374648,-4.64786381644416,
384.337089304254));
#52537=CARTESIAN_POINT('Ctrl Pts',(-2.87680390283758,-3.72700357899221,
384.257961428794));
#52538=CARTESIAN_POINT('Ctrl Pts',(-4.30609303856287,-1.90371193105537,
384.178833553335));
#52539=CARTESIAN_POINT('Ctrl Pts',(-4.69273396316942,0.380531633531783,
384.099705677874));
#52540=CARTESIAN_POINT('Ctrl Pts',(-3.94310806118005,2.5726358450156,384.020577802415));
#52541=CARTESIAN_POINT('Ctrl Pts',(-2.23872467266656,4.14181943271266,383.941449926955));
#52542=CARTESIAN_POINT('Ctrl Pts',(0.00772834932661786,4.70813090788891,
383.862322051495));
#52543=CARTESIAN_POINT('Ctrl Pts',(2.2523100811437,4.13444744452999,383.783194176035));
#52544=CARTESIAN_POINT('Ctrl Pts',(3.9515327006614,2.55967687195196,383.704066300576));
#52545=CARTESIAN_POINT('Ctrl Pts',(4.69395794849557,0.365123473577542,383.624938425116));
#52546=CARTESIAN_POINT('Ctrl Pts',(4.29982000221476,-1.91783845038001,383.545810549656));
#52547=CARTESIAN_POINT('Ctrl Pts',(2.86455275536081,-3.73642795795088,383.466682674196));
#52548=CARTESIAN_POINT('Ctrl Pts',(0.735682100664791,-4.65030409972978,
383.387554798737));
#52549=CARTESIAN_POINT('Ctrl Pts',(-1.571321636466,-4.43818709474668,383.308426923276));
#52550=CARTESIAN_POINT('Ctrl Pts',(-3.49785619221092,-3.15143751831031,
383.229299047817));
#52551=CARTESIAN_POINT('Ctrl Pts',(-4.57744353411293,-1.10162020007351,
383.150171172357));
#52552=CARTESIAN_POINT('Ctrl Pts',(-4.54867969326092,1.21493597416402,383.071043296898));
#52553=CARTESIAN_POINT('Ctrl Pts',(-3.41852935131432,3.23731577814161,382.991915421438));
#52554=CARTESIAN_POINT('Ctrl Pts',(-1.46063945964488,4.47583385997855,382.912787545978));
#52555=CARTESIAN_POINT('Ctrl Pts',(0.850919780561573,4.6306038375412,382.833659670518));
#52556=CARTESIAN_POINT('Ctrl Pts',(2.95644306681562,3.66415075643457,382.754531795058));
#52557=CARTESIAN_POINT('Ctrl Pts',(4.3461132474158,1.81048502171076,382.675403919598));
#52558=CARTESIAN_POINT('Ctrl Pts',(4.68344499450879,-0.481559297088858,
382.596276044139));
#52559=CARTESIAN_POINT('Ctrl Pts',(3.88675908298024,-2.65700210840579,382.517148168679));
#52560=CARTESIAN_POINT('Ctrl Pts',(2.14895964496101,-4.18909642017598,382.438020293219));
#52561=CARTESIAN_POINT('Ctrl Pts',(-0.109174330542496,-4.70687128980098,
382.358892417759));
#52562=CARTESIAN_POINT('Ctrl Pts',(-2.34087357288517,-4.08495621628556,
382.2797645423));
#52563=CARTESIAN_POINT('Ctrl Pts',(-4.00576953871563,-2.47393750444512,
382.20063666684));
#52564=CARTESIAN_POINT('Ctrl Pts',(-4.7007355921423,-0.263896316701532,
382.12150879138));
#52565=CARTESIAN_POINT('Ctrl Pts',(-4.25749735871386,2.01004293828431,382.04238091592));
#52566=CARTESIAN_POINT('Ctrl Pts',(-2.78337754303629,3.79728400651352,381.963253040461));
#52567=CARTESIAN_POINT('Ctrl Pts',(-0.635309535778666,4.66507643741782,
381.884125165001));
#52568=CARTESIAN_POINT('Ctrl Pts',(1.6665880206908,4.40329884773815,381.804997289541));
#52569=CARTESIAN_POINT('Ctrl Pts',(3.56494923856197,3.07533629050199,381.725869414081));
#52570=CARTESIAN_POINT('Ctrl Pts',(4.60011778664443,1.00273262747343,381.646741538621));
#52571=CARTESIAN_POINT('Ctrl Pts',(4.52144496199587,-1.31266592430991,381.567613663161));
#52572=CARTESIAN_POINT('Ctrl Pts',(3.34798006967052,-3.31022443744999,381.488485787702));
#52573=CARTESIAN_POINT('Ctrl Pts',(1.36385795297921,-4.50626761936056,381.409357912242));
#52574=CARTESIAN_POINT('Ctrl Pts',(-0.950499493547971,-4.6111936725719,
381.330230036783));
#52575=CARTESIAN_POINT('Ctrl Pts',(-3.03470942869027,-3.59959651303038,
381.251102161322));
#52576=CARTESIAN_POINT('Ctrl Pts',(-4.38411537126835,-1.71641742726257,
381.171974285863));
#52577=CARTESIAN_POINT('Ctrl Pts',(-4.67198130338802,0.582363352208024,
381.092846410403));
#52578=CARTESIAN_POINT('Ctrl Pts',(-3.82860531743164,2.74013461284959,381.013718534943));
#52579=CARTESIAN_POINT('Ctrl Pts',(-2.05819676400615,4.23442823222176,380.934590659483));
#52580=CARTESIAN_POINT('Ctrl Pts',(0.210569617479083,4.70342607142888,380.855462784024));
#52581=CARTESIAN_POINT('Ctrl Pts',(2.42835009758821,4.03356816934405,380.776334908564));
#52582=CARTESIAN_POINT('Ctrl Pts',(4.05814632781095,2.38704938266401,380.697207033104));
#52583=CARTESIAN_POINT('Ctrl Pts',(4.70533048456991,0.162546621555695,380.618079157644));
#52584=CARTESIAN_POINT('Ctrl Pts',(4.2131977783341,-2.10131407786716,380.538951282185));
#52585=CARTESIAN_POINT('Ctrl Pts',(2.7009098902828,-3.85637681480619,380.459823406725));
#52586=CARTESIAN_POINT('Ctrl Pts',(0.53464196968763,-4.67768258194704,380.380695531265));
#52587=CARTESIAN_POINT('Ctrl Pts',(-1.76108053730214,-4.36636596202583,
380.301567655805));
#52588=CARTESIAN_POINT('Ctrl Pts',(-3.63038692754518,-2.99780705341609,
380.222439780345));
#52589=CARTESIAN_POINT('Ctrl Pts',(-4.62065600907807,-0.903379443519156,
380.143311904886));
#52590=CARTESIAN_POINT('Ctrl Pts',(-4.49211073176741,1.40978634790602,380.064184029426));
#52591=CARTESIAN_POINT('Ctrl Pts',(-3.27587617866081,3.38159601893615,379.985056153966));
#52592=CARTESIAN_POINT('Ctrl Pts',(-1.26644314913044,4.53460892726404,379.905928278506));
#52593=CARTESIAN_POINT('Ctrl Pts',(1.049637849243,4.58964233450045,379.826800403046));
#52594=CARTESIAN_POINT('Ctrl Pts',(3.11156664606508,3.53337082405704,379.747672527587));
#52595=CARTESIAN_POINT('Ctrl Pts',(4.42008176412018,1.62155282729066,379.668544652127));
#52596=CARTESIAN_POINT('Ctrl Pts',(4.65834821288585,-0.682896991284513,
379.589416776667));
#52597=CARTESIAN_POINT('Ctrl Pts',(3.76867376779785,-2.82199475639389,379.510288901207));
#52598=CARTESIAN_POINT('Ctrl Pts',(1.96647817486303,-4.27779381936408,379.431161025748));
#52599=CARTESIAN_POINT('Ctrl Pts',(-0.311867127997482,-4.69779685253383,
379.352033150288));
#52600=CARTESIAN_POINT('Ctrl Pts',(-2.51469903618647,-3.9803071653586,379.272905274828));
#52601=CARTESIAN_POINT('Ctrl Pts',(-4.1086387471793,-2.29905285245449,379.193777399368));
#52602=CARTESIAN_POINT('Ctrl Pts',(-4.70774049217468,-0.0611214491085228,
379.114649523908));
#52603=CARTESIAN_POINT('Ctrl Pts',(-4.16694183125235,2.19160948806155,379.035521648449));
#52604=CARTESIAN_POINT('Ctrl Pts',(-2.61718809033458,3.91367894352783,378.956393772989));
#52605=CARTESIAN_POINT('Ctrl Pts',(-0.433726146618794,4.68811667974907,
378.877265897529));
#52606=CARTESIAN_POINT('Ctrl Pts',(1.85475530941073,4.32740558711739,378.798138022069));
#52607=CARTESIAN_POINT('Ctrl Pts',(3.69413887366186,2.91888580717067,378.71901014661));
#52608=CARTESIAN_POINT('Ctrl Pts',(4.63904866464471,0.803606782114387,378.63988227115));
#52609=CARTESIAN_POINT('Ctrl Pts',(4.46069062370475,-1.50625214781415,378.56075439569));
#52610=CARTESIAN_POINT('Ctrl Pts',(3.20225115918455,-3.45139738174314,378.48162652023));
#52611=CARTESIAN_POINT('Ctrl Pts',(1.16844028192984,-4.56084462361588,378.40249864477));
#52612=CARTESIAN_POINT('Ctrl Pts',(-1.14828881349689,-4.56595983052853,
378.323370769311));
#52613=CARTESIAN_POINT('Ctrl Pts',(-3.18697903086916,-3.46550444091513,
378.244242893851));
#52614=CARTESIAN_POINT('Ctrl Pts',(-4.45399572524721,-1.5259352714587,378.165115018391));
#52615=CARTESIAN_POINT('Ctrl Pts',(-4.64255205342532,0.783113532278959,
378.085987142931));
#52616=CARTESIAN_POINT('Ctrl Pts',(-3.7069922628433,2.90254452789652,378.006859267472));
#52617=CARTESIAN_POINT('Ctrl Pts',(-1.8738464663689,4.31917304511859,377.927731392012));
#52618=CARTESIAN_POINT('Ctrl Pts',(0.413019825360475,4.68998624700131,377.848603516552));
#52619=CARTESIAN_POINT('Ctrl Pts',(2.59988029319979,3.92519793567579,377.769475641092));
#52620=CARTESIAN_POINT('Ctrl Pts',(4.15722335104551,2.20998877434347,377.690347765632));
#52621=CARTESIAN_POINT('Ctrl Pts',(4.70796449588766,-0.0403321046239016,
377.611219890173));
#52622=CARTESIAN_POINT('Ctrl Pts',(4.11875099606982,-2.28088724087274,377.532092014713));
#52623=CARTESIAN_POINT('Ctrl Pts',(2.53225101877986,-3.9691637848658,377.452964139253));
#52624=CARTESIAN_POINT('Ctrl Pts',(0.332608926075814,-4.69637388582909,
377.373836263793));
#52625=CARTESIAN_POINT('Ctrl Pts',(-1.94756883984043,-4.28643581396986,
377.294708388333));
#52626=CARTESIAN_POINT('Ctrl Pts',(-3.75617547417524,-2.83860919825332,
377.215580512874));
#52627=CARTESIAN_POINT('Ctrl Pts',(-4.65528721285309,-0.703460971943434,
377.136452637414));
#52628=CARTESIAN_POINT('Ctrl Pts',(-4.42719922749879,1.60201853086424,377.057324761954));
#52629=CARTESIAN_POINT('Ctrl Pts',(-3.12713919846579,3.51959611413589,376.978196886494));
#52630=CARTESIAN_POINT('Ctrl Pts',(-1.06989485827222,4.58496252606164,376.899069011035));
#52631=CARTESIAN_POINT('Ctrl Pts',(1.24640657847665,4.54015715746168,376.819941135575));
#52632=CARTESIAN_POINT('Ctrl Pts',(3.26091156592763,3.39602887682211,376.740813260115));
#52633=CARTESIAN_POINT('Ctrl Pts',(4.48584150695881,1.4296091591174,376.661685384655));
#52634=CARTESIAN_POINT('Ctrl Pts',(4.62460015982963,-0.882966440516176,
376.582557509196));
#52635=CARTESIAN_POINT('Ctrl Pts',(3.64358944392086,-2.9817465244189,376.503429633736));
#52636=CARTESIAN_POINT('Ctrl Pts',(1.7803446513398,-4.35854669589912,376.424301758276));
#52637=CARTESIAN_POINT('Ctrl Pts',(-0.513980740029185,-4.67999788047178,
376.345173882816));
#52638=CARTESIAN_POINT('Ctrl Pts',(-2.68385431544624,-3.86826607229696,
376.266046007356));
#52639=CARTESIAN_POINT('Ctrl Pts',(-4.20387757931463,-2.11989849939269,
376.186918131897));
#52640=CARTESIAN_POINT('Ctrl Pts',(-4.7060023921165,0.141766919500427,376.107790256437));
#52641=CARTESIAN_POINT('Ctrl Pts',(-4.0686476489454,2.36910590400946,376.028662380977));
#52642=CARTESIAN_POINT('Ctrl Pts',(-2.44613811739875,4.02280552584175,375.949534505517));
#52643=CARTESIAN_POINT('Ctrl Pts',(-0.231337257081005,4.70245046971741,
375.870406630058));
#52644=CARTESIAN_POINT('Ctrl Pts',(2.03947802286674,4.24347544716049,375.791278754597));
#52645=CARTESIAN_POINT('Ctrl Pts',(3.81646794076225,2.75701496679917,375.712150879138));
#52646=CARTESIAN_POINT('Ctrl Pts',(4.66936407560377,0.602987532497468,375.633023003678));
#52647=CARTESIAN_POINT('Ctrl Pts',(4.39165217497973,-1.6970389500669,375.553895128218));
#52648=CARTESIAN_POINT('Ctrl Pts',(3.05057500604089,-3.58616494858208,375.474767252759));
#52649=CARTESIAN_POINT('Ctrl Pts',(0.970853006392586,-4.60694213867371,
375.395639377299));
#52650=CARTESIAN_POINT('Ctrl Pts',(-1.34394626652729,-4.51226606546036,
375.316511501839));
#52651=CARTESIAN_POINT('Ctrl Pts',(-3.33332776428957,-3.32493525307769,
375.23738362638));
#52652=CARTESIAN_POINT('Ctrl Pts',(-4.51560361732968,-1.33271151243227,
375.158255750919));
#52653=CARTESIAN_POINT('Ctrl Pts',(-4.60446635415931,0.982571567271653,
375.07912787546));
#52654=CARTESIAN_POINT('Ctrl Pts',(-3.92033033613572,2.36677696691101,375.026375958487));
#52655=CARTESIAN_POINT('Ctrl Pts',(-3.43378788736318,2.93584158412846,375.));
#52656=CARTESIAN_POINT('Ctrl Pts',(-4.51766328535307,-0.00011344722995056,
399.112583302492));
#52657=CARTESIAN_POINT('Ctrl Pts',(-4.51713673458649,0.545949625983492,
399.093346914919));
#52658=CARTESIAN_POINT('Ctrl Pts',(-4.41799450573444,1.09219871675483,399.074110527346));
#52659=CARTESIAN_POINT('Ctrl Pts',(-4.22436256903118,1.60260114106826,399.054874139773));
#52660=CARTESIAN_POINT('Ctrl Pts',(-3.95886428330821,2.3024390448317,399.028498181286));
#52661=CARTESIAN_POINT('Ctrl Pts',(-3.51572059597365,2.93488341331845,399.002122222799));
#52662=CARTESIAN_POINT('Ctrl Pts',(-2.94858141451404,3.42336635011963,398.975746264313));
#52663=CARTESIAN_POINT('Ctrl Pts',(-2.38144223305443,3.91184928692081,398.949370305826));
#52664=CARTESIAN_POINT('Ctrl Pts',(-1.69030755746978,4.25637079203641,398.92299434734));
#52665=CARTESIAN_POINT('Ctrl Pts',(-0.958850722305057,4.4152208122577,398.896618388853));
#52666=CARTESIAN_POINT('Ctrl Pts',(-0.227393887140339,4.57407083247899,
398.870242430366));
#52667=CARTESIAN_POINT('Ctrl Pts',(0.544385107604448,4.54724936780597,398.84386647188));
#52668=CARTESIAN_POINT('Ctrl Pts',(1.26304959160632,4.33800360262792,398.817490513393));
#52669=CARTESIAN_POINT('Ctrl Pts',(1.98171407560819,4.12875783744988,398.791114554907));
#52670=CARTESIAN_POINT('Ctrl Pts',(2.64726404886714,3.73708777176682,398.76473859642));
#52671=CARTESIAN_POINT('Ctrl Pts',(3.1791236295575,3.21041157417997,398.738362637933));
#52672=CARTESIAN_POINT('Ctrl Pts',(3.71098321024786,2.68373537659312,398.711986679447));
#52673=CARTESIAN_POINT('Ctrl Pts',(4.10915239836962,2.02205304710248,398.68561072096));
#52674=CARTESIAN_POINT('Ctrl Pts',(4.32542619827246,1.30547222526591,398.659234762474));
#52675=CARTESIAN_POINT('Ctrl Pts',(4.5416999981753,0.588891403429356,398.632858803987));
#52676=CARTESIAN_POINT('Ctrl Pts',(4.57607840985923,-0.182587910753133,
398.6064828455));
#52677=CARTESIAN_POINT('Ctrl Pts',(4.42439935544928,-0.915565328667223,
398.580106887014));
#52678=CARTESIAN_POINT('Ctrl Pts',(4.27272030103931,-1.64854274658133,398.553730928527));
#52679=CARTESIAN_POINT('Ctrl Pts',(3.93498378053545,-2.34301826822704,398.527354970041));
#52680=CARTESIAN_POINT('Ctrl Pts',(3.45207841102396,-2.91491409337733,398.500979011554));
#52681=CARTESIAN_POINT('Ctrl Pts',(2.96917304151247,-3.48680991852761,398.474603053068));
#52682=CARTESIAN_POINT('Ctrl Pts',(2.34109882299336,-3.93612604718246,398.448227094581));
#52683=CARTESIAN_POINT('Ctrl Pts',(1.64389457471586,-4.20846529685206,398.421851136094));
#52684=CARTESIAN_POINT('Ctrl Pts',(0.946690326438348,-4.48080454652167,
398.395475177608));
#52685=CARTESIAN_POINT('Ctrl Pts',(0.180356048402448,-4.57616691720601,
398.369099219121));
#52686=CARTESIAN_POINT('Ctrl Pts',(-0.562330762839376,-4.483007209538,398.342723260635));
#52687=CARTESIAN_POINT('Ctrl Pts',(-1.3050175740812,-4.38984750186999,398.316347302148));
#52688=CARTESIAN_POINT('Ctrl Pts',(-2.02405691852894,-4.10816571584963,
398.289971343661));
#52689=CARTESIAN_POINT('Ctrl Pts',(-2.63239713711321,-3.67206411165684,
398.263595385175));
#52690=CARTESIAN_POINT('Ctrl Pts',(-3.24073735569747,-3.23596250746405,
398.237219426688));
#52691=CARTESIAN_POINT('Ctrl Pts',(-3.73837844841825,-2.64544108509883,
398.210843468202));
#52692=CARTESIAN_POINT('Ctrl Pts',(-4.0650726929841,-1.97199227390868,398.184467509715));
#52693=CARTESIAN_POINT('Ctrl Pts',(-4.36186009740405,-1.36019354158502,
398.160506107307));
#52694=CARTESIAN_POINT('Ctrl Pts',(-4.51756632872819,-0.679955446831048,
398.1365447049));
#52695=CARTESIAN_POINT('Ctrl Pts',(-4.51805439081064,6.66898104614677E-5,
398.112583302492));
#52696=CARTESIAN_POINT('Ctrl Pts',(-1.31303618635555,-4.90075024188347,
400.));
#52697=CARTESIAN_POINT('Ctrl Pts',(-1.45291589482402,-4.85500689927294,
400.));
#52698=CARTESIAN_POINT('Ctrl Pts',(-1.59044602699472,-4.80315746369625,
400.));
#52699=CARTESIAN_POINT('Ctrl Pts',(-1.72529743087534,-4.74548509357023,
400.));
#52700=CARTESIAN_POINT('Ctrl Pts',(-1.86151474898354,-4.68722855814354,
400.));
#52701=CARTESIAN_POINT('Ctrl Pts',(-1.99499946782598,-4.62303013629637,
400.));
#52702=CARTESIAN_POINT('Ctrl Pts',(-2.12539163452376,-4.55313283560557,
400.));
#52703=CARTESIAN_POINT('Ctrl Pts',(-2.25520494367751,-4.48354583407488,
400.));
#52704=CARTESIAN_POINT('Ctrl Pts',(-2.38195370500541,-4.40830995570903,
400.));
#52705=CARTESIAN_POINT('Ctrl Pts',(-2.50525282411489,-4.32762357969483,
400.));
#52706=CARTESIAN_POINT('Ctrl Pts',(-2.6270809920476,-4.24789978736008,400.));
#52707=CARTESIAN_POINT('Ctrl Pts',(-2.74554186145885,-4.1628542844716,400.));
#52708=CARTESIAN_POINT('Ctrl Pts',(-2.86022634881304,-4.07264517835143,
400.));
#52709=CARTESIAN_POINT('Ctrl Pts',(-2.90206457395326,-4.03973585487948,
400.));
#52710=CARTESIAN_POINT('Ctrl Pts',(-2.94339980617641,-4.00613903342865,
400.));
#52711=CARTESIAN_POINT('Ctrl Pts',(-2.98421070502804,-3.97186145992605,
400.));
#52712=CARTESIAN_POINT('Ctrl Pts',(-3.00176471409307,-3.95711763283762,
400.));
#52713=CARTESIAN_POINT('Ctrl Pts',(-3.01922333710064,-3.94224634426854,
400.));
#52714=CARTESIAN_POINT('Ctrl Pts',(-3.0365678292172,-3.92726308267954,400.));
#52715=CARTESIAN_POINT('Ctrl Pts',(-3.14698675201001,-3.83187628245151,
400.));
#52716=CARTESIAN_POINT('Ctrl Pts',(-3.25293553514171,-3.73182827889012,
400.));
#52717=CARTESIAN_POINT('Ctrl Pts',(-3.35406834590596,-3.62734196551097,
400.));
#52718=CARTESIAN_POINT('Ctrl Pts',(-3.36860939901959,-3.61231873990287,
400.));
#52719=CARTESIAN_POINT('Ctrl Pts',(-3.3830508320319,-3.59720369462607,400.));
#52720=CARTESIAN_POINT('Ctrl Pts',(-3.3973915556082,-3.58199742790278,400.));
#52721=CARTESIAN_POINT('Ctrl Pts',(-3.49724054898418,-3.4761219874308,400.));
#52722=CARTESIAN_POINT('Ctrl Pts',(-3.59221081092533,-3.36582685075802,
400.));
#52723=CARTESIAN_POINT('Ctrl Pts',(-3.68210185106465,-3.25150412359693,
400.));
#52724=CARTESIAN_POINT('Ctrl Pts',(-3.77205159485829,-3.13710673758391,
400.));
#52725=CARTESIAN_POINT('Ctrl Pts',(-3.85691583765602,-3.01867577562728,
400.));
#52726=CARTESIAN_POINT('Ctrl Pts',(-3.93644802914845,-2.89657936297904,
400.));
#52727=CARTESIAN_POINT('Ctrl Pts',(-4.00696577927717,-2.78832176115549,
400.));
#52728=CARTESIAN_POINT('Ctrl Pts',(-4.07329120966267,-2.67718185514111,
400.));
#52729=CARTESIAN_POINT('Ctrl Pts',(-4.13521902572865,-2.56340683612714,
400.));
#52730=CARTESIAN_POINT('Ctrl Pts',(-4.14927174249539,-2.53758890455934,
400.));
#52731=CARTESIAN_POINT('Ctrl Pts',(-4.16309787710306,-2.511635261477,400.));
#52732=CARTESIAN_POINT('Ctrl Pts',(-4.17669478808166,-2.48554876582588,
400.));
#52733=CARTESIAN_POINT('Ctrl Pts',(-4.18567658693009,-2.46831664178184,
400.));
#52734=CARTESIAN_POINT('Ctrl Pts',(-4.19455855900594,-2.45102602806576,
400.));
#52735=CARTESIAN_POINT('Ctrl Pts',(-4.20333295387386,-2.43369188245622,
400.));
#52736=CARTESIAN_POINT('Ctrl Pts',(-4.26826574456287,-2.30541472311025,
400.));
#52737=CARTESIAN_POINT('Ctrl Pts',(-4.32740788322074,-2.17457173953832,
400.));
#52738=CARTESIAN_POINT('Ctrl Pts',(-4.38057216155237,-2.04153956135574,
400.));
#52739=CARTESIAN_POINT('Ctrl Pts',(-4.43343069026291,-1.90927245587513,
400.));
#52740=CARTESIAN_POINT('Ctrl Pts',(-4.48038018757078,-1.77484054207341,
400.));
#52741=CARTESIAN_POINT('Ctrl Pts',(-4.52118875294636,-1.63859604986007,
400.));
#52742=CARTESIAN_POINT('Ctrl Pts',(-4.53639547739945,-1.58782650105892,
400.));
#52743=CARTESIAN_POINT('Ctrl Pts',(-4.55074898869301,-1.53680513764063,
400.));
#52744=CARTESIAN_POINT('Ctrl Pts',(-4.56423545493657,-1.48554984951531,
400.));
#52745=CARTESIAN_POINT('Ctrl Pts',(-4.60065397684761,-1.34714132945246,
400.));
#52746=CARTESIAN_POINT('Ctrl Pts',(-4.63075368245775,-1.20702677925683,
400.));
#52747=CARTESIAN_POINT('Ctrl Pts',(-4.65449674508562,-1.06564398750406,
400.));
#52748=CARTESIAN_POINT('Ctrl Pts',(-4.6677938749007,-0.986463581630512,
400.));
#52749=CARTESIAN_POINT('Ctrl Pts',(-4.67909632529634,-0.906885415400295,
400.));
#52750=CARTESIAN_POINT('Ctrl Pts',(-4.68839036132626,-0.826987472477294,
400.));
#52751=CARTESIAN_POINT('Ctrl Pts',(-4.69350021378828,-0.783059656936131,
400.));
#52752=CARTESIAN_POINT('Ctrl Pts',(-4.69800287543295,-0.73903519996531,
400.));
#52753=CARTESIAN_POINT('Ctrl Pts',(-4.70189541038099,-0.69492725727482,
400.));
#52754=CARTESIAN_POINT('Ctrl Pts',(-4.70335699391325,-0.678365442534775,
400.));
#52755=CARTESIAN_POINT('Ctrl Pts',(-4.70473233460286,-0.661793969471143,
400.));
#52756=CARTESIAN_POINT('Ctrl Pts',(-4.70602072340745,-0.645222510455179,
400.));
#52757=CARTESIAN_POINT('Ctrl Pts',(-4.71697947907218,-0.504269275129255,
400.));
#52758=CARTESIAN_POINT('Ctrl Pts',(-4.72166837458957,-0.363132695636631,
400.));
#52759=CARTESIAN_POINT('Ctrl Pts',(-4.7201177742283,-0.222235244668839,
400.));
#52760=CARTESIAN_POINT('Ctrl Pts',(-4.71856870881553,-0.0814772689241232,
400.));
#52761=CARTESIAN_POINT('Ctrl Pts',(-4.71079242396856,0.0590428483946887,
400.));
#52762=CARTESIAN_POINT('Ctrl Pts',(-4.69676735600276,0.19890200600945,400.));
#52763=CARTESIAN_POINT('Ctrl Pts',(-4.68295624998761,0.33662751705272,400.));
#52764=CARTESIAN_POINT('Ctrl Pts',(-4.66308539592085,0.473712790055481,
400.));
#52765=CARTESIAN_POINT('Ctrl Pts',(-4.63708587274883,0.609740845579473,
400.));
#52766=CARTESIAN_POINT('Ctrl Pts',(-4.62194193613231,0.6889730775437,400.));
#52767=CARTESIAN_POINT('Ctrl Pts',(-4.60471782759541,0.767846329349665,
400.));
#52768=CARTESIAN_POINT('Ctrl Pts',(-4.58539250818854,0.846274698465189,
400.));
#52769=CARTESIAN_POINT('Ctrl Pts',(-4.57105296447468,0.904469184344614,
400.));
#52770=CARTESIAN_POINT('Ctrl Pts',(-4.55555640760633,0.962418671522469,
400.));
#52771=CARTESIAN_POINT('Ctrl Pts',(-4.53891410477628,1.02009082935325,400.));
#52772=CARTESIAN_POINT('Ctrl Pts',(-4.53055828962656,1.04904703181158,400.));
#52773=CARTESIAN_POINT('Ctrl Pts',(-4.52191362534324,1.07793330641511,400.));
#52774=CARTESIAN_POINT('Ctrl Pts',(-4.51298141319226,1.1067454537709,400.));
#52775=CARTESIAN_POINT('Ctrl Pts',(-4.50751626468392,1.12437408388872,400.));
#52776=CARTESIAN_POINT('Ctrl Pts',(-4.50194375351087,1.14197390912326,400.));
#52777=CARTESIAN_POINT('Ctrl Pts',(-4.49626740324529,1.15953444897625,400.));
#52778=CARTESIAN_POINT('Ctrl Pts',(-4.45341464273149,1.29210512795207,400.));
#52779=CARTESIAN_POINT('Ctrl Pts',(-4.4046021744809,1.42258699257377,400.));
#52780=CARTESIAN_POINT('Ctrl Pts',(-4.35004408840361,1.55060321390413,400.));
#52781=CARTESIAN_POINT('Ctrl Pts',(-4.29958883856276,1.66899245545036,400.));
#52782=CARTESIAN_POINT('Ctrl Pts',(-4.24421884943669,1.7852731960868,400.));
#52783=CARTESIAN_POINT('Ctrl Pts',(-4.18406982393872,1.89912668839153,400.));
#52784=CARTESIAN_POINT('Ctrl Pts',(-4.15968128005935,1.94529070966877,400.));
#52785=CARTESIAN_POINT('Ctrl Pts',(-4.13450669520302,1.99105541062324,400.));
#52786=CARTESIAN_POINT('Ctrl Pts',(-4.10855377241811,2.03639833327113,400.));
#52787=CARTESIAN_POINT('Ctrl Pts',(-4.09598731345164,2.05835347033207,400.));
#52788=CARTESIAN_POINT('Ctrl Pts',(-4.08323760980602,2.0802109712186,400.));
#52789=CARTESIAN_POINT('Ctrl Pts',(-4.07030781226104,2.10196429342508,400.));
#52790=CARTESIAN_POINT('Ctrl Pts',(-3.9998914613058,2.22043401931249,400.));
#52791=CARTESIAN_POINT('Ctrl Pts',(-3.92427608656828,2.33558378339706,400.));
#52792=CARTESIAN_POINT('Ctrl Pts',(-3.84364635340467,2.44703278518893,400.));
#52793=CARTESIAN_POINT('Ctrl Pts',(-3.76407407271829,2.55702014226977,400.));
#52794=CARTESIAN_POINT('Ctrl Pts',(-3.67961761227173,2.66340373121656,400.));
#52795=CARTESIAN_POINT('Ctrl Pts',(-3.59041821150276,2.76578232711007,400.));
#52796=CARTESIAN_POINT('Ctrl Pts',(-3.56727357293573,2.79234658178586,400.));
#52797=CARTESIAN_POINT('Ctrl Pts',(-3.5438094445685,2.81864098904491,400.));
#52798=CARTESIAN_POINT('Ctrl Pts',(-3.52002794801113,2.84465807439287,400.));
#52799=CARTESIAN_POINT('Ctrl Pts',(-3.49182454546321,2.87551274871592,400.));
#52800=CARTESIAN_POINT('Ctrl Pts',(-3.46317478144493,2.90597739162215,400.));
#52801=CARTESIAN_POINT('Ctrl Pts',(-3.43408816619831,2.93604416807489,400.));
#52802=CARTESIAN_POINT('Origin',(0.,0.,387.));
#52803=CARTESIAN_POINT('Origin',(0.,0.,374.));
#52804=CARTESIAN_POINT('',(-4.,-4.89858719658941E-16,374.));
#52805=CARTESIAN_POINT('Origin',(0.,0.,374.));
#52806=CARTESIAN_POINT('Origin',(-17.,5.,0.));
#52807=CARTESIAN_POINT('',(-16.,5.,400.));
#52808=CARTESIAN_POINT('',(-17.,4.,400.));
#52809=CARTESIAN_POINT('Origin',(-17.,5.,400.));
#52810=CARTESIAN_POINT('',(-17.,4.,0.));
#52811=CARTESIAN_POINT('',(-17.,4.,0.));
#52812=CARTESIAN_POINT('',(-16.,5.,0.));
#52813=CARTESIAN_POINT('Origin',(-17.,5.,0.));
#52814=CARTESIAN_POINT('',(-16.,5.,0.));
#52815=CARTESIAN_POINT('Origin',(-20.,4.,0.));
#52816=CARTESIAN_POINT('',(-19.,4.,400.));
#52817=CARTESIAN_POINT('',(-16.,4.,400.));
#52818=CARTESIAN_POINT('',(-19.,4.,0.));
#52819=CARTESIAN_POINT('',(-19.,4.,0.));
#52820=CARTESIAN_POINT('',(-16.,4.,0.));
#52821=CARTESIAN_POINT('Origin',(0.,0.,400.));
#52822=CARTESIAN_POINT('',(-16.,6.,400.));
#52823=CARTESIAN_POINT('',(-16.,7.,400.));
#52824=CARTESIAN_POINT('',(-15.,7.,400.));
#52825=CARTESIAN_POINT('Origin',(-15.,6.,400.));
#52826=CARTESIAN_POINT('',(-9.,7.,400.));
#52827=CARTESIAN_POINT('',(-8.,7.,400.));
#52828=CARTESIAN_POINT('',(-8.,6.,400.));
#52829=CARTESIAN_POINT('Origin',(-9.,6.,400.));
#52830=CARTESIAN_POINT('',(-8.,-6.,400.));
#52831=CARTESIAN_POINT('',(-8.,-7.,400.));
#52832=CARTESIAN_POINT('',(-9.,-7.,400.));
#52833=CARTESIAN_POINT('Origin',(-9.,-6.,400.));
#52834=CARTESIAN_POINT('',(-15.,-7.,400.));
#52835=CARTESIAN_POINT('',(-16.,-7.,400.));
#52836=CARTESIAN_POINT('',(-16.,-6.,400.));
#52837=CARTESIAN_POINT('Origin',(-15.,-6.,400.));
#52838=CARTESIAN_POINT('',(-16.,-5.,400.));
#52839=CARTESIAN_POINT('',(-16.,-4.,400.));
#52840=CARTESIAN_POINT('',(-17.,-4.,400.));
#52841=CARTESIAN_POINT('Origin',(-17.,-5.,400.));
#52842=CARTESIAN_POINT('',(-19.,-4.,400.));
#52843=CARTESIAN_POINT('',(-20.,-4.,400.));
#52844=CARTESIAN_POINT('',(-20.,-5.,400.));
#52845=CARTESIAN_POINT('Origin',(-19.,-5.,400.));
#52846=CARTESIAN_POINT('',(-20.,-19.,400.));
#52847=CARTESIAN_POINT('',(-20.,-20.,400.));
#52848=CARTESIAN_POINT('',(-19.,-20.,400.));
#52849=CARTESIAN_POINT('Origin',(-19.,-19.,400.));
#52850=CARTESIAN_POINT('',(-5.,-20.,400.));
#52851=CARTESIAN_POINT('',(-4.,-20.,400.));
#52852=CARTESIAN_POINT('',(-4.,-19.,400.));
#52853=CARTESIAN_POINT('Origin',(-5.,-19.,400.));
#52854=CARTESIAN_POINT('',(-4.,-17.,400.));
#52855=CARTESIAN_POINT('',(-4.,-16.,400.));
#52856=CARTESIAN_POINT('',(-5.,-16.,400.));
#52857=CARTESIAN_POINT('Origin',(-5.,-17.,400.));
#52858=CARTESIAN_POINT('',(-6.,-16.,400.));
#52859=CARTESIAN_POINT('',(-7.,-16.,400.));
#52860=CARTESIAN_POINT('',(-7.,-15.,400.));
#52861=CARTESIAN_POINT('Origin',(-6.,-15.,400.));
#52862=CARTESIAN_POINT('',(-7.,-9.,400.));
#52863=CARTESIAN_POINT('',(-7.,-8.,400.));
#52864=CARTESIAN_POINT('',(-6.,-8.,400.));
#52865=CARTESIAN_POINT('Origin',(-6.,-9.,400.));
#52866=CARTESIAN_POINT('',(6.,-8.,400.));
#52867=CARTESIAN_POINT('',(7.,-8.,400.));
#52868=CARTESIAN_POINT('',(7.,-9.,400.));
#52869=CARTESIAN_POINT('Origin',(6.,-9.,400.));
#52870=CARTESIAN_POINT('',(7.,-15.,400.));
#52871=CARTESIAN_POINT('',(7.,-16.,400.));
#52872=CARTESIAN_POINT('',(6.,-16.,400.));
#52873=CARTESIAN_POINT('Origin',(6.,-15.,400.));
#52874=CARTESIAN_POINT('',(5.,-16.,400.));
#52875=CARTESIAN_POINT('',(4.,-16.,400.));
#52876=CARTESIAN_POINT('',(4.,-17.,400.));
#52877=CARTESIAN_POINT('Origin',(5.,-17.,400.));
#52878=CARTESIAN_POINT('',(4.,-19.,400.));
#52879=CARTESIAN_POINT('',(4.,-20.,400.));
#52880=CARTESIAN_POINT('',(5.,-20.,400.));
#52881=CARTESIAN_POINT('Origin',(5.,-19.,400.));
#52882=CARTESIAN_POINT('',(19.,-20.,400.));
#52883=CARTESIAN_POINT('',(20.,-20.,400.));
#52884=CARTESIAN_POINT('',(20.,-19.,400.));
#52885=CARTESIAN_POINT('Origin',(19.,-19.,400.));
#52886=CARTESIAN_POINT('',(20.,-5.,400.));
#52887=CARTESIAN_POINT('',(20.,-4.,400.));
#52888=CARTESIAN_POINT('',(19.,-4.,400.));
#52889=CARTESIAN_POINT('Origin',(19.,-5.,400.));
#52890=CARTESIAN_POINT('',(17.,-4.,400.));
#52891=CARTESIAN_POINT('',(16.,-4.,400.));
#52892=CARTESIAN_POINT('',(16.,-5.,400.));
#52893=CARTESIAN_POINT('Origin',(17.,-5.,400.));
#52894=CARTESIAN_POINT('',(16.,-6.,400.));
#52895=CARTESIAN_POINT('',(16.,-7.,400.));
#52896=CARTESIAN_POINT('',(15.,-7.,400.));
#52897=CARTESIAN_POINT('Origin',(15.,-6.,400.));
#52898=CARTESIAN_POINT('',(9.,-7.,400.));
#52899=CARTESIAN_POINT('',(8.,-7.,400.));
#52900=CARTESIAN_POINT('',(8.,-6.,400.));
#52901=CARTESIAN_POINT('Origin',(9.,-6.,400.));
#52902=CARTESIAN_POINT('',(8.,6.,400.));
#52903=CARTESIAN_POINT('',(8.,7.,400.));
#52904=CARTESIAN_POINT('',(9.,7.,400.));
#52905=CARTESIAN_POINT('Origin',(9.,6.,400.));
#52906=CARTESIAN_POINT('',(15.,7.,400.));
#52907=CARTESIAN_POINT('',(16.,7.,400.));
#52908=CARTESIAN_POINT('',(16.,6.,400.));
#52909=CARTESIAN_POINT('Origin',(15.,6.,400.));
#52910=CARTESIAN_POINT('',(16.,5.,400.));
#52911=CARTESIAN_POINT('',(16.,4.,400.));
#52912=CARTESIAN_POINT('',(17.,4.,400.));
#52913=CARTESIAN_POINT('Origin',(17.,5.,400.));
#52914=CARTESIAN_POINT('',(19.,4.,400.));
#52915=CARTESIAN_POINT('',(20.,4.,400.));
#52916=CARTESIAN_POINT('',(20.,5.,400.));
#52917=CARTESIAN_POINT('Origin',(19.,5.,400.));
#52918=CARTESIAN_POINT('',(20.,19.,400.));
#52919=CARTESIAN_POINT('',(20.,20.,400.));
#52920=CARTESIAN_POINT('',(19.,20.,400.));
#52921=CARTESIAN_POINT('Origin',(19.,19.,400.));
#52922=CARTESIAN_POINT('',(5.,20.,400.));
#52923=CARTESIAN_POINT('',(4.,20.,400.));
#52924=CARTESIAN_POINT('',(4.,19.,400.));
#52925=CARTESIAN_POINT('Origin',(5.,19.,400.));
#52926=CARTESIAN_POINT('',(4.,17.,400.));
#52927=CARTESIAN_POINT('',(4.,16.,400.));
#52928=CARTESIAN_POINT('',(5.,16.,400.));
#52929=CARTESIAN_POINT('Origin',(5.,17.,400.));
#52930=CARTESIAN_POINT('',(6.,16.,400.));
#52931=CARTESIAN_POINT('',(7.,16.,400.));
#52932=CARTESIAN_POINT('',(7.,15.,400.));
#52933=CARTESIAN_POINT('Origin',(6.,15.,400.));
#52934=CARTESIAN_POINT('',(7.,9.,400.));
#52935=CARTESIAN_POINT('',(7.,8.,400.));
#52936=CARTESIAN_POINT('',(6.,8.,400.));
#52937=CARTESIAN_POINT('Origin',(6.,9.,400.));
#52938=CARTESIAN_POINT('',(-6.,8.,400.));
#52939=CARTESIAN_POINT('',(-7.,8.,400.));
#52940=CARTESIAN_POINT('',(-7.,9.,400.));
#52941=CARTESIAN_POINT('Origin',(-6.,9.,400.));
#52942=CARTESIAN_POINT('',(-7.,15.,400.));
#52943=CARTESIAN_POINT('',(-7.,16.,400.));
#52944=CARTESIAN_POINT('',(-6.,16.,400.));
#52945=CARTESIAN_POINT('Origin',(-6.,15.,400.));
#52946=CARTESIAN_POINT('',(-5.,16.,400.));
#52947=CARTESIAN_POINT('',(-4.,16.,400.));
#52948=CARTESIAN_POINT('',(-4.,17.,400.));
#52949=CARTESIAN_POINT('Origin',(-5.,17.,400.));
#52950=CARTESIAN_POINT('',(-4.,19.,400.));
#52951=CARTESIAN_POINT('',(-4.,20.,400.));
#52952=CARTESIAN_POINT('',(-5.,20.,400.));
#52953=CARTESIAN_POINT('Origin',(-5.,19.,400.));
#52954=CARTESIAN_POINT('',(-19.,20.,400.));
#52955=CARTESIAN_POINT('',(-20.,20.,400.));
#52956=CARTESIAN_POINT('',(-20.,19.,400.));
#52957=CARTESIAN_POINT('Origin',(-19.,19.,400.));
#52958=CARTESIAN_POINT('',(-20.,5.,400.));
#52959=CARTESIAN_POINT('',(-20.,4.,400.));
#52960=CARTESIAN_POINT('Origin',(-19.,5.,400.));
#52961=CARTESIAN_POINT('',(-15.,-12.,400.));
#52962=CARTESIAN_POINT('Origin',(-12.,-12.,400.));
#52963=CARTESIAN_POINT('',(-15.,12.,400.));
#52964=CARTESIAN_POINT('Origin',(-12.,12.,400.));
#52965=CARTESIAN_POINT('',(9.,12.,400.));
#52966=CARTESIAN_POINT('Origin',(12.,12.,400.));
#52967=CARTESIAN_POINT('',(9.,-12.,400.));
#52968=CARTESIAN_POINT('Origin',(12.,-12.,400.));
#52969=CARTESIAN_POINT('Origin',(-15.,6.,0.));
#52970=CARTESIAN_POINT('',(-16.,6.,0.));
#52971=CARTESIAN_POINT('',(-15.,7.,0.));
#52972=CARTESIAN_POINT('Origin',(-15.,6.,0.));
#52973=CARTESIAN_POINT('',(-15.,7.,0.));
#52974=CARTESIAN_POINT('',(-16.,6.,0.));
#52975=CARTESIAN_POINT('Origin',(-16.,7.,0.));
#52976=CARTESIAN_POINT('',(-9.,7.,0.));
#52977=CARTESIAN_POINT('',(-8.,7.,0.));
#52978=CARTESIAN_POINT('',(-9.,7.,0.));
#52979=CARTESIAN_POINT('Origin',(-9.,6.,0.));
#52980=CARTESIAN_POINT('',(-8.,6.,0.));
#52981=CARTESIAN_POINT('Origin',(-9.,6.,0.));
#52982=CARTESIAN_POINT('',(-8.,6.,0.));
#52983=CARTESIAN_POINT('Origin',(-8.,7.,0.));
#52984=CARTESIAN_POINT('',(-8.,-6.,0.));
#52985=CARTESIAN_POINT('',(-8.,-7.,0.));
#52986=CARTESIAN_POINT('',(-8.,-6.,0.));
#52987=CARTESIAN_POINT('Origin',(-9.,-6.,0.));
#52988=CARTESIAN_POINT('',(-9.,-7.,0.));
#52989=CARTESIAN_POINT('Origin',(-9.,-6.,0.));
#52990=CARTESIAN_POINT('',(-9.,-7.,0.));
#52991=CARTESIAN_POINT('Origin',(-8.,-7.,0.));
#52992=CARTESIAN_POINT('',(-15.,-7.,0.));
#52993=CARTESIAN_POINT('',(-16.,-7.,0.));
#52994=CARTESIAN_POINT('',(-15.,-7.,0.));
#52995=CARTESIAN_POINT('Origin',(-15.,-6.,0.));
#52996=CARTESIAN_POINT('',(-16.,-6.,0.));
#52997=CARTESIAN_POINT('Origin',(-15.,-6.,0.));
#52998=CARTESIAN_POINT('',(-16.,-6.,0.));
#52999=CARTESIAN_POINT('Origin',(-16.,-7.,0.));
#53000=CARTESIAN_POINT('',(-16.,-5.,0.));
#53001=CARTESIAN_POINT('',(-16.,-4.,0.));
#53002=CARTESIAN_POINT('',(-16.,-5.,0.));
#53003=CARTESIAN_POINT('Origin',(-17.,-5.,0.));
#53004=CARTESIAN_POINT('',(-17.,-4.,0.));
#53005=CARTESIAN_POINT('Origin',(-17.,-5.,0.));
#53006=CARTESIAN_POINT('',(-17.,-4.,0.));
#53007=CARTESIAN_POINT('Origin',(-19.,-5.,0.));
#53008=CARTESIAN_POINT('',(-19.,-4.,0.));
#53009=CARTESIAN_POINT('',(-19.,-4.,0.));
#53010=CARTESIAN_POINT('',(-20.,-5.,0.));
#53011=CARTESIAN_POINT('Origin',(-19.,-5.,0.));
#53012=CARTESIAN_POINT('',(-20.,-5.,0.));
#53013=CARTESIAN_POINT('Origin',(-20.,-4.,0.));
#53014=CARTESIAN_POINT('',(-20.,-19.,0.));
#53015=CARTESIAN_POINT('',(-20.,-20.,0.));
#53016=CARTESIAN_POINT('',(-20.,-19.,0.));
#53017=CARTESIAN_POINT('Origin',(-19.,-19.,0.));
#53018=CARTESIAN_POINT('',(-19.,-20.,0.));
#53019=CARTESIAN_POINT('Origin',(-19.,-19.,0.));
#53020=CARTESIAN_POINT('',(-19.,-20.,0.));
#53021=CARTESIAN_POINT('Origin',(-5.,-19.,0.));
#53022=CARTESIAN_POINT('',(-5.,-20.,0.));
#53023=CARTESIAN_POINT('',(-5.,-20.,0.));
#53024=CARTESIAN_POINT('',(-4.,-19.,0.));
#53025=CARTESIAN_POINT('Origin',(-5.,-19.,0.));
#53026=CARTESIAN_POINT('',(-4.,-19.,0.));
#53027=CARTESIAN_POINT('Origin',(-4.,-20.,0.));
#53028=CARTESIAN_POINT('',(-4.,-17.,0.));
#53029=CARTESIAN_POINT('',(-4.,-16.,0.));
#53030=CARTESIAN_POINT('',(-4.,-17.,0.));
#53031=CARTESIAN_POINT('Origin',(-5.,-17.,0.));
#53032=CARTESIAN_POINT('',(-5.,-16.,0.));
#53033=CARTESIAN_POINT('Origin',(-5.,-17.,0.));
#53034=CARTESIAN_POINT('',(-5.,-16.,0.));
#53035=CARTESIAN_POINT('Origin',(-6.,-15.,0.));
#53036=CARTESIAN_POINT('',(-6.,-16.,0.));
#53037=CARTESIAN_POINT('',(-7.,-15.,0.));
#53038=CARTESIAN_POINT('Origin',(-6.,-15.,0.));
#53039=CARTESIAN_POINT('',(-7.,-15.,0.));
#53040=CARTESIAN_POINT('',(-6.,-16.,0.));
#53041=CARTESIAN_POINT('Origin',(-7.,-16.,0.));
#53042=CARTESIAN_POINT('',(-7.,-9.,0.));
#53043=CARTESIAN_POINT('',(-7.,-8.,0.));
#53044=CARTESIAN_POINT('',(-7.,-9.,0.));
#53045=CARTESIAN_POINT('Origin',(-6.,-9.,0.));
#53046=CARTESIAN_POINT('',(-6.,-8.,0.));
#53047=CARTESIAN_POINT('Origin',(-6.,-9.,0.));
#53048=CARTESIAN_POINT('',(-6.,-8.,0.));
#53049=CARTESIAN_POINT('Origin',(-7.,-8.,0.));
#53050=CARTESIAN_POINT('',(6.,-8.,0.));
#53051=CARTESIAN_POINT('',(7.,-8.,0.));
#53052=CARTESIAN_POINT('',(6.,-8.,0.));
#53053=CARTESIAN_POINT('Origin',(6.,-9.,0.));
#53054=CARTESIAN_POINT('',(7.,-9.,0.));
#53055=CARTESIAN_POINT('Origin',(6.,-9.,0.));
#53056=CARTESIAN_POINT('',(7.,-9.,0.));
#53057=CARTESIAN_POINT('Origin',(7.,-8.,0.));
#53058=CARTESIAN_POINT('',(7.,-15.,0.));
#53059=CARTESIAN_POINT('',(7.,-16.,0.));
#53060=CARTESIAN_POINT('',(7.,-15.,0.));
#53061=CARTESIAN_POINT('Origin',(6.,-15.,0.));
#53062=CARTESIAN_POINT('',(6.,-16.,0.));
#53063=CARTESIAN_POINT('Origin',(6.,-15.,0.));
#53064=CARTESIAN_POINT('',(6.,-16.,0.));
#53065=CARTESIAN_POINT('Origin',(7.,-16.,0.));
#53066=CARTESIAN_POINT('',(5.,-16.,0.));
#53067=CARTESIAN_POINT('',(4.,-16.,0.));
#53068=CARTESIAN_POINT('',(5.,-16.,0.));
#53069=CARTESIAN_POINT('Origin',(5.,-17.,0.));
#53070=CARTESIAN_POINT('',(4.,-17.,0.));
#53071=CARTESIAN_POINT('Origin',(5.,-17.,0.));
#53072=CARTESIAN_POINT('',(4.,-17.,0.));
#53073=CARTESIAN_POINT('Origin',(5.,-19.,0.));
#53074=CARTESIAN_POINT('',(4.,-19.,0.));
#53075=CARTESIAN_POINT('',(4.,-19.,0.));
#53076=CARTESIAN_POINT('',(5.,-20.,0.));
#53077=CARTESIAN_POINT('Origin',(5.,-19.,0.));
#53078=CARTESIAN_POINT('',(5.,-20.,0.));
#53079=CARTESIAN_POINT('Origin',(4.,-20.,0.));
#53080=CARTESIAN_POINT('',(19.,-20.,0.));
#53081=CARTESIAN_POINT('',(20.,-20.,0.));
#53082=CARTESIAN_POINT('',(19.,-20.,0.));
#53083=CARTESIAN_POINT('Origin',(19.,-19.,0.));
#53084=CARTESIAN_POINT('',(20.,-19.,0.));
#53085=CARTESIAN_POINT('Origin',(19.,-19.,0.));
#53086=CARTESIAN_POINT('',(20.,-19.,0.));
#53087=CARTESIAN_POINT('Origin',(19.,-5.,0.));
#53088=CARTESIAN_POINT('',(20.,-5.,0.));
#53089=CARTESIAN_POINT('',(20.,-5.,0.));
#53090=CARTESIAN_POINT('',(19.,-4.,0.));
#53091=CARTESIAN_POINT('Origin',(19.,-5.,0.));
#53092=CARTESIAN_POINT('',(19.,-4.,0.));
#53093=CARTESIAN_POINT('Origin',(20.,-4.,0.));
#53094=CARTESIAN_POINT('',(17.,-4.,0.));
#53095=CARTESIAN_POINT('',(16.,-4.,0.));
#53096=CARTESIAN_POINT('',(17.,-4.,0.));
#53097=CARTESIAN_POINT('Origin',(17.,-5.,0.));
#53098=CARTESIAN_POINT('',(16.,-5.,0.));
#53099=CARTESIAN_POINT('Origin',(17.,-5.,0.));
#53100=CARTESIAN_POINT('',(16.,-5.,0.));
#53101=CARTESIAN_POINT('Origin',(15.,-6.,0.));
#53102=CARTESIAN_POINT('',(16.,-6.,0.));
#53103=CARTESIAN_POINT('',(15.,-7.,0.));
#53104=CARTESIAN_POINT('Origin',(15.,-6.,0.));
#53105=CARTESIAN_POINT('',(15.,-7.,0.));
#53106=CARTESIAN_POINT('',(16.,-6.,0.));
#53107=CARTESIAN_POINT('Origin',(16.,-7.,0.));
#53108=CARTESIAN_POINT('',(9.,-7.,0.));
#53109=CARTESIAN_POINT('',(8.,-7.,0.));
#53110=CARTESIAN_POINT('',(9.,-7.,0.));
#53111=CARTESIAN_POINT('Origin',(9.,-6.,0.));
#53112=CARTESIAN_POINT('',(8.,-6.,0.));
#53113=CARTESIAN_POINT('Origin',(9.,-6.,0.));
#53114=CARTESIAN_POINT('',(8.,-6.,0.));
#53115=CARTESIAN_POINT('Origin',(8.,-7.,0.));
#53116=CARTESIAN_POINT('',(8.,6.,0.));
#53117=CARTESIAN_POINT('',(8.,7.,0.));
#53118=CARTESIAN_POINT('',(8.,6.,0.));
#53119=CARTESIAN_POINT('Origin',(9.,6.,0.));
#53120=CARTESIAN_POINT('',(9.,7.,0.));
#53121=CARTESIAN_POINT('Origin',(9.,6.,0.));
#53122=CARTESIAN_POINT('',(9.,7.,0.));
#53123=CARTESIAN_POINT('Origin',(8.,7.,0.));
#53124=CARTESIAN_POINT('',(15.,7.,0.));
#53125=CARTESIAN_POINT('',(16.,7.,0.));
#53126=CARTESIAN_POINT('',(15.,7.,0.));
#53127=CARTESIAN_POINT('Origin',(15.,6.,0.));
#53128=CARTESIAN_POINT('',(16.,6.,0.));
#53129=CARTESIAN_POINT('Origin',(15.,6.,0.));
#53130=CARTESIAN_POINT('',(16.,6.,0.));
#53131=CARTESIAN_POINT('Origin',(16.,7.,0.));
#53132=CARTESIAN_POINT('',(16.,5.,0.));
#53133=CARTESIAN_POINT('',(16.,4.,0.));
#53134=CARTESIAN_POINT('',(16.,5.,0.));
#53135=CARTESIAN_POINT('Origin',(17.,5.,0.));
#53136=CARTESIAN_POINT('',(17.,4.,0.));
#53137=CARTESIAN_POINT('Origin',(17.,5.,0.));
#53138=CARTESIAN_POINT('',(17.,4.,0.));
#53139=CARTESIAN_POINT('Origin',(19.,5.,0.));
#53140=CARTESIAN_POINT('',(19.,4.,0.));
#53141=CARTESIAN_POINT('',(19.,4.,0.));
#53142=CARTESIAN_POINT('',(20.,5.,0.));
#53143=CARTESIAN_POINT('Origin',(19.,5.,0.));
#53144=CARTESIAN_POINT('',(20.,5.,0.));
#53145=CARTESIAN_POINT('Origin',(20.,4.,0.));
#53146=CARTESIAN_POINT('',(20.,19.,0.));
#53147=CARTESIAN_POINT('',(20.,20.,0.));
#53148=CARTESIAN_POINT('',(20.,19.,0.));
#53149=CARTESIAN_POINT('Origin',(19.,19.,0.));
#53150=CARTESIAN_POINT('',(19.,20.,0.));
#53151=CARTESIAN_POINT('Origin',(19.,19.,0.));
#53152=CARTESIAN_POINT('',(19.,20.,0.));
#53153=CARTESIAN_POINT('Origin',(5.,19.,0.));
#53154=CARTESIAN_POINT('',(5.,20.,0.));
#53155=CARTESIAN_POINT('',(5.,20.,0.));
#53156=CARTESIAN_POINT('',(4.,19.,0.));
#53157=CARTESIAN_POINT('Origin',(5.,19.,0.));
#53158=CARTESIAN_POINT('',(4.,19.,0.));
#53159=CARTESIAN_POINT('Origin',(4.,20.,0.));
#53160=CARTESIAN_POINT('',(4.,17.,0.));
#53161=CARTESIAN_POINT('',(4.,16.,0.));
#53162=CARTESIAN_POINT('',(4.,17.,0.));
#53163=CARTESIAN_POINT('Origin',(5.,17.,0.));
#53164=CARTESIAN_POINT('',(5.,16.,0.));
#53165=CARTESIAN_POINT('Origin',(5.,17.,0.));
#53166=CARTESIAN_POINT('',(5.,16.,0.));
#53167=CARTESIAN_POINT('Origin',(6.,15.,0.));
#53168=CARTESIAN_POINT('',(6.,16.,0.));
#53169=CARTESIAN_POINT('',(7.,15.,0.));
#53170=CARTESIAN_POINT('Origin',(6.,15.,0.));
#53171=CARTESIAN_POINT('',(7.,15.,0.));
#53172=CARTESIAN_POINT('',(6.,16.,0.));
#53173=CARTESIAN_POINT('Origin',(7.,16.,0.));
#53174=CARTESIAN_POINT('',(7.,9.,0.));
#53175=CARTESIAN_POINT('',(7.,8.,0.));
#53176=CARTESIAN_POINT('',(7.,9.,0.));
#53177=CARTESIAN_POINT('Origin',(6.,9.,0.));
#53178=CARTESIAN_POINT('',(6.,8.,0.));
#53179=CARTESIAN_POINT('Origin',(6.,9.,0.));
#53180=CARTESIAN_POINT('',(6.,8.,0.));
#53181=CARTESIAN_POINT('Origin',(7.,8.,0.));
#53182=CARTESIAN_POINT('',(-6.,8.,0.));
#53183=CARTESIAN_POINT('',(-7.,8.,0.));
#53184=CARTESIAN_POINT('',(-6.,8.,0.));
#53185=CARTESIAN_POINT('Origin',(-6.,9.,0.));
#53186=CARTESIAN_POINT('',(-7.,9.,0.));
#53187=CARTESIAN_POINT('Origin',(-6.,9.,0.));
#53188=CARTESIAN_POINT('',(-7.,9.,0.));
#53189=CARTESIAN_POINT('Origin',(-7.,8.,0.));
#53190=CARTESIAN_POINT('',(-7.,15.,0.));
#53191=CARTESIAN_POINT('',(-7.,16.,0.));
#53192=CARTESIAN_POINT('',(-7.,15.,0.));
#53193=CARTESIAN_POINT('Origin',(-6.,15.,0.));
#53194=CARTESIAN_POINT('',(-6.,16.,0.));
#53195=CARTESIAN_POINT('Origin',(-6.,15.,0.));
#53196=CARTESIAN_POINT('',(-6.,16.,0.));
#53197=CARTESIAN_POINT('Origin',(-7.,16.,0.));
#53198=CARTESIAN_POINT('',(-5.,16.,0.));
#53199=CARTESIAN_POINT('',(-4.,16.,0.));
#53200=CARTESIAN_POINT('',(-5.,16.,0.));
#53201=CARTESIAN_POINT('Origin',(-5.,17.,0.));
#53202=CARTESIAN_POINT('',(-4.,17.,0.));
#53203=CARTESIAN_POINT('Origin',(-5.,17.,0.));
#53204=CARTESIAN_POINT('',(-4.,17.,0.));
#53205=CARTESIAN_POINT('Origin',(-5.,19.,0.));
#53206=CARTESIAN_POINT('',(-4.,19.,0.));
#53207=CARTESIAN_POINT('',(-4.,19.,0.));
#53208=CARTESIAN_POINT('',(-5.,20.,0.));
#53209=CARTESIAN_POINT('Origin',(-5.,19.,0.));
#53210=CARTESIAN_POINT('',(-5.,20.,0.));
#53211=CARTESIAN_POINT('Origin',(-4.,20.,0.));
#53212=CARTESIAN_POINT('',(-19.,20.,0.));
#53213=CARTESIAN_POINT('',(-20.,20.,0.));
#53214=CARTESIAN_POINT('',(-19.,20.,0.));
#53215=CARTESIAN_POINT('Origin',(-19.,19.,0.));
#53216=CARTESIAN_POINT('',(-20.,19.,0.));
#53217=CARTESIAN_POINT('Origin',(-19.,19.,0.));
#53218=CARTESIAN_POINT('',(-20.,19.,0.));
#53219=CARTESIAN_POINT('Origin',(-19.,5.,0.));
#53220=CARTESIAN_POINT('',(-20.,5.,0.));
#53221=CARTESIAN_POINT('',(-20.,5.,0.));
#53222=CARTESIAN_POINT('Origin',(-19.,5.,0.));
#53223=CARTESIAN_POINT('Origin',(12.,-12.,0.));
#53224=CARTESIAN_POINT('',(9.,-12.,0.));
#53225=CARTESIAN_POINT('',(9.,-12.,0.));
#53226=CARTESIAN_POINT('Origin',(12.,-12.,0.));
#53227=CARTESIAN_POINT('Origin',(12.,12.,0.));
#53228=CARTESIAN_POINT('',(9.,12.,0.));
#53229=CARTESIAN_POINT('',(9.,12.,0.));
#53230=CARTESIAN_POINT('Origin',(12.,12.,0.));
#53231=CARTESIAN_POINT('Origin',(0.,0.,0.));
#53232=CARTESIAN_POINT('',(-4.,-4.89858719658941E-16,0.));
#53233=CARTESIAN_POINT('Origin',(-12.,12.,0.));
#53234=CARTESIAN_POINT('',(-15.,12.,0.));
#53235=CARTESIAN_POINT('',(-15.,12.,0.));
#53236=CARTESIAN_POINT('Origin',(-12.,12.,0.));
#53237=CARTESIAN_POINT('Origin',(-12.,-12.,0.));
#53238=CARTESIAN_POINT('',(-15.,-12.,0.));
#53239=CARTESIAN_POINT('',(-15.,-12.,0.));
#53240=CARTESIAN_POINT('Origin',(-12.,-12.,0.));
#53241=CARTESIAN_POINT('Origin',(-20.,20.,0.));
#53242=CARTESIAN_POINT('',(-20.,4.,0.));
#53243=CARTESIAN_POINT('Origin',(-4.,16.,0.));
#53244=CARTESIAN_POINT('',(-4.,20.,0.));
#53245=CARTESIAN_POINT('Origin',(4.,16.,0.));
#53246=CARTESIAN_POINT('',(7.,16.,0.));
#53247=CARTESIAN_POINT('Origin',(20.,20.,0.));
#53248=CARTESIAN_POINT('',(4.,20.,0.));
#53249=CARTESIAN_POINT('Origin',(16.,4.,0.));
#53250=CARTESIAN_POINT('',(20.,4.,0.));
#53251=CARTESIAN_POINT('Origin',(16.,-4.,0.));
#53252=CARTESIAN_POINT('',(16.,-7.,0.));
#53253=CARTESIAN_POINT('Origin',(20.,-20.,0.));
#53254=CARTESIAN_POINT('',(20.,-4.,0.));
#53255=CARTESIAN_POINT('Origin',(4.,-16.,0.));
#53256=CARTESIAN_POINT('',(4.,-20.,0.));
#53257=CARTESIAN_POINT('Origin',(-4.,-16.,0.));
#53258=CARTESIAN_POINT('',(-7.,-16.,0.));
#53259=CARTESIAN_POINT('Origin',(-20.,-20.,0.));
#53260=CARTESIAN_POINT('',(-4.,-20.,0.));
#53261=CARTESIAN_POINT('Origin',(-16.,-4.,0.));
#53262=CARTESIAN_POINT('',(-20.,-4.,0.));
#53263=CARTESIAN_POINT('Origin',(-16.,4.,0.));
#53264=CARTESIAN_POINT('',(-16.,7.,0.));
#53265=CARTESIAN_POINT('Origin',(0.,0.,0.));
#97438=UNCERTAINTY_MEASURE_WITH_UNIT(LENGTH_MEASURE(0.01),#97476,
'DISTANCE_ACCURACY_VALUE',
'Maximum model space distance between geometric entities at asserted c
onnectivities');
#97452=UNCERTAINTY_MEASURE_WITH_UNIT(LENGTH_MEASURE(0.01),#97476,
'DISTANCE_ACCURACY_VALUE',
'Maximum model space distance between geometric entities at asserted c
onnectivities');
#97461=(
GEOMETRIC_REPRESENTATION_CONTEXT(3)
GLOBAL_UNCERTAINTY_ASSIGNED_CONTEXT((#97438))
GLOBAL_UNIT_ASSIGNED_CONTEXT((#97476,#97478,#97479))
REPRESENTATION_CONTEXT('','3D')
);
#97475=(
GEOMETRIC_REPRESENTATION_CONTEXT(3)
GLOBAL_UNCERTAINTY_ASSIGNED_CONTEXT((#97452))
GLOBAL_UNIT_ASSIGNED_CONTEXT((#97476,#97478,#97479))
REPRESENTATION_CONTEXT('','3D')
);
#97476=(
LENGTH_UNIT()
NAMED_UNIT(*)
SI_UNIT(.MILLI.,.METRE.)
);
#97478=(
NAMED_UNIT(*)
PLANE_ANGLE_UNIT()
SI_UNIT($,.RADIAN.)
);
#97479=(
NAMED_UNIT(*)
SI_UNIT($,.STERADIAN.)
SOLID_ANGLE_UNIT()
);
#97488=SHAPE_DEFINITION_REPRESENTATION(#97550,#97611);
#97550=PRODUCT_DEFINITION_SHAPE('',$,#97634);
#97611=SHAPE_REPRESENTATION('',(#22297),#97461);
#97625=PRODUCT_DEFINITION_CONTEXT('part definition',#97693,'design');
#97634=PRODUCT_DEFINITION('Leg post','Leg post',#97656,#97625);
#97656=PRODUCT_DEFINITION_FORMATION('',$,#97703);
#97693=APPLICATION_CONTEXT(
'Core Data for Automotive Mechanical Design Process');
#97694=PRODUCT_CONTEXT('part definition',#97693,'mechanical');
#97703=PRODUCT('Leg post','Leg post',
'Independent aluminum extrusion section. Whole-mm nominal die dimensio
ns; parametric saw-cut length. Select structural loading, tolerances a
nd finish for the assembly application.',(#97694));
#97718=PRESENTATION_STYLE_ASSIGNMENT((#97725));
#97725=SURFACE_STYLE_USAGE(.BOTH.,#97732);
#97732=SURFACE_SIDE_STYLE('',(#97739));
#97739=SURFACE_STYLE_FILL_AREA(#97746);
#97746=FILL_AREA_STYLE('Dark blue',(#97753));
#97753=FILL_AREA_STYLE_COLOUR('Dark blue',#97760);
#97760=COLOUR_RGB('Dark blue',0.0901960784313725,0.270588235294118,0.513725490196078);
ENDSEC;
END-ISO-10303-21;
